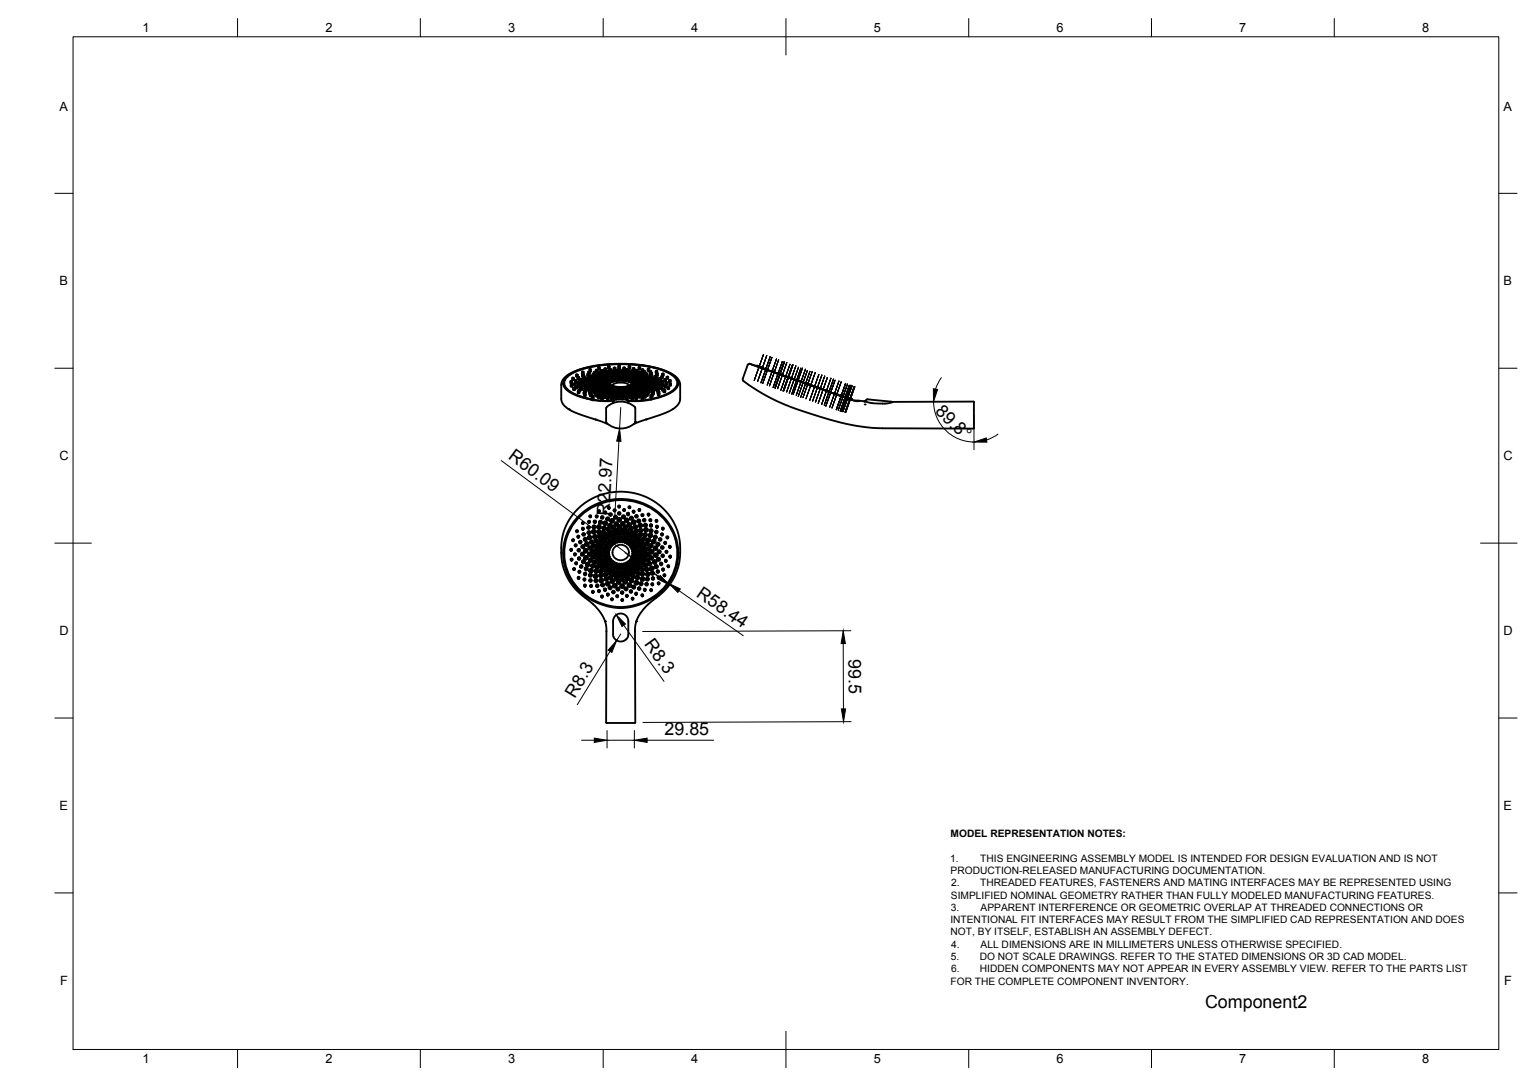
ISO-10303-21;
HEADER;
/* Generated by software containing ST-Developer
 * from STEP Tools, Inc. (www.steptools.com) 
 */

FILE_DESCRIPTION(
/* description */ ('STEP AP214'),
/* implementation_level */ '2;1');

FILE_NAME(
/* name */ 'Component2.step',
/* time_stamp */ '2026-10-06T11:02:40-07:00',
/* author */ (''),
/* organization */ (''),
/* preprocessor_version */ 'ST-DEVELOPER v20.2',
/* originating_system */ 'Autodesk Translation Framework v15.15.0.0',
/* authorisation */ '');

FILE_SCHEMA (('AUTOMOTIVE_DESIGN { 1 0 10303 214 3 1 1 }'));
ENDSEC;

DATA;
#10=MECHANICAL_DESIGN_GEOMETRIC_PRESENTATION_REPRESENTATION('',(#2937),#130910);
#45=B_SPLINE_SURFACE_WITH_KNOTS('',5,5,((#80582,#80583,#80584,#80585,#80586,
#80587),(#80588,#80589,#80590,#80591,#80592,#80593),(#80594,#80595,#80596,
#80597,#80598,#80599),(#80600,#80601,#80602,#80603,#80604,#80605),(#80606,
#80607,#80608,#80609,#80610,#80611),(#80612,#80613,#80614,#80615,#80616,
#80617),(#80618,#80619,#80620,#80621,#80622,#80623),(#80624,#80625,#80626,
#80627,#80628,#80629),(#80630,#80631,#80632,#80633,#80634,#80635),(#80636,
#80637,#80638,#80639,#80640,#80641),(#80642,#80643,#80644,#80645,#80646,
#80647),(#80648,#80649,#80650,#80651,#80652,#80653),(#80654,#80655,#80656,
#80657,#80658,#80659),(#80660,#80661,#80662,#80663,#80664,#80665),(#80666,
#80667,#80668,#80669,#80670,#80671),(#80672,#80673,#80674,#80675,#80676,
#80677),(#80678,#80679,#80680,#80681,#80682,#80683),(#80684,#80685,#80686,
#80687,#80688,#80689),(#80690,#80691,#80692,#80693,#80694,#80695),(#80696,
#80697,#80698,#80699,#80700,#80701),(#80702,#80703,#80704,#80705,#80706,
#80707),(#80708,#80709,#80710,#80711,#80712,#80713)),.UNSPECIFIED.,.F.,
 .F.,.F.,(6,4,4,4,4,6),(6,6),(0.,0.25,0.375,0.5,0.75,1.),(-5.17415755595432E-6,
1.),.UNSPECIFIED.);
#46=B_SPLINE_SURFACE_WITH_KNOTS('',5,5,((#80915,#80916,#80917,#80918,#80919,
#80920),(#80921,#80922,#80923,#80924,#80925,#80926),(#80927,#80928,#80929,
#80930,#80931,#80932),(#80933,#80934,#80935,#80936,#80937,#80938),(#80939,
#80940,#80941,#80942,#80943,#80944),(#80945,#80946,#80947,#80948,#80949,
#80950),(#80951,#80952,#80953,#80954,#80955,#80956),(#80957,#80958,#80959,
#80960,#80961,#80962),(#80963,#80964,#80965,#80966,#80967,#80968),(#80969,
#80970,#80971,#80972,#80973,#80974),(#80975,#80976,#80977,#80978,#80979,
#80980),(#80981,#80982,#80983,#80984,#80985,#80986),(#80987,#80988,#80989,
#80990,#80991,#80992),(#80993,#80994,#80995,#80996,#80997,#80998),(#80999,
#81000,#81001,#81002,#81003,#81004),(#81005,#81006,#81007,#81008,#81009,
#81010),(#81011,#81012,#81013,#81014,#81015,#81016),(#81017,#81018,#81019,
#81020,#81021,#81022),(#81023,#81024,#81025,#81026,#81027,#81028),(#81029,
#81030,#81031,#81032,#81033,#81034),(#81035,#81036,#81037,#81038,#81039,
#81040),(#81041,#81042,#81043,#81044,#81045,#81046)),.UNSPECIFIED.,.F.,
 .F.,.F.,(6,4,4,4,4,6),(6,6),(0.,0.25,0.5,0.625,0.75,1.),(-4.87729692394977E-6,
1.),.UNSPECIFIED.);
#47=B_SPLINE_SURFACE_WITH_KNOTS('',5,5,((#81337,#81338,#81339,#81340,#81341,
#81342),(#81343,#81344,#81345,#81346,#81347,#81348),(#81349,#81350,#81351,
#81352,#81353,#81354),(#81355,#81356,#81357,#81358,#81359,#81360),(#81361,
#81362,#81363,#81364,#81365,#81366),(#81367,#81368,#81369,#81370,#81371,
#81372),(#81373,#81374,#81375,#81376,#81377,#81378),(#81379,#81380,#81381,
#81382,#81383,#81384),(#81385,#81386,#81387,#81388,#81389,#81390),(#81391,
#81392,#81393,#81394,#81395,#81396),(#81397,#81398,#81399,#81400,#81401,
#81402),(#81403,#81404,#81405,#81406,#81407,#81408),(#81409,#81410,#81411,
#81412,#81413,#81414),(#81415,#81416,#81417,#81418,#81419,#81420),(#81421,
#81422,#81423,#81424,#81425,#81426),(#81427,#81428,#81429,#81430,#81431,
#81432),(#81433,#81434,#81435,#81436,#81437,#81438),(#81439,#81440,#81441,
#81442,#81443,#81444),(#81445,#81446,#81447,#81448,#81449,#81450),(#81451,
#81452,#81453,#81454,#81455,#81456),(#81457,#81458,#81459,#81460,#81461,
#81462),(#81463,#81464,#81465,#81466,#81467,#81468),(#81469,#81470,#81471,
#81472,#81473,#81474),(#81475,#81476,#81477,#81478,#81479,#81480),(#81481,
#81482,#81483,#81484,#81485,#81486),(#81487,#81488,#81489,#81490,#81491,
#81492),(#81493,#81494,#81495,#81496,#81497,#81498),(#81499,#81500,#81501,
#81502,#81503,#81504),(#81505,#81506,#81507,#81508,#81509,#81510),(#81511,
#81512,#81513,#81514,#81515,#81516),(#81517,#81518,#81519,#81520,#81521,
#81522),(#81523,#81524,#81525,#81526,#81527,#81528),(#81529,#81530,#81531,
#81532,#81533,#81534),(#81535,#81536,#81537,#81538,#81539,#81540),(#81541,
#81542,#81543,#81544,#81545,#81546),(#81547,#81548,#81549,#81550,#81551,
#81552),(#81553,#81554,#81555,#81556,#81557,#81558),(#81559,#81560,#81561,
#81562,#81563,#81564),(#81565,#81566,#81567,#81568,#81569,#81570),(#81571,
#81572,#81573,#81574,#81575,#81576),(#81577,#81578,#81579,#81580,#81581,
#81582),(#81583,#81584,#81585,#81586,#81587,#81588),(#81589,#81590,#81591,
#81592,#81593,#81594),(#81595,#81596,#81597,#81598,#81599,#81600),(#81601,
#81602,#81603,#81604,#81605,#81606),(#81607,#81608,#81609,#81610,#81611,
#81612)),.UNSPECIFIED.,.F.,.F.,.F.,(6,4,4,4,4,4,4,4,4,4,4,6),(6,6),(0.,
0.0625,0.125,0.25,0.3125,0.375,0.5,0.625,0.6875,0.75,0.875,1.),(0.,1.),
 .UNSPECIFIED.);
#48=B_SPLINE_SURFACE_WITH_KNOTS('',5,5,((#82412,#82413,#82414,#82415,#82416,
#82417),(#82418,#82419,#82420,#82421,#82422,#82423),(#82424,#82425,#82426,
#82427,#82428,#82429),(#82430,#82431,#82432,#82433,#82434,#82435),(#82436,
#82437,#82438,#82439,#82440,#82441),(#82442,#82443,#82444,#82445,#82446,
#82447),(#82448,#82449,#82450,#82451,#82452,#82453),(#82454,#82455,#82456,
#82457,#82458,#82459),(#82460,#82461,#82462,#82463,#82464,#82465),(#82466,
#82467,#82468,#82469,#82470,#82471)),.UNSPECIFIED.,.F.,.F.,.F.,(6,4,6),
(6,6),(0.,0.5,1.),(-3.3767936030343E-7,1.),.UNSPECIFIED.);
#49=B_SPLINE_SURFACE_WITH_KNOTS('',5,5,((#83493,#83494,#83495,#83496,#83497,
#83498),(#83499,#83500,#83501,#83502,#83503,#83504),(#83505,#83506,#83507,
#83508,#83509,#83510),(#83511,#83512,#83513,#83514,#83515,#83516),(#83517,
#83518,#83519,#83520,#83521,#83522),(#83523,#83524,#83525,#83526,#83527,
#83528),(#83529,#83530,#83531,#83532,#83533,#83534),(#83535,#83536,#83537,
#83538,#83539,#83540),(#83541,#83542,#83543,#83544,#83545,#83546),(#83547,
#83548,#83549,#83550,#83551,#83552)),.UNSPECIFIED.,.F.,.F.,.F.,(6,4,6),
(6,6),(0.,0.5,1.),(0.,1.),.UNSPECIFIED.);
#58=SPHERICAL_SURFACE('',#47449,40.9182954767619);
#59=SPHERICAL_SURFACE('',#47518,216.25);
#71=CONICAL_SURFACE('',#47414,8.99091713639496,1.30899693899566);
#72=CONICAL_SURFACE('',#47466,6.3031389659941,0.785398163397445);
#73=CONICAL_SURFACE('',#47469,6.3031389659941,0.785398163397445);
#74=CONICAL_SURFACE('',#47523,22.9751982564137,0.00349065850398867);
#75=CONICAL_SURFACE('',#47530,22.9751982564137,0.00349065850398867);
#83=FACE_BOUND('',#13544,.T.);
#84=FACE_BOUND('',#13545,.T.);
#85=FACE_BOUND('',#13546,.T.);
#86=FACE_BOUND('',#13547,.T.);
#87=FACE_BOUND('',#13548,.T.);
#88=FACE_BOUND('',#13549,.T.);
#89=FACE_BOUND('',#13550,.T.);
#90=FACE_BOUND('',#13551,.T.);
#91=FACE_BOUND('',#13552,.T.);
#92=FACE_BOUND('',#13553,.T.);
#93=FACE_BOUND('',#13554,.T.);
#94=FACE_BOUND('',#13555,.T.);
#95=FACE_BOUND('',#13556,.T.);
#96=FACE_BOUND('',#13557,.T.);
#97=FACE_BOUND('',#13558,.T.);
#98=FACE_BOUND('',#13559,.T.);
#99=FACE_BOUND('',#13560,.T.);
#100=FACE_BOUND('',#13561,.T.);
#101=FACE_BOUND('',#13562,.T.);
#102=FACE_BOUND('',#13563,.T.);
#103=FACE_BOUND('',#13564,.T.);
#104=FACE_BOUND('',#13565,.T.);
#105=FACE_BOUND('',#13566,.T.);
#106=FACE_BOUND('',#13567,.T.);
#107=FACE_BOUND('',#13568,.T.);
#108=FACE_BOUND('',#13569,.T.);
#109=FACE_BOUND('',#13570,.T.);
#110=FACE_BOUND('',#13571,.T.);
#111=FACE_BOUND('',#13572,.T.);
#112=FACE_BOUND('',#13573,.T.);
#113=FACE_BOUND('',#13574,.T.);
#114=FACE_BOUND('',#13575,.T.);
#115=FACE_BOUND('',#13576,.T.);
#116=FACE_BOUND('',#13577,.T.);
#117=FACE_BOUND('',#13578,.T.);
#118=FACE_BOUND('',#13579,.T.);
#119=FACE_BOUND('',#13580,.T.);
#120=FACE_BOUND('',#13581,.T.);
#121=FACE_BOUND('',#13582,.T.);
#122=FACE_BOUND('',#13583,.T.);
#123=FACE_BOUND('',#13584,.T.);
#124=FACE_BOUND('',#13585,.T.);
#125=FACE_BOUND('',#13586,.T.);
#126=FACE_BOUND('',#13587,.T.);
#127=FACE_BOUND('',#13588,.T.);
#128=FACE_BOUND('',#13589,.T.);
#129=FACE_BOUND('',#13590,.T.);
#130=FACE_BOUND('',#13591,.T.);
#131=FACE_BOUND('',#13605,.T.);
#132=FACE_BOUND('',#13670,.T.);
#133=FACE_BOUND('',#13671,.T.);
#134=FACE_BOUND('',#13672,.T.);
#135=FACE_BOUND('',#13673,.T.);
#136=FACE_BOUND('',#13674,.T.);
#137=FACE_BOUND('',#13675,.T.);
#138=FACE_BOUND('',#13676,.T.);
#139=FACE_BOUND('',#13677,.T.);
#140=FACE_BOUND('',#13678,.T.);
#141=FACE_BOUND('',#13679,.T.);
#142=FACE_BOUND('',#13680,.T.);
#143=FACE_BOUND('',#13681,.T.);
#144=FACE_BOUND('',#13682,.T.);
#145=FACE_BOUND('',#13683,.T.);
#146=FACE_BOUND('',#13684,.T.);
#147=FACE_BOUND('',#13685,.T.);
#148=FACE_BOUND('',#13686,.T.);
#149=FACE_BOUND('',#13687,.T.);
#150=FACE_BOUND('',#13689,.T.);
#151=FACE_BOUND('',#13690,.T.);
#152=FACE_BOUND('',#13691,.T.);
#153=FACE_BOUND('',#13692,.T.);
#154=FACE_BOUND('',#13693,.T.);
#155=FACE_BOUND('',#13694,.T.);
#156=FACE_BOUND('',#13695,.T.);
#157=FACE_BOUND('',#13696,.T.);
#158=FACE_BOUND('',#13697,.T.);
#159=FACE_BOUND('',#13698,.T.);
#160=FACE_BOUND('',#13699,.T.);
#161=FACE_BOUND('',#13700,.T.);
#162=FACE_BOUND('',#13701,.T.);
#163=FACE_BOUND('',#13702,.T.);
#164=FACE_BOUND('',#13703,.T.);
#165=FACE_BOUND('',#13704,.T.);
#166=FACE_BOUND('',#13705,.T.);
#167=FACE_BOUND('',#13706,.T.);
#168=FACE_BOUND('',#13707,.T.);
#169=FACE_BOUND('',#13708,.T.);
#170=FACE_BOUND('',#13709,.T.);
#171=FACE_BOUND('',#13710,.T.);
#172=FACE_BOUND('',#13711,.T.);
#173=FACE_BOUND('',#13712,.T.);
#174=FACE_BOUND('',#13713,.T.);
#175=FACE_BOUND('',#13714,.T.);
#176=FACE_BOUND('',#13715,.T.);
#177=FACE_BOUND('',#13716,.T.);
#178=FACE_BOUND('',#13717,.T.);
#179=FACE_BOUND('',#13718,.T.);
#180=FACE_BOUND('',#13719,.T.);
#181=FACE_BOUND('',#13720,.T.);
#182=FACE_BOUND('',#13721,.T.);
#183=FACE_BOUND('',#13722,.T.);
#184=FACE_BOUND('',#13723,.T.);
#185=FACE_BOUND('',#13724,.T.);
#186=FACE_BOUND('',#13725,.T.);
#187=FACE_BOUND('',#13726,.T.);
#188=FACE_BOUND('',#13727,.T.);
#189=FACE_BOUND('',#13728,.T.);
#190=FACE_BOUND('',#13729,.T.);
#191=FACE_BOUND('',#13730,.T.);
#192=FACE_BOUND('',#13731,.T.);
#193=FACE_BOUND('',#13732,.T.);
#194=FACE_BOUND('',#13733,.T.);
#195=FACE_BOUND('',#13734,.T.);
#196=FACE_BOUND('',#13735,.T.);
#197=FACE_BOUND('',#13736,.T.);
#198=FACE_BOUND('',#13737,.T.);
#199=FACE_BOUND('',#13738,.T.);
#200=FACE_BOUND('',#13739,.T.);
#201=FACE_BOUND('',#13740,.T.);
#202=FACE_BOUND('',#13741,.T.);
#203=FACE_BOUND('',#13742,.T.);
#204=FACE_BOUND('',#13743,.T.);
#205=FACE_BOUND('',#13744,.T.);
#206=FACE_BOUND('',#13745,.T.);
#207=FACE_BOUND('',#13746,.T.);
#208=FACE_BOUND('',#13747,.T.);
#209=FACE_BOUND('',#13748,.T.);
#210=FACE_BOUND('',#13749,.T.);
#211=FACE_BOUND('',#13750,.T.);
#212=FACE_BOUND('',#13751,.T.);
#213=FACE_BOUND('',#13752,.T.);
#214=FACE_BOUND('',#13753,.T.);
#215=FACE_BOUND('',#13754,.T.);
#216=FACE_BOUND('',#13755,.T.);
#217=FACE_BOUND('',#13756,.T.);
#218=FACE_BOUND('',#13757,.T.);
#219=FACE_BOUND('',#13758,.T.);
#220=FACE_BOUND('',#13759,.T.);
#221=FACE_BOUND('',#13760,.T.);
#222=FACE_BOUND('',#13761,.T.);
#223=FACE_BOUND('',#13762,.T.);
#224=FACE_BOUND('',#13763,.T.);
#225=FACE_BOUND('',#13764,.T.);
#226=FACE_BOUND('',#13765,.T.);
#227=FACE_BOUND('',#13766,.T.);
#228=FACE_BOUND('',#13767,.T.);
#229=FACE_BOUND('',#13768,.T.);
#230=FACE_BOUND('',#13769,.T.);
#231=FACE_BOUND('',#13770,.T.);
#232=FACE_BOUND('',#13771,.T.);
#233=FACE_BOUND('',#13772,.T.);
#234=FACE_BOUND('',#13773,.T.);
#235=FACE_BOUND('',#13774,.T.);
#236=FACE_BOUND('',#13775,.T.);
#237=FACE_BOUND('',#13776,.T.);
#238=FACE_BOUND('',#13777,.T.);
#239=FACE_BOUND('',#13778,.T.);
#240=FACE_BOUND('',#13779,.T.);
#241=FACE_BOUND('',#13780,.T.);
#242=FACE_BOUND('',#13781,.T.);
#243=FACE_BOUND('',#13782,.T.);
#244=FACE_BOUND('',#13783,.T.);
#245=FACE_BOUND('',#13784,.T.);
#246=FACE_BOUND('',#13785,.T.);
#247=FACE_BOUND('',#13786,.T.);
#248=FACE_BOUND('',#13787,.T.);
#249=FACE_BOUND('',#13788,.T.);
#250=FACE_BOUND('',#13789,.T.);
#251=FACE_BOUND('',#13790,.T.);
#252=FACE_BOUND('',#13791,.T.);
#253=FACE_BOUND('',#13792,.T.);
#254=FACE_BOUND('',#13793,.T.);
#255=FACE_BOUND('',#13794,.T.);
#256=FACE_BOUND('',#13795,.T.);
#257=FACE_BOUND('',#13796,.T.);
#258=FACE_BOUND('',#13797,.T.);
#259=FACE_BOUND('',#13798,.T.);
#260=FACE_BOUND('',#13799,.T.);
#261=FACE_BOUND('',#13800,.T.);
#262=FACE_BOUND('',#13801,.T.);
#263=FACE_BOUND('',#13802,.T.);
#264=FACE_BOUND('',#13803,.T.);
#265=FACE_BOUND('',#13804,.T.);
#266=FACE_BOUND('',#13805,.T.);
#267=FACE_BOUND('',#13806,.T.);
#268=FACE_BOUND('',#13807,.T.);
#269=FACE_BOUND('',#13808,.T.);
#270=FACE_BOUND('',#13809,.T.);
#271=FACE_BOUND('',#13810,.T.);
#272=FACE_BOUND('',#13811,.T.);
#273=FACE_BOUND('',#13812,.T.);
#274=FACE_BOUND('',#13813,.T.);
#275=FACE_BOUND('',#13814,.T.);
#276=FACE_BOUND('',#13815,.T.);
#277=FACE_BOUND('',#13816,.T.);
#278=FACE_BOUND('',#13817,.T.);
#279=FACE_BOUND('',#13818,.T.);
#280=FACE_BOUND('',#13819,.T.);
#281=FACE_BOUND('',#13820,.T.);
#282=FACE_BOUND('',#13821,.T.);
#283=FACE_BOUND('',#13822,.T.);
#284=FACE_BOUND('',#13823,.T.);
#285=FACE_BOUND('',#13824,.T.);
#286=FACE_BOUND('',#13825,.T.);
#287=FACE_BOUND('',#13826,.T.);
#288=FACE_BOUND('',#13827,.T.);
#289=FACE_BOUND('',#13828,.T.);
#290=FACE_BOUND('',#13829,.T.);
#291=FACE_BOUND('',#13830,.T.);
#292=FACE_BOUND('',#13831,.T.);
#293=FACE_BOUND('',#13832,.T.);
#294=FACE_BOUND('',#13833,.T.);
#295=FACE_BOUND('',#13834,.T.);
#296=FACE_BOUND('',#13835,.T.);
#297=FACE_BOUND('',#13836,.T.);
#298=FACE_BOUND('',#13837,.T.);
#299=FACE_BOUND('',#13838,.T.);
#300=FACE_BOUND('',#13839,.T.);
#301=FACE_BOUND('',#13840,.T.);
#302=FACE_BOUND('',#13841,.T.);
#303=FACE_BOUND('',#13842,.T.);
#304=FACE_BOUND('',#13843,.T.);
#305=FACE_BOUND('',#13844,.T.);
#306=FACE_BOUND('',#13845,.T.);
#307=FACE_BOUND('',#13846,.T.);
#308=FACE_BOUND('',#13847,.T.);
#309=FACE_BOUND('',#13848,.T.);
#310=FACE_BOUND('',#13849,.T.);
#311=FACE_BOUND('',#13850,.T.);
#312=FACE_BOUND('',#13851,.T.);
#313=FACE_BOUND('',#13852,.T.);
#314=FACE_BOUND('',#13853,.T.);
#315=FACE_BOUND('',#13854,.T.);
#316=FACE_BOUND('',#13855,.T.);
#317=FACE_BOUND('',#13856,.T.);
#318=FACE_BOUND('',#13857,.T.);
#319=FACE_BOUND('',#13858,.T.);
#320=FACE_BOUND('',#13859,.T.);
#321=FACE_BOUND('',#13860,.T.);
#322=FACE_BOUND('',#13861,.T.);
#323=FACE_BOUND('',#13862,.T.);
#324=FACE_BOUND('',#13863,.T.);
#325=FACE_BOUND('',#13864,.T.);
#326=FACE_BOUND('',#13865,.T.);
#327=FACE_BOUND('',#13866,.T.);
#328=FACE_BOUND('',#13867,.T.);
#329=FACE_BOUND('',#13868,.T.);
#330=FACE_BOUND('',#13869,.T.);
#331=FACE_BOUND('',#13870,.T.);
#332=FACE_BOUND('',#13871,.T.);
#333=FACE_BOUND('',#13872,.T.);
#334=FACE_BOUND('',#13873,.T.);
#335=FACE_BOUND('',#13874,.T.);
#336=FACE_BOUND('',#13875,.T.);
#337=FACE_BOUND('',#13876,.T.);
#338=FACE_BOUND('',#13877,.T.);
#339=FACE_BOUND('',#13878,.T.);
#340=FACE_BOUND('',#13879,.T.);
#341=FACE_BOUND('',#13880,.T.);
#342=FACE_BOUND('',#13881,.T.);
#343=FACE_BOUND('',#13882,.T.);
#344=FACE_BOUND('',#13883,.T.);
#345=FACE_BOUND('',#13884,.T.);
#346=FACE_BOUND('',#13885,.T.);
#347=FACE_BOUND('',#13886,.T.);
#348=FACE_BOUND('',#13887,.T.);
#349=FACE_BOUND('',#13888,.T.);
#350=FACE_BOUND('',#13889,.T.);
#351=FACE_BOUND('',#13890,.T.);
#352=FACE_BOUND('',#13891,.T.);
#353=FACE_BOUND('',#13892,.T.);
#354=FACE_BOUND('',#13893,.T.);
#355=FACE_BOUND('',#13894,.T.);
#356=FACE_BOUND('',#13895,.T.);
#357=FACE_BOUND('',#13896,.T.);
#358=FACE_BOUND('',#13897,.T.);
#359=FACE_BOUND('',#13898,.T.);
#360=FACE_BOUND('',#13899,.T.);
#361=FACE_BOUND('',#13900,.T.);
#362=FACE_BOUND('',#13901,.T.);
#363=FACE_BOUND('',#13902,.T.);
#364=FACE_BOUND('',#13903,.T.);
#365=FACE_BOUND('',#13904,.T.);
#366=FACE_BOUND('',#13905,.T.);
#367=FACE_BOUND('',#13906,.T.);
#368=FACE_BOUND('',#13907,.T.);
#369=FACE_BOUND('',#13908,.T.);
#370=FACE_BOUND('',#13909,.T.);
#371=FACE_BOUND('',#13910,.T.);
#372=FACE_BOUND('',#13911,.T.);
#373=FACE_BOUND('',#13912,.T.);
#374=FACE_BOUND('',#13913,.T.);
#375=FACE_BOUND('',#13914,.T.);
#376=FACE_BOUND('',#13915,.T.);
#377=FACE_BOUND('',#13916,.T.);
#378=FACE_BOUND('',#13917,.T.);
#379=FACE_BOUND('',#13918,.T.);
#380=FACE_BOUND('',#13919,.T.);
#381=FACE_BOUND('',#13920,.T.);
#382=FACE_BOUND('',#13921,.T.);
#383=FACE_BOUND('',#13922,.T.);
#384=FACE_BOUND('',#13923,.T.);
#385=FACE_BOUND('',#13924,.T.);
#386=FACE_BOUND('',#13933,.T.);
#387=FACE_BOUND('',#13936,.T.);
#388=FACE_BOUND('',#13939,.T.);
#389=FACE_BOUND('',#13942,.T.);
#390=FACE_BOUND('',#13945,.T.);
#391=FACE_BOUND('',#13948,.T.);
#392=FACE_BOUND('',#13951,.T.);
#393=FACE_BOUND('',#13954,.T.);
#394=FACE_BOUND('',#13957,.T.);
#395=FACE_BOUND('',#13960,.T.);
#396=FACE_BOUND('',#13963,.T.);
#397=FACE_BOUND('',#13966,.T.);
#398=FACE_BOUND('',#13969,.T.);
#399=FACE_BOUND('',#13972,.T.);
#400=FACE_BOUND('',#13975,.T.);
#401=FACE_BOUND('',#13978,.T.);
#402=FACE_BOUND('',#13981,.T.);
#403=FACE_BOUND('',#13984,.T.);
#404=FACE_BOUND('',#13987,.T.);
#405=FACE_BOUND('',#13990,.T.);
#406=FACE_BOUND('',#13993,.T.);
#407=FACE_BOUND('',#13996,.T.);
#408=FACE_BOUND('',#13999,.T.);
#409=FACE_BOUND('',#14002,.T.);
#410=FACE_BOUND('',#14005,.T.);
#411=FACE_BOUND('',#14008,.T.);
#412=FACE_BOUND('',#14011,.T.);
#413=FACE_BOUND('',#14014,.T.);
#414=FACE_BOUND('',#14017,.T.);
#415=FACE_BOUND('',#14020,.T.);
#416=FACE_BOUND('',#14023,.T.);
#417=FACE_BOUND('',#14026,.T.);
#418=FACE_BOUND('',#14029,.T.);
#419=FACE_BOUND('',#14032,.T.);
#420=FACE_BOUND('',#14035,.T.);
#421=FACE_BOUND('',#14038,.T.);
#422=FACE_BOUND('',#14041,.T.);
#423=FACE_BOUND('',#14044,.T.);
#424=FACE_BOUND('',#14047,.T.);
#425=FACE_BOUND('',#14050,.T.);
#426=FACE_BOUND('',#14053,.T.);
#427=FACE_BOUND('',#14056,.T.);
#428=FACE_BOUND('',#14059,.T.);
#429=FACE_BOUND('',#14062,.T.);
#430=FACE_BOUND('',#14065,.T.);
#431=FACE_BOUND('',#14068,.T.);
#432=FACE_BOUND('',#14071,.T.);
#433=FACE_BOUND('',#14074,.T.);
#434=FACE_BOUND('',#14077,.T.);
#435=FACE_BOUND('',#14080,.T.);
#436=FACE_BOUND('',#14083,.T.);
#437=FACE_BOUND('',#14086,.T.);
#438=FACE_BOUND('',#14089,.T.);
#439=FACE_BOUND('',#14092,.T.);
#440=FACE_BOUND('',#14095,.T.);
#441=FACE_BOUND('',#14098,.T.);
#442=FACE_BOUND('',#14101,.T.);
#443=FACE_BOUND('',#14104,.T.);
#444=FACE_BOUND('',#14107,.T.);
#445=FACE_BOUND('',#14110,.T.);
#446=FACE_BOUND('',#14113,.T.);
#447=FACE_BOUND('',#14116,.T.);
#448=FACE_BOUND('',#14119,.T.);
#449=FACE_BOUND('',#14122,.T.);
#450=FACE_BOUND('',#14125,.T.);
#451=FACE_BOUND('',#14128,.T.);
#452=FACE_BOUND('',#14131,.T.);
#453=FACE_BOUND('',#14134,.T.);
#454=FACE_BOUND('',#14137,.T.);
#455=FACE_BOUND('',#14140,.T.);
#456=FACE_BOUND('',#14143,.T.);
#457=FACE_BOUND('',#14146,.T.);
#458=FACE_BOUND('',#14149,.T.);
#459=FACE_BOUND('',#14152,.T.);
#460=FACE_BOUND('',#14155,.T.);
#461=FACE_BOUND('',#14158,.T.);
#462=FACE_BOUND('',#14161,.T.);
#463=FACE_BOUND('',#14164,.T.);
#464=FACE_BOUND('',#14167,.T.);
#465=FACE_BOUND('',#14170,.T.);
#466=FACE_BOUND('',#14173,.T.);
#467=FACE_BOUND('',#14176,.T.);
#468=FACE_BOUND('',#14179,.T.);
#469=FACE_BOUND('',#14182,.T.);
#470=FACE_BOUND('',#14185,.T.);
#471=FACE_BOUND('',#14188,.T.);
#472=FACE_BOUND('',#14191,.T.);
#473=FACE_BOUND('',#14194,.T.);
#474=FACE_BOUND('',#14197,.T.);
#475=FACE_BOUND('',#14200,.T.);
#476=FACE_BOUND('',#14203,.T.);
#477=FACE_BOUND('',#14206,.T.);
#478=FACE_BOUND('',#14209,.T.);
#479=FACE_BOUND('',#14212,.T.);
#480=FACE_BOUND('',#14215,.T.);
#481=FACE_BOUND('',#14218,.T.);
#482=FACE_BOUND('',#14221,.T.);
#483=FACE_BOUND('',#14224,.T.);
#484=FACE_BOUND('',#14227,.T.);
#485=FACE_BOUND('',#14230,.T.);
#486=FACE_BOUND('',#14233,.T.);
#487=FACE_BOUND('',#14236,.T.);
#488=FACE_BOUND('',#14239,.T.);
#489=FACE_BOUND('',#14242,.T.);
#490=FACE_BOUND('',#14245,.T.);
#491=FACE_BOUND('',#14248,.T.);
#492=FACE_BOUND('',#14251,.T.);
#493=FACE_BOUND('',#14254,.T.);
#494=FACE_BOUND('',#14257,.T.);
#495=FACE_BOUND('',#14260,.T.);
#496=FACE_BOUND('',#14263,.T.);
#497=FACE_BOUND('',#14266,.T.);
#498=FACE_BOUND('',#14269,.T.);
#499=FACE_BOUND('',#14272,.T.);
#500=FACE_BOUND('',#14275,.T.);
#501=FACE_BOUND('',#14278,.T.);
#502=FACE_BOUND('',#14281,.T.);
#503=FACE_BOUND('',#14284,.T.);
#504=FACE_BOUND('',#14287,.T.);
#505=FACE_BOUND('',#14290,.T.);
#506=FACE_BOUND('',#14293,.T.);
#507=FACE_BOUND('',#14296,.T.);
#508=FACE_BOUND('',#14299,.T.);
#509=FACE_BOUND('',#14302,.T.);
#510=FACE_BOUND('',#14305,.T.);
#511=FACE_BOUND('',#14308,.T.);
#512=FACE_BOUND('',#14311,.T.);
#513=FACE_BOUND('',#14314,.T.);
#514=FACE_BOUND('',#14317,.T.);
#515=FACE_BOUND('',#14320,.T.);
#516=FACE_BOUND('',#14323,.T.);
#517=FACE_BOUND('',#14326,.T.);
#518=FACE_BOUND('',#14329,.T.);
#519=FACE_BOUND('',#14332,.T.);
#520=FACE_BOUND('',#14335,.T.);
#521=FACE_BOUND('',#14338,.T.);
#522=FACE_BOUND('',#14341,.T.);
#523=FACE_BOUND('',#14344,.T.);
#524=FACE_BOUND('',#14347,.T.);
#525=FACE_BOUND('',#14350,.T.);
#526=FACE_BOUND('',#14353,.T.);
#527=FACE_BOUND('',#14356,.T.);
#528=FACE_BOUND('',#14359,.T.);
#529=FACE_BOUND('',#14362,.T.);
#530=FACE_BOUND('',#14365,.T.);
#531=FACE_BOUND('',#14368,.T.);
#532=FACE_BOUND('',#14371,.T.);
#533=FACE_BOUND('',#14374,.T.);
#534=FACE_BOUND('',#14377,.T.);
#535=FACE_BOUND('',#14380,.T.);
#536=FACE_BOUND('',#14383,.T.);
#537=FACE_BOUND('',#14386,.T.);
#538=FACE_BOUND('',#14389,.T.);
#539=FACE_BOUND('',#14392,.T.);
#540=FACE_BOUND('',#14395,.T.);
#541=FACE_BOUND('',#14398,.T.);
#542=FACE_BOUND('',#14401,.T.);
#543=FACE_BOUND('',#14404,.T.);
#544=FACE_BOUND('',#14407,.T.);
#545=FACE_BOUND('',#14410,.T.);
#546=FACE_BOUND('',#14413,.T.);
#547=FACE_BOUND('',#14416,.T.);
#548=FACE_BOUND('',#14419,.T.);
#549=FACE_BOUND('',#14422,.T.);
#550=FACE_BOUND('',#14425,.T.);
#551=FACE_BOUND('',#14428,.T.);
#552=FACE_BOUND('',#14431,.T.);
#553=FACE_BOUND('',#14434,.T.);
#554=FACE_BOUND('',#14437,.T.);
#555=FACE_BOUND('',#14440,.T.);
#556=FACE_BOUND('',#14443,.T.);
#557=FACE_BOUND('',#14446,.T.);
#558=FACE_BOUND('',#14449,.T.);
#559=FACE_BOUND('',#14452,.T.);
#560=FACE_BOUND('',#14455,.T.);
#561=FACE_BOUND('',#14458,.T.);
#562=FACE_BOUND('',#14461,.T.);
#563=FACE_BOUND('',#14464,.T.);
#564=FACE_BOUND('',#14467,.T.);
#565=FACE_BOUND('',#14470,.T.);
#566=FACE_BOUND('',#14473,.T.);
#567=FACE_BOUND('',#14476,.T.);
#568=FACE_BOUND('',#14479,.T.);
#569=FACE_BOUND('',#14482,.T.);
#570=FACE_BOUND('',#14485,.T.);
#571=FACE_BOUND('',#14488,.T.);
#572=FACE_BOUND('',#14491,.T.);
#573=FACE_BOUND('',#14494,.T.);
#574=FACE_BOUND('',#14497,.T.);
#575=FACE_BOUND('',#14500,.T.);
#576=FACE_BOUND('',#14503,.T.);
#577=FACE_BOUND('',#14506,.T.);
#578=FACE_BOUND('',#14509,.T.);
#579=FACE_BOUND('',#14512,.T.);
#580=FACE_BOUND('',#14515,.T.);
#581=FACE_BOUND('',#14518,.T.);
#582=FACE_BOUND('',#14521,.T.);
#583=FACE_BOUND('',#14524,.T.);
#584=FACE_BOUND('',#14527,.T.);
#585=FACE_BOUND('',#14530,.T.);
#586=FACE_BOUND('',#14533,.T.);
#587=FACE_BOUND('',#14536,.T.);
#588=FACE_BOUND('',#14539,.T.);
#589=FACE_BOUND('',#14542,.T.);
#590=FACE_BOUND('',#14545,.T.);
#591=FACE_BOUND('',#14548,.T.);
#592=FACE_BOUND('',#14551,.T.);
#593=FACE_BOUND('',#14554,.T.);
#594=FACE_BOUND('',#14557,.T.);
#595=FACE_BOUND('',#14560,.T.);
#596=FACE_BOUND('',#14563,.T.);
#597=FACE_BOUND('',#14566,.T.);
#598=FACE_BOUND('',#14569,.T.);
#599=FACE_BOUND('',#14572,.T.);
#600=FACE_BOUND('',#14575,.T.);
#601=FACE_BOUND('',#14578,.T.);
#602=FACE_BOUND('',#14581,.T.);
#603=FACE_BOUND('',#14584,.T.);
#604=FACE_BOUND('',#14587,.T.);
#605=FACE_BOUND('',#14590,.T.);
#606=FACE_BOUND('',#14593,.T.);
#607=FACE_BOUND('',#14596,.T.);
#608=FACE_BOUND('',#14599,.T.);
#609=FACE_BOUND('',#14602,.T.);
#610=FACE_BOUND('',#14605,.T.);
#611=FACE_BOUND('',#14608,.T.);
#612=FACE_BOUND('',#14611,.T.);
#613=FACE_BOUND('',#14614,.T.);
#614=FACE_BOUND('',#14617,.T.);
#615=FACE_BOUND('',#14620,.T.);
#616=FACE_BOUND('',#14623,.T.);
#617=FACE_BOUND('',#14626,.T.);
#618=FACE_BOUND('',#14629,.T.);
#619=FACE_BOUND('',#14632,.T.);
#620=FACE_BOUND('',#14635,.T.);
#621=FACE_BOUND('',#14638,.T.);
#622=FACE_BOUND('',#14641,.T.);
#623=FACE_BOUND('',#14644,.T.);
#624=FACE_BOUND('',#14647,.T.);
#625=FACE_BOUND('',#14650,.T.);
#626=FACE_BOUND('',#14653,.T.);
#627=FACE_BOUND('',#14656,.T.);
#628=FACE_BOUND('',#14659,.T.);
#629=FACE_BOUND('',#14662,.T.);
#630=FACE_BOUND('',#14665,.T.);
#631=FACE_BOUND('',#14668,.T.);
#632=FACE_BOUND('',#14671,.T.);
#633=FACE_BOUND('',#14674,.T.);
#634=FACE_BOUND('',#14677,.T.);
#635=FACE_BOUND('',#14680,.T.);
#636=FACE_BOUND('',#14683,.T.);
#637=FACE_BOUND('',#14686,.T.);
#638=FACE_BOUND('',#14689,.T.);
#639=FACE_BOUND('',#14692,.T.);
#640=FACE_BOUND('',#14695,.T.);
#641=FACE_BOUND('',#14698,.T.);
#642=FACE_BOUND('',#14701,.T.);
#643=FACE_BOUND('',#14704,.T.);
#644=FACE_BOUND('',#14707,.T.);
#645=FACE_BOUND('',#14710,.T.);
#646=FACE_BOUND('',#14713,.T.);
#647=FACE_BOUND('',#14716,.T.);
#648=FACE_BOUND('',#14719,.T.);
#649=FACE_BOUND('',#14722,.T.);
#650=FACE_BOUND('',#14725,.T.);
#651=FACE_BOUND('',#14728,.T.);
#652=FACE_BOUND('',#14731,.T.);
#653=FACE_BOUND('',#14734,.T.);
#654=FACE_BOUND('',#14737,.T.);
#655=FACE_BOUND('',#14740,.T.);
#656=FACE_BOUND('',#14743,.T.);
#657=FACE_BOUND('',#14746,.T.);
#658=FACE_BOUND('',#14749,.T.);
#659=FACE_BOUND('',#14752,.T.);
#660=FACE_BOUND('',#14755,.T.);
#661=FACE_BOUND('',#14758,.T.);
#662=FACE_BOUND('',#14761,.T.);
#663=FACE_BOUND('',#14764,.T.);
#664=FACE_BOUND('',#14767,.T.);
#665=FACE_BOUND('',#14770,.T.);
#666=FACE_BOUND('',#14773,.T.);
#667=FACE_BOUND('',#14776,.T.);
#668=FACE_BOUND('',#14779,.T.);
#669=FACE_BOUND('',#14782,.T.);
#670=FACE_BOUND('',#14785,.T.);
#671=FACE_BOUND('',#14788,.T.);
#672=FACE_BOUND('',#14791,.T.);
#673=FACE_BOUND('',#14794,.T.);
#674=FACE_BOUND('',#14797,.T.);
#675=FACE_BOUND('',#14800,.T.);
#676=FACE_BOUND('',#14803,.T.);
#677=FACE_BOUND('',#14806,.T.);
#678=FACE_BOUND('',#14809,.T.);
#679=FACE_BOUND('',#14812,.T.);
#680=FACE_BOUND('',#14815,.T.);
#681=FACE_BOUND('',#14818,.T.);
#682=FACE_BOUND('',#14821,.T.);
#683=FACE_BOUND('',#14824,.T.);
#684=FACE_BOUND('',#14827,.T.);
#685=FACE_BOUND('',#14830,.T.);
#686=FACE_BOUND('',#14833,.T.);
#687=FACE_BOUND('',#14836,.T.);
#688=FACE_BOUND('',#14839,.T.);
#689=FACE_BOUND('',#14842,.T.);
#690=FACE_BOUND('',#14845,.T.);
#691=FACE_BOUND('',#14848,.T.);
#692=FACE_BOUND('',#14851,.T.);
#693=FACE_BOUND('',#14854,.T.);
#694=FACE_BOUND('',#14857,.T.);
#695=FACE_BOUND('',#14860,.T.);
#696=FACE_BOUND('',#14863,.T.);
#697=FACE_BOUND('',#14866,.T.);
#698=FACE_BOUND('',#14869,.T.);
#699=FACE_BOUND('',#14872,.T.);
#700=FACE_BOUND('',#14875,.T.);
#701=FACE_BOUND('',#14878,.T.);
#702=FACE_BOUND('',#14881,.T.);
#703=FACE_BOUND('',#14884,.T.);
#704=FACE_BOUND('',#14887,.T.);
#705=FACE_BOUND('',#14890,.T.);
#706=FACE_BOUND('',#14893,.T.);
#707=FACE_BOUND('',#14896,.T.);
#708=FACE_BOUND('',#14899,.T.);
#709=FACE_BOUND('',#14901,.T.);
#710=FACE_BOUND('',#14904,.T.);
#711=FACE_BOUND('',#14907,.T.);
#712=FACE_BOUND('',#14910,.T.);
#713=FACE_BOUND('',#14913,.T.);
#714=FACE_BOUND('',#14916,.T.);
#1517=(
BOUNDED_SURFACE()
B_SPLINE_SURFACE(2,2,((#77343,#77344,#77345,#77346,#77347,#77348,#77349,
#77350,#77351),(#77352,#77353,#77354,#77355,#77356,#77357,#77358,#77359,
#77360),(#77361,#77362,#77363,#77364,#77365,#77366,#77367,#77368,#77369)),
 .UNSPECIFIED.,.F.,.F.,.F.)
B_SPLINE_SURFACE_WITH_KNOTS((3,3),(3,2,2,2,3),(1.3311777581657,1.5707963267949),
(-2.52686466384705,-1.26345162727942,-3.85907117990136E-5,1.26337444585582,
2.52678748242345),.UNSPECIFIED.)
GEOMETRIC_REPRESENTATION_ITEM()
RATIONAL_B_SPLINE_SURFACE(((1.,0.807020945928444,1.,0.807020945928444,1.,
0.807020945928444,1.,0.807020945928444,1.),(0.992831448793889,0.801235774953152,
0.992831448793889,0.801235774953152,0.992831448793889,0.801235774953152,
0.992831448793889,0.801235774953152,0.992831448793889),(1.,0.807020945928444,
1.,0.807020945928444,1.,0.807020945928444,1.,0.807020945928444,1.)))
REPRESENTATION_ITEM('')
SURFACE()
);
#1518=(
BOUNDED_SURFACE()
B_SPLINE_SURFACE(2,3,((#77987,#77988,#77989,#77990),(#77991,#77992,#77993,
#77994),(#77995,#77996,#77997,#77998)),.UNSPECIFIED.,.F.,.F.,.F.)
B_SPLINE_SURFACE_WITH_KNOTS((3,3),(4,4),(0.122256864728636,0.285813497577799),
(0.,1.),.UNSPECIFIED.)
GEOMETRIC_REPRESENTATION_ITEM()
RATIONAL_B_SPLINE_SURFACE(((1.,0.999857188395218,0.999857188395218,1.),
(1.,0.999857188395218,0.999857188395218,1.),(1.,0.999857188395218,0.999857188395218,
1.)))
REPRESENTATION_ITEM('')
SURFACE()
);
#1519=(
BOUNDED_SURFACE()
B_SPLINE_SURFACE(3,2,((#78330,#78331,#78332),(#78333,#78334,#78335),(#78336,
#78337,#78338),(#78339,#78340,#78341),(#78342,#78343,#78344),(#78345,#78346,
#78347),(#78348,#78349,#78350),(#78351,#78352,#78353)),.UNSPECIFIED.,.F.,
 .F.,.F.)
B_SPLINE_SURFACE_WITH_KNOTS((4,2,2,4),(3,3),(-0.000825561057166025,0.00287128254447656,
0.00574256508895301,0.012310691235072),(0.,1.00082556105717),
 .UNSPECIFIED.)
GEOMETRIC_REPRESENTATION_ITEM()
RATIONAL_B_SPLINE_SURFACE(((1.,0.548378337711978,1.00074568251392),(1.,
0.548355519536473,1.00074572018951),(1.,0.548039556019421,1.00074624188386),
(1.,0.550338775294527,1.00074244559207),(1.,0.552341143417591,1.00073913943778),
(1.,0.563047839052552,1.00072146137585),(1.,0.577111435906181,1.00069824066007),
(1.,0.593159390799436,1.00067174352686)))
REPRESENTATION_ITEM('')
SURFACE()
);
#1520=(
BOUNDED_SURFACE()
B_SPLINE_SURFACE(3,2,((#78409,#78410,#78411),(#78412,#78413,#78414),(#78415,
#78416,#78417),(#78418,#78419,#78420),(#78421,#78422,#78423),(#78424,#78425,
#78426),(#78427,#78428,#78429),(#78430,#78431,#78432),(#78433,#78434,#78435),
(#78436,#78437,#78438),(#78439,#78440,#78441),(#78442,#78443,#78444),(#78445,
#78446,#78447),(#78448,#78449,#78450),(#78451,#78452,#78453),(#78454,#78455,
#78456),(#78457,#78458,#78459),(#78460,#78461,#78462),(#78463,#78464,#78465),
(#78466,#78467,#78468),(#78469,#78470,#78471),(#78472,#78473,#78474),(#78475,
#78476,#78477),(#78478,#78479,#78480),(#78481,#78482,#78483),(#78484,#78485,
#78486),(#78487,#78488,#78489),(#78490,#78491,#78492),(#78493,#78494,#78495),
(#78496,#78497,#78498),(#78499,#78500,#78501),(#78502,#78503,#78504),(#78505,
#78506,#78507),(#78508,#78509,#78510),(#78511,#78512,#78513),(#78514,#78515,
#78516),(#78517,#78518,#78519),(#78520,#78521,#78522),(#78523,#78524,#78525),
(#78526,#78527,#78528),(#78529,#78530,#78531),(#78532,#78533,#78534),(#78535,
#78536,#78537),(#78538,#78539,#78540),(#78541,#78542,#78543),(#78544,#78545,
#78546),(#78547,#78548,#78549),(#78550,#78551,#78552),(#78553,#78554,#78555),
(#78556,#78557,#78558)),.UNSPECIFIED.,.F.,.F.,.F.)
B_SPLINE_SURFACE_WITH_KNOTS((4,2,2,2,2,2,2,2,2,2,2,2,2,2,2,2,2,2,2,2,2,
2,2,2,4),(3,3),(-8.67361737988404E-19,0.00173990906147062,0.00260986359220593,
0.00347981812294124,0.00521972718441186,0.00608968171514717,0.00695963624588248,
0.00869954530735309,0.0095694998380884,0.0104394543688237,0.011309408899559,
0.0121793634302943,0.013919272491765,0.0147892270225003,0.0156591815532356,
0.0173990906147062,0.0182690451454415,0.0191389996761768,0.0200089542069121,
0.0208789087376474,0.022618817799118,0.0234887723298534,0.0243587268605887,
0.0260986359220593,0.0278385449835299),(0.,1.),.UNSPECIFIED.)
GEOMETRIC_REPRESENTATION_ITEM()
RATIONAL_B_SPLINE_SURFACE(((1.,0.587551834406292,1.),(1.,0.594699344437623,
1.),(1.,0.60382457287242,1.),(1.,0.618585716818677,1.),(1.,0.623688783259158,
1.),(1.,0.63402443640501,1.),(1.,0.639270861094579,1.),(1.,0.654612725815785,
1.),(1.,0.664393776262156,1.),(1.,0.677891309661685,1.),(1.,0.682215510713266,
1.),(1.,0.690382450875376,1.),(1.,0.694194502561824,1.),(1.,0.70485633352738,
1.),(1.,0.710933841358089,1.),(1.,0.718683431814466,1.),(1.,0.721040520492153,
1.),(1.,0.72523171526594,1.),(1.,0.727081934015882,1.),(1.,0.730342541173125,
1.),(1.,0.731752928390573,1.),(1.,0.734165338317436,1.),(1.,0.735170559598651,
1.),(1.,0.73756891973958,1.),(1.,0.738337302433501,1.),(1.,0.738350513419653,
1.),(1.,0.738161957403833,1.),(1.,0.737381790844921,1.),(1.,0.736790346153837,
1.),(1.,0.734428150437933,1.),(1.,0.732073793565705,1.),(1.,0.727166869065942,
1.),(1.,0.72528892033234,1.),(1.,0.721100474370705,1.),(1.,0.718783894149779,
1.),(1.,0.713670637512177,1.),(1.,0.710873855381012,1.),(1.,0.704754666210018,
1.),(1.,0.701414681407374,1.),(1.,0.690657616069657,1.),(1.,0.682568234525227,
1.),(1.,0.66911478968892,1.),(1.,0.664412058412855,1.),(1.,0.654618386970392,
1.),(1.,0.64955633063672,1.),(1.,0.634259701134918,1.),(1.,0.623798684793027,
1.),(1.,0.603998854527123,1.),(1.,0.594654550866798,1.),(1.,0.587551863023681,
1.)))
REPRESENTATION_ITEM('')
SURFACE()
);
#1521=(
BOUNDED_SURFACE()
B_SPLINE_SURFACE(3,2,((#78907,#78908,#78909),(#78910,#78911,#78912),(#78913,
#78914,#78915),(#78916,#78917,#78918),(#78919,#78920,#78921),(#78922,#78923,
#78924),(#78925,#78926,#78927),(#78928,#78929,#78930)),.UNSPECIFIED.,.F.,
 .F.,.F.)
B_SPLINE_SURFACE_WITH_KNOTS((4,2,2,4),(3,3),(-0.000839894778808834,0.00577703258153561,
0.00866554887230341,0.0123250319154216),(0.,1.00083989477881),
 .UNSPECIFIED.)
GEOMETRIC_REPRESENTATION_ITEM()
RATIONAL_B_SPLINE_SURFACE(((1.,0.59326054090623,1.00068323669606),(1.,0.577077765226871,
1.00071042035366),(1.,0.562913931262478,1.00073421261405),(1.,0.552227354080058,
1.0007521638148),(1.,0.550251225165873,1.00075548329552),(1.,0.548035546079893,
1.00075920517011),(1.,0.548356794981543,1.00075866553956),(1.,0.548365499452713,
1.00075865091788)))
REPRESENTATION_ITEM('')
SURFACE()
);
#1522=(
BOUNDED_SURFACE()
B_SPLINE_SURFACE(3,2,((#79061,#79062,#79063),(#79064,#79065,#79066),(#79067,
#79068,#79069),(#79070,#79071,#79072)),.UNSPECIFIED.,.F.,.F.,.F.)
B_SPLINE_SURFACE_WITH_KNOTS((4,4),(3,3),(0.,0.00312507179263297),(0.,1.),
 .UNSPECIFIED.)
GEOMETRIC_REPRESENTATION_ITEM()
RATIONAL_B_SPLINE_SURFACE(((1.,0.705667563680649,1.),(1.,0.683141011037701,
1.),(1.,0.667195074226265,1.),(1.,0.657315835427036,1.)))
REPRESENTATION_ITEM('')
SURFACE()
);
#1523=(
BOUNDED_SURFACE()
B_SPLINE_SURFACE(3,2,((#79086,#79087,#79088),(#79089,#79090,#79091),(#79092,
#79093,#79094),(#79095,#79096,#79097),(#79098,#79099,#79100),(#79101,#79102,
#79103),(#79104,#79105,#79106),(#79107,#79108,#79109),(#79110,#79111,#79112),
(#79113,#79114,#79115),(#79116,#79117,#79118),(#79119,#79120,#79121),(#79122,
#79123,#79124),(#79125,#79126,#79127),(#79128,#79129,#79130),(#79131,#79132,
#79133),(#79134,#79135,#79136),(#79137,#79138,#79139),(#79140,#79141,#79142),
(#79143,#79144,#79145),(#79146,#79147,#79148),(#79149,#79150,#79151),(#79152,
#79153,#79154),(#79155,#79156,#79157),(#79158,#79159,#79160),(#79161,#79162,
#79163),(#79164,#79165,#79166),(#79167,#79168,#79169),(#79170,#79171,#79172),
(#79173,#79174,#79175),(#79176,#79177,#79178),(#79179,#79180,#79181),(#79182,
#79183,#79184),(#79185,#79186,#79187),(#79188,#79189,#79190),(#79191,#79192,
#79193),(#79194,#79195,#79196),(#79197,#79198,#79199)),.UNSPECIFIED.,.F.,
 .F.,.F.)
B_SPLINE_SURFACE_WITH_KNOTS((4,2,2,2,2,2,2,2,2,2,2,2,2,2,2,2,2,2,4),(3,
3),(0.177629622043919,0.182227008052906,0.186824394061894,0.191421780070882,
0.19601916607987,0.200616552088858,0.205213938097846,0.209811324106834,
0.212110017111328,0.214408710115822,0.21900609612481,0.223603482133797,
0.228200868142785,0.230499561147279,0.232798254151773,0.237395640160761,
0.241993026169749,0.246590412178737,0.251187798187725),(-0.0011272803117177,
1.),.UNSPECIFIED.)
GEOMETRIC_REPRESENTATION_ITEM()
RATIONAL_B_SPLINE_SURFACE(((1.00066433836603,0.705335771802172,1.),(1.0006672369253,
0.704050129161315,1.),(1.00067174234902,0.702051769185273,1.),(1.00067937529164,
0.698666212576715,1.),(1.00068246888629,0.697294062890189,1.),(1.00068363404296,
0.696777263006209,1.),(1.00068168398229,0.697642203450054,1.),(1.00067057469206,
0.702569678060129,1.),(1.0006614418033,0.706620528884515,1.),(1.00063696614129,
0.717476596249883,1.),(1.0006216381699,0.724275247496527,1.),(1.00058883922152,
0.738823070267793,1.),(1.00057145082916,0.746535611763709,1.),(1.00054028106102,
0.760360819129251,1.),(1.00052657168104,0.766441551595995,1.),(1.00051230540889,
0.772769291024644,1.),(1.00050858517592,0.774419383257745,1.),(1.00050358230416,
0.776638384027486,1.),(1.00050231593974,0.777200074144778,1.),(1.00050237161857,
0.777175378053496,1.),(1.00050761438758,0.774849971960635,1.),(1.00052653204965,
0.766459129919287,1.),(1.00054018535901,0.760403267317986,1.),(1.00057139341204,
0.746561078861873,1.),(1.00058887691054,0.738806353479752,1.),(1.00061367660858,
0.727806561420185,1.),(1.00062171490961,0.724241209950337,1.),(1.00063661263986,
0.717633390187928,1.),(1.0006434784523,0.714588090641112,1.),(1.00066174186374,
0.706487438457221,1.),(1.00067070720977,0.702510900441748,1.),(1.00068161675471,
0.69767202193592,1.),(1.00068360383072,0.696790663504269,1.),(1.00068252855983,
0.697267594964546,1.),(1.00067947813414,0.698620597255677,1.),(1.00067181783581,
0.702018287367237,1.),(1.00066724002584,0.704048753932027,1.),(1.00066433837343,
0.705335768520302,1.)))
REPRESENTATION_ITEM('')
SURFACE()
);
#1524=(
BOUNDED_SURFACE()
B_SPLINE_SURFACE(3,2,((#79482,#79483,#79484),(#79485,#79486,#79487),(#79488,
#79489,#79490),(#79491,#79492,#79493)),.UNSPECIFIED.,.F.,.F.,.F.)
B_SPLINE_SURFACE_WITH_KNOTS((4,4),(3,3),(-2.75071984392645E-5,0.00458060955690249),
(0.,1.),.UNSPECIFIED.)
GEOMETRIC_REPRESENTATION_ITEM()
RATIONAL_B_SPLINE_SURFACE(((1.,0.641978469944238,1.),(1.,0.641650471821333,
1.),(1.,0.64244455436399,1.),(1.,0.657315835410222,1.)))
REPRESENTATION_ITEM('')
SURFACE()
);
#1525=(
BOUNDED_SURFACE()
B_SPLINE_SURFACE(3,2,((#79501,#79502,#79503),(#79504,#79505,#79506),(#79507,
#79508,#79509),(#79510,#79511,#79512)),.UNSPECIFIED.,.F.,.F.,.F.)
B_SPLINE_SURFACE_WITH_KNOTS((4,4),(3,3),(-2.46898855527089E-13,0.00312495174925659),
(0.,1.),.UNSPECIFIED.)
GEOMETRIC_REPRESENTATION_ITEM()
RATIONAL_B_SPLINE_SURFACE(((1.,0.657316968304524,1.),(1.,0.667197332814039,
1.),(1.,0.683144406660839,1.),(1.,0.7056675669599,1.)))
REPRESENTATION_ITEM('')
SURFACE()
);
#1526=(
BOUNDED_SURFACE()
B_SPLINE_SURFACE(3,2,((#79523,#79524,#79525),(#79526,#79527,#79528),(#79529,
#79530,#79531),(#79532,#79533,#79534)),.UNSPECIFIED.,.F.,.F.,.F.)
B_SPLINE_SURFACE_WITH_KNOTS((4,4),(3,3),(-2.7488975911652E-5,0.00458149598527533),
(0.,1.),.UNSPECIFIED.)
GEOMETRIC_REPRESENTATION_ITEM()
RATIONAL_B_SPLINE_SURFACE(((1.,0.641978587954326,1.),(1.,0.641650294890703,
1.),(1.,0.642442143358719,1.),(1.,0.657316968289027,1.)))
REPRESENTATION_ITEM('')
SURFACE()
);
#1527=(
BOUNDED_SURFACE()
B_SPLINE_SURFACE(3,2,((#79542,#79543,#79544),(#79545,#79546,#79547),(#79548,
#79549,#79550),(#79551,#79552,#79553),(#79554,#79555,#79556),(#79557,#79558,
#79559),(#79560,#79561,#79562),(#79563,#79564,#79565)),.UNSPECIFIED.,.F.,
 .F.,.F.)
B_SPLINE_SURFACE_WITH_KNOTS((4,2,2,4),(3,3),(0.,0.000314760444717589,0.000629520889435179,
0.00125904177887036),(0.,1.),.UNSPECIFIED.)
GEOMETRIC_REPRESENTATION_ITEM()
RATIONAL_B_SPLINE_SURFACE(((1.,0.705871570678672,1.),(1.,0.705832198773769,
1.),(1.,0.705802677875688,1.),(1.,0.705762810535011,1.),(1.,0.705752530546662,
1.),(1.,0.705752443860712,1.),(1.,0.705792484302677,1.),(1.,0.705871570678672,
1.)))
REPRESENTATION_ITEM('')
SURFACE()
);
#1528=(
BOUNDED_SURFACE()
B_SPLINE_SURFACE(3,2,((#79592,#79593,#79594),(#79595,#79596,#79597),(#79598,
#79599,#79600),(#79601,#79602,#79603),(#79604,#79605,#79606),(#79607,#79608,
#79609),(#79610,#79611,#79612),(#79613,#79614,#79615)),.UNSPECIFIED.,.F.,
 .F.,.F.)
B_SPLINE_SURFACE_WITH_KNOTS((4,2,2,4),(3,3),(0.,0.000314760444717589,0.000629520889435178,
0.00125904177887036),(0.,1.),.UNSPECIFIED.)
GEOMETRIC_REPRESENTATION_ITEM()
RATIONAL_B_SPLINE_SURFACE(((1.,0.705871570678664,1.),(1.,0.705832198778323,
1.),(1.,0.705802677887727,1.),(1.,0.705762810539017,1.),(1.,0.705752530546526,
1.),(1.,0.705752443861208,1.),(1.,0.705792484282721,1.),(1.,0.705871570678672,
1.)))
REPRESENTATION_ITEM('')
SURFACE()
);
#1529=(
BOUNDED_SURFACE()
B_SPLINE_SURFACE(3,2,((#79636,#79637,#79638),(#79639,#79640,#79641),(#79642,
#79643,#79644),(#79645,#79646,#79647),(#79648,#79649,#79650),(#79651,#79652,
#79653),(#79654,#79655,#79656),(#79657,#79658,#79659)),.UNSPECIFIED.,.F.,
 .F.,.F.)
B_SPLINE_SURFACE_WITH_KNOTS((4,2,2,4),(3,3),(0.,0.000314760444717595,0.000629520889435189,
0.00125904177887038),(0.,1.),.UNSPECIFIED.)
GEOMETRIC_REPRESENTATION_ITEM()
RATIONAL_B_SPLINE_SURFACE(((1.,0.705871570678672,1.),(1.,0.705832198778314,
1.),(1.,0.705802677887727,1.),(1.,0.705762810539017,1.),(1.,0.705752530546536,
1.),(1.,0.7057524438612,1.),(1.,0.705792484282725,1.),(1.,0.705871570678672,
1.)))
REPRESENTATION_ITEM('')
SURFACE()
);
#1530=(
BOUNDED_SURFACE()
B_SPLINE_SURFACE(3,2,((#79683,#79684,#79685),(#79686,#79687,#79688),(#79689,
#79690,#79691),(#79692,#79693,#79694),(#79695,#79696,#79697),(#79698,#79699,
#79700),(#79701,#79702,#79703),(#79704,#79705,#79706)),.UNSPECIFIED.,.F.,
 .F.,.F.)
B_SPLINE_SURFACE_WITH_KNOTS((4,2,2,4),(3,3),(-1.36609473733174E-17,0.000314760444717569,
0.000629520889435153,0.00125904177887032),(0.,1.),.UNSPECIFIED.)
GEOMETRIC_REPRESENTATION_ITEM()
RATIONAL_B_SPLINE_SURFACE(((1.,0.705871570678672,1.),(1.,0.705832198773852,
1.),(1.,0.705802677875577,1.),(1.,0.705762810535121,1.),(1.,0.705752530546451,
1.),(1.,0.705752443861133,1.),(1.,0.705792484302369,1.),(1.,0.705871570678672,
1.)))
REPRESENTATION_ITEM('')
SURFACE()
);
#1531=(
BOUNDED_SURFACE()
B_SPLINE_SURFACE(3,2,((#79724,#79725,#79726),(#79727,#79728,#79729),(#79730,
#79731,#79732),(#79733,#79734,#79735),(#79736,#79737,#79738),(#79739,#79740,
#79741),(#79742,#79743,#79744),(#79745,#79746,#79747),(#79748,#79749,#79750),
(#79751,#79752,#79753),(#79754,#79755,#79756),(#79757,#79758,#79759),(#79760,
#79761,#79762),(#79763,#79764,#79765)),.UNSPECIFIED.,.F.,.F.,.F.)
B_SPLINE_SURFACE_WITH_KNOTS((4,2,2,2,2,2,4),(3,3),(0.0964178567359105,0.0969969483064025,
0.097141430047764,0.0974303935304871,0.0980083204959333,0.0991641744268257,
0.101910812839202),(-0.0156147939957968,0.908717315728862),
 .UNSPECIFIED.)
GEOMETRIC_REPRESENTATION_ITEM()
RATIONAL_B_SPLINE_SURFACE(((1.01039996590636,0.697849574056477,0.945601885810221),
(1.00920776855038,0.732486508654537,0.951837799321068),(1.00928443570073,
0.730259096339428,0.951436783737236),(1.00928198827333,0.730330201498752,
0.951449585263377),(1.00928121023475,0.730352805869793,0.9514536548759),
(1.00927803608829,0.730445024412888,0.951470257582389),(1.00927479988541,
0.730539045882487,0.951487184881511),(1.00926195866405,0.73091212215395,
0.951554352238807),(1.00924922181827,0.731282165999437,0.951620973648653),
(1.00920031293424,0.73270311682538,0.951876796704491),(1.00915348816192,
0.734063517910211,0.952121718595055),(1.00896275601819,0.739604862851685,
0.953119363109207),(1.00877459790181,0.745071424523457,0.954103543902988),
(1.00857970487406,0.750733655715106,0.955122952358132)))
REPRESENTATION_ITEM('')
SURFACE()
);
#1532=(
BOUNDED_SURFACE()
B_SPLINE_SURFACE(3,2,((#79838,#79839,#79840),(#79841,#79842,#79843),(#79844,
#79845,#79846),(#79847,#79848,#79849),(#79850,#79851,#79852),(#79853,#79854,
#79855),(#79856,#79857,#79858),(#79859,#79860,#79861),(#79862,#79863,#79864),
(#79865,#79866,#79867),(#79868,#79869,#79870),(#79871,#79872,#79873),(#79874,
#79875,#79876),(#79877,#79878,#79879)),.UNSPECIFIED.,.F.,.F.,.F.)
B_SPLINE_SURFACE_WITH_KNOTS((4,2,2,2,2,2,4),(3,3),(0.0924478328249838,0.0927448966007841,
0.0928885691804298,0.0931759143397212,0.0937506046583039,0.0948999852954695,
0.0973806489601807),(0.0912830955164557,1.),.UNSPECIFIED.)
GEOMETRIC_REPRESENTATION_ITEM()
RATIONAL_B_SPLINE_SURFACE(((0.950792246120108,0.730466229253696,1.),(0.951545496940602,
0.734592134582775,1.),(0.951441568640601,0.734022870912366,1.),(0.951449313493617,
0.734065293077013,1.),(0.951453334853521,0.734087319936867,1.),(0.951469744567059,
0.734177203575482,1.),(0.951486478882703,0.734268865210911,1.),(0.951552891707438,
0.734632639162483,1.),(0.951618775955208,0.734993517851996,1.),(0.951871831973123,
0.736379623441885,1.),(0.9521141728944,0.737707037460359,1.),(0.95303809490497,
0.742767788332922,1.),(0.953900490476868,0.747491530264648,1.),(0.954811659448391,
0.752482426806707,1.)))
REPRESENTATION_ITEM('')
SURFACE()
);
#1533=(
BOUNDED_SURFACE()
B_SPLINE_SURFACE(3,2,((#79936,#79937,#79938),(#79939,#79940,#79941),(#79942,
#79943,#79944),(#79945,#79946,#79947),(#79948,#79949,#79950),(#79951,#79952,
#79953),(#79954,#79955,#79956),(#79957,#79958,#79959),(#79960,#79961,#79962),
(#79963,#79964,#79965),(#79966,#79967,#79968),(#79969,#79970,#79971),(#79972,
#79973,#79974),(#79975,#79976,#79977),(#79978,#79979,#79980),(#79981,#79982,
#79983),(#79984,#79985,#79986),(#79987,#79988,#79989),(#79990,#79991,#79992),
(#79993,#79994,#79995),(#79996,#79997,#79998),(#79999,#80000,#80001),(#80002,
#80003,#80004),(#80005,#80006,#80007),(#80008,#80009,#80010),(#80011,#80012,
#80013)),.UNSPECIFIED.,.F.,.F.,.F.)
B_SPLINE_SURFACE_WITH_KNOTS((4,2,2,2,2,2,2,2,2,2,2,2,4),(3,3),(0.0594208250393089,
0.0624427293703808,0.0654646337014528,0.0684865380325247,0.0715084423635966,
0.0745303466946686,0.0775522510257405,0.0835960596878844,0.0896398683500283,
0.0956836770121721,0.101727485674316,0.104749390005388,0.10777129433646),
(0.,1.),.UNSPECIFIED.)
GEOMETRIC_REPRESENTATION_ITEM()
RATIONAL_B_SPLINE_SURFACE(((1.,0.910520832001509,1.),(1.,0.9105597736334,
1.),(1.,0.910319336406336,1.),(1.,0.908142721689739,1.),(1.,0.906245529262798,
1.),(1.,0.901234434942702,1.),(1.,0.898144388409968,1.),(1.,0.891406127314929,
1.),(1.,0.887761424599258,1.),(1.,0.880392731230951,1.),(1.,0.876718575830069,
1.),(1.,0.869691185417515,1.),(1.,0.866327693994065,1.),(1.,0.856764909704854,
1.),(1.,0.851141864877978,1.),(1.,0.840201694261591,1.),(1.,0.834927827340277,
1.),(1.,0.822462805562699,1.),(1.,0.815237195282872,1.),(1.,0.796337704941202,
1.),(1.,0.784465640270227,1.),(1.,0.763309807388115,1.),(1.,0.755741399790356,
1.),(1.,0.740595302762885,1.),(1.,0.733036463112068,1.),(1.,0.726414797481264,
1.)))
REPRESENTATION_ITEM('')
SURFACE()
);
#1534=(
BOUNDED_SURFACE()
B_SPLINE_SURFACE(3,2,((#80259,#80260,#80261),(#80262,#80263,#80264),(#80265,
#80266,#80267),(#80268,#80269,#80270),(#80271,#80272,#80273),(#80274,#80275,
#80276),(#80277,#80278,#80279),(#80280,#80281,#80282),(#80283,#80284,#80285),
(#80286,#80287,#80288),(#80289,#80290,#80291),(#80292,#80293,#80294),(#80295,
#80296,#80297),(#80298,#80299,#80300),(#80301,#80302,#80303),(#80304,#80305,
#80306),(#80307,#80308,#80309),(#80310,#80311,#80312),(#80313,#80314,#80315),
(#80316,#80317,#80318),(#80319,#80320,#80321),(#80322,#80323,#80324),(#80325,
#80326,#80327),(#80328,#80329,#80330)),.UNSPECIFIED.,.F.,.F.,.F.)
B_SPLINE_SURFACE_WITH_KNOTS((4,2,2,2,2,2,2,2,2,2,2,4),(3,3),(0.0606605585620472,
0.0636555247412189,0.0666504909203906,0.0696454570995622,0.0726404232787339,
0.0786303556370772,0.0846202879954206,0.0906102203537639,0.0966001527121072,
0.102590085070451,0.105585051249622,0.108580017428794),(0.,1.),
 .UNSPECIFIED.)
GEOMETRIC_REPRESENTATION_ITEM()
RATIONAL_B_SPLINE_SURFACE(((1.,0.910520832008251,1.),(1.,0.910557149201625,
1.),(1.,0.910326426062521,1.),(1.,0.908197427220197,1.),(1.,0.906334049728144,
1.),(1.,0.901360304418425,1.),(1.,0.898273108952946,1.),(1.,0.891491725305196,
1.),(1.,0.887782421911941,1.),(1.,0.876777623836887,1.),(1.,0.869626693180036,
1.),(1.,0.856891658692805,1.),(1.,0.851262654293129,1.),(1.,0.8403112833867,
1.),(1.,0.835034820594825,1.),(1.,0.822574702116822,1.),(1.,0.815355066496494,
1.),(1.,0.796454715054513,1.),(1.,0.784574360623197,1.),(1.,0.763378174579001,
1.),(1.,0.755789676929053,1.),(1.,0.740619606484873,1.),(1.,0.733047686471531,
1.),(1.,0.726415577619866,1.)))
REPRESENTATION_ITEM('')
SURFACE()
);
#1535=(
BOUNDED_SURFACE()
B_SPLINE_SURFACE(3,2,((#82000,#82001,#82002),(#82003,#82004,#82005),(#82006,
#82007,#82008),(#82009,#82010,#82011)),.UNSPECIFIED.,.F.,.F.,.F.)
B_SPLINE_SURFACE_WITH_KNOTS((4,4),(3,3),(0.216396890133946,0.218669589029756),
(-1.61816610990125E-8,1.00000001618164),.UNSPECIFIED.)
GEOMETRIC_REPRESENTATION_ITEM()
RATIONAL_B_SPLINE_SURFACE(((1.00000000633075,0.804385064253204,1.00000000633074),
(1.0000000063304,0.804395878645463,1.00000000633039),(1.00000000633075,
0.804385034103866,1.00000000633074),(1.00000000632997,0.804409130794161,
1.00000000632996)))
REPRESENTATION_ITEM('')
SURFACE()
);
#1536=(
BOUNDED_SURFACE()
B_SPLINE_SURFACE(3,2,((#82049,#82050,#82051),(#82052,#82053,#82054),(#82055,
#82056,#82057),(#82058,#82059,#82060),(#82061,#82062,#82063),(#82064,#82065,
#82066),(#82067,#82068,#82069),(#82070,#82071,#82072),(#82073,#82074,#82075),
(#82076,#82077,#82078),(#82079,#82080,#82081),(#82082,#82083,#82084),(#82085,
#82086,#82087),(#82088,#82089,#82090),(#82091,#82092,#82093),(#82094,#82095,
#82096),(#82097,#82098,#82099),(#82100,#82101,#82102),(#82103,#82104,#82105),
(#82106,#82107,#82108),(#82109,#82110,#82111),(#82112,#82113,#82114),(#82115,
#82116,#82117),(#82118,#82119,#82120),(#82121,#82122,#82123),(#82124,#82125,
#82126),(#82127,#82128,#82129),(#82130,#82131,#82132),(#82133,#82134,#82135),
(#82136,#82137,#82138),(#82139,#82140,#82141),(#82142,#82143,#82144)),
 .UNSPECIFIED.,.F.,.F.,.F.)
B_SPLINE_SURFACE_WITH_KNOTS((4,2,2,2,2,2,2,2,2,2,2,2,2,2,2,4),(3,3),(0.0174491083826989,
0.0224393045100345,0.0274148701487939,0.0373660014263126,0.0473171327038314,
0.0572682639813502,0.0622438296201096,0.067219395258869,0.0721949608976284,
0.0771705265363878,0.0796583093557675,0.0821460921751472,0.0871216578139065,
0.0896094406332862,0.0920972234526659,0.0970881741758769),(-1.53850844515961E-5,
1.),.UNSPECIFIED.)
GEOMETRIC_REPRESENTATION_ITEM()
RATIONAL_B_SPLINE_SURFACE(((1.00000601573862,0.804494455691282,1.),(1.00000601347822,
0.804567916370663,1.),(1.00000598439474,0.80551310069534,1.),(1.00000592861333,
0.807325941125275,1.),(1.00000590213421,0.808186486425802,1.),(1.00000584309961,
0.8101050523979,1.),(1.00000582785138,0.810600604914554,1.),(1.00000576773212,
0.812554421336114,1.),(1.00000572109564,0.814070060616225,1.),(1.00000555112649,
0.819593889563631,1.),(1.00000542866216,0.823573859054488,1.),(1.00000517883153,
0.831693106854347,1.),(1.00000508467203,0.834753197277551,1.),(1.00000487522662,
0.841559965551597,1.),(1.00000475986163,0.845309213420213,1.),(1.00000450905516,
0.853460175211236,1.),(1.00000437351983,0.857864939115207,1.),(1.00000408592671,
0.867211430603691,1.),(1.00000393358681,0.872162326389599,1.),(1.00000370102243,
0.879720438187042,1.),(1.00000362262617,0.882268239125395,1.),(1.00000347023075,
0.887220939280501,1.),(1.00000339603593,0.889632197256966,1.),(1.00000318536523,
0.896478786368241,1.),(1.00000306133323,0.900509703409517,1.),(1.00000292228749,
0.90502855208934,1.),(1.00000288369192,0.906282870115633,1.),(1.00000282289798,
0.908258612681891,1.),(1.00000280075343,0.908978288843577,1.),(1.00000275537084,
0.910453178046207,1.),(1.00000275328214,0.910521058617971,1.),(1.000002752855,
0.910534940276836,0.999999999999999)))
REPRESENTATION_ITEM('')
SURFACE()
);
#1537=(
BOUNDED_SURFACE()
B_SPLINE_SURFACE(3,2,((#82158,#82159,#82160),(#82161,#82162,#82163),(#82164,
#82165,#82166),(#82167,#82168,#82169),(#82170,#82171,#82172),(#82173,#82174,
#82175),(#82176,#82177,#82178),(#82179,#82180,#82181),(#82182,#82183,#82184),
(#82185,#82186,#82187),(#82188,#82189,#82190),(#82191,#82192,#82193),(#82194,
#82195,#82196),(#82197,#82198,#82199),(#82200,#82201,#82202),(#82203,#82204,
#82205),(#82206,#82207,#82208),(#82209,#82210,#82211),(#82212,#82213,#82214),
(#82215,#82216,#82217),(#82218,#82219,#82220),(#82221,#82222,#82223),(#82224,
#82225,#82226),(#82227,#82228,#82229),(#82230,#82231,#82232),(#82233,#82234,
#82235),(#82236,#82237,#82238),(#82239,#82240,#82241),(#82242,#82243,#82244),
(#82245,#82246,#82247),(#82248,#82249,#82250),(#82251,#82252,#82253),(#82254,
#82255,#82256),(#82257,#82258,#82259),(#82260,#82261,#82262),(#82263,#82264,
#82265),(#82266,#82267,#82268),(#82269,#82270,#82271),(#82272,#82273,#82274),
(#82275,#82276,#82277),(#82278,#82279,#82280),(#82281,#82282,#82283)),
 .UNSPECIFIED.,.F.,.F.,.F.)
B_SPLINE_SURFACE_WITH_KNOTS((4,2,2,2,2,2,2,2,2,2,2,2,2,2,2,2,2,2,2,2,4),
(3,3),(0.0202219973471745,0.0205361900892103,0.0206932864602282,0.0208503828312461,
0.0214787683153177,0.0227355392834609,0.0252490812197474,0.0302761650923202,
0.0403303328374658,0.0503845005826114,0.060438668327757,0.0654657522003299,
0.0704928360729027,0.0755199199454755,0.0805470038180483,0.0830605457543347,
0.0855740876906211,0.0906011715631939,0.0956282554357667,0.0981417973720531,
0.10065533930834),(0.,1.),.UNSPECIFIED.)
GEOMETRIC_REPRESENTATION_ITEM()
RATIONAL_B_SPLINE_SURFACE(((1.,0.807165688592199,1.),(1.,0.806582212610433,
1.),(1.,0.805998311839245,1.),(1.,0.805121971305601,1.),(1.,0.804829775055439,
1.),(1.,0.804245234526162,1.),(1.,0.804494537678017,1.),(1.,0.804512504992895,
1.),(1.,0.804541617021244,1.),(1.,0.804665694249588,1.),(1.,0.804797226303217,
1.),(1.,0.805283123878148,1.),(1.,0.805724879158345,1.),(1.,0.807081366668598,
1.),(1.,0.807987348168922,1.),(1.,0.810007014899584,1.),(1.,0.810518600716015,
1.),(1.,0.812400911040395,1.),(1.,0.813844794272986,1.),(1.,0.819230623807962,
1.),(1.,0.823143123389045,1.),(1.,0.831181433207098,1.),(1.,0.834218469870357,
1.),(1.,0.840986673920921,1.),(1.,0.844720392224904,1.),(1.,0.852849711004914,
1.),(1.,0.85724827861479,1.),(1.,0.866596658340533,1.),(1.,0.871555644103613,
1.),(1.,0.879143902650669,1.),(1.,0.881695428003563,1.),(1.,0.886744320440305,
1.),(1.,0.88920804734286,1.),(1.,0.896192729532698,1.),(1.,0.900300234614913,
1.),(1.,0.906436112516518,1.),(1.,0.908421979022621,1.),(1.,0.909940953080824,
1.),(1.,0.910217476180097,1.),(1.,0.910507345346127,1.),(1.,0.910523722940057,
1.),(1.,0.910536186741694,1.)))
REPRESENTATION_ITEM('')
SURFACE()
);
#1538=(
BOUNDED_SURFACE()
B_SPLINE_SURFACE(3,2,((#82322,#82323,#82324),(#82325,#82326,#82327),(#82328,
#82329,#82330),(#82331,#82332,#82333)),.UNSPECIFIED.,.F.,.F.,.F.)
B_SPLINE_SURFACE_WITH_KNOTS((4,4),(3,3),(0.216508113827287,0.218767312738254),
(0.,1.),.UNSPECIFIED.)
GEOMETRIC_REPRESENTATION_ITEM()
RATIONAL_B_SPLINE_SURFACE(((1.,0.804378955100775,1.),(1.,0.804378707109012,
1.),(1.,0.804379610342439,1.),(1.,0.804401469359353,1.)))
REPRESENTATION_ITEM('')
SURFACE()
);
#1539=(
BOUNDED_SURFACE()
B_SPLINE_SURFACE(3,2,((#82334,#82335,#82336),(#82337,#82338,#82339),(#82340,
#82341,#82342),(#82343,#82344,#82345)),.UNSPECIFIED.,.F.,.F.,.F.)
B_SPLINE_SURFACE_WITH_KNOTS((4,4),(3,3),(0.10574004256303,0.205836563902916),
(-5.04238789072631E-7,1.00000050424698),.UNSPECIFIED.)
GEOMETRIC_REPRESENTATION_ITEM()
RATIONAL_B_SPLINE_SURFACE(((1.00000008857927,0.912165313998971,1.00000008858071),
(1.00000008909479,0.91165412809819,1.00000008909623),(1.00000008961932,
0.911134000853112,1.00000008962078),(1.00000009015337,0.910604444656701,
1.00000009015483)))
REPRESENTATION_ITEM('')
SURFACE()
);
#1540=(
BOUNDED_SURFACE()
B_SPLINE_SURFACE(3,2,((#82358,#82359,#82360),(#82361,#82362,#82363),(#82364,
#82365,#82366),(#82367,#82368,#82369)),.UNSPECIFIED.,.F.,.F.,.F.)
B_SPLINE_SURFACE_WITH_KNOTS((4,4),(3,3),(0.115644169265868,0.215740688922389),
(-5.04243592763465E-7,1.00000050424162),.UNSPECIFIED.)
GEOMETRIC_REPRESENTATION_ITEM()
RATIONAL_B_SPLINE_SURFACE(((1.00000009015423,0.910604444683308,1.00000009015387),
(1.00000008962018,0.911134000870471,1.00000008961982),(1.00000008909563,
0.911654128106663,1.00000008909529),(1.00000008858011,0.912165313998868,
1.00000008857976)))
REPRESENTATION_ITEM('')
SURFACE()
);
#1541=(
BOUNDED_SURFACE()
B_SPLINE_SURFACE(3,2,((#82378,#82379,#82380),(#82381,#82382,#82383),(#82384,
#82385,#82386),(#82387,#82388,#82389)),.UNSPECIFIED.,.F.,.F.,.F.)
B_SPLINE_SURFACE_WITH_KNOTS((4,4),(3,3),(0.10574004257307,0.205836562229605),
(-5.04246958612367E-7,1.00000050424698),.UNSPECIFIED.)
GEOMETRIC_REPRESENTATION_ITEM()
RATIONAL_B_SPLINE_SURFACE(((1.0000000885807,0.9121653139981,1.00000008858071),
(1.00000008909623,0.911654128105911,1.00000008909623),(1.00000008962077,
0.911134000869722,1.00000008962078),(1.00000009015483,0.910604444682528,
1.00000009015483)))
REPRESENTATION_ITEM('')
SURFACE()
);
#1542=(
BOUNDED_SURFACE()
B_SPLINE_SURFACE(3,2,((#82394,#82395,#82396),(#82397,#82398,#82399),(#82400,
#82401,#82402),(#82403,#82404,#82405)),.UNSPECIFIED.,.F.,.F.,.F.)
B_SPLINE_SURFACE_WITH_KNOTS((4,4),(3,3),(0.11564416787367,0.21574068893074),
(-5.04246457809262E-7,1.00000050424698),.UNSPECIFIED.)
GEOMETRIC_REPRESENTATION_ITEM()
RATIONAL_B_SPLINE_SURFACE(((1.00000009015474,0.910604444660476,1.00000009015483),
(1.00000008962069,0.911134000855317,1.00000008962078),(1.00000008909614,
0.911654128098913,1.00000008909623),(1.00000008858061,0.912165313998272,
1.00000008858071)))
REPRESENTATION_ITEM('')
SURFACE()
);
#1543=(
BOUNDED_SURFACE()
B_SPLINE_SURFACE(3,2,((#82662,#82663,#82664),(#82665,#82666,#82667),(#82668,
#82669,#82670),(#82671,#82672,#82673),(#82674,#82675,#82676),(#82677,#82678,
#82679),(#82680,#82681,#82682),(#82683,#82684,#82685),(#82686,#82687,#82688),
(#82689,#82690,#82691),(#82692,#82693,#82694),(#82695,#82696,#82697),(#82698,
#82699,#82700),(#82701,#82702,#82703),(#82704,#82705,#82706),(#82707,#82708,
#82709),(#82710,#82711,#82712),(#82713,#82714,#82715),(#82716,#82717,#82718),
(#82719,#82720,#82721),(#82722,#82723,#82724),(#82725,#82726,#82727),(#82728,
#82729,#82730),(#82731,#82732,#82733),(#82734,#82735,#82736),(#82737,#82738,
#82739),(#82740,#82741,#82742),(#82743,#82744,#82745),(#82746,#82747,#82748),
(#82749,#82750,#82751),(#82752,#82753,#82754),(#82755,#82756,#82757),(#82758,
#82759,#82760),(#82761,#82762,#82763),(#82764,#82765,#82766),(#82767,#82768,
#82769),(#82770,#82771,#82772),(#82773,#82774,#82775)),.UNSPECIFIED.,.F.,
 .F.,.F.)
B_SPLINE_SURFACE_WITH_KNOTS((4,2,2,2,2,2,2,2,2,2,2,2,2,2,2,2,2,2,4),(3,
3),(-0.000153005044684754,0.00487935154325309,0.00975870308650617,0.0146380546297593,
0.0195174061730123,0.0219570819446389,0.0243967577162654,0.0292761092595185,
0.0341554608027716,0.0390348123460247,0.0414744881176512,0.0439141638892778,
0.0487935154325309,0.0536728669757839,0.058552218519037,0.0634315700622901,
0.0683109216055432,0.0731902731487963,0.0782226297367341),(-0.0169255195142288,
1.00015300504468),.UNSPECIFIED.)
GEOMETRIC_REPRESENTATION_ITEM()
RATIONAL_B_SPLINE_SURFACE(((1.0100822613812,0.702111663841635,1.00008963941067),
(1.0100867902307,0.701977855424187,1.00008967967579),(1.01004679985172,
0.703159402599464,1.00008932412916),(1.00994454152905,0.706180705107466,
1.00008841497045),(1.00988572291064,0.707918547414101,1.00008789202564),
(1.00982367182762,0.709751895427783,1.00008734034161),(1.00982036137587,
0.70984970532654,1.00008731090904),(1.00991672914796,0.707002443764782,
1.00008816769602),(1.01001697409506,0.704040628020217,1.0000890589542),
(1.01025875007564,0.696897166662037,1.00009120853708),(1.0103545597349,
0.694066394982443,1.00009206036199),(1.01057160703966,0.68765356178565,
1.00009399008705),(1.01069283755543,0.684071710922103,1.00009506792382),
(1.01108293972011,0.672545835885354,1.00009853624574),(1.01137949432823,
0.663783896926268,1.00010117285466),(1.01194225591252,0.647156663644023,
1.00010617625765),(1.01220631384047,0.639354864639494,1.00010852394495),
(1.01258477234773,0.628173010611811,1.0001118887454),(1.01269712171499,
0.624853560260868,1.00011288762161),(1.01270485754633,0.624624999044277,
1.00011295639937),(1.0126812274977,0.625323167401867,1.00011274630924),
(1.01258396260394,0.628196935128459,1.00011188154612),(1.01251079042069,
0.630358864788737,1.00011123098658),(1.01223331549631,0.638557079497002,
1.00010876401139),(1.01197060246929,0.646319142346594,1.00010642828133),
(1.01140779312517,0.662947786730735,1.00010142445372),(1.01110987446146,
0.671750027784363,1.00009877571724),(1.01058580635657,0.687234031808314,
1.0000941163304),(1.01036033377541,0.693895796417769,1.00009211169785),
(1.0100292848136,0.703676898165709,1.00008916840639),(1.00992329109318,
0.706808565936043,1.00008822603699),(1.0098208881916,0.709834140141601,
1.00008731559285),(1.00982288319264,0.709775196268177,1.00008733333001),
(1.00988403419022,0.707968441985946,1.00008787701155),(1.00994325766289,
0.706218637942392,1.00008840355585),(1.01004641341464,0.703170820186587,
1.00008932069343),(1.010086856497,0.701975897534046,1.00008968026495),(1.01008225630153,
0.7021118139247,1.00008963936551)))
REPRESENTATION_ITEM('')
SURFACE()
);
#1544=(
BOUNDED_SURFACE()
B_SPLINE_SURFACE(3,2,((#82814,#82815,#82816),(#82817,#82818,#82819),(#82820,
#82821,#82822),(#82823,#82824,#82825),(#82826,#82827,#82828),(#82829,#82830,
#82831),(#82832,#82833,#82834),(#82835,#82836,#82837),(#82838,#82839,#82840),
(#82841,#82842,#82843),(#82844,#82845,#82846),(#82847,#82848,#82849),(#82850,
#82851,#82852),(#82853,#82854,#82855),(#82856,#82857,#82858),(#82859,#82860,
#82861),(#82862,#82863,#82864),(#82865,#82866,#82867),(#82868,#82869,#82870),
(#82871,#82872,#82873),(#82874,#82875,#82876),(#82877,#82878,#82879),(#82880,
#82881,#82882),(#82883,#82884,#82885),(#82886,#82887,#82888),(#82889,#82890,
#82891),(#82892,#82893,#82894),(#82895,#82896,#82897),(#82898,#82899,#82900),
(#82901,#82902,#82903),(#82904,#82905,#82906),(#82907,#82908,#82909),(#82910,
#82911,#82912),(#82913,#82914,#82915),(#82916,#82917,#82918),(#82919,#82920,
#82921),(#82922,#82923,#82924),(#82925,#82926,#82927),(#82928,#82929,#82930),
(#82931,#82932,#82933),(#82934,#82935,#82936),(#82937,#82938,#82939),(#82940,
#82941,#82942),(#82943,#82944,#82945),(#82946,#82947,#82948),(#82949,#82950,
#82951),(#82952,#82953,#82954),(#82955,#82956,#82957),(#82958,#82959,#82960),
(#82961,#82962,#82963),(#82964,#82965,#82966),(#82967,#82968,#82969),(#82970,
#82971,#82972),(#82973,#82974,#82975),(#82976,#82977,#82978),(#82979,#82980,
#82981),(#82982,#82983,#82984),(#82985,#82986,#82987),(#82988,#82989,#82990),
(#82991,#82992,#82993),(#82994,#82995,#82996),(#82997,#82998,#82999),(#83000,
#83001,#83002),(#83003,#83004,#83005),(#83006,#83007,#83008),(#83009,#83010,
#83011),(#83012,#83013,#83014),(#83015,#83016,#83017),(#83018,#83019,#83020),
(#83021,#83022,#83023),(#83024,#83025,#83026),(#83027,#83028,#83029),(#83030,
#83031,#83032),(#83033,#83034,#83035),(#83036,#83037,#83038),(#83039,#83040,
#83041),(#83042,#83043,#83044),(#83045,#83046,#83047),(#83048,#83049,#83050),
(#83051,#83052,#83053),(#83054,#83055,#83056),(#83057,#83058,#83059),(#83060,
#83061,#83062),(#83063,#83064,#83065)),.UNSPECIFIED.,.F.,.F.,.F.)
B_SPLINE_SURFACE_WITH_KNOTS((4,2,2,2,2,2,2,2,2,2,2,2,2,2,2,2,2,2,2,2,2,
2,2,2,2,2,2,2,2,2,2,2,2,2,2,2,2,2,2,2,2,4),(3,3),(0.143336734946112,0.145077233025809,
0.14676220431832,0.14844717561083,0.149289661257085,0.150132146903341,0.150974632549596,
0.151395875372724,0.151817118195851,0.152238361018979,0.152659603842107,
0.153080846665234,0.153502089488362,0.154344575134617,0.155187060780872,
0.156029546427128,0.156872032073383,0.158557003365894,0.160241974658404,
0.163611917243425,0.166981859828446,0.170351802413467,0.173721744998489,
0.17709168758351,0.180461630168531,0.182146601461041,0.183831572753552,
0.184674058399807,0.185516544046062,0.186359029692318,0.187201515338573,
0.187622758161701,0.188044000984828,0.188465243807956,0.188886486631084,
0.189728972277339,0.190571457923594,0.191413943569849,0.192256429216105,
0.193941400508615,0.195626371801126,0.197366417069027),(-5.55267871867606E-5,
1.),.UNSPECIFIED.)
GEOMETRIC_REPRESENTATION_ITEM()
RATIONAL_B_SPLINE_SURFACE(((1.0000007961373,0.992831051955489,1.),(1.00000079614004,
0.99283102735741,1.),(1.00000079610334,0.992831357779363,1.),(1.00000079553568,
0.992836469390048,1.),(1.00000079502573,0.992841061353999,1.),(1.00000079388901,
0.992851297090919,1.),(1.00000079321307,0.992857383722212,1.),(1.00000079328263,
0.992856757367858,1.),(1.00000079349646,0.992854831864327,1.),(1.00000079489792,
0.99284221223048,1.),(1.0000007960679,0.992831676885065,1.),(1.00000080065879,
0.992790337525115,1.),(1.00000080402759,0.99276000259259,1.),(1.00000081291108,
0.99268000979147,1.),(1.0000008165308,0.992647415417328,1.),(1.00000082570108,
0.992564840127059,1.),(1.00000083126436,0.992514744632364,1.),(1.00000084494363,
0.992391567460146,1.),(1.00000085308652,0.992318243506232,1.),(1.00000087193122,
0.992148553332822,1.),(1.00000088262546,0.992052255238254,1.),(1.00000090544812,
0.99184674487725,1.),(1.00000091755832,0.99173769661988,1.),(1.00000094174194,
0.9915199312853,1.),(1.00000095374568,0.991411841667855,1.),(1.0000009885794,
0.991098175741489,1.),(1.00000101018179,0.990903653484852,1.),(1.0000010498042,
0.990546867101254,1.),(1.00000106791611,0.990383775459736,1.),(1.00000110147245,
0.990081611875504,1.),(1.000001116925,0.989942466912265,1.),(1.00000114577958,
0.989682641089782,1.),(1.00000115917998,0.989561975013968,1.),(1.00000119692308,
0.989222111151196,1.),(1.00000121884368,0.98902472358164,1.),(1.0000012581359,
0.988670910349041,1.),(1.00000127548289,0.988514706508194,1.),(1.00000132214589,
0.98809452195995,1.),(1.00000134616352,0.987878251318118,1.),(1.0000013836916,
0.987540323616174,1.),(1.00000139708822,0.987419691529657,1.),(1.00000141461613,
0.987261858649905,1.),(1.00000141873575,0.987224762828979,1.),(1.00000141813951,
0.987230131741563,1.),(1.00000141342297,0.987272602591746,1.),(1.00000139474718,
0.987440771836899,1.),(1.00000138080777,0.987566291546218,1.),(1.00000134224022,
0.987913579257289,1.),(1.00000131768873,0.988134657203702,1.),(1.00000127005862,
0.98856355026087,1.),(1.00000125236095,0.988722911871249,1.),(1.00000121226484,
0.98908396376986,1.),(1.0000011898936,0.989285409256699,1.),(1.00000115132915,
0.989632669120568,1.),(1.00000113763001,0.989756025257267,1.),(1.00000110810876,
0.990021854183857,1.),(1.00000109228755,0.990164318811314,1.),(1.00000105790784,
0.990473896506666,1.),(1.00000103933542,0.990641134935092,1.),(1.00000099876335,
0.991006472756129,1.),(1.00000097663901,0.991205694949805,1.),(1.00000094145119,
0.991522549380576,1.),(1.00000092941198,0.991630958408669,1.),(1.00000090553833,
0.991845932574461,1.),(1.00000089369581,0.991952570533307,1.),(1.00000087196574,
0.992148242439595,1.),(1.00000086207814,0.992237276976211,1.),(1.00000084501282,
0.992390944434512,1.),(1.0000008378228,0.992455688157901,1.),(1.00000081985816,
0.992617453680996,1.),(1.00000081255367,0.992683228105805,1.),(1.0000008023705,
0.992774924164358,1.),(1.00000079947944,0.992800957134375,1.),(1.00000079555182,
0.992836324009601,1.),(1.00000079455633,0.992845288063244,1.),(1.00000079339196,
0.992855772879035,1.),(1.00000079324102,0.992857132057369,1.),(1.00000079329672,
0.992856630423569,1.),(1.00000079396815,0.992850584467251,1.),(1.00000079508137,
0.992840560290287,1.),(1.00000079556752,0.992836182715642,1.),(1.00000079610664,
0.99283132804581,1.),(1.00000079613978,0.992831029688952,1.),(1.00000079613732,
0.992831051827691,1.)))
REPRESENTATION_ITEM('')
SURFACE()
);
#1545=(
BOUNDED_SURFACE()
B_SPLINE_SURFACE(3,2,((#83553,#83554,#83555),(#83556,#83557,#83558),(#83559,
#83560,#83561),(#83562,#83563,#83564),(#83565,#83566,#83567),(#83568,#83569,
#83570),(#83571,#83572,#83573),(#83574,#83575,#83576),(#83577,#83578,#83579),
(#83580,#83581,#83582),(#83583,#83584,#83585),(#83586,#83587,#83588),(#83589,
#83590,#83591),(#83592,#83593,#83594),(#83595,#83596,#83597),(#83598,#83599,
#83600),(#83601,#83602,#83603),(#83604,#83605,#83606),(#83607,#83608,#83609),
(#83610,#83611,#83612),(#83613,#83614,#83615),(#83616,#83617,#83618),(#83619,
#83620,#83621),(#83622,#83623,#83624),(#83625,#83626,#83627),(#83628,#83629,
#83630),(#83631,#83632,#83633),(#83634,#83635,#83636),(#83637,#83638,#83639),
(#83640,#83641,#83642),(#83643,#83644,#83645),(#83646,#83647,#83648),(#83649,
#83650,#83651),(#83652,#83653,#83654),(#83655,#83656,#83657),(#83658,#83659,
#83660),(#83661,#83662,#83663),(#83664,#83665,#83666),(#83667,#83668,#83669),
(#83670,#83671,#83672),(#83673,#83674,#83675),(#83676,#83677,#83678),(#83679,
#83680,#83681),(#83682,#83683,#83684),(#83685,#83686,#83687),(#83688,#83689,
#83690)),.UNSPECIFIED.,.F.,.F.,.F.)
B_SPLINE_SURFACE_WITH_KNOTS((4,2,2,2,2,2,2,2,2,2,2,2,2,2,2,2,2,2,2,2,2,
2,4),(3,3),(0.,0.00173795884810334,0.00260693827215501,0.00347591769620668,
0.00521387654431002,0.00608285596836169,0.00695183539241337,0.00868979424051671,
0.01042775308862,0.0112967325126717,0.0121657119367234,0.0139036707848267,
0.0147726502088784,0.0156416296329301,0.0173795884810334,0.0191175473291368,
0.0199865267531884,0.0208555061772401,0.0225934650253434,0.0234624444493951,
0.0243314238734468,0.0260693827215501,0.0278073415696535),(0.,1.),
 .UNSPECIFIED.)
GEOMETRIC_REPRESENTATION_ITEM()
RATIONAL_B_SPLINE_SURFACE(((1.,0.548774182857018,1.),(1.,0.548893499031212,
1.),(1.,0.551454790284224,1.),(1.,0.558414139525284,1.),(1.,0.561252468336352,
1.),(1.,0.567859325258193,1.),(1.,0.571621573059519,1.),(1.,0.583808409735634,
1.),(1.,0.593194455071645,1.),(1.,0.608188368401722,1.),(1.,0.613360873897966,
1.),(1.,0.62366572039419,1.),(1.,0.628817963503084,1.),(1.,0.644073171070199,
1.),(1.,0.654001656968634,1.),(1.,0.67225025019413,1.),(1.,0.68032620635555,
1.),(1.,0.690419184626026,1.),(1.,0.693446892845268,1.),(1.,0.698746884637556,
1.),(1.,0.7010212029547,1.),(1.,0.70645959379097,1.),(1.,0.708316472383437,
1.),(1.,0.70835119300799,1.),(1.,0.70789791374197,1.),(1.,0.706062313929642,
1.),(1.,0.70469165429023,1.),(1.,0.699305887702423,1.),(1.,0.69401802314486,
1.),(1.,0.680392676022202,1.),(1.,0.672280667494579,1.),(1.,0.658740368498969,
1.),(1.,0.653997319012882,1.),(1.,0.644149376735424,1.),(1.,0.639064976044898,
1.),(1.,0.623754379898659,1.),(1.,0.613373212611566,1.),(1.,0.598394950949806,
1.),(1.,0.593477175295379,1.),(1.,0.584180333306127,1.),(1.,0.579796878582778,
1.),(1.,0.567666674638681,1.),(1.,0.560935688280663,1.),(1.,0.551485305881092,
1.),(1.,0.548874864843112,1.),(1.,0.548774182857018,1.)))
REPRESENTATION_ITEM('')
SURFACE()
);
#1546=(
BOUNDED_SURFACE()
B_SPLINE_SURFACE(2,3,((#84213,#84214,#84215,#84216),(#84217,#84218,#84219,
#84220),(#84221,#84222,#84223,#84224)),.UNSPECIFIED.,.F.,.F.,.F.)
B_SPLINE_SURFACE_WITH_KNOTS((3,3),(4,4),(0.119519500000458,0.283084102927177),
(0.,1.),.UNSPECIFIED.)
GEOMETRIC_REPRESENTATION_ITEM()
RATIONAL_B_SPLINE_SURFACE(((1.,0.999857616157758,0.999857616157758,1.),
(1.,0.999857616157758,0.999857616157758,1.),(1.,0.999857616157758,0.999857616157758,
1.)))
REPRESENTATION_ITEM('')
SURFACE()
);
#1547=(
BOUNDED_SURFACE()
B_SPLINE_SURFACE(2,3,((#84226,#84227,#84228,#84229),(#84230,#84231,#84232,
#84233),(#84234,#84235,#84236,#84237)),.UNSPECIFIED.,.F.,.F.,.F.)
B_SPLINE_SURFACE_WITH_KNOTS((3,3),(4,4),(0.446518847929411,0.592183392830318),
(0.,1.),.UNSPECIFIED.)
GEOMETRIC_REPRESENTATION_ITEM()
RATIONAL_B_SPLINE_SURFACE(((1.,0.999895190835713,0.999895190835713,1.),
(1.,0.999895190835713,0.999895190835713,1.),(1.,0.999895190835713,0.999895190835713,
1.)))
REPRESENTATION_ITEM('')
SURFACE()
);
#1548=(
BOUNDED_SURFACE()
B_SPLINE_SURFACE(2,3,((#84239,#84240,#84241,#84242),(#84243,#84244,#84245,
#84246),(#84247,#84248,#84249,#84250)),.UNSPECIFIED.,.F.,.F.,.F.)
B_SPLINE_SURFACE_WITH_KNOTS((3,3),(4,4),(0.444107179195925,0.589622570294522),
(0.,1.),.UNSPECIFIED.)
GEOMETRIC_REPRESENTATION_ITEM()
RATIONAL_B_SPLINE_SURFACE(((1.,0.999894134350414,0.999894134350414,1.),
(1.,0.999894134350414,0.999894134350414,1.),(1.,0.999894134350414,0.999894134350414,
1.)))
REPRESENTATION_ITEM('')
SURFACE()
);
#1549=(
BOUNDED_SURFACE()
B_SPLINE_SURFACE(2,3,((#84252,#84253,#84254,#84255),(#84256,#84257,#84258,
#84259),(#84260,#84261,#84262,#84263)),.UNSPECIFIED.,.F.,.F.,.F.)
B_SPLINE_SURFACE_WITH_KNOTS((3,3),(4,4),(0.116491116663128,0.280009921526958),
(0.,1.),.UNSPECIFIED.)
GEOMETRIC_REPRESENTATION_ITEM()
RATIONAL_B_SPLINE_SURFACE(((1.,0.999856284631683,0.999856284631683,1.),
(1.,0.999856284631683,0.999856284631683,1.),(1.,0.999856284631683,0.999856284631683,
1.)))
REPRESENTATION_ITEM('')
SURFACE()
);
#1550=(
BOUNDED_SURFACE()
B_SPLINE_SURFACE(2,3,((#84265,#84266,#84267,#84268),(#84269,#84270,#84271,
#84272),(#84273,#84274,#84275,#84276)),.UNSPECIFIED.,.F.,.F.,.F.)
B_SPLINE_SURFACE_WITH_KNOTS((3,3),(4,4),(0.4413524597824,0.586836701733118),
(0.,1.),.UNSPECIFIED.)
GEOMETRIC_REPRESENTATION_ITEM()
RATIONAL_B_SPLINE_SURFACE(((1.,0.99989457919486,0.99989457919486,1.),(1.,
0.99989457919486,0.99989457919486,1.),(1.,0.99989457919486,0.99989457919486,
1.)))
REPRESENTATION_ITEM('')
SURFACE()
);
#1551=(
BOUNDED_SURFACE()
B_SPLINE_SURFACE(2,3,((#84278,#84279,#84280,#84281),(#84282,#84283,#84284,
#84285),(#84286,#84287,#84288,#84289)),.UNSPECIFIED.,.F.,.F.,.F.)
B_SPLINE_SURFACE_WITH_KNOTS((3,3),(4,4),(0.11378820966997,0.27774209483516),
(0.,1.),.UNSPECIFIED.)
GEOMETRIC_REPRESENTATION_ITEM()
RATIONAL_B_SPLINE_SURFACE(((1.,0.99985641298154,0.99985641298154,1.),(1.,
0.99985641298154,0.99985641298154,1.),(1.,0.99985641298154,0.99985641298154,
1.)))
REPRESENTATION_ITEM('')
SURFACE()
);
#1552=(
BOUNDED_SURFACE()
B_SPLINE_SURFACE(2,3,((#84291,#84292,#84293,#84294),(#84295,#84296,#84297,
#84298),(#84299,#84300,#84301,#84302)),.UNSPECIFIED.,.F.,.F.,.F.)
B_SPLINE_SURFACE_WITH_KNOTS((3,3),(4,4),(0.439204842985634,0.585079578178692),
(0.,1.),.UNSPECIFIED.)
GEOMETRIC_REPRESENTATION_ITEM()
RATIONAL_B_SPLINE_SURFACE(((1.,0.999894006880548,0.999894006880548,1.),
(1.,0.999894006880548,0.999894006880548,1.),(1.,0.999894006880548,0.999894006880548,
1.)))
REPRESENTATION_ITEM('')
SURFACE()
);
#1553=(
BOUNDED_SURFACE()
B_SPLINE_SURFACE(2,3,((#84304,#84305,#84306,#84307),(#84308,#84309,#84310,
#84311),(#84312,#84313,#84314,#84315)),.UNSPECIFIED.,.F.,.F.,.F.)
B_SPLINE_SURFACE_WITH_KNOTS((3,3),(4,4),(0.111781170302558,0.275355623142002),
(0.,1.),.UNSPECIFIED.)
GEOMETRIC_REPRESENTATION_ITEM()
RATIONAL_B_SPLINE_SURFACE(((1.,0.999855716855875,0.999855716855875,1.),
(1.,0.999855716855875,0.999855716855875,1.),(1.,0.999855716855875,0.999855716855875,
1.)))
REPRESENTATION_ITEM('')
SURFACE()
);
#1554=(
BOUNDED_SURFACE()
B_SPLINE_SURFACE(2,3,((#84317,#84318,#84319,#84320),(#84321,#84322,#84323,
#84324),(#84325,#84326,#84327,#84328)),.UNSPECIFIED.,.F.,.F.,.F.)
B_SPLINE_SURFACE_WITH_KNOTS((3,3),(4,4),(0.437631507199148,0.58331506862024),
(0.,1.),.UNSPECIFIED.)
GEOMETRIC_REPRESENTATION_ITEM()
RATIONAL_B_SPLINE_SURFACE(((1.,0.999893875799735,0.999893875799735,1.),
(1.,0.999893875799735,0.999893875799735,1.),(1.,0.999893875799735,0.999893875799735,
1.)))
REPRESENTATION_ITEM('')
SURFACE()
);
#1555=(
BOUNDED_SURFACE()
B_SPLINE_SURFACE(2,3,((#84330,#84331,#84332,#84333),(#84334,#84335,#84336,
#84337),(#84338,#84339,#84340,#84341)),.UNSPECIFIED.,.F.,.F.,.F.)
B_SPLINE_SURFACE_WITH_KNOTS((3,3),(4,4),(0.109326350548543,0.273102821567692),
(0.,1.),.UNSPECIFIED.)
GEOMETRIC_REPRESENTATION_ITEM()
RATIONAL_B_SPLINE_SURFACE(((1.,0.999856457285684,0.999856457285684,1.),
(1.,0.999856457285684,0.999856457285684,1.),(1.,0.999856457285684,0.999856457285684,
1.)))
REPRESENTATION_ITEM('')
SURFACE()
);
#1556=(
BOUNDED_SURFACE()
B_SPLINE_SURFACE(2,3,((#84343,#84344,#84345,#84346),(#84347,#84348,#84349,
#84350),(#84351,#84352,#84353,#84354)),.UNSPECIFIED.,.F.,.F.,.F.)
B_SPLINE_SURFACE_WITH_KNOTS((3,3),(4,4),(0.4362431045186,0.582003553328225),
(0.,1.),.UNSPECIFIED.)
GEOMETRIC_REPRESENTATION_ITEM()
RATIONAL_B_SPLINE_SURFACE(((1.,0.999894314506178,0.999894314506178,1.),
(1.,0.999894314506178,0.999894314506178,1.),(1.,0.999894314506178,0.999894314506178,
1.)))
REPRESENTATION_ITEM('')
SURFACE()
);
#1557=(
BOUNDED_SURFACE()
B_SPLINE_SURFACE(2,3,((#84356,#84357,#84358,#84359),(#84360,#84361,#84362,
#84363),(#84364,#84365,#84366,#84367)),.UNSPECIFIED.,.F.,.F.,.F.)
B_SPLINE_SURFACE_WITH_KNOTS((3,3),(4,4),(0.107751460645953,0.271675591859108),
(0.,1.),.UNSPECIFIED.)
GEOMETRIC_REPRESENTATION_ITEM()
RATIONAL_B_SPLINE_SURFACE(((1.,0.999855488146839,0.999855488146839,1.),
(1.,0.999855488146839,0.999855488146839,1.),(1.,0.999855488146839,0.999855488146839,
1.)))
REPRESENTATION_ITEM('')
SURFACE()
);
#1558=(
BOUNDED_SURFACE()
B_SPLINE_SURFACE(2,3,((#84369,#84370,#84371,#84372),(#84373,#84374,#84375,
#84376),(#84377,#84378,#84379,#84380)),.UNSPECIFIED.,.F.,.F.,.F.)
B_SPLINE_SURFACE_WITH_KNOTS((3,3),(4,4),(0.435648728780737,0.581287225202112),
(0.,1.),.UNSPECIFIED.)
GEOMETRIC_REPRESENTATION_ITEM()
RATIONAL_B_SPLINE_SURFACE(((1.,0.999893801137434,0.999893801137434,1.),
(1.,0.999893801137434,0.999893801137434,1.),(1.,0.999893801137434,0.999893801137434,
1.)))
REPRESENTATION_ITEM('')
SURFACE()
);
#1559=(
BOUNDED_SURFACE()
B_SPLINE_SURFACE(2,3,((#84382,#84383,#84384,#84385),(#84386,#84387,#84388,
#84389),(#84390,#84391,#84392,#84393)),.UNSPECIFIED.,.F.,.F.,.F.)
B_SPLINE_SURFACE_WITH_KNOTS((3,3),(4,4),(0.106721261020608,0.270558651464622),
(0.,1.),.UNSPECIFIED.)
GEOMETRIC_REPRESENTATION_ITEM()
RATIONAL_B_SPLINE_SURFACE(((1.,0.999855390875252,0.999855390875252,1.),
(1.,0.999855390875252,0.999855390875252,1.),(1.,0.999855390875252,0.999855390875252,
1.)))
REPRESENTATION_ITEM('')
SURFACE()
);
#1560=(
BOUNDED_SURFACE()
B_SPLINE_SURFACE(2,3,((#84397,#84398,#84399,#84400),(#84401,#84402,#84403,
#84404),(#84405,#84406,#84407,#84408)),.UNSPECIFIED.,.F.,.F.,.F.)
B_SPLINE_SURFACE_WITH_KNOTS((3,3),(4,4),(0.435592989219888,0.580856308187753),
(0.,1.),.UNSPECIFIED.)
GEOMETRIC_REPRESENTATION_ITEM()
RATIONAL_B_SPLINE_SURFACE(((1.,0.999893836126727,0.999893836126727,1.),
(1.,0.999893836126727,0.999893836126727,1.),(1.,0.999893836126727,0.999893836126727,
1.)))
REPRESENTATION_ITEM('')
SURFACE()
);
#1561=(
BOUNDED_SURFACE()
B_SPLINE_SURFACE(2,3,((#84410,#84411,#84412,#84413),(#84414,#84415,#84416,
#84417),(#84418,#84419,#84420,#84421)),.UNSPECIFIED.,.F.,.F.,.F.)
B_SPLINE_SURFACE_WITH_KNOTS((3,3),(4,4),(0.106356611558605,0.270154561740801),
(0.,1.),.UNSPECIFIED.)
GEOMETRIC_REPRESENTATION_ITEM()
RATIONAL_B_SPLINE_SURFACE(((1.,0.999856152844613,0.999856152844613,1.),
(1.,0.999856152844613,0.999856152844613,1.),(1.,0.999856152844613,0.999856152844613,
1.)))
REPRESENTATION_ITEM('')
SURFACE()
);
#1562=(
BOUNDED_SURFACE()
B_SPLINE_SURFACE(2,3,((#84425,#84426,#84427,#84428),(#84429,#84430,#84431,
#84432),(#84433,#84434,#84435,#84436)),.UNSPECIFIED.,.F.,.F.,.F.)
B_SPLINE_SURFACE_WITH_KNOTS((3,3),(4,4),(0.435593699966305,0.581365752295347),
(0.,1.),.UNSPECIFIED.)
GEOMETRIC_REPRESENTATION_ITEM()
RATIONAL_B_SPLINE_SURFACE(((1.,0.999894372975926,0.999894372975926,1.),
(1.,0.999894372975926,0.999894372975926,1.),(1.,0.999894372975926,0.999894372975926,
1.)))
REPRESENTATION_ITEM('')
SURFACE()
);
#1563=(
BOUNDED_SURFACE()
B_SPLINE_SURFACE(2,3,((#84438,#84439,#84440,#84441),(#84442,#84443,#84444,
#84445),(#84446,#84447,#84448,#84449)),.UNSPECIFIED.,.F.,.F.,.F.)
B_SPLINE_SURFACE_WITH_KNOTS((3,3),(4,4),(0.10645020218376,0.269987102818262),
(0.,1.),.UNSPECIFIED.)
GEOMETRIC_REPRESENTATION_ITEM()
RATIONAL_B_SPLINE_SURFACE(((1.,0.999855425942098,0.999855425942098,1.),
(1.,0.999855425942098,0.999855425942098,1.),(1.,0.999855425942098,0.999855425942098,
1.)))
REPRESENTATION_ITEM('')
SURFACE()
);
#1564=(
BOUNDED_SURFACE()
B_SPLINE_SURFACE(2,3,((#84455,#84456,#84457,#84458),(#84459,#84460,#84461,
#84462),(#84463,#84464,#84465,#84466)),.UNSPECIFIED.,.F.,.F.,.F.)
B_SPLINE_SURFACE_WITH_KNOTS((3,3),(4,4),(0.43676522787172,0.582408838010634),
(0.,1.),.UNSPECIFIED.)
GEOMETRIC_REPRESENTATION_ITEM()
RATIONAL_B_SPLINE_SURFACE(((1.,0.999893765134106,0.999893765134106,1.),
(1.,0.999893765134106,0.999893765134106,1.),(1.,0.999893765134106,0.999893765134106,
1.)))
REPRESENTATION_ITEM('')
SURFACE()
);
#1565=(
BOUNDED_SURFACE()
B_SPLINE_SURFACE(2,3,((#84468,#84469,#84470,#84471),(#84472,#84473,#84474,
#84475),(#84476,#84477,#84478,#84479)),.UNSPECIFIED.,.F.,.F.,.F.)
B_SPLINE_SURFACE_WITH_KNOTS((3,3),(4,4),(0.106848672671777,0.270925177669003),
(0.,1.),.UNSPECIFIED.)
GEOMETRIC_REPRESENTATION_ITEM()
RATIONAL_B_SPLINE_SURFACE(((1.,0.999855651237632,0.999855651237632,1.),
(1.,0.999855651237632,0.999855651237632,1.),(1.,0.999855651237632,0.999855651237632,
1.)))
REPRESENTATION_ITEM('')
SURFACE()
);
#1566=(
BOUNDED_SURFACE()
B_SPLINE_SURFACE(2,3,((#84485,#84486,#84487,#84488),(#84489,#84490,#84491,
#84492),(#84493,#84494,#84495,#84496)),.UNSPECIFIED.,.F.,.F.,.F.)
B_SPLINE_SURFACE_WITH_KNOTS((3,3),(4,4),(0.437930879651441,0.583845036959533),
(0.,1.),.UNSPECIFIED.)
GEOMETRIC_REPRESENTATION_ITEM()
RATIONAL_B_SPLINE_SURFACE(((1.,0.999894219919845,0.999894219919845,1.),
(1.,0.999894219919845,0.999894219919845,1.),(1.,0.999894219919845,0.999894219919845,
1.)))
REPRESENTATION_ITEM('')
SURFACE()
);
#1567=(
BOUNDED_SURFACE()
B_SPLINE_SURFACE(2,3,((#84498,#84499,#84500,#84501),(#84502,#84503,#84504,
#84505),(#84506,#84507,#84508,#84509)),.UNSPECIFIED.,.F.,.F.,.F.)
B_SPLINE_SURFACE_WITH_KNOTS((3,3),(4,4),(0.108080512552553,0.271754524433647),
(0.,1.),.UNSPECIFIED.)
GEOMETRIC_REPRESENTATION_ITEM()
RATIONAL_B_SPLINE_SURFACE(((1.,0.999855950268206,0.999855950268206,1.),
(1.,0.999855950268206,0.999855950268206,1.),(1.,0.999855950268206,0.999855950268206,
1.)))
REPRESENTATION_ITEM('')
SURFACE()
);
#1568=(
BOUNDED_SURFACE()
B_SPLINE_SURFACE(2,3,((#84511,#84512,#84513,#84514),(#84515,#84516,#84517,
#84518),(#84519,#84520,#84521,#84522)),.UNSPECIFIED.,.F.,.F.,.F.)
B_SPLINE_SURFACE_WITH_KNOTS((3,3),(4,4),(0.439818550318335,0.585360171796468),
(0.,1.),.UNSPECIFIED.)
GEOMETRIC_REPRESENTATION_ITEM()
RATIONAL_B_SPLINE_SURFACE(((1.,0.999894184107649,0.999894184107649,1.),
(1.,0.999894184107649,0.999894184107649,1.),(1.,0.999894184107649,0.999894184107649,
1.)))
REPRESENTATION_ITEM('')
SURFACE()
);
#1569=(
BOUNDED_SURFACE()
B_SPLINE_SURFACE(2,3,((#84524,#84525,#84526,#84527),(#84528,#84529,#84530,
#84531),(#84532,#84533,#84534,#84535)),.UNSPECIFIED.,.F.,.F.,.F.)
B_SPLINE_SURFACE_WITH_KNOTS((3,3),(4,4),(0.110237303004777,0.27386314548445),
(0.,1.),.UNSPECIFIED.)
GEOMETRIC_REPRESENTATION_ITEM()
RATIONAL_B_SPLINE_SURFACE(((1.,0.999855610234961,0.999855610234961,1.),
(1.,0.999855610234961,0.999855610234961,1.),(1.,0.999855610234961,0.999855610234961,
1.)))
REPRESENTATION_ITEM('')
SURFACE()
);
#1570=(
BOUNDED_SURFACE()
B_SPLINE_SURFACE(2,3,((#84537,#84538,#84539,#84540),(#84541,#84542,#84543,
#84544),(#84545,#84546,#84547,#84548)),.UNSPECIFIED.,.F.,.F.,.F.)
B_SPLINE_SURFACE_WITH_KNOTS((3,3),(4,4),(0.442417506739257,0.587930688159455),
(0.,1.),.UNSPECIFIED.)
GEOMETRIC_REPRESENTATION_ITEM()
RATIONAL_B_SPLINE_SURFACE(((1.,0.999894126686531,0.999894126686531,1.),
(1.,0.999894126686531,0.999894126686531,1.),(1.,0.999894126686531,0.999894126686531,
1.)))
REPRESENTATION_ITEM('')
SURFACE()
);
#1571=(
BOUNDED_SURFACE()
B_SPLINE_SURFACE(2,3,((#84550,#84551,#84552,#84553),(#84554,#84555,#84556,
#84557),(#84558,#84559,#84560,#84561)),.UNSPECIFIED.,.F.,.F.,.F.)
B_SPLINE_SURFACE_WITH_KNOTS((3,3),(4,4),(0.112034372975308,0.275982742979846),
(0.,1.),.UNSPECIFIED.)
GEOMETRIC_REPRESENTATION_ITEM()
RATIONAL_B_SPLINE_SURFACE(((1.,0.99985664856181,0.99985664856181,1.),(1.,
0.99985664856181,0.99985664856181,1.),(1.,0.99985664856181,0.99985664856181,
1.)))
REPRESENTATION_ITEM('')
SURFACE()
);
#1572=(
BOUNDED_SURFACE()
B_SPLINE_SURFACE(2,3,((#84563,#84564,#84565,#84566),(#84567,#84568,#84569,
#84570),(#84571,#84572,#84573,#84574)),.UNSPECIFIED.,.F.,.F.,.F.)
B_SPLINE_SURFACE_WITH_KNOTS((3,3),(4,4),(0.444647530372542,0.590398629876671),
(0.,1.),.UNSPECIFIED.)
GEOMETRIC_REPRESENTATION_ITEM()
RATIONAL_B_SPLINE_SURFACE(((1.,0.999894743750065,0.999894743750065,1.),
(1.,0.999894743750065,0.999894743750065,1.),(1.,0.999894743750065,0.999894743750065,
1.)))
REPRESENTATION_ITEM('')
SURFACE()
);
#1573=(
BOUNDED_SURFACE()
B_SPLINE_SURFACE(2,3,((#84576,#84577,#84578,#84579),(#84580,#84581,#84582,
#84583),(#84584,#84585,#84586,#84587)),.UNSPECIFIED.,.F.,.F.,.F.)
B_SPLINE_SURFACE_WITH_KNOTS((3,3),(4,4),(0.114586911656446,0.278222488663965),
(0.,1.),.UNSPECIFIED.)
GEOMETRIC_REPRESENTATION_ITEM()
RATIONAL_B_SPLINE_SURFACE(((1.,0.99985598038009,0.99985598038009,1.),(1.,
0.99985598038009,0.99985598038009,1.),(1.,0.99985598038009,0.99985598038009,
1.)))
REPRESENTATION_ITEM('')
SURFACE()
);
#1574=(
BOUNDED_SURFACE()
B_SPLINE_SURFACE(2,3,((#84589,#84590,#84591,#84592),(#84593,#84594,#84595,
#84596),(#84597,#84598,#84599,#84600)),.UNSPECIFIED.,.F.,.F.,.F.)
B_SPLINE_SURFACE_WITH_KNOTS((3,3),(4,4),(0.447384652812814,0.592887765650982),
(0.,1.),.UNSPECIFIED.)
GEOMETRIC_REPRESENTATION_ITEM()
RATIONAL_B_SPLINE_SURFACE(((1.,0.999894664792425,0.999894664792425,1.),
(1.,0.999894664792425,0.999894664792425,1.),(1.,0.999894664792425,0.999894664792425,
1.)))
REPRESENTATION_ITEM('')
SURFACE()
);
#1575=(
BOUNDED_SURFACE()
B_SPLINE_SURFACE(2,3,((#84602,#84603,#84604,#84605),(#84606,#84607,#84608,
#84609),(#84610,#84611,#84612,#84613)),.UNSPECIFIED.,.F.,.F.,.F.)
B_SPLINE_SURFACE_WITH_KNOTS((3,3),(4,4),(0.117361364034985,0.281017412150302),
(0.,1.),.UNSPECIFIED.)
GEOMETRIC_REPRESENTATION_ITEM()
RATIONAL_B_SPLINE_SURFACE(((1.,0.99985654046593,0.99985654046593,1.),(1.,
0.99985654046593,0.99985654046593,1.),(1.,0.99985654046593,0.99985654046593,
1.)))
REPRESENTATION_ITEM('')
SURFACE()
);
#1576=(
BOUNDED_SURFACE()
B_SPLINE_SURFACE(2,3,((#84615,#84616,#84617,#84618),(#84619,#84620,#84621,
#84622),(#84623,#84624,#84625,#84626)),.UNSPECIFIED.,.F.,.F.,.F.)
B_SPLINE_SURFACE_WITH_KNOTS((3,3),(4,4),(0.450061410330926,0.59563674968253),
(0.,1.),.UNSPECIFIED.)
GEOMETRIC_REPRESENTATION_ITEM()
RATIONAL_B_SPLINE_SURFACE(((1.,0.999895034648578,0.999895034648578,1.),
(1.,0.999895034648578,0.999895034648578,1.),(1.,0.999895034648578,0.999895034648578,
1.)))
REPRESENTATION_ITEM('')
SURFACE()
);
#1577=(
BOUNDED_SURFACE()
B_SPLINE_SURFACE(2,3,((#84628,#84629,#84630,#84631),(#84632,#84633,#84634,
#84635),(#84636,#84637,#84638,#84639)),.UNSPECIFIED.,.F.,.F.,.F.)
B_SPLINE_SURFACE_WITH_KNOTS((3,3),(4,4),(0.120146383290712,0.283727976150696),
(0.,1.),.UNSPECIFIED.)
GEOMETRIC_REPRESENTATION_ITEM()
RATIONAL_B_SPLINE_SURFACE(((1.,0.999857826216213,0.999857826216213,1.),
(1.,0.999857826216213,0.999857826216213,1.),(1.,0.999857826216213,0.999857826216213,
1.)))
REPRESENTATION_ITEM('')
SURFACE()
);
#1578=(
BOUNDED_SURFACE()
B_SPLINE_SURFACE(2,3,((#84641,#84642,#84643,#84644),(#84645,#84646,#84647,
#84648),(#84649,#84650,#84651,#84652)),.UNSPECIFIED.,.F.,.F.,.F.)
B_SPLINE_SURFACE_WITH_KNOTS((3,3),(4,4),(0.452662415799281,0.598065007501956),
(0.,1.),.UNSPECIFIED.)
GEOMETRIC_REPRESENTATION_ITEM()
RATIONAL_B_SPLINE_SURFACE(((1.,0.999894544464411,0.999894544464411,1.),
(1.,0.999894544464411,0.999894544464411,1.),(1.,0.999894544464411,0.999894544464411,
1.)))
REPRESENTATION_ITEM('')
SURFACE()
);
#1579=(
BOUNDED_SURFACE()
B_SPLINE_SURFACE(2,3,((#84654,#84655,#84656,#84657),(#84658,#84659,#84660,
#84661),(#84662,#84663,#84664,#84665)),.UNSPECIFIED.,.F.,.F.,.F.)
B_SPLINE_SURFACE_WITH_KNOTS((3,3),(4,4),(0.123248945302883,0.286626574700324),
(0.,1.),.UNSPECIFIED.)
GEOMETRIC_REPRESENTATION_ITEM()
RATIONAL_B_SPLINE_SURFACE(((1.,0.999857334762909,0.999857334762909,1.),
(1.,0.999857334762909,0.999857334762909,1.),(1.,0.999857334762909,0.999857334762909,
1.)))
REPRESENTATION_ITEM('')
SURFACE()
);
#1580=(
BOUNDED_SURFACE()
B_SPLINE_SURFACE(2,3,((#84667,#84668,#84669,#84670),(#84671,#84672,#84673,
#84674),(#84675,#84676,#84677,#84678)),.UNSPECIFIED.,.F.,.F.,.F.)
B_SPLINE_SURFACE_WITH_KNOTS((3,3),(4,4),(0.455532155630731,0.600703145607525),
(0.,1.),.UNSPECIFIED.)
GEOMETRIC_REPRESENTATION_ITEM()
RATIONAL_B_SPLINE_SURFACE(((1.,0.999895073920667,0.999895073920667,1.),
(1.,0.999895073920667,0.999895073920667,1.),(1.,0.999895073920667,0.999895073920667,
1.)))
REPRESENTATION_ITEM('')
SURFACE()
);
#1581=(
BOUNDED_SURFACE()
B_SPLINE_SURFACE(2,3,((#84680,#84681,#84682,#84683),(#84684,#84685,#84686,
#84687),(#84688,#84689,#84690,#84691)),.UNSPECIFIED.,.F.,.F.,.F.)
B_SPLINE_SURFACE_WITH_KNOTS((3,3),(4,4),(0.125578640126081,0.289268722273738),
(0.,1.),.UNSPECIFIED.)
GEOMETRIC_REPRESENTATION_ITEM()
RATIONAL_B_SPLINE_SURFACE(((1.,0.999857143537026,0.999857143537026,1.),
(1.,0.999857143537026,0.999857143537026,1.),(1.,0.999857143537026,0.999857143537026,
1.)))
REPRESENTATION_ITEM('')
SURFACE()
);
#1582=(
BOUNDED_SURFACE()
B_SPLINE_SURFACE(2,3,((#84693,#84694,#84695,#84696),(#84697,#84698,#84699,
#84700),(#84701,#84702,#84703,#84704)),.UNSPECIFIED.,.F.,.F.,.F.)
B_SPLINE_SURFACE_WITH_KNOTS((3,3),(4,4),(0.45725674537802,0.602810602402847),
(0.,1.),.UNSPECIFIED.)
GEOMETRIC_REPRESENTATION_ITEM()
RATIONAL_B_SPLINE_SURFACE(((1.,0.999895364461255,0.999895364461255,1.),
(1.,0.999895364461255,0.999895364461255,1.),(1.,0.999895364461255,0.999895364461255,
1.)))
REPRESENTATION_ITEM('')
SURFACE()
);
#1583=(
BOUNDED_SURFACE()
B_SPLINE_SURFACE(2,3,((#84706,#84707,#84708,#84709),(#84710,#84711,#84712,
#84713),(#84714,#84715,#84716,#84717)),.UNSPECIFIED.,.F.,.F.,.F.)
B_SPLINE_SURFACE_WITH_KNOTS((3,3),(4,4),(0.128000754786,0.291182820426702),
(0.,1.),.UNSPECIFIED.)
GEOMETRIC_REPRESENTATION_ITEM()
RATIONAL_B_SPLINE_SURFACE(((1.,0.999856825985705,0.999856825985705,1.),
(1.,0.999856825985705,0.999856825985705,1.),(1.,0.999856825985705,0.999856825985705,
1.)))
REPRESENTATION_ITEM('')
SURFACE()
);
#1584=(
BOUNDED_SURFACE()
B_SPLINE_SURFACE(2,3,((#84719,#84720,#84721,#84722),(#84723,#84724,#84725,
#84726),(#84727,#84728,#84729,#84730)),.UNSPECIFIED.,.F.,.F.,.F.)
B_SPLINE_SURFACE_WITH_KNOTS((3,3),(4,4),(0.459038110287163,0.604290998985184),
(0.,1.),.UNSPECIFIED.)
GEOMETRIC_REPRESENTATION_ITEM()
RATIONAL_B_SPLINE_SURFACE(((1.,0.999895063286365,0.999895063286365,1.),
(1.,0.999895063286365,0.999895063286365,1.),(1.,0.999895063286365,0.999895063286365,
1.)))
REPRESENTATION_ITEM('')
SURFACE()
);
#1585=(
BOUNDED_SURFACE()
B_SPLINE_SURFACE(2,3,((#84732,#84733,#84734,#84735),(#84736,#84737,#84738,
#84739),(#84740,#84741,#84742,#84743)),.UNSPECIFIED.,.F.,.F.,.F.)
B_SPLINE_SURFACE_WITH_KNOTS((3,3),(4,4),(0.130338341892577,0.293624277563459),
(0.,1.),.UNSPECIFIED.)
GEOMETRIC_REPRESENTATION_ITEM()
RATIONAL_B_SPLINE_SURFACE(((1.,0.99985730936314,0.99985730936314,1.),(1.,
0.99985730936314,0.99985730936314,1.),(1.,0.99985730936314,0.99985730936314,
1.)))
REPRESENTATION_ITEM('')
SURFACE()
);
#1586=(
BOUNDED_SURFACE()
B_SPLINE_SURFACE(2,3,((#84745,#84746,#84747,#84748),(#84749,#84750,#84751,
#84752),(#84753,#84754,#84755,#84756)),.UNSPECIFIED.,.F.,.F.,.F.)
B_SPLINE_SURFACE_WITH_KNOTS((3,3),(4,4),(0.46039588922153,0.605713534640108),
(0.,1.),.UNSPECIFIED.)
GEOMETRIC_REPRESENTATION_ITEM()
RATIONAL_B_SPLINE_SURFACE(((1.,0.999895090466177,0.999895090466177,1.),
(1.,0.999895090466177,0.999895090466177,1.),(1.,0.999895090466177,0.999895090466177,
1.)))
REPRESENTATION_ITEM('')
SURFACE()
);
#1587=(
BOUNDED_SURFACE()
B_SPLINE_SURFACE(2,3,((#84758,#84759,#84760,#84761),(#84762,#84763,#84764,
#84765),(#84766,#84767,#84768,#84769)),.UNSPECIFIED.,.F.,.F.,.F.)
B_SPLINE_SURFACE_WITH_KNOTS((3,3),(4,4),(0.131726348549557,0.295159314599406),
(0.,1.),.UNSPECIFIED.)
GEOMETRIC_REPRESENTATION_ITEM()
RATIONAL_B_SPLINE_SURFACE(((1.,0.999857853682077,0.999857853682077,1.),
(1.,0.999857853682077,0.999857853682077,1.),(1.,0.999857853682077,0.999857853682077,
1.)))
REPRESENTATION_ITEM('')
SURFACE()
);
#1588=(
BOUNDED_SURFACE()
B_SPLINE_SURFACE(2,3,((#84771,#84772,#84773,#84774),(#84775,#84776,#84777,
#84778),(#84779,#84780,#84781,#84782)),.UNSPECIFIED.,.F.,.F.,.F.)
B_SPLINE_SURFACE_WITH_KNOTS((3,3),(4,4),(0.461107076972092,0.606286854344933),
(0.,1.),.UNSPECIFIED.)
GEOMETRIC_REPRESENTATION_ITEM()
RATIONAL_B_SPLINE_SURFACE(((1.,0.999895120190421,0.999895120190421,1.),
(1.,0.999895120190421,0.999895120190421,1.),(1.,0.999895120190421,0.999895120190421,
1.)))
REPRESENTATION_ITEM('')
SURFACE()
);
#1589=(
BOUNDED_SURFACE()
B_SPLINE_SURFACE(2,3,((#84784,#84785,#84786,#84787),(#84788,#84789,#84790,
#84791),(#84792,#84793,#84794,#84795)),.UNSPECIFIED.,.F.,.F.,.F.)
B_SPLINE_SURFACE_WITH_KNOTS((3,3),(4,4),(0.132862776548585,0.29611733043446),
(0.,1.),.UNSPECIFIED.)
GEOMETRIC_REPRESENTATION_ITEM()
RATIONAL_B_SPLINE_SURFACE(((1.,0.999857587798397,0.999857587798397,1.),
(1.,0.999857587798397,0.999857587798397,1.),(1.,0.999857587798397,0.999857587798397,
1.)))
REPRESENTATION_ITEM('')
SURFACE()
);
#1590=(
BOUNDED_SURFACE()
B_SPLINE_SURFACE(2,3,((#84797,#84798,#84799,#84800),(#84801,#84802,#84803,
#84804),(#84805,#84806,#84807,#84808)),.UNSPECIFIED.,.F.,.F.,.F.)
B_SPLINE_SURFACE_WITH_KNOTS((3,3),(4,4),(0.46154805509299,0.606328036429091),
(0.,1.),.UNSPECIFIED.)
GEOMETRIC_REPRESENTATION_ITEM()
RATIONAL_B_SPLINE_SURFACE(((1.,0.999895578580056,0.999895578580056,1.),
(1.,0.999895578580056,0.999895578580056,1.),(1.,0.999895578580056,0.999895578580056,
1.)))
REPRESENTATION_ITEM('')
SURFACE()
);
#1591=(
BOUNDED_SURFACE()
B_SPLINE_SURFACE(2,3,((#84810,#84811,#84812,#84813),(#84814,#84815,#84816,
#84817),(#84818,#84819,#84820,#84821)),.UNSPECIFIED.,.F.,.F.,.F.)
B_SPLINE_SURFACE_WITH_KNOTS((3,3),(4,4),(0.133282157276565,0.296502083979664),
(0.,1.),.UNSPECIFIED.)
GEOMETRIC_REPRESENTATION_ITEM()
RATIONAL_B_SPLINE_SURFACE(((1.,0.999857405537845,0.999857405537845,1.),
(1.,0.999857405537845,0.999857405537845,1.),(1.,0.999857405537845,0.999857405537845,
1.)))
REPRESENTATION_ITEM('')
SURFACE()
);
#1592=(
BOUNDED_SURFACE()
B_SPLINE_SURFACE(2,3,((#84823,#84824,#84825,#84826),(#84827,#84828,#84829,
#84830),(#84831,#84832,#84833,#84834)),.UNSPECIFIED.,.F.,.F.,.F.)
B_SPLINE_SURFACE_WITH_KNOTS((3,3),(4,4),(0.461051817256631,0.606319374173236),
(0.,1.),.UNSPECIFIED.)
GEOMETRIC_REPRESENTATION_ITEM()
RATIONAL_B_SPLINE_SURFACE(((1.,0.999895294476726,0.999895294476726,1.),
(1.,0.999895294476726,0.999895294476726,1.),(1.,0.999895294476726,0.999895294476726,
1.)))
REPRESENTATION_ITEM('')
SURFACE()
);
#1593=(
BOUNDED_SURFACE()
B_SPLINE_SURFACE(2,3,((#84836,#84837,#84838,#84839),(#84840,#84841,#84842,
#84843),(#84844,#84845,#84846,#84847)),.UNSPECIFIED.,.F.,.F.,.F.)
B_SPLINE_SURFACE_WITH_KNOTS((3,3),(4,4),(0.133462377346205,0.296408008484315),
(0.,1.),.UNSPECIFIED.)
GEOMETRIC_REPRESENTATION_ITEM()
RATIONAL_B_SPLINE_SURFACE(((1.,0.99985728327432,0.99985728327432,1.),(1.,
0.99985728327432,0.99985728327432,1.),(1.,0.99985728327432,0.99985728327432,
1.)))
REPRESENTATION_ITEM('')
SURFACE()
);
#1594=(
BOUNDED_SURFACE()
B_SPLINE_SURFACE(2,3,((#84849,#84850,#84851,#84852),(#84853,#84854,#84855,
#84856),(#84857,#84858,#84859,#84860)),.UNSPECIFIED.,.F.,.F.,.F.)
B_SPLINE_SURFACE_WITH_KNOTS((3,3),(4,4),(0.459951997369159,0.605164063679616),
(0.,1.),.UNSPECIFIED.)
GEOMETRIC_REPRESENTATION_ITEM()
RATIONAL_B_SPLINE_SURFACE(((1.,0.999894901788882,0.999894901788882,1.),
(1.,0.999894901788882,0.999894901788882,1.),(1.,0.999894901788882,0.999894901788882,
1.)))
REPRESENTATION_ITEM('')
SURFACE()
);
#1595=(
BOUNDED_SURFACE()
B_SPLINE_SURFACE(2,3,((#84862,#84863,#84864,#84865),(#84866,#84867,#84868,
#84869),(#84870,#84871,#84872,#84873)),.UNSPECIFIED.,.F.,.F.,.F.)
B_SPLINE_SURFACE_WITH_KNOTS((3,3),(4,4),(0.132492075185841,0.296014197565379),
(0.,1.),.UNSPECIFIED.)
GEOMETRIC_REPRESENTATION_ITEM()
RATIONAL_B_SPLINE_SURFACE(((1.,0.999857956642642,0.999857956642642,1.),
(1.,0.999857956642642,0.999857956642642,1.),(1.,0.999857956642642,0.999857956642642,
1.)))
REPRESENTATION_ITEM('')
SURFACE()
);
#1596=(
BOUNDED_SURFACE()
B_SPLINE_SURFACE(2,3,((#84875,#84876,#84877,#84878),(#84879,#84880,#84881,
#84882),(#84883,#84884,#84885,#84886)),.UNSPECIFIED.,.F.,.F.,.F.)
B_SPLINE_SURFACE_WITH_KNOTS((3,3),(4,4),(0.458503447428235,0.604044265656637),
(0.,1.),.UNSPECIFIED.)
GEOMETRIC_REPRESENTATION_ITEM()
RATIONAL_B_SPLINE_SURFACE(((1.,0.99989525299666,0.99989525299666,1.),(1.,
0.99989525299666,0.99989525299666,1.),(1.,0.99989525299666,0.99989525299666,
1.)))
REPRESENTATION_ITEM('')
SURFACE()
);
#1597=(
BOUNDED_SURFACE()
B_SPLINE_SURFACE(2,3,((#84888,#84889,#84890,#84891),(#84892,#84893,#84894,
#84895),(#84896,#84897,#84898,#84899)),.UNSPECIFIED.,.F.,.F.,.F.)
B_SPLINE_SURFACE_WITH_KNOTS((3,3),(4,4),(0.13173580484991,0.294818644607769),
(0.,1.),.UNSPECIFIED.)
GEOMETRIC_REPRESENTATION_ITEM()
RATIONAL_B_SPLINE_SURFACE(((1.,0.999857776424627,0.999857776424627,1.),
(1.,0.999857776424627,0.999857776424627,1.),(1.,0.999857776424627,0.999857776424627,
1.)))
REPRESENTATION_ITEM('')
SURFACE()
);
#1598=(
BOUNDED_SURFACE()
B_SPLINE_SURFACE(2,3,((#84901,#84902,#84903,#84904),(#84905,#84906,#84907,
#84908),(#84909,#84910,#84911,#84912)),.UNSPECIFIED.,.F.,.F.,.F.)
B_SPLINE_SURFACE_WITH_KNOTS((3,3),(4,4),(0.457070219990733,0.602201786761517),
(0.,1.),.UNSPECIFIED.)
GEOMETRIC_REPRESENTATION_ITEM()
RATIONAL_B_SPLINE_SURFACE(((1.,0.999895375004805,0.999895375004805,1.),
(1.,0.999895375004805,0.999895375004805,1.),(1.,0.999895375004805,0.999895375004805,
1.)))
REPRESENTATION_ITEM('')
SURFACE()
);
#1599=(
BOUNDED_SURFACE()
B_SPLINE_SURFACE(2,3,((#84914,#84915,#84916,#84917),(#84918,#84919,#84920,
#84921),(#84922,#84923,#84924,#84925)),.UNSPECIFIED.,.F.,.F.,.F.)
B_SPLINE_SURFACE_WITH_KNOTS((3,3),(4,4),(0.129525912426222,0.29278263731982),
(0.,1.),.UNSPECIFIED.)
GEOMETRIC_REPRESENTATION_ITEM()
RATIONAL_B_SPLINE_SURFACE(((1.,0.999856990812476,0.999856990812476,1.),
(1.,0.999856990812476,0.999856990812476,1.),(1.,0.999856990812476,0.999856990812476,
1.)))
REPRESENTATION_ITEM('')
SURFACE()
);
#1600=(
BOUNDED_SURFACE()
B_SPLINE_SURFACE(2,3,((#84927,#84928,#84929,#84930),(#84931,#84932,#84933,
#84934),(#84935,#84936,#84937,#84938)),.UNSPECIFIED.,.F.,.F.,.F.)
B_SPLINE_SURFACE_WITH_KNOTS((3,3),(4,4),(0.454381854054376,0.599708978407689),
(0.,1.),.UNSPECIFIED.)
GEOMETRIC_REPRESENTATION_ITEM()
RATIONAL_B_SPLINE_SURFACE(((1.,0.999894752812304,0.999894752812304,1.),
(1.,0.999894752812304,0.999894752812304,1.),(1.,0.999894752812304,0.999894752812304,
1.)))
REPRESENTATION_ITEM('')
SURFACE()
);
#1601=(
BOUNDED_SURFACE()
B_SPLINE_SURFACE(2,3,((#84940,#84941,#84942,#84943),(#84944,#84945,#84946,
#84947),(#84948,#84949,#84950,#84951)),.UNSPECIFIED.,.F.,.F.,.F.)
B_SPLINE_SURFACE_WITH_KNOTS((3,3),(4,4),(0.127384118218686,0.29096643518866),
(0.,1.),.UNSPECIFIED.)
GEOMETRIC_REPRESENTATION_ITEM()
RATIONAL_B_SPLINE_SURFACE(((1.,0.999857013359022,0.999857013359022,1.),
(1.,0.999857013359022,0.999857013359022,1.),(1.,0.999857013359022,0.999857013359022,
1.)))
REPRESENTATION_ITEM('')
SURFACE()
);
#1602=(
BOUNDED_SURFACE()
B_SPLINE_SURFACE(2,3,((#84953,#84954,#84955,#84956),(#84957,#84958,#84959,
#84960),(#84961,#84962,#84963,#84964)),.UNSPECIFIED.,.F.,.F.,.F.)
B_SPLINE_SURFACE_WITH_KNOTS((3,3),(4,4),(0.451885461485502,0.597476529771293),
(0.,1.),.UNSPECIFIED.)
GEOMETRIC_REPRESENTATION_ITEM()
RATIONAL_B_SPLINE_SURFACE(((1.,0.999894655481396,0.999894655481396,1.),
(1.,0.999894655481396,0.999894655481396,1.),(1.,0.999894655481396,0.999894655481396,
1.)))
REPRESENTATION_ITEM('')
SURFACE()
);
#1603=(
BOUNDED_SURFACE()
B_SPLINE_SURFACE(2,3,((#84966,#84967,#84968,#84969),(#84970,#84971,#84972,
#84973),(#84974,#84975,#84976,#84977)),.UNSPECIFIED.,.F.,.F.,.F.)
B_SPLINE_SURFACE_WITH_KNOTS((3,3),(4,4),(0.125053932102849,0.288479498956097),
(0.,1.),.UNSPECIFIED.)
GEOMETRIC_REPRESENTATION_ITEM()
RATIONAL_B_SPLINE_SURFACE(((1.,0.999857122345165,0.999857122345165,1.),
(1.,0.999857122345165,0.999857122345165,1.),(1.,0.999857122345165,0.999857122345165,
1.)))
REPRESENTATION_ITEM('')
SURFACE()
);
#1604=(
BOUNDED_SURFACE()
B_SPLINE_SURFACE(2,3,((#84979,#84980,#84981,#84982),(#84983,#84984,#84985,
#84986),(#84987,#84988,#84989,#84990)),.UNSPECIFIED.,.F.,.F.,.F.)
B_SPLINE_SURFACE_WITH_KNOTS((3,3),(4,4),(0.449312907381874,0.594798425786394),
(0.,1.),.UNSPECIFIED.)
GEOMETRIC_REPRESENTATION_ITEM()
RATIONAL_B_SPLINE_SURFACE(((1.,0.999894852716433,0.999894852716433,1.),
(1.,0.999894852716433,0.999894852716433,1.),(1.,0.999894852716433,0.999894852716433,
1.)))
REPRESENTATION_ITEM('')
SURFACE()
);
#1808=B_SPLINE_CURVE_WITH_KNOTS('',3,(#65625,#65626,#65627,#65628,#65629,
#65630,#65631,#65632,#65633,#65634,#65635,#65636,#65637,#65638,#65639,#65640,
#65641,#65642,#65643,#65644,#65645),.UNSPECIFIED.,.F.,.F.,(4,2,2,2,2,2,
2,2,3,4),(-0.301207075635748,-0.262710648076985,-0.224963089028706,-0.187920887348923,
-0.151298118741226,-0.114507144214601,-0.0770611386627541,-0.0389186460799617,
0.,0.000154759158804522),.UNSPECIFIED.);
#1809=B_SPLINE_CURVE_WITH_KNOTS('',3,(#65648,#65649,#65650,#65651,#65652,
#65653,#65654,#65655,#65656,#65657,#65658,#65659,#65660,#65661,#65662,#65663,
#65664,#65665,#65666,#65667,#65668,#65669,#65670,#65671,#65672,#65673,#65674,
#65675,#65676,#65677,#65678,#65679,#65680,#65681,#65682,#65683),
 .UNSPECIFIED.,.T.,.F.,(4,2,2,2,2,2,2,2,2,2,2,2,2,2,2,2,2,4),(0.,0.0355202696276814,
0.0730229242192624,0.109881947978595,0.147332215352117,0.185244244852364,
0.223245130807779,0.259644256147526,0.294838797511801,0.330228485407574,
0.366554345821638,0.404791218300025,0.442165216596553,0.480056587425708,
0.518291371447407,0.552548743077857,0.58852966840272,0.599949959198704),
 .UNSPECIFIED.);
#1810=B_SPLINE_CURVE_WITH_KNOTS('',3,(#65684,#65685,#65686,#65687,#65688,
#65689,#65690,#65691,#65692,#65693,#65694,#65695,#65696,#65697,#65698,#65699,
#65700,#65701,#65702,#65703),.UNSPECIFIED.,.F.,.F.,(4,2,2,2,2,2,2,2,2,4),
(0.000154759158804522,0.0372889614373737,0.0752199300055963,0.112924529730869,
0.149859365579758,0.187155736640999,0.224850670418274,0.262646502930588,
0.300853550272872,0.301114086264827),.UNSPECIFIED.);
#1811=B_SPLINE_CURVE_WITH_KNOTS('',3,(#65709,#65710,#65711,#65712,#65713,
#65714,#65715,#65716,#65717,#65718,#65719,#65720,#65721,#65722,#65723,#65724,
#65725,#65726,#65727,#65728,#65729,#65730,#65731,#65732,#65733,#65734,#65735,
#65736,#65737,#65738,#65739,#65740,#65741,#65742),.UNSPECIFIED.,.T.,.F.,
(4,2,2,2,2,2,2,2,2,2,2,2,2,2,2,2,4),(-0.31764321474939,-0.297585218798245,
-0.277672851988763,-0.258107799080609,-0.238754678175866,-0.21934156864919,
-0.199630721249192,-0.179486526168813,-0.159056300074024,-0.13875563311955,
-0.118621969325576,-0.0989972178555827,-0.0795589853250667,-0.0601192898607882,
-0.040316055511345,-0.0202331842178355,0.),.UNSPECIFIED.);
#1812=B_SPLINE_CURVE_WITH_KNOTS('',3,(#65746,#65747,#65748,#65749,#65750,
#65751,#65752,#65753,#65754,#65755,#65756,#65757,#65758,#65759,#65760,#65761,
#65762,#65763,#65764,#65765),.UNSPECIFIED.,.F.,.F.,(4,2,2,2,2,2,2,2,2,4),
(-0.322456793629602,-0.321930945694818,-0.281120714431957,-0.240874004386435,
-0.200756138465722,-0.160810087223787,-0.12089229981328,-0.0807982385809383,
-0.0404605678798725,-5.67197663269965E-6),.UNSPECIFIED.);
#1813=B_SPLINE_CURVE_WITH_KNOTS('',3,(#65768,#65769,#65770,#65771,#65772,
#65773,#65774,#65775,#65776,#65777,#65778,#65779,#65780,#65781,#65782,#65783,
#65784,#65785,#65786,#65787,#65788,#65789,#65790,#65791,#65792,#65793,#65794,
#65795,#65796,#65797,#65798,#65799,#65800,#65801,#65802,#65803),
 .UNSPECIFIED.,.T.,.F.,(4,2,2,2,2,2,2,2,2,2,2,2,2,2,2,2,2,4),(0.,0.0399541104209996,
0.0799101633968203,0.120042188030658,0.160349494009884,0.200700062460061,
0.240669149748206,0.281146928547698,0.321688268052451,0.361827692829584,
0.401937446248238,0.441912733331546,0.482224630786286,0.523014478227826,
0.563360237934725,0.603655558776063,0.623959945525968,0.644496878439197),
 .UNSPECIFIED.);
#1814=B_SPLINE_CURVE_WITH_KNOTS('',3,(#65804,#65805,#65806,#65807,#65808,
#65809,#65810,#65811,#65812,#65813,#65814,#65815,#65816,#65817,#65818,#65819,
#65820,#65821,#65822,#65823,#65824),.UNSPECIFIED.,.F.,.F.,(4,3,2,2,2,2,
2,2,2,4),(-5.67197663269965E-6,0.,0.0395310619276315,0.0803390393793353,
0.120710239662218,0.161056371560083,0.201562793815772,0.242068779839465,
0.282414440590624,0.322260650653274),.UNSPECIFIED.);
#1815=B_SPLINE_CURVE_WITH_KNOTS('',3,(#65830,#65831,#65832,#65833,#65834,
#65835,#65836,#65837,#65838,#65839,#65840,#65841,#65842,#65843,#65844,#65845,
#65846,#65847,#65848,#65849,#65850,#65851,#65852,#65853,#65854,#65855,#65856,
#65857,#65858,#65859,#65860,#65861,#65862,#65863),.UNSPECIFIED.,.T.,.F.,
(4,2,2,2,2,2,2,2,2,2,2,2,2,2,2,2,4),(-0.315589981954352,-0.297256657266753,
-0.277538667548594,-0.257873603172813,-0.238278181150012,-0.218708538295045,
-0.199094835855894,-0.179399406131129,-0.159642486979386,-0.139670907982114,
-0.119619104317766,-0.0996819381389054,-0.0797621233342936,-0.0598091169008165,
-0.039854339317345,-0.0199328473099917,0.),.UNSPECIFIED.);
#1816=B_SPLINE_CURVE_WITH_KNOTS('',3,(#65867,#65868,#65869,#65870,#65871,
#65872,#65873,#65874,#65875,#65876,#65877,#65878,#65879,#65880,#65881,#65882,
#65883,#65884,#65885,#65886,#65887,#65888,#65889),.UNSPECIFIED.,.F.,.F.,
(4,2,2,2,2,2,2,2,2,3,4),(-0.301165935385473,-0.300788234391116,-0.262281544053756,
-0.22421926833655,-0.186818821875507,-0.15004770924054,-0.113427897963337,
-0.0763613905919923,-0.0385473925034182,0.,0.000181127945344951),
 .UNSPECIFIED.);
#1817=B_SPLINE_CURVE_WITH_KNOTS('',3,(#65892,#65893,#65894,#65895,#65896,
#65897,#65898,#65899,#65900,#65901,#65902,#65903,#65904,#65905,#65906,#65907,
#65908,#65909,#65910,#65911,#65912,#65913,#65914,#65915,#65916,#65917,#65918,
#65919,#65920,#65921,#65922,#65923,#65924,#65925,#65926,#65927),
 .UNSPECIFIED.,.T.,.F.,(4,2,2,2,2,2,2,2,2,2,2,2,2,2,2,2,2,4),(0.,0.0355202696276384,
0.0730229242190651,0.109881947978276,0.14733221535191,0.18524424485214,
0.223245130807427,0.259644256147236,0.294838797511598,0.330228485407464,
0.366554345821612,0.4047912183001,0.442165216596848,0.480056587426246,0.518291371448191,
0.552548743078774,0.588529668403866,0.599949959199946),.UNSPECIFIED.);
#1818=B_SPLINE_CURVE_WITH_KNOTS('',3,(#65928,#65929,#65930,#65931,#65932,
#65933,#65934,#65935,#65936,#65937,#65938,#65939,#65940,#65941,#65942,#65943,
#65944,#65945),.UNSPECIFIED.,.F.,.F.,(4,2,2,2,2,2,2,2,4),(0.000181127945344951,
0.0376469167067535,0.0758399504044883,0.113626377029077,0.151312096065185,
0.18817171823677,0.225871250407431,0.263579914127532,0.301176733243773),
 .UNSPECIFIED.);
#1819=B_SPLINE_CURVE_WITH_KNOTS('',3,(#65951,#65952,#65953,#65954,#65955,
#65956,#65957,#65958,#65959,#65960,#65961,#65962,#65963,#65964,#65965,#65966,
#65967,#65968,#65969,#65970,#65971,#65972,#65973,#65974,#65975,#65976,#65977,
#65978,#65979,#65980,#65981,#65982,#65983,#65984),.UNSPECIFIED.,.T.,.F.,
(4,2,2,2,2,2,2,2,2,2,2,2,2,2,2,2,4),(-0.317651970798428,-0.29815178689123,
-0.277708377482877,-0.257961131709923,-0.238526287372716,-0.219184977021519,
-0.19965572209791,-0.179773340350517,-0.159321772514999,-0.13892751869627,
-0.118697905777899,-0.0986211371345974,-0.0791085006013058,-0.0596989356638533,
-0.0401874040480438,-0.0201536713619323,0.),.UNSPECIFIED.);
#1820=B_SPLINE_CURVE_WITH_KNOTS('',3,(#65988,#65989,#65990,#65991,#65992,
#65993,#65994,#65995,#65996,#65997,#65998,#65999,#66000,#66001,#66002,#66003,
#66004,#66005,#66006,#66007),.UNSPECIFIED.,.F.,.F.,(4,2,2,2,2,2,2,2,2,4),
(-0.322457248719835,-0.321529294029697,-0.281003068363887,-0.240747294879843,
-0.20053995746929,-0.160507771051919,-0.120603186514104,-0.0806274654213206,
-0.0404172639125648,-3.12966711858995E-5),.UNSPECIFIED.);
#1821=B_SPLINE_CURVE_WITH_KNOTS('',3,(#66010,#66011,#66012,#66013,#66014,
#66015,#66016,#66017,#66018,#66019,#66020,#66021,#66022,#66023,#66024,#66025,
#66026,#66027,#66028,#66029,#66030,#66031,#66032,#66033,#66034,#66035,#66036,
#66037,#66038,#66039,#66040,#66041,#66042,#66043,#66044,#66045),
 .UNSPECIFIED.,.T.,.F.,(4,2,2,2,2,2,2,2,2,2,2,2,2,2,2,2,2,4),(0.,0.0399541104211576,
0.0799101633974278,0.120042188031722,0.160349494011448,0.20070006246199,
0.240669149750381,0.281146928550143,0.321688268055072,0.361827692832458,
0.401937446251656,0.44191273333538,0.482224630790607,0.523014478232421,
0.563360237939489,0.603655558781071,0.623959945531265,0.644496878444614),
 .UNSPECIFIED.);
#1822=B_SPLINE_CURVE_WITH_KNOTS('',3,(#66046,#66047,#66048,#66049,#66050,
#66051,#66052,#66053,#66054,#66055,#66056,#66057,#66058,#66059,#66060,#66061,
#66062,#66063,#66064,#66065,#66066),.UNSPECIFIED.,.F.,.F.,(4,3,2,2,2,2,
2,2,2,4),(-3.12966711858995E-5,0.,0.0394735202592785,0.0806056751944302,
0.121148951974962,0.161462087232505,0.201894298596311,0.242442947719733,
0.282882236373443,0.322267164573172),.UNSPECIFIED.);
#1823=B_SPLINE_CURVE_WITH_KNOTS('',3,(#66072,#66073,#66074,#66075,#66076,
#66077,#66078,#66079,#66080,#66081,#66082,#66083,#66084,#66085,#66086,#66087,
#66088,#66089,#66090,#66091,#66092,#66093,#66094,#66095,#66096,#66097,#66098,
#66099,#66100,#66101,#66102,#66103,#66104,#66105),.UNSPECIFIED.,.T.,.F.,
(4,2,2,2,2,2,2,2,2,2,2,2,2,2,2,2,4),(-0.315593239578836,-0.297155229491326,
-0.277429616910152,-0.257728814722726,-0.238097547859077,-0.218523354285244,
-0.198942519291424,-0.179292718177143,-0.159563077843648,-0.139793456325068,
-0.119664685919836,-0.0996815350600369,-0.0797642526410489,-0.0598256812499414,
-0.0398597186100538,-0.0199163208441135,0.),.UNSPECIFIED.);
#1824=B_SPLINE_CURVE_WITH_KNOTS('',3,(#66109,#66110,#66111,#66112,#66113,
#66114,#66115,#66116,#66117,#66118,#66119,#66120,#66121,#66122,#66123,#66124,
#66125,#66126,#66127,#66128,#66129,#66130,#66131),.UNSPECIFIED.,.F.,.F.,
(4,2,2,2,2,2,2,2,2,3,4),(-0.301161917452386,-0.300838295583177,-0.262579133327298,
-0.223756342411398,-0.185991834148995,-0.14894433741301,-0.112334627077444,
-0.0755690315276266,-0.0381431397130738,0.,0.000141379885012664),
 .UNSPECIFIED.);
#1825=B_SPLINE_CURVE_WITH_KNOTS('',3,(#66134,#66135,#66136,#66137,#66138,
#66139,#66140,#66141,#66142,#66143,#66144,#66145,#66146,#66147,#66148,#66149,
#66150,#66151,#66152,#66153,#66154,#66155,#66156,#66157,#66158,#66159,#66160,
#66161,#66162,#66163,#66164,#66165,#66166,#66167,#66168,#66169),
 .UNSPECIFIED.,.T.,.F.,(4,2,2,2,2,2,2,2,2,2,2,2,2,2,2,2,2,4),(0.,0.035520269627735,
0.0730229242195194,0.109881947979011,0.147332215352631,0.185244244852754,
0.223245130808132,0.259644256148007,0.294838797512386,0.330228485408292,
0.366554345822388,0.404791218300835,0.442165216597801,0.480056587427053,
0.518291371449001,0.552548743079509,0.588529668404388,0.599949959200391),
 .UNSPECIFIED.);
#1826=B_SPLINE_CURVE_WITH_KNOTS('',3,(#66170,#66171,#66172,#66173,#66174,
#66175,#66176,#66177,#66178,#66179,#66180,#66181,#66182,#66183,#66184,#66185,
#66186,#66187),.UNSPECIFIED.,.F.,.F.,(4,2,2,2,2,2,2,2,4),(0.000141379885012664,
0.0375906403896581,0.0761417945336856,0.114138356543264,0.151831601486628,
0.188756872156502,0.226035096963817,0.263685590536988,0.301167081091413),
 .UNSPECIFIED.);
#1827=B_SPLINE_CURVE_WITH_KNOTS('',3,(#66193,#66194,#66195,#66196,#66197,
#66198,#66199,#66200,#66201,#66202,#66203,#66204,#66205,#66206,#66207,#66208,
#66209,#66210,#66211,#66212,#66213,#66214,#66215,#66216,#66217,#66218,#66219,
#66220,#66221,#66222,#66223,#66224,#66225,#66226),.UNSPECIFIED.,.T.,.F.,
(4,2,2,2,2,2,2,2,2,2,2,2,2,2,2,2,4),(-0.317642803625192,-0.297848684457,
-0.277420857385532,-0.257494471404098,-0.237922107431991,-0.218574026097491,
-0.199176141984307,-0.179480980704758,-0.159354591123693,-0.138883902901578,
-0.118529867925916,-0.0983635747576582,-0.0787362066700163,-0.0593026472197343,
-0.0398721579205076,-0.0200860310405472,0.),.UNSPECIFIED.);
#1828=B_SPLINE_CURVE_WITH_KNOTS('',3,(#66230,#66231,#66232,#66233,#66234,
#66235,#66236,#66237,#66238,#66239,#66240,#66241,#66242,#66243,#66244,#66245,
#66246,#66247,#66248,#66249,#66250,#66251,#66252),.UNSPECIFIED.,.F.,.F.,
(4,2,2,2,2,2,2,2,2,3,4),(-0.322302397770585,-0.321865205480829,-0.281475562271467,
-0.240625403307893,-0.200376862230115,-0.160259298530777,-0.120320752093,
-0.0804184780332567,-0.0403383378354368,0.,0.000100255797653548),
 .UNSPECIFIED.);
#1829=B_SPLINE_CURVE_WITH_KNOTS('',3,(#66255,#66256,#66257,#66258,#66259,
#66260,#66261,#66262,#66263,#66264,#66265,#66266,#66267,#66268,#66269,#66270,
#66271,#66272,#66273,#66274,#66275,#66276,#66277,#66278,#66279,#66280,#66281,
#66282,#66283,#66284,#66285,#66286,#66287,#66288,#66289,#66290),
 .UNSPECIFIED.,.T.,.F.,(4,2,2,2,2,2,2,2,2,2,2,2,2,2,2,2,2,4),(0.,0.0399541104210705,
0.0799101633969787,0.120042188030797,0.160349494010289,0.200700062460403,
0.240669149748371,0.281146928547758,0.321688268052559,0.361827692829776,
0.401937446248424,0.441912733331591,0.482224630786227,0.523014478227558,
0.56336023793413,0.603655558775227,0.623959945525105,0.64449687843833),
 .UNSPECIFIED.);
#1830=B_SPLINE_CURVE_WITH_KNOTS('',3,(#66291,#66292,#66293,#66294,#66295,
#66296,#66297,#66298,#66299,#66300,#66301,#66302,#66303,#66304,#66305,#66306,
#66307,#66308),.UNSPECIFIED.,.F.,.F.,(4,2,2,2,2,2,2,2,4),(0.000100255797653548,
0.0395671716758544,0.0800121271978018,0.120938471359253,0.16136281430439,
0.201675954298304,0.242101002732803,0.282537408146094,0.322421957479456),
 .UNSPECIFIED.);
#1831=B_SPLINE_CURVE_WITH_KNOTS('',3,(#66314,#66315,#66316,#66317,#66318,
#66319,#66320,#66321,#66322,#66323,#66324,#66325,#66326,#66327,#66328,#66329,
#66330,#66331,#66332,#66333,#66334,#66335,#66336,#66337,#66338,#66339,#66340,
#66341,#66342,#66343,#66344,#66345,#66346,#66347),.UNSPECIFIED.,.T.,.F.,
(4,2,2,2,2,2,2,2,2,2,2,2,2,2,2,2,4),(-0.315594444981776,-0.297150257709209,
-0.277089673960405,-0.257371001063089,-0.237708755743781,-0.218118780490078,
-0.198554739122427,-0.178943293168605,-0.159244534976724,-0.139480293177502,
-0.119705544795745,-0.0996065223937357,-0.0796463317455234,-0.0597393894595519,
-0.0398237825108839,-0.019905987916103,0.),.UNSPECIFIED.);
#1832=B_SPLINE_CURVE_WITH_KNOTS('',3,(#66351,#66352,#66353,#66354,#66355,
#66356,#66357,#66358,#66359,#66360,#66361,#66362,#66363,#66364,#66365,#66366,
#66367,#66368,#66369,#66370,#66371,#66372,#66373),.UNSPECIFIED.,.F.,.F.,
(4,2,2,2,2,2,2,2,2,3,4),(-0.301138647978451,-0.300148980683225,-0.262187460405049,
-0.223694248594581,-0.185606204515038,-0.148180061349361,-0.111404035321645,
-0.0748077387741857,-0.0377816370688137,0.,9.36180134758838E-5),
 .UNSPECIFIED.);
#1833=B_SPLINE_CURVE_WITH_KNOTS('',3,(#66376,#66377,#66378,#66379,#66380,
#66381,#66382,#66383,#66384,#66385,#66386,#66387,#66388,#66389,#66390,#66391,
#66392,#66393,#66394,#66395,#66396,#66397,#66398,#66399,#66400,#66401,#66402,
#66403,#66404,#66405,#66406,#66407,#66408,#66409,#66410,#66411),
 .UNSPECIFIED.,.T.,.F.,(4,2,2,2,2,2,2,2,2,2,2,2,2,2,2,2,2,4),(0.,0.0355202696276501,
0.0730229242191375,0.109881947978365,0.147332215351896,0.185244244852142,
0.223245130807564,0.259644256147409,0.294838797511695,0.330228485407438,
0.366554345821406,0.404791218299827,0.442165216596728,0.48005658742597,
0.518291371447828,0.552548743078327,0.588529668403252,0.599949959199292),
 .UNSPECIFIED.);
#1834=B_SPLINE_CURVE_WITH_KNOTS('',3,(#66412,#66413,#66414,#66415,#66416,
#66417,#66418,#66419,#66420,#66421,#66422,#66423,#66424,#66425,#66426,#66427,
#66428,#66429),.UNSPECIFIED.,.F.,.F.,(4,2,2,2,2,2,2,2,4),(9.36180134758838E-5,
0.0374299437225984,0.0762103935681948,0.114435762991268,0.152233330864938,
0.189908215887392,0.226754855658746,0.264441309346417,0.301150344435867),
 .UNSPECIFIED.);
#1835=B_SPLINE_CURVE_WITH_KNOTS('',3,(#66435,#66436,#66437,#66438,#66439,
#66440,#66441,#66442,#66443,#66444,#66445,#66446,#66447,#66448,#66449,#66450,
#66451,#66452,#66453,#66454,#66455,#66456,#66457,#66458,#66459,#66460,#66461,
#66462,#66463,#66464,#66465,#66466,#66467,#66468),.UNSPECIFIED.,.T.,.F.,
(4,2,2,2,2,2,2,2,2,2,2,2,2,2,2,2,4),(-0.317624209562258,-0.298289597345508,
-0.277972697831312,-0.257527888571395,-0.237763251490301,-0.218322761768441,
-0.198992662014899,-0.179486146547689,-0.159624742417884,-0.139172721329641,
-0.118765873430163,-0.0985217268535809,-0.0784385072884339,-0.0589223902968011,
-0.0395209714294252,-0.0200261862458832,0.),.UNSPECIFIED.);
#1836=B_SPLINE_CURVE_WITH_KNOTS('',3,(#66472,#66473,#66474,#66475,#66476,
#66477,#66478,#66479,#66480,#66481,#66482,#66483,#66484,#66485,#66486,#66487,
#66488,#66489,#66490,#66491,#66492,#66493,#66494),.UNSPECIFIED.,.F.,.F.,
(4,2,2,2,2,2,2,2,2,3,4),(-0.322297560764302,-0.321398021306828,-0.281085553827047,
-0.240561930877692,-0.200304325379963,-0.16008994753857,-0.120052587150318,
-0.0801539535150511,-0.0401950225836323,0.,7.70459312222638E-5),
 .UNSPECIFIED.);
#1837=B_SPLINE_CURVE_WITH_KNOTS('',3,(#66497,#66498,#66499,#66500,#66501,
#66502,#66503,#66504,#66505,#66506,#66507,#66508,#66509,#66510,#66511,#66512,
#66513,#66514,#66515,#66516,#66517,#66518,#66519,#66520,#66521,#66522,#66523,
#66524,#66525,#66526,#66527,#66528,#66529,#66530,#66531,#66532),
 .UNSPECIFIED.,.T.,.F.,(4,2,2,2,2,2,2,2,2,2,2,2,2,2,2,2,2,4),(0.,0.0399541104210288,
0.0799101633969753,0.120042188031154,0.160349494011009,0.200700062461553,
0.240669149749968,0.281146928549773,0.321688268054745,0.361827692832095,
0.401937446251242,0.441912733335269,0.482224630790471,0.523014478232509,
0.563360237939814,0.603655558781587,0.623959945531849,0.644496878445225),
 .UNSPECIFIED.);
#1838=B_SPLINE_CURVE_WITH_KNOTS('',3,(#66533,#66534,#66535,#66536,#66537,
#66538,#66539,#66540,#66541,#66542,#66543,#66544,#66545,#66546,#66547,#66548,
#66549,#66550),.UNSPECIFIED.,.F.,.F.,(4,2,2,2,2,2,2,2,4),(7.70459312222638E-5,
0.0397955677791879,0.0802687034398072,0.121068716980965,0.161667866029956,
0.201985897549818,0.242384262176046,0.282897418235116,0.322422982766503),
 .UNSPECIFIED.);
#1839=B_SPLINE_CURVE_WITH_KNOTS('',3,(#66556,#66557,#66558,#66559,#66560,
#66561,#66562,#66563,#66564,#66565,#66566,#66567,#66568,#66569,#66570,#66571,
#66572,#66573,#66574,#66575,#66576,#66577,#66578,#66579,#66580,#66581,#66582,
#66583,#66584,#66585,#66586,#66587,#66588,#66589),.UNSPECIFIED.,.T.,.F.,
(4,2,2,2,2,2,2,2,2,2,2,2,2,2,2,2,4),(-0.315594596112197,-0.297212238945519,
-0.277244382715483,-0.257516629840736,-0.237813342886634,-0.218181203303342,
-0.198609433310666,-0.179033482143113,-0.159387625583977,-0.139657909631806,
-0.119884576737678,-0.0997305737884784,-0.0797274953574875,-0.0598072340293335,
-0.0398813658942522,-0.0199326208918523,0.),.UNSPECIFIED.);
#1840=B_SPLINE_CURVE_WITH_KNOTS('',3,(#66593,#66594,#66595,#66596,#66597,
#66598,#66599,#66600,#66601,#66602,#66603,#66604,#66605,#66606,#66607,#66608,
#66609,#66610,#66611,#66612,#66613,#66614,#66615),.UNSPECIFIED.,.F.,.F.,
(4,2,2,2,2,2,2,2,2,3,4),(-0.301061346698403,-0.300154233107256,-0.262390271276384,
-0.224265876054378,-0.185595957927573,-0.147776554844827,-0.110684741630273,
-0.0740733635944757,-0.0373547309855255,0.,9.9963037913639E-5),
 .UNSPECIFIED.);
#1841=B_SPLINE_CURVE_WITH_KNOTS('',3,(#66618,#66619,#66620,#66621,#66622,
#66623,#66624,#66625,#66626,#66627,#66628,#66629,#66630,#66631,#66632,#66633,
#66634,#66635,#66636,#66637,#66638,#66639,#66640,#66641,#66642,#66643,#66644,
#66645,#66646,#66647,#66648,#66649,#66650,#66651,#66652,#66653),
 .UNSPECIFIED.,.T.,.F.,(4,2,2,2,2,2,2,2,2,2,2,2,2,2,2,2,2,4),(0.,0.0355202696277959,
0.0730229242197281,0.109881947979451,0.14733221535353,0.185244244854458,
0.223245130810672,0.259644256151418,0.294838797516899,0.330228485413916,
0.366554345829066,0.404791218309081,0.442165216607522,0.480056587438502,
0.518291371462249,0.552548743094609,0.588529668421804,0.59994995921808),
 .UNSPECIFIED.);
#1842=B_SPLINE_CURVE_WITH_KNOTS('',3,(#66654,#66655,#66656,#66657,#66658,
#66659,#66660,#66661,#66662,#66663,#66664,#66665,#66666,#66667,#66668,#66669,
#66670,#66671),.UNSPECIFIED.,.F.,.F.,(4,2,2,2,2,2,2,2,4),(9.9963037913639E-5,
0.0375956597039427,0.0765101512186815,0.114950962752918,0.152884443087743,
0.190596119807599,0.227522757249408,0.264361209646464,0.301167798081618),
 .UNSPECIFIED.);
#1843=B_SPLINE_CURVE_WITH_KNOTS('',3,(#66677,#66678,#66679,#66680,#66681,
#66682,#66683,#66684,#66685,#66686,#66687,#66688,#66689,#66690,#66691,#66692,
#66693,#66694,#66695,#66696,#66697,#66698,#66699,#66700,#66701,#66702,#66703,
#66704,#66705,#66706,#66707,#66708,#66709,#66710),.UNSPECIFIED.,.T.,.F.,
(4,2,2,2,2,2,2,2,2,2,2,2,2,2,2,2,4),(-0.317595599740568,-0.297703490970376,
-0.277509143763147,-0.257154452491718,-0.237202102860055,-0.217609159241214,
-0.198259786702619,-0.178882547663072,-0.159219940579443,-0.139111795431245,
-0.118694444304224,-0.0983996654619764,-0.0782652805385247,-0.0586175735931439,
-0.0391812471909454,-0.0197681563368876,0.),.UNSPECIFIED.);
#1844=B_SPLINE_CURVE_WITH_KNOTS('',3,(#66714,#66715,#66716,#66717,#66718,
#66719,#66720,#66721,#66722,#66723,#66724,#66725,#66726,#66727,#66728,#66729,
#66730,#66731,#66732,#66733,#66734,#66735,#66736),.UNSPECIFIED.,.F.,.F.,
(4,2,2,2,2,2,2,2,2,3,4),(-0.322354039166853,-0.321726786837625,-0.28131793661759,
-0.241002699918155,-0.200356598490939,-0.160084029752791,-0.119921696599811,
-0.0799481541673699,-0.0400452631944034,0.,7.17856074681361E-6),
 .UNSPECIFIED.);
#1845=B_SPLINE_CURVE_WITH_KNOTS('',3,(#66739,#66740,#66741,#66742,#66743,
#66744,#66745,#66746,#66747,#66748,#66749,#66750,#66751,#66752,#66753,#66754,
#66755,#66756,#66757,#66758,#66759,#66760,#66761,#66762,#66763,#66764,#66765,
#66766,#66767,#66768,#66769,#66770,#66771,#66772,#66773,#66774),
 .UNSPECIFIED.,.T.,.F.,(4,2,2,2,2,2,2,2,2,2,2,2,2,2,2,2,2,4),(0.,0.0399541104211525,
0.0799101633973132,0.120042188031252,0.160349494010639,0.200700062460746,
0.24066914974878,0.281146928548183,0.321688268052773,0.361827692829693,
0.401937446248195,0.441912733331337,0.482224630785847,0.523014478227025,
0.563360237933407,0.603655558774048,0.623959945523888,0.644496878437146),
 .UNSPECIFIED.);
#1846=B_SPLINE_CURVE_WITH_KNOTS('',3,(#66775,#66776,#66777,#66778,#66779,
#66780,#66781,#66782,#66783,#66784,#66785,#66786,#66787,#66788,#66789,#66790,
#66791,#66792),.UNSPECIFIED.,.F.,.F.,(4,2,2,2,2,2,2,2,4),(7.17856074681361E-6,
0.0390237938020301,0.0794667944515802,0.120295929995562,0.16108166723615,
0.201434585894493,0.241793385121914,0.282373009958602,0.322362267042215),
 .UNSPECIFIED.);
#1847=B_SPLINE_CURVE_WITH_KNOTS('',3,(#66798,#66799,#66800,#66801,#66802,
#66803,#66804,#66805,#66806,#66807,#66808,#66809,#66810,#66811,#66812,#66813,
#66814,#66815,#66816,#66817,#66818,#66819,#66820,#66821,#66822,#66823,#66824,
#66825,#66826,#66827,#66828,#66829,#66830,#66831),.UNSPECIFIED.,.T.,.F.,
(4,2,2,2,2,2,2,2,2,2,2,2,2,2,2,2,4),(-0.315594622373487,-0.297533870662118,
-0.277622157510714,-0.257651723875446,-0.237921713542688,-0.218237311660376,
-0.198628601130043,-0.179061340536985,-0.159464238093167,-0.139788278396831,
-0.120041716967774,-0.0998694200192435,-0.0798494940937937,-0.0599296759610903,
-0.0399990336273364,-0.0200054074132563,0.),.UNSPECIFIED.);
#1848=B_SPLINE_CURVE_WITH_KNOTS('',3,(#66835,#66836,#66837,#66838,#66839,
#66840,#66841,#66842,#66843,#66844,#66845,#66846,#66847,#66848,#66849,#66850,
#66851,#66852,#66853,#66854),.UNSPECIFIED.,.F.,.F.,(4,2,2,2,2,2,2,2,2,4),
(-0.301147961624379,-0.300062316631199,-0.262394637047186,-0.224420968944876,
-0.185887448097902,-0.1477829056142,-0.110335991047362,-0.0735563535339244,
-0.036984133703636,-4.35690811094724E-5),.UNSPECIFIED.);
#1849=B_SPLINE_CURVE_WITH_KNOTS('',3,(#66857,#66858,#66859,#66860,#66861,
#66862,#66863,#66864,#66865,#66866,#66867,#66868,#66869,#66870,#66871,#66872,
#66873,#66874,#66875,#66876,#66877,#66878,#66879,#66880,#66881,#66882,#66883,
#66884,#66885,#66886,#66887,#66888,#66889,#66890,#66891,#66892),
 .UNSPECIFIED.,.T.,.F.,(4,2,2,2,2,2,2,2,2,2,2,2,2,2,2,2,2,4),(0.,0.0355202696275203,
0.0730229242186996,0.109881947977571,0.147332215350384,0.185244244849724,
0.223245130804017,0.259644256142594,0.294838797505521,0.330228485399748,
0.366554345812062,0.40479121828863,0.442165216583351,0.48005658741036,0.518291371429938,
0.552548743058257,0.588529668380768,0.599949959176512),.UNSPECIFIED.);
#1850=B_SPLINE_CURVE_WITH_KNOTS('',3,(#66893,#66894,#66895,#66896,#66897,
#66898,#66899,#66900,#66901,#66902,#66903,#66904,#66905,#66906,#66907,#66908,
#66909,#66910,#66911,#66912,#66913),.UNSPECIFIED.,.F.,.F.,(4,3,2,2,2,2,
2,2,2,4),(-4.35690811094724E-5,0.,0.0365327773178391,0.0750112777319575,
0.113889864865708,0.152210652521084,0.190038882754267,0.227668024742707,
0.264502667827508,0.301030361353156),.UNSPECIFIED.);
#1851=B_SPLINE_CURVE_WITH_KNOTS('',3,(#66919,#66920,#66921,#66922,#66923,
#66924,#66925,#66926,#66927,#66928,#66929,#66930,#66931,#66932,#66933,#66934,
#66935,#66936,#66937,#66938,#66939,#66940,#66941,#66942,#66943,#66944,#66945,
#66946,#66947,#66948,#66949,#66950,#66951,#66952),.UNSPECIFIED.,.T.,.F.,
(4,2,2,2,2,2,2,2,2,2,2,2,2,2,2,2,4),(-0.31757151244209,-0.298332728669395,
-0.27818234576115,-0.2578362591579,-0.23736096878236,-0.217588804779534,
-0.198148148450172,-0.178828387511107,-0.159338797938639,-0.139491768304976,
-0.119229310805976,-0.098777940027667,-0.078489708879422,-0.0583916924149346,
-0.0388763803889898,-0.0194825025044759,0.),.UNSPECIFIED.);
#1852=B_SPLINE_CURVE_WITH_KNOTS('',3,(#66956,#66957,#66958,#66959,#66960,
#66961,#66962,#66963,#66964,#66965,#66966,#66967,#66968,#66969,#66970,#66971,
#66972,#66973,#66974,#66975),.UNSPECIFIED.,.F.,.F.,(4,2,2,2,2,2,2,2,2,4),
(-0.322405728416197,-0.321546706061062,-0.281198364753022,-0.2408951979842,
-0.200323869063384,-0.160069256043837,-0.119861454351153,-0.0798327506359469,
-0.0399463257727349,-5.45498490094123E-5),.UNSPECIFIED.);
#1853=B_SPLINE_CURVE_WITH_KNOTS('',3,(#66978,#66979,#66980,#66981,#66982,
#66983,#66984,#66985,#66986,#66987,#66988,#66989,#66990,#66991,#66992,#66993,
#66994,#66995,#66996,#66997,#66998,#66999,#67000,#67001,#67002,#67003,#67004,
#67005,#67006,#67007,#67008,#67009,#67010,#67011,#67012,#67013),
 .UNSPECIFIED.,.T.,.F.,(4,2,2,2,2,2,2,2,2,2,2,2,2,2,2,2,2,4),(0.,0.0399541104209913,
0.0799101633967558,0.120042188030517,0.1603494940098,0.200700062459717,
0.240669149747544,0.281146928546853,0.321688268051145,0.361827692827755,
0.401937446246095,0.4419127333289,0.482224630783017,0.523014478224009,0.563360237930216,
0.603655558770796,0.623959945520647,0.644496878433936),.UNSPECIFIED.);
#1854=B_SPLINE_CURVE_WITH_KNOTS('',3,(#67014,#67015,#67016,#67017,#67018,
#67019,#67020,#67021,#67022,#67023,#67024,#67025,#67026,#67027,#67028,#67029,
#67030,#67031,#67032,#67033,#67034),.UNSPECIFIED.,.F.,.F.,(4,3,2,2,2,2,
2,2,2,4),(-5.45498490094123E-5,0.,0.0396635395521475,0.080088963912866,
0.12057975818371,0.161389406329886,0.202107242285931,0.242444716121441,
0.282765523937027,0.322306952019563),.UNSPECIFIED.);
#1855=B_SPLINE_CURVE_WITH_KNOTS('',3,(#67040,#67041,#67042,#67043,#67044,
#67045,#67046,#67047,#67048,#67049,#67050,#67051,#67052,#67053,#67054,#67055,
#67056,#67057,#67058,#67059,#67060,#67061,#67062,#67063,#67064,#67065,#67066,
#67067,#67068,#67069,#67070,#67071,#67072,#67073),.UNSPECIFIED.,.T.,.F.,
(4,2,2,2,2,2,2,2,2,2,2,2,2,2,2,2,4),(-0.315593063776311,-0.29700803323264,
-0.277101906790985,-0.25710555612465,-0.237377416904486,-0.217678261420823,
-0.198052738861469,-0.178487401632928,-0.158914692523433,-0.139266634878621,
-0.119529894293757,-0.0997490751108272,-0.0797713096896962,-0.05971623206454,
-0.0397855249884807,-0.0198939142348958,0.),.UNSPECIFIED.);
#1856=B_SPLINE_CURVE_WITH_KNOTS('',3,(#67077,#67078,#67079,#67080,#67081,
#67082,#67083,#67084,#67085,#67086,#67087,#67088,#67089,#67090,#67091,#67092,
#67093,#67094,#67095,#67096),.UNSPECIFIED.,.F.,.F.,(4,2,2,2,2,2,2,2,2,4),
(-0.301118946487766,-0.300527485838102,-0.262862138850157,-0.22510653196151,
-0.186960746251741,-0.148254876835345,-0.110408214249886,-0.0732924492929095,
-0.0366839954349046,-4.93896356226975E-5),.UNSPECIFIED.);
#1857=B_SPLINE_CURVE_WITH_KNOTS('',3,(#67099,#67100,#67101,#67102,#67103,
#67104,#67105,#67106,#67107,#67108,#67109,#67110,#67111,#67112,#67113,#67114,
#67115,#67116,#67117,#67118,#67119,#67120,#67121,#67122,#67123,#67124,#67125,
#67126,#67127,#67128,#67129,#67130,#67131,#67132,#67133,#67134),
 .UNSPECIFIED.,.T.,.F.,(4,2,2,2,2,2,2,2,2,2,2,2,2,2,2,2,2,4),(0.,0.0355202696277843,
0.0730229242196146,0.10988194797903,0.147332215352703,0.185244244852949,
0.223245130808307,0.25964425614813,0.294838797512346,0.330228485408035,
0.366554345822135,0.404791218300662,0.442165216597325,0.480056587426433,
0.51829137144813,0.552548743078511,0.588529668403261,0.599949959199294),
 .UNSPECIFIED.);
#1858=B_SPLINE_CURVE_WITH_KNOTS('',3,(#67135,#67136,#67137,#67138,#67139,
#67140,#67141,#67142,#67143,#67144,#67145,#67146,#67147,#67148,#67149,#67150,
#67151,#67152,#67153,#67154,#67155),.UNSPECIFIED.,.F.,.F.,(4,3,2,2,2,2,
2,2,2,4),(-4.93896356226975E-5,0.,0.0365695267012744,0.074616322225757,
0.113601961148227,0.152149562549399,0.190151155062694,0.227853759249584,
0.264779511262172,0.301013530103241),.UNSPECIFIED.);
#1859=B_SPLINE_CURVE_WITH_KNOTS('',3,(#67161,#67162,#67163,#67164,#67165,
#67166,#67167,#67168,#67169,#67170,#67171,#67172,#67173,#67174,#67175,#67176,
#67177,#67178,#67179,#67180,#67181,#67182,#67183,#67184,#67185,#67186,#67187,
#67188,#67189,#67190,#67191,#67192,#67193,#67194),.UNSPECIFIED.,.T.,.F.,
(4,2,2,2,2,2,2,2,2,2,2,2,2,2,2,2,4),(-0.317551766644571,-0.298486525081855,
-0.278428882026584,-0.258221088221274,-0.237842005071232,-0.217867604593861,
-0.198254586659461,-0.178902478996899,-0.159544153524827,-0.139911897737489,
-0.119838709236774,-0.0993894180525655,-0.0790440450201523,-0.0588750365855975,
-0.0388400330894688,-0.0194039455565196,0.),.UNSPECIFIED.);
#1860=B_SPLINE_CURVE_WITH_KNOTS('',3,(#67198,#67199,#67200,#67201,#67202,
#67203,#67204,#67205,#67206,#67207,#67208,#67209,#67210,#67211,#67212,#67213,
#67214,#67215,#67216,#67217),.UNSPECIFIED.,.F.,.F.,(4,2,2,2,2,2,2,2,2,4),
(-0.322355554522363,-0.322178904200381,-0.281704619582365,-0.241356636912598,
-0.201005058459337,-0.16025826339261,-0.119996742027504,-0.0798488072456165,
-0.0398898126128195,-2.20474994749807E-6),.UNSPECIFIED.);
#1861=B_SPLINE_CURVE_WITH_KNOTS('',3,(#67220,#67221,#67222,#67223,#67224,
#67225,#67226,#67227,#67228,#67229,#67230,#67231,#67232,#67233,#67234,#67235,
#67236,#67237,#67238,#67239,#67240,#67241,#67242,#67243,#67244,#67245,#67246,
#67247,#67248,#67249,#67250,#67251,#67252,#67253,#67254,#67255),
 .UNSPECIFIED.,.T.,.F.,(4,2,2,2,2,2,2,2,2,2,2,2,2,2,2,2,2,4),(0.,0.0399541104211012,
0.0799101633971579,0.120042188031192,0.160349494010781,0.200700062461153,
0.240669149749436,0.281146928549182,0.321688268054342,0.361827692831924,
0.401937446250896,0.441912733334278,0.482224630789236,0.523014478230996,
0.563360237938004,0.603655558779501,0.623959945529625,0.644496878442948),
 .UNSPECIFIED.);
#1862=B_SPLINE_CURVE_WITH_KNOTS('',3,(#67256,#67257,#67258,#67259,#67260,
#67261,#67262,#67263,#67264,#67265,#67266,#67267,#67268,#67269,#67270,#67271,
#67272,#67273,#67274,#67275,#67276),.UNSPECIFIED.,.F.,.F.,(4,3,2,2,2,2,
2,2,2,4),(-2.20474994749807E-6,0.,0.0391360015106571,0.0794317419925186,
0.119897010292482,0.160355079753466,0.201332782499759,0.241783415181495,
0.282097330185288,0.32235683326756),.UNSPECIFIED.);
#1863=B_SPLINE_CURVE_WITH_KNOTS('',3,(#67282,#67283,#67284,#67285,#67286,
#67287,#67288,#67289,#67290,#67291,#67292,#67293,#67294,#67295,#67296,#67297,
#67298,#67299,#67300,#67301,#67302,#67303,#67304,#67305,#67306,#67307,#67308,
#67309,#67310,#67311,#67312,#67313,#67314,#67315),.UNSPECIFIED.,.T.,.F.,
(4,2,2,2,2,2,2,2,2,2,2,2,2,2,2,2,4),(-0.315592915588056,-0.297157230115009,
-0.277242481766554,-0.257314550571046,-0.237282993015635,-0.217557856490286,
-0.197884126696601,-0.178286261599438,-0.158724647806166,-0.139124925349899,
-0.119439049162832,-0.0996807653366323,-0.0799033227642352,-0.0598016412664598,
-0.0398382198951536,-0.0199265333829655,0.),.UNSPECIFIED.);
#1864=B_SPLINE_CURVE_WITH_KNOTS('',3,(#67319,#67320,#67321,#67322,#67323,
#67324,#67325,#67326,#67327,#67328,#67329,#67330,#67331,#67332,#67333,#67334,
#67335,#67336,#67337,#67338),.UNSPECIFIED.,.F.,.F.,(4,2,2,2,2,2,2,2,2,4),
(-0.301058381607661,-0.300695934659419,-0.263083586410712,-0.225429745929767,
-0.187495787142987,-0.149014527999422,-0.110874845528449,-0.0733724375687369,
-0.0365583584387441,-2.17004182293026E-6),.UNSPECIFIED.);
#1865=B_SPLINE_CURVE_WITH_KNOTS('',3,(#67341,#67342,#67343,#67344,#67345,
#67346,#67347,#67348,#67349,#67350,#67351,#67352,#67353,#67354,#67355,#67356,
#67357,#67358,#67359,#67360,#67361,#67362,#67363,#67364,#67365,#67366,#67367,
#67368,#67369,#67370,#67371,#67372,#67373,#67374,#67375,#67376),
 .UNSPECIFIED.,.T.,.F.,(4,2,2,2,2,2,2,2,2,2,2,2,2,2,2,2,2,4),(0.,0.0355202696277563,
0.0730229242195573,0.109881947979313,0.147332215353586,0.185244244854587,
0.223245130811004,0.259644256151833,0.294838797517268,0.330228485414355,
0.366554345829942,0.404791218310431,0.442165216609281,0.480056587440684,
0.518291371464912,0.552548743097934,0.588529668425773,0.599949959222132),
 .UNSPECIFIED.);
#1866=B_SPLINE_CURVE_WITH_KNOTS('',3,(#67377,#67378,#67379,#67380,#67381,
#67382,#67383,#67384,#67385,#67386,#67387,#67388,#67389,#67390,#67391,#67392,
#67393,#67394,#67395,#67396,#67397),.UNSPECIFIED.,.F.,.F.,(4,3,2,2,2,2,
2,2,2,4),(-2.17004182293026E-6,0.,0.0357498274067009,0.0734077363203498,
0.111837190993789,0.150741885695325,0.189101783842794,0.226953230384565,
0.264585676093243,0.301058061735977),.UNSPECIFIED.);
#1867=B_SPLINE_CURVE_WITH_KNOTS('',3,(#67403,#67404,#67405,#67406,#67407,
#67408,#67409,#67410,#67411,#67412,#67413,#67414,#67415,#67416,#67417,#67418,
#67419,#67420,#67421,#67422,#67423,#67424,#67425,#67426,#67427,#67428,#67429,
#67430,#67431,#67432,#67433,#67434,#67435,#67436),.UNSPECIFIED.,.T.,.F.,
(4,2,2,2,2,2,2,2,2,2,2,2,2,2,2,2,4),(-0.31754433338207,-0.298803281332166,
-0.278807800538721,-0.258673081016315,-0.238343826302372,-0.217876028762562,
-0.19807748660554,-0.178620027297595,-0.159304922169407,-0.139840169793005,
-0.120023736794459,-0.0997855989498413,-0.0793300681815676,-0.0590301788462695,
-0.0389218783466252,-0.0193925721148871,0.),.UNSPECIFIED.);
#1868=B_SPLINE_CURVE_WITH_KNOTS('',3,(#67440,#67441,#67442,#67443,#67444,
#67445,#67446,#67447,#67448,#67449,#67450,#67451,#67452,#67453,#67454,#67455,
#67456,#67457,#67458,#67459),.UNSPECIFIED.,.F.,.F.,(4,2,2,2,2,2,2,2,2,4),
(-0.322354756361963,-0.322205918870643,-0.281689949818391,-0.241237699113221,
-0.20092186741425,-0.160456629709274,-0.120204465960691,-0.0799716249211841,
-0.039906809364872,-5.39397368838195E-6),.UNSPECIFIED.);
#1869=B_SPLINE_CURVE_WITH_KNOTS('',3,(#67462,#67463,#67464,#67465,#67466,
#67467,#67468,#67469,#67470,#67471,#67472,#67473,#67474,#67475,#67476,#67477,
#67478,#67479,#67480,#67481,#67482,#67483,#67484,#67485,#67486,#67487,#67488,
#67489,#67490,#67491,#67492,#67493,#67494,#67495,#67496,#67497),
 .UNSPECIFIED.,.T.,.F.,(4,2,2,2,2,2,2,2,2,2,2,2,2,2,2,2,2,4),(0.,0.0399541104210428,
0.0799101633969861,0.120042188031056,0.160349494010698,0.200700062460998,
0.240669149749349,0.281146928549081,0.321688268054021,0.361827692831356,
0.401937446250295,0.44191273333395,0.482224630789036,0.52301447823097,0.563360237938078,
0.603655558779622,0.623959945529193,0.644496878442225),.UNSPECIFIED.);
#1870=B_SPLINE_CURVE_WITH_KNOTS('',3,(#67498,#67499,#67500,#67501,#67502,
#67503,#67504,#67505,#67506,#67507,#67508,#67509,#67510,#67511,#67512,#67513,
#67514,#67515,#67516,#67517,#67518),.UNSPECIFIED.,.F.,.F.,(4,3,2,2,2,2,
2,2,2,4),(-5.39397368838195E-6,0.,0.0393075887039707,0.0794597964783887,
0.119850067157852,0.160325694985967,0.201138041009554,0.241798684361789,
0.282127159463835,0.322359660598591),.UNSPECIFIED.);
#1871=B_SPLINE_CURVE_WITH_KNOTS('',3,(#67524,#67525,#67526,#67527,#67528,
#67529,#67530,#67531,#67532,#67533,#67534,#67535,#67536,#67537,#67538,#67539,
#67540,#67541,#67542,#67543,#67544,#67545,#67546,#67547,#67548,#67549,#67550,
#67551,#67552,#67553,#67554,#67555,#67556,#67557),.UNSPECIFIED.,.T.,.F.,
(4,2,2,2,2,2,2,2,2,2,2,2,2,2,2,2,4),(-0.315593410768126,-0.29754747075378,
-0.277605746518463,-0.257690189723362,-0.237736453581343,-0.217652321280653,
-0.197942437206122,-0.178301549934773,-0.15872624759116,-0.139155513391519,
-0.119520099622689,-0.099798701851234,-0.080027130270589,-0.0598618542633545,
-0.0398484241333443,-0.0199251752696053,0.),.UNSPECIFIED.);
#1872=B_SPLINE_CURVE_WITH_KNOTS('',3,(#67561,#67562,#67563,#67564,#67565,
#67566,#67567,#67568,#67569,#67570,#67571,#67572,#67573,#67574,#67575,#67576,
#67577,#67578,#67579,#67580,#67581),.UNSPECIFIED.,.F.,.F.,(4,2,2,2,2,2,
2,2,3,4),(-0.300978142018712,-0.263914525329246,-0.226284750703183,-0.188545296544232,
-0.150403990415101,-0.111688584966917,-0.0737943243144371,-0.0366264406025384,
0.,8.00110665434538E-5),.UNSPECIFIED.);
#1873=B_SPLINE_CURVE_WITH_KNOTS('',3,(#67584,#67585,#67586,#67587,#67588,
#67589,#67590,#67591,#67592,#67593,#67594,#67595,#67596,#67597,#67598,#67599,
#67600,#67601,#67602,#67603,#67604,#67605,#67606,#67607,#67608,#67609,#67610,
#67611,#67612,#67613,#67614,#67615,#67616,#67617,#67618,#67619),
 .UNSPECIFIED.,.T.,.F.,(4,2,2,2,2,2,2,2,2,2,2,2,2,2,2,2,2,4),(0.,0.0355202696274643,
0.0730229242183205,0.109881947976405,0.147332215348248,0.185244244846206,
0.223245130798705,0.259644256135453,0.294838797496282,0.330228485388232,
0.366554345798093,0.404791218271537,0.442165216563109,0.480056587386566,
0.518291371402324,0.55254874302685,0.58852966834476,0.599949959139978),
 .UNSPECIFIED.);
#1874=B_SPLINE_CURVE_WITH_KNOTS('',3,(#67620,#67621,#67622,#67623,#67624,
#67625,#67626,#67627,#67628,#67629,#67630,#67631,#67632,#67633,#67634,#67635,
#67636,#67637,#67638,#67639),.UNSPECIFIED.,.F.,.F.,(4,2,2,2,2,2,2,2,2,4),
(8.00110665434538E-5,0.0353108547782378,0.0725312692972248,0.110518938547593,
0.149564323404323,0.188222355253345,0.226307975094044,0.264023560479495,
0.300970351665515,0.301144794938351),.UNSPECIFIED.);
#1875=B_SPLINE_CURVE_WITH_KNOTS('',3,(#67645,#67646,#67647,#67648,#67649,
#67650,#67651,#67652,#67653,#67654,#67655,#67656,#67657,#67658,#67659,#67660,
#67661,#67662,#67663,#67664,#67665,#67666,#67667,#67668,#67669,#67670,#67671,
#67672,#67673,#67674,#67675,#67676,#67677,#67678),.UNSPECIFIED.,.T.,.F.,
(4,2,2,2,2,2,2,2,2,2,2,2,2,2,2,2,4),(-0.31754678186458,-0.298854543535332,
-0.279132590217806,-0.25908366028776,-0.238869461524636,-0.218473096805952,
-0.198477657185613,-0.17884202633409,-0.159481005232111,-0.140133917139174,
-0.120526215304075,-0.100546056505587,-0.0800747095050212,-0.0596878946432227,
-0.0394856419211679,-0.019444442213569,0.),.UNSPECIFIED.);
#1876=B_SPLINE_CURVE_WITH_KNOTS('',3,(#67682,#67683,#67684,#67685,#67686,
#67687,#67688,#67689,#67690,#67691,#67692,#67693,#67694,#67695,#67696,#67697,
#67698,#67699),.UNSPECIFIED.,.F.,.F.,(4,2,2,2,2,2,2,2,4),(-0.322410599568958,
-0.282381736564621,-0.241782820187053,-0.201359211265473,-0.161045994561305,
-0.120443581321846,-0.0801730862382622,-0.0399924380800003,-6.45926737957721E-5),
 .UNSPECIFIED.);
#1877=B_SPLINE_CURVE_WITH_KNOTS('',3,(#67702,#67703,#67704,#67705,#67706,
#67707,#67708,#67709,#67710,#67711,#67712,#67713,#67714,#67715,#67716,#67717,
#67718,#67719,#67720,#67721,#67722,#67723,#67724,#67725,#67726,#67727,#67728,
#67729,#67730,#67731,#67732,#67733,#67734,#67735,#67736,#67737),
 .UNSPECIFIED.,.T.,.F.,(4,2,2,2,2,2,2,2,2,2,2,2,2,2,2,2,2,4),(0.,0.0399541104209861,
0.0799101633967313,0.120042188030496,0.160349494009841,0.200700062459914,
0.240669149747714,0.281146928546904,0.321688268051343,0.361827692828311,
0.401937446247057,0.441912733330249,0.482224630784895,0.523014478226398,
0.563360237933181,0.603655558774504,0.623959945523992,0.644496878437005),
 .UNSPECIFIED.);
#1878=B_SPLINE_CURVE_WITH_KNOTS('',3,(#67738,#67739,#67740,#67741,#67742,
#67743,#67744,#67745,#67746,#67747,#67748,#67749,#67750,#67751,#67752,#67753,
#67754,#67755,#67756,#67757,#67758,#67759,#67760),.UNSPECIFIED.,.F.,.F.,
(4,3,2,2,2,2,2,2,2,2,4),(-6.45926737957721E-5,0.,0.0390108812553356,0.0790243539467953,
0.119283184671902,0.159719989985786,0.200170808743092,0.241073441282928,
0.281478872292121,0.321809987466221,0.322307943731577),.UNSPECIFIED.);
#1879=B_SPLINE_CURVE_WITH_KNOTS('',3,(#67766,#67767,#67768,#67769,#67770,
#67771,#67772,#67773,#67774,#67775,#67776,#67777,#67778,#67779,#67780,#67781,
#67782,#67783,#67784,#67785,#67786,#67787,#67788,#67789,#67790,#67791,#67792,
#67793,#67794,#67795,#67796,#67797,#67798,#67799),.UNSPECIFIED.,.T.,.F.,
(4,2,2,2,2,2,2,2,2,2,2,2,2,2,2,2,4),(-0.31559325345182,-0.297317730854205,
-0.277323673584106,-0.257372580958333,-0.237457900008399,-0.217484430544864,
-0.197755119221471,-0.178067553902672,-0.158455097163848,-0.138887603657002,
-0.119294455824915,-0.0996233242918477,-0.0798789996652367,-0.0599063556623395,
-0.0398565846628778,-0.0199228180997341,0.),.UNSPECIFIED.);
#1880=B_SPLINE_CURVE_WITH_KNOTS('',3,(#67803,#67804,#67805,#67806,#67807,
#67808,#67809,#67810,#67811,#67812,#67813,#67814,#67815,#67816,#67817,#67818,
#67819,#67820,#67821,#67822,#67823,#67824,#67825),.UNSPECIFIED.,.F.,.F.,
(4,2,2,2,2,2,2,2,2,3,4),(-0.301050544014646,-0.300701045912431,-0.263849573346669,
-0.226560847894422,-0.188894701836328,-0.151018078542583,-0.112639483085741,
-0.0744561853366415,-0.0368753905065712,0.,7.74278383810611E-6),
 .UNSPECIFIED.);
#1881=B_SPLINE_CURVE_WITH_KNOTS('',3,(#67828,#67829,#67830,#67831,#67832,
#67833,#67834,#67835,#67836,#67837,#67838,#67839,#67840,#67841,#67842,#67843,
#67844,#67845,#67846,#67847,#67848,#67849,#67850,#67851,#67852,#67853,#67854,
#67855,#67856,#67857,#67858,#67859,#67860,#67861,#67862,#67863),
 .UNSPECIFIED.,.T.,.F.,(4,2,2,2,2,2,2,2,2,2,2,2,2,2,2,2,2,4),(0.,0.0355202696275411,
0.0730229242188105,0.10988194797803,0.147332215351439,0.185244244851336,
0.223245130806424,0.259644256145998,0.294838797510073,0.330228485405602,
0.366554345819332,0.404791218297467,0.442165216593924,0.480056587422867,
0.518291371444443,0.552548743074661,0.588529668399372,0.599949959195358),
 .UNSPECIFIED.);
#1882=B_SPLINE_CURVE_WITH_KNOTS('',3,(#67864,#67865,#67866,#67867,#67868,
#67869,#67870,#67871,#67872,#67873,#67874,#67875,#67876,#67877,#67878,#67879,
#67880,#67881),.UNSPECIFIED.,.F.,.F.,(4,2,2,2,2,2,2,2,4),(7.74278383810611E-6,
0.0358556004554429,0.0727165890303891,0.110307479935514,0.148690120729207,
0.187575552003323,0.225931327919466,0.263793633053924,0.301107698759479),
 .UNSPECIFIED.);
#1883=B_SPLINE_CURVE_WITH_KNOTS('',3,(#67887,#67888,#67889,#67890,#67891,
#67892,#67893,#67894,#67895,#67896,#67897,#67898,#67899,#67900,#67901,#67902,
#67903,#67904,#67905,#67906,#67907,#67908,#67909,#67910,#67911,#67912,#67913,
#67914,#67915,#67916,#67917,#67918,#67919,#67920),.UNSPECIFIED.,.T.,.F.,
(4,2,2,2,2,2,2,2,2,2,2,2,2,2,2,2,4),(-0.317562554188654,-0.298753170810319,
-0.279306735529762,-0.259305046894606,-0.239193146172324,-0.21890439655601,
-0.198468405269086,-0.178635579958314,-0.159150751579314,-0.139831347137531,
-0.120387634799293,-0.100604124620228,-0.0803902771831579,-0.0599545013953302,
-0.0396660633012328,-0.0195543258745943,0.),.UNSPECIFIED.);
#1884=B_SPLINE_CURVE_WITH_KNOTS('',3,(#67924,#67925,#67926,#67927,#67928,
#67929,#67930,#67931,#67932,#67933,#67934,#67935,#67936,#67937,#67938,#67939,
#67940,#67941),.UNSPECIFIED.,.F.,.F.,(4,2,2,2,2,2,2,2,4),(-0.322408809219383,
-0.282264936011648,-0.241770195002564,-0.201321774169933,-0.161005070722384,
-0.120554276389559,-0.0803107265542591,-0.0400757886480797,-8.3535166333862E-5),
 .UNSPECIFIED.);
#1885=B_SPLINE_CURVE_WITH_KNOTS('',3,(#67944,#67945,#67946,#67947,#67948,
#67949,#67950,#67951,#67952,#67953,#67954,#67955,#67956,#67957,#67958,#67959,
#67960,#67961,#67962,#67963,#67964,#67965,#67966,#67967,#67968,#67969,#67970,
#67971,#67972,#67973,#67974,#67975,#67976,#67977,#67978,#67979),
 .UNSPECIFIED.,.T.,.F.,(4,2,2,2,2,2,2,2,2,2,2,2,2,2,2,2,2,4),(0.,0.0399541104210371,
0.0799101633969276,0.120042188030811,0.160349494010247,0.200700062460135,
0.240669149748269,0.281146928547783,0.321688268052386,0.361827692829341,
0.401937446247806,0.441912733330861,0.48222463078534,0.5230144782264,0.563360237932858,
0.603655558773727,0.623959945523498,0.644496878436718),.UNSPECIFIED.);
#1886=B_SPLINE_CURVE_WITH_KNOTS('',3,(#67980,#67981,#67982,#67983,#67984,
#67985,#67986,#67987,#67988,#67989,#67990,#67991,#67992,#67993,#67994,#67995,
#67996,#67997,#67998,#67999,#68000,#68001,#68002),.UNSPECIFIED.,.F.,.F.,
(4,3,2,2,2,2,2,2,2,2,4),(-8.3535166333862E-5,0.,0.0393019758222067,0.0792300811977625,
0.119369024266062,0.159749636133907,0.200224937322439,0.241039083207198,
0.281753542603645,0.322095726126061,0.322313417546895),.UNSPECIFIED.);
#1887=B_SPLINE_CURVE_WITH_KNOTS('',3,(#68008,#68009,#68010,#68011,#68012,
#68013,#68014,#68015,#68016,#68017,#68018,#68019,#68020,#68021,#68022,#68023,
#68024,#68025,#68026,#68027,#68028,#68029,#68030,#68031,#68032,#68033,#68034,
#68035,#68036,#68037,#68038,#68039,#68040,#68041),.UNSPECIFIED.,.T.,.F.,
(4,2,2,2,2,2,2,2,2,2,2,2,2,2,2,2,4),(-0.315593216159719,-0.297386462000642,
-0.277445073116452,-0.257509675245072,-0.23759598204093,-0.217641702014589,
-0.197556079016382,-0.177846611841745,-0.158203876776851,-0.138626450407983,
-0.119055296324289,-0.0994213253944243,-0.0797018271356818,-0.0599314841789836,
-0.0399559588412318,-0.0199275817504349,0.),.UNSPECIFIED.);
#1888=B_SPLINE_CURVE_WITH_KNOTS('',3,(#68045,#68046,#68047,#68048,#68049,
#68050,#68051,#68052,#68053,#68054,#68055,#68056,#68057,#68058,#68059,#68060,
#68061,#68062),.UNSPECIFIED.,.F.,.F.,(4,2,2,2,2,2,2,2,4),(-0.301100921471536,
-0.264139472742094,-0.227310847047349,-0.18966289503287,-0.151936985647909,
-0.113847516176928,-0.0751904625710873,-0.0372387069697444,-4.04142026933364E-5),
 .UNSPECIFIED.);
#1889=B_SPLINE_CURVE_WITH_KNOTS('',3,(#68065,#68066,#68067,#68068,#68069,
#68070,#68071,#68072,#68073,#68074,#68075,#68076,#68077,#68078,#68079,#68080,
#68081,#68082,#68083,#68084,#68085,#68086,#68087,#68088,#68089,#68090,#68091,
#68092,#68093,#68094,#68095,#68096,#68097,#68098,#68099,#68100),
 .UNSPECIFIED.,.T.,.F.,(4,2,2,2,2,2,2,2,2,2,2,2,2,2,2,2,2,4),(0.,0.0355202696276432,
0.0730229242191987,0.10988194797855,0.14733221535206,0.185244244852172,
0.223245130807611,0.259644256147649,0.294838797512173,0.330228485408115,
0.366554345822225,0.404791218300779,0.442165216597644,0.48005658742687,
0.518291371448558,0.552548743079322,0.588529668404772,0.59994995920088),
 .UNSPECIFIED.);
#1890=B_SPLINE_CURVE_WITH_KNOTS('',3,(#68101,#68102,#68103,#68104,#68105,
#68106,#68107,#68108,#68109,#68110,#68111,#68112,#68113,#68114,#68115,#68116,
#68117,#68118,#68119,#68120,#68121,#68122,#68123),.UNSPECIFIED.,.F.,.F.,
(4,3,2,2,2,2,2,2,2,2,4),(-4.04142026933364E-5,0.,0.03615915200202,0.0727912610659081,
0.109971042269411,0.147916803776992,0.186554927423317,0.225238144277993,
0.263352588611955,0.301088646814997,0.301107134483528),.UNSPECIFIED.);
#1891=B_SPLINE_CURVE_WITH_KNOTS('',3,(#68129,#68130,#68131,#68132,#68133,
#68134,#68135,#68136,#68137,#68138,#68139,#68140,#68141,#68142,#68143,#68144,
#68145,#68146,#68147,#68148,#68149,#68150,#68151,#68152,#68153,#68154,#68155,
#68156,#68157,#68158,#68159,#68160,#68161,#68162),.UNSPECIFIED.,.T.,.F.,
(4,2,2,2,2,2,2,2,2,2,2,2,2,2,2,2,4),(-0.317584181788589,-0.298794557913286,
-0.279396413811771,-0.259685398425666,-0.239643320269254,-0.219448537685349,
-0.199071862622537,-0.179049482147542,-0.159380904563574,-0.140000463388759,
-0.120658150946535,-0.101075283083877,-0.0811229435079882,-0.0606564184644852,
-0.0402655107884883,-0.0200531994927753,0.),.UNSPECIFIED.);
#1892=B_SPLINE_CURVE_WITH_KNOTS('',3,(#68166,#68167,#68168,#68169,#68170,
#68171,#68172,#68173,#68174,#68175,#68176,#68177,#68178,#68179,#68180,#68181,
#68182,#68183),.UNSPECIFIED.,.F.,.F.,(4,2,2,2,2,2,2,2,4),(-0.322367453094563,
-0.282589671050591,-0.242222087757724,-0.201802504566437,-0.161472574115384,
-0.121132041451418,-0.0804114872777562,-0.0401588574067352,-6.49995567824529E-5),
 .UNSPECIFIED.);
#1893=B_SPLINE_CURVE_WITH_KNOTS('',3,(#68186,#68187,#68188,#68189,#68190,
#68191,#68192,#68193,#68194,#68195,#68196,#68197,#68198,#68199,#68200,#68201,
#68202,#68203,#68204,#68205,#68206,#68207,#68208,#68209,#68210,#68211,#68212,
#68213,#68214,#68215,#68216,#68217,#68218,#68219,#68220,#68221),
 .UNSPECIFIED.,.T.,.F.,(4,2,2,2,2,2,2,2,2,2,2,2,2,2,2,2,2,4),(0.,0.0399541104210577,
0.0799101633970396,0.120042188031162,0.160349494011025,0.200700062461786,
0.240669149750123,0.281146928549829,0.321688268054903,0.361827692832479,
0.401937446251727,0.441912733335557,0.482224630790908,0.523014478233397,
0.563360237941084,0.603655558783352,0.623959945533176,0.644496878446289),
 .UNSPECIFIED.);
#1894=B_SPLINE_CURVE_WITH_KNOTS('',3,(#68222,#68223,#68224,#68225,#68226,
#68227,#68228,#68229,#68230,#68231,#68232,#68233,#68234,#68235,#68236,#68237,
#68238,#68239,#68240,#68241,#68242,#68243,#68244),.UNSPECIFIED.,.F.,.F.,
(4,3,2,2,2,2,2,2,2,2,4),(-6.49995567824529E-5,0.,0.0390494216426324,0.0789385757792174,
0.118952328471186,0.159225359712887,0.199685658614001,0.240152451429887,
0.281286390433688,0.321830207846101,0.322355904221303),.UNSPECIFIED.);
#1895=B_SPLINE_CURVE_WITH_KNOTS('',3,(#68250,#68251,#68252,#68253,#68254,
#68255,#68256,#68257,#68258,#68259,#68260,#68261,#68262,#68263,#68264,#68265,
#68266,#68267,#68268,#68269,#68270,#68271,#68272,#68273,#68274,#68275,#68276,
#68277,#68278,#68279,#68280,#68281,#68282,#68283),.UNSPECIFIED.,.T.,.F.,
(4,2,2,2,2,2,2,2,2,2,2,2,2,2,2,2,4),(-0.315592124455107,-0.297184981883786,
-0.277286589738207,-0.257382966676634,-0.237485648421939,-0.217559378959289,
-0.19751848279024,-0.177796769809496,-0.158121997499943,-0.138520769293498,
-0.118957847887096,-0.0993605170780253,-0.0796782175625232,-0.0599216742760547,
-0.0401442832093851,-0.0199940413345806,0.),.UNSPECIFIED.);
#1896=B_SPLINE_CURVE_WITH_KNOTS('',3,(#68287,#68288,#68289,#68290,#68291,
#68292,#68293,#68294,#68295,#68296,#68297,#68298,#68299,#68300,#68301,#68302,
#68303,#68304),.UNSPECIFIED.,.F.,.F.,(4,2,2,2,2,2,2,2,4),(-0.301134002178748,
-0.264338890436258,-0.227452398713043,-0.190161791067931,-0.152441756292719,
-0.114634728995588,-0.0764184751015692,-0.0376670804260189,-7.69005437173066E-5),
 .UNSPECIFIED.);
#1897=B_SPLINE_CURVE_WITH_KNOTS('',3,(#68307,#68308,#68309,#68310,#68311,
#68312,#68313,#68314,#68315,#68316,#68317,#68318,#68319,#68320,#68321,#68322,
#68323,#68324,#68325,#68326,#68327,#68328,#68329,#68330,#68331,#68332,#68333,
#68334,#68335,#68336,#68337,#68338,#68339,#68340,#68341,#68342),
 .UNSPECIFIED.,.T.,.F.,(4,2,2,2,2,2,2,2,2,2,2,2,2,2,2,2,2,4),(0.,0.0355202696275121,
0.0730229242186736,0.109881947977543,0.147332215350511,0.185244244850115,
0.223245130804628,0.259644256143591,0.29483879750692,0.330228485401583,
0.366554345814411,0.404791218291486,0.442165216586747,0.480056587414318,
0.518291371434548,0.552548743063418,0.588529668386507,0.599949959182332),
 .UNSPECIFIED.);
#1898=B_SPLINE_CURVE_WITH_KNOTS('',3,(#68343,#68344,#68345,#68346,#68347,
#68348,#68349,#68350,#68351,#68352,#68353,#68354,#68355,#68356,#68357,#68358,
#68359,#68360,#68361,#68362,#68363,#68364,#68365),.UNSPECIFIED.,.F.,.F.,
(4,3,2,2,2,2,2,2,2,2,4),(-7.69005437173066E-5,0.,0.0360098100406934,0.0725977261367332,
0.109413926555899,0.146922956928712,0.185251849369556,0.224065827656858,
0.262360606682867,0.300207053497309,0.301127729713689),.UNSPECIFIED.);
#1899=B_SPLINE_CURVE_WITH_KNOTS('',3,(#68371,#68372,#68373,#68374,#68375,
#68376,#68377,#68378,#68379,#68380,#68381,#68382,#68383,#68384,#68385,#68386,
#68387,#68388,#68389,#68390,#68391,#68392,#68393,#68394,#68395,#68396,#68397,
#68398,#68399,#68400,#68401,#68402,#68403,#68404),.UNSPECIFIED.,.T.,.F.,
(4,2,2,2,2,2,2,2,2,2,2,2,2,2,2,2,4),(-0.317612772210092,-0.29817683215515,
-0.278761042396339,-0.259321595298189,-0.239494618350438,-0.219410736380407,
-0.199190916813444,-0.178820497886802,-0.158948070546673,-0.139427101945941,
-0.120094699680415,-0.100667107706439,-0.0809176240818496,-0.0607258855069793,
-0.0403404075805791,-0.0200982006130535,0.),.UNSPECIFIED.);
#1900=B_SPLINE_CURVE_WITH_KNOTS('',3,(#68408,#68409,#68410,#68411,#68412,
#68413,#68414,#68415,#68416,#68417,#68418,#68419,#68420,#68421,#68422,#68423,
#68424,#68425,#68426,#68427,#68428),.UNSPECIFIED.,.F.,.F.,(4,2,2,2,2,2,
2,2,3,4),(-0.322272493248835,-0.283311097305131,-0.242918471103494,-0.202337942338775,
-0.161792707575712,-0.121445031217079,-0.0810725197347086,-0.0402471007473572,
0.,8.22734960809895E-6),.UNSPECIFIED.);
#1901=B_SPLINE_CURVE_WITH_KNOTS('',3,(#68431,#68432,#68433,#68434,#68435,
#68436,#68437,#68438,#68439,#68440,#68441,#68442,#68443,#68444,#68445,#68446,
#68447,#68448,#68449,#68450,#68451,#68452,#68453,#68454,#68455,#68456,#68457,
#68458,#68459,#68460,#68461,#68462,#68463,#68464,#68465,#68466),
 .UNSPECIFIED.,.T.,.F.,(4,2,2,2,2,2,2,2,2,2,2,2,2,2,2,2,2,4),(0.,0.0399541104210513,
0.0799101633969759,0.120042188030928,0.160349494010625,0.200700062460617,
0.240669149748604,0.281146928548014,0.321688268052903,0.361827692830282,
0.401937446249133,0.441912733332665,0.482224630787743,0.523014478229303,
0.563360237936166,0.603655558777767,0.623959945527549,0.644496878440685),
 .UNSPECIFIED.);
#1902=B_SPLINE_CURVE_WITH_KNOTS('',3,(#68467,#68468,#68469,#68470,#68471,
#68472,#68473,#68474,#68475,#68476,#68477,#68478,#68479,#68480,#68481,#68482,
#68483,#68484,#68485,#68486),.UNSPECIFIED.,.F.,.F.,(4,2,2,2,2,2,2,2,2,4),
(8.22734960809895E-6,0.0388137442425556,0.0787567868575889,0.118683761763293,
0.158793716743972,0.19913884956911,0.239593065809621,0.280403847371113,
0.321081099617034,0.322446122896613),.UNSPECIFIED.);
#1903=B_SPLINE_CURVE_WITH_KNOTS('',3,(#68492,#68493,#68494,#68495,#68496,
#68497,#68498,#68499,#68500,#68501,#68502,#68503,#68504,#68505,#68506,#68507,
#68508,#68509,#68510,#68511,#68512,#68513,#68514,#68515,#68516,#68517,#68518,
#68519,#68520,#68521,#68522,#68523,#68524,#68525),.UNSPECIFIED.,.T.,.F.,
(4,2,2,2,2,2,2,2,2,2,2,2,2,2,2,2,4),(-0.315589991769754,-0.297543654155397,
-0.277607478676899,-0.257621899085537,-0.237642557654303,-0.21771469574947,
-0.197788689069841,-0.177759014798792,-0.158043966994748,-0.138388532458108,
-0.118799826628472,-0.0992263512383482,-0.0796005434512017,-0.0598945213917012,
-0.04013518410926,-0.0199929772862508,0.),.UNSPECIFIED.);
#1904=B_SPLINE_CURVE_WITH_KNOTS('',3,(#68529,#68530,#68531,#68532,#68533,
#68534,#68535,#68536,#68537,#68538,#68539,#68540,#68541,#68542,#68543,#68544,
#68545,#68546),.UNSPECIFIED.,.F.,.F.,(4,2,2,2,2,2,2,2,4),(-0.301156891144586,
-0.264547753021578,-0.226893649082149,-0.190048717511566,-0.152393534543418,
-0.114675560216569,-0.0766170892067709,-0.0379948570526523,-0.000119814599371271),
 .UNSPECIFIED.);
#1905=B_SPLINE_CURVE_WITH_KNOTS('',3,(#68549,#68550,#68551,#68552,#68553,
#68554,#68555,#68556,#68557,#68558,#68559,#68560,#68561,#68562,#68563,#68564,
#68565,#68566,#68567,#68568,#68569,#68570,#68571,#68572,#68573,#68574,#68575,
#68576,#68577,#68578,#68579,#68580,#68581,#68582,#68583,#68584),
 .UNSPECIFIED.,.T.,.F.,(4,2,2,2,2,2,2,2,2,2,2,2,2,2,2,2,2,4),(0.,0.0355202696278532,
0.0730229242199749,0.109881947980052,0.147332215354528,0.185244244855757,
0.223245130812486,0.259644256153658,0.294838797519483,0.330228485416982,
0.366554345832849,0.40479121831343,0.44216521661239,0.480056587444108,0.518291371468795,
0.552548743101786,0.588529668429641,0.599949959225988),.UNSPECIFIED.);
#1906=B_SPLINE_CURVE_WITH_KNOTS('',3,(#68585,#68586,#68587,#68588,#68589,
#68590,#68591,#68592,#68593,#68594,#68595,#68596,#68597,#68598,#68599,#68600,
#68601,#68602,#68603,#68604,#68605,#68606,#68607),.UNSPECIFIED.,.F.,.F.,
(4,3,2,2,2,2,2,2,2,2,4),(-0.000119814599371271,0.,0.0361408497492226,0.0728594924793139,
0.109485135803451,0.14661099959075,0.18449654911239,0.223091526309962,0.261828300698411,
0.299996368157121,0.301150010874056),.UNSPECIFIED.);
#1907=B_SPLINE_CURVE_WITH_KNOTS('',3,(#68613,#68614,#68615,#68616,#68617,
#68618,#68619,#68620,#68621,#68622,#68623,#68624,#68625,#68626,#68627,#68628,
#68629,#68630,#68631,#68632,#68633,#68634,#68635,#68636,#68637,#68638,#68639,
#68640,#68641,#68642,#68643,#68644,#68645,#68646),.UNSPECIFIED.,.T.,.F.,
(4,2,2,2,2,2,2,2,2,2,2,2,2,2,2,2,4),(-0.317634341816681,-0.298273465275683,
-0.278787654783001,-0.25938260516859,-0.239674569645085,-0.219635485556022,
-0.199447957928304,-0.179077235091592,-0.159038453352017,-0.139345729329634,
-0.119946990249479,-0.100601607582497,-0.0810308238562121,-0.06109602261861,
-0.0406271433249967,-0.0202254737216437,0.),.UNSPECIFIED.);
#1908=B_SPLINE_CURVE_WITH_KNOTS('',3,(#68650,#68651,#68652,#68653,#68654,
#68655,#68656,#68657,#68658,#68659,#68660,#68661,#68662,#68663,#68664,#68665,
#68666,#68667),.UNSPECIFIED.,.F.,.F.,(4,2,2,2,2,2,2,2,4),(-0.322263458289222,
-0.282900889548461,-0.242587226965438,-0.202121378962893,-0.161558213341175,
-0.121131727269642,-0.0808194109808987,-0.0402525098016497,-1.03876710068041E-5),
 .UNSPECIFIED.);
#1909=B_SPLINE_CURVE_WITH_KNOTS('',3,(#68670,#68671,#68672,#68673,#68674,
#68675,#68676,#68677,#68678,#68679,#68680,#68681,#68682,#68683,#68684,#68685,
#68686,#68687,#68688,#68689,#68690,#68691,#68692,#68693,#68694,#68695,#68696,
#68697,#68698,#68699,#68700,#68701,#68702,#68703,#68704,#68705),
 .UNSPECIFIED.,.T.,.F.,(4,2,2,2,2,2,2,2,2,2,2,2,2,2,2,2,2,4),(0.,0.0399541104210523,
0.0799101633969911,0.120042188030941,0.160349494010304,0.200700062459907,
0.240669149747547,0.281146928546813,0.321688268051475,0.361827692828482,
0.401937446246947,0.441912733330034,0.482224630784599,0.523014478226203,
0.563360237932926,0.603655558773891,0.623959945523787,0.644496878437038),
 .UNSPECIFIED.);
#1910=B_SPLINE_CURVE_WITH_KNOTS('',3,(#68706,#68707,#68708,#68709,#68710,
#68711,#68712,#68713,#68714,#68715,#68716,#68717,#68718,#68719,#68720,#68721,
#68722,#68723,#68724,#68725,#68726,#68727,#68728),.UNSPECIFIED.,.F.,.F.,
(4,3,2,2,2,2,2,2,2,2,4),(-1.03876710068041E-5,0.,0.0392625678077015,0.0792796756538265,
0.119187885161736,0.159187268402346,0.199422118099274,0.239844848466983,
0.280293454869346,0.321327404961611,0.322443487755003),.UNSPECIFIED.);
#1911=B_SPLINE_CURVE_WITH_KNOTS('',3,(#68734,#68735,#68736,#68737,#68738,
#68739,#68740,#68741,#68742,#68743,#68744,#68745,#68746,#68747,#68748,#68749,
#68750,#68751,#68752,#68753,#68754,#68755,#68756,#68757,#68758,#68759,#68760,
#68761,#68762,#68763,#68764,#68765,#68766,#68767),.UNSPECIFIED.,.T.,.F.,
(4,2,2,2,2,2,2,2,2,2,2,2,2,2,2,2,4),(-0.315584858250283,-0.297326864181455,
-0.27741097433004,-0.257461582863128,-0.237487701039889,-0.217544474680261,
-0.197628413501937,-0.177651504562011,-0.157929072796535,-0.138241416178837,
-0.118623507039874,-0.0990510100831163,-0.0794575655906757,-0.0597904016325671,
-0.0400512984940925,-0.0200862920905489,0.),.UNSPECIFIED.);
#1912=B_SPLINE_CURVE_WITH_KNOTS('',3,(#68771,#68772,#68773,#68774,#68775,
#68776,#68777,#68778,#68779,#68780,#68781,#68782,#68783,#68784,#68785,#68786,
#68787,#68788),.UNSPECIFIED.,.F.,.F.,(4,2,2,2,2,2,2,2,4),(-0.301172697629259,
-0.264933081927209,-0.227255014847489,-0.190345810670057,-0.152699661165205,
-0.115048750531758,-0.077207473536471,-0.0388798599000017,-0.000160983825265968),
 .UNSPECIFIED.);
#1913=B_SPLINE_CURVE_WITH_KNOTS('',3,(#68791,#68792,#68793,#68794,#68795,
#68796,#68797,#68798,#68799,#68800,#68801,#68802,#68803,#68804,#68805,#68806,
#68807,#68808,#68809,#68810,#68811,#68812,#68813,#68814,#68815,#68816,#68817,
#68818,#68819,#68820,#68821,#68822,#68823,#68824,#68825,#68826),
 .UNSPECIFIED.,.T.,.F.,(4,2,2,2,2,2,2,2,2,2,2,2,2,2,2,2,2,4),(0.,0.0355202696277295,
0.0730229242194867,0.109881947979006,0.147332215352552,0.185244244852634,
0.223245130807763,0.259644256147242,0.294838797511455,0.330228485407204,
0.366554345821095,0.404791218299421,0.44216521659611,0.480056587425235,
0.518291371446824,0.552548743077254,0.588529668402066,0.599949959198078),
 .UNSPECIFIED.);
#1914=B_SPLINE_CURVE_WITH_KNOTS('',3,(#68827,#68828,#68829,#68830,#68831,
#68832,#68833,#68834,#68835,#68836,#68837,#68838,#68839,#68840,#68841,#68842,
#68843,#68844,#68845,#68846,#68847,#68848,#68849),.UNSPECIFIED.,.F.,.F.,
(4,3,2,2,2,2,2,2,2,2,4),(-0.000160983825265968,0.,0.0358793027228612,0.0728886733477424,
0.10949360406576,0.14629244320943,0.183767821004726,0.2219434550389,0.260934846486396,
0.299438510889526,0.301156987828858),.UNSPECIFIED.);
#1915=B_SPLINE_CURVE_WITH_KNOTS('',3,(#68855,#68856,#68857,#68858,#68859,
#68860,#68861,#68862,#68863,#68864,#68865,#68866,#68867,#68868,#68869,#68870,
#68871,#68872,#68873,#68874,#68875,#68876,#68877,#68878,#68879,#68880,#68881,
#68882,#68883,#68884,#68885,#68886,#68887,#68888),.UNSPECIFIED.,.T.,.F.,
(4,2,2,2,2,2,2,2,2,2,2,2,2,2,2,2,4),(-0.317647719239506,-0.298200520794536,
-0.278596926941396,-0.25917026528438,-0.239726352873434,-0.21973739477608,
-0.199634745171728,-0.179348387513285,-0.158901547715117,-0.139020909227822,
-0.119487985266671,-0.100147621029955,-0.0807199456085233,-0.060975594285225,
-0.0408050752255367,-0.0203363613524164,0.),.UNSPECIFIED.);
#1916=B_SPLINE_CURVE_WITH_KNOTS('',3,(#68892,#68893,#68894,#68895,#68896,
#68897,#68898,#68899,#68900,#68901,#68902,#68903,#68904,#68905,#68906,#68907,
#68908,#68909),.UNSPECIFIED.,.F.,.F.,(4,2,2,2,2,2,2,2,4),(-0.322308096898006,
-0.283403399723437,-0.243105674074854,-0.202689452701646,-0.162028412209055,
-0.121388392100284,-0.0810028958206459,-0.0406912162856388,-6.69647710747405E-5),
 .UNSPECIFIED.);
#1917=B_SPLINE_CURVE_WITH_KNOTS('',3,(#68912,#68913,#68914,#68915,#68916,
#68917,#68918,#68919,#68920,#68921,#68922,#68923,#68924,#68925,#68926,#68927,
#68928,#68929,#68930,#68931,#68932,#68933,#68934,#68935,#68936,#68937,#68938,
#68939,#68940,#68941,#68942,#68943,#68944,#68945,#68946,#68947),
 .UNSPECIFIED.,.T.,.F.,(4,2,2,2,2,2,2,2,2,2,2,2,2,2,2,2,2,4),(0.,0.0399541104210872,
0.0799101633970701,0.120042188030963,0.160349494010509,0.200700062460821,
0.240669149749049,0.281146928548708,0.32168826805372,0.361827692831149,
0.401937446250155,0.441912733333774,0.482224630788839,0.523014478230791,
0.563360237937848,0.603655558779499,0.623959945529538,0.644496878442784),
 .UNSPECIFIED.);
#1918=B_SPLINE_CURVE_WITH_KNOTS('',3,(#68948,#68949,#68950,#68951,#68952,
#68953,#68954,#68955,#68956,#68957,#68958,#68959,#68960,#68961,#68962,#68963,
#68964,#68965,#68966,#68967,#68968,#68969,#68970),.UNSPECIFIED.,.F.,.F.,
(4,3,2,2,2,2,2,2,2,2,4),(-6.69647710747405E-5,0.,0.0389899751502963,0.0791272762346116,
0.119095234364202,0.159026497444346,0.199115825652264,0.239429199251524,
0.279858625606866,0.320661061518468,0.322378864463958),.UNSPECIFIED.);
#1919=B_SPLINE_CURVE_WITH_KNOTS('',3,(#68976,#68977,#68978,#68979,#68980,
#68981,#68982,#68983,#68984,#68985,#68986,#68987,#68988,#68989,#68990,#68991,
#68992,#68993,#68994,#68995,#68996,#68997,#68998,#68999,#69000,#69001,#69002,
#69003,#69004,#69005,#69006,#69007,#69008,#69009),.UNSPECIFIED.,.T.,.F.,
(4,2,2,2,2,2,2,2,2,2,2,2,2,2,2,2,4),(-0.315576748184792,-0.297053244765837,
-0.277151967701907,-0.257199189469323,-0.237571593074575,-0.217547892466614,
-0.197602911587109,-0.177701138303981,-0.157724828227981,-0.138006616652287,
-0.118340280590273,-0.0987405684270933,-0.079163582765697,-0.0595443936454144,
-0.0398513567435344,-0.0201041897531687,0.),.UNSPECIFIED.);
#1920=B_SPLINE_CURVE_WITH_KNOTS('',3,(#69013,#69014,#69015,#69016,#69017,
#69018,#69019,#69020,#69021,#69022,#69023,#69024,#69025,#69026,#69027,#69028,
#69029,#69030),.UNSPECIFIED.,.F.,.F.,(4,2,2,2,2,2,2,2,4),(-0.301120281951729,
-0.263576382922298,-0.225818802173902,-0.188754997605974,-0.151895401076345,
-0.114142761407066,-0.0764203504572131,-0.0384663620558447,-0.000147603040413052),
 .UNSPECIFIED.);
#1921=B_SPLINE_CURVE_WITH_KNOTS('',3,(#69033,#69034,#69035,#69036,#69037,
#69038,#69039,#69040,#69041,#69042,#69043,#69044,#69045,#69046,#69047,#69048,
#69049,#69050,#69051,#69052,#69053,#69054,#69055,#69056,#69057,#69058,#69059,
#69060,#69061,#69062,#69063,#69064,#69065,#69066,#69067,#69068),
 .UNSPECIFIED.,.T.,.F.,(4,2,2,2,2,2,2,2,2,2,2,2,2,2,2,2,2,4),(0.,0.0355202696276992,
0.0730229242193473,0.109881947978628,0.147332215351885,0.185244244851691,
0.223245130806753,0.259644256146375,0.294838797510505,0.330228485406038,
0.366554345819724,0.404791218297806,0.442165216594333,0.480056587423189,
0.518291371444511,0.552548743074586,0.588529668399033,0.599949959194981),
 .UNSPECIFIED.);
#1922=B_SPLINE_CURVE_WITH_KNOTS('',3,(#69069,#69070,#69071,#69072,#69073,
#69074,#69075,#69076,#69077,#69078,#69079,#69080,#69081,#69082,#69083,#69084,
#69085,#69086,#69087,#69088,#69089,#69090,#69091),.UNSPECIFIED.,.F.,.F.,
(4,3,2,2,2,2,2,2,2,2,4),(-0.000147603040413052,0.,0.0377539037831993,0.0751281221644984,
0.111887841210243,0.148520861419402,0.185616402493165,0.223453147294145,
0.262021736554917,0.300656505695179,0.301204822429525),.UNSPECIFIED.);
#1923=B_SPLINE_CURVE_WITH_KNOTS('',3,(#69097,#69098,#69099,#69100,#69101,
#69102,#69103,#69104,#69105,#69106,#69107,#69108,#69109,#69110,#69111,#69112,
#69113,#69114,#69115,#69116,#69117,#69118,#69119,#69120,#69121,#69122,#69123,
#69124,#69125,#69126,#69127,#69128,#69129,#69130),.UNSPECIFIED.,.T.,.F.,
(4,2,2,2,2,2,2,2,2,2,2,2,2,2,2,2,4),(-0.31764769122437,-0.298126594757583,
-0.278061059087757,-0.25855168614256,-0.239139946378455,-0.219621724224507,
-0.199578995246519,-0.179441223078379,-0.159144891999467,-0.138727517362643,
-0.119005202378359,-0.0995832877709888,-0.080234028709081,-0.060680702994594,
-0.0407740894175593,-0.0203443038622857,0.),.UNSPECIFIED.);
#1924=B_SPLINE_CURVE_WITH_KNOTS('',3,(#69134,#69135,#69136,#69137,#69138,
#69139,#69140,#69141,#69142,#69143,#69144,#69145,#69146,#69147,#69148,#69149,
#69150,#69151),.UNSPECIFIED.,.F.,.F.,(4,2,2,2,2,2,2,2,4),(-0.322294993083104,
-0.283085587582025,-0.242573319111423,-0.202265149720554,-0.161825459085777,
-0.121278611006667,-0.0808520831048596,-0.0405436064875047,-6.00049658257628E-5),
 .UNSPECIFIED.);
#1925=B_SPLINE_CURVE_WITH_KNOTS('',3,(#69154,#69155,#69156,#69157,#69158,
#69159,#69160,#69161,#69162,#69163,#69164,#69165,#69166,#69167,#69168,#69169,
#69170,#69171,#69172,#69173,#69174,#69175,#69176,#69177,#69178,#69179,#69180,
#69181,#69182,#69183,#69184,#69185,#69186,#69187,#69188,#69189),
 .UNSPECIFIED.,.T.,.F.,(4,2,2,2,2,2,2,2,2,2,2,2,2,2,2,2,2,4),(0.,0.0399541104211089,
0.0799101633971605,0.120042188031111,0.160349494010587,0.200700062460756,
0.240669149748765,0.281146928548236,0.321688268053059,0.361827692830262,
0.401937446248863,0.441912733332053,0.482224630786682,0.523014478228254,
0.563360237935002,0.603655558776195,0.623959945526125,0.644496878439372),
 .UNSPECIFIED.);
#1926=B_SPLINE_CURVE_WITH_KNOTS('',3,(#69190,#69191,#69192,#69193,#69194,
#69195,#69196,#69197,#69198,#69199,#69200,#69201,#69202,#69203,#69204,#69205,
#69206,#69207,#69208,#69209,#69210,#69211,#69212),.UNSPECIFIED.,.F.,.F.,
(4,3,2,2,2,2,2,2,2,2,4),(-6.00049658257628E-5,0.,0.0392897850588587,0.079479345871773,
0.119504351273332,0.159417323923056,0.199410327075563,0.239631683305099,
0.280043161873825,0.320485699897508,0.322364974673507),.UNSPECIFIED.);
#1927=B_SPLINE_CURVE_WITH_KNOTS('',3,(#69218,#69219,#69220,#69221,#69222,
#69223,#69224,#69225,#69226,#69227,#69228,#69229,#69230,#69231,#69232,#69233,
#69234,#69235,#69236,#69237,#69238,#69239,#69240,#69241,#69242,#69243,#69244,
#69245,#69246,#69247,#69248,#69249,#69250,#69251),.UNSPECIFIED.,.T.,.F.,
(4,2,2,2,2,2,2,2,2,2,2,2,2,2,2,2,4),(-0.315565835813836,-0.296977761293976,
-0.27700797437709,-0.257093427677873,-0.237151911102798,-0.217186116270328,
-0.197247154373207,-0.177332194059719,-0.157355502362145,-0.137638223444148,
-0.117952752060795,-0.098333751530719,-0.078758992743179,-0.0591645986628483,
-0.039498859894482,-0.0197630645862081,0.),.UNSPECIFIED.);
#1928=B_SPLINE_CURVE_WITH_KNOTS('',3,(#69255,#69256,#69257,#69258,#69259,
#69260,#69261,#69262,#69263,#69264,#69265,#69266,#69267,#69268,#69269,#69270,
#69271,#69272),.UNSPECIFIED.,.F.,.F.,(4,2,2,2,2,2,2,2,4),(-0.301047223106738,
-0.263578632733685,-0.225649522088337,-0.18795353439141,-0.151022848397426,
-0.113722078451354,-0.076039607899864,-0.0382349400305562,-9.66538702340807E-5),
 .UNSPECIFIED.);
#1929=B_SPLINE_CURVE_WITH_KNOTS('',3,(#69275,#69276,#69277,#69278,#69279,
#69280,#69281,#69282,#69283,#69284,#69285,#69286,#69287,#69288,#69289,#69290,
#69291,#69292,#69293,#69294,#69295,#69296,#69297,#69298,#69299,#69300,#69301,
#69302,#69303,#69304,#69305,#69306,#69307,#69308,#69309,#69310),
 .UNSPECIFIED.,.T.,.F.,(4,2,2,2,2,2,2,2,2,2,2,2,2,2,2,2,2,4),(0.,0.0355202696276597,
0.0730229242192084,0.109881947978522,0.147332215351905,0.185244244851805,
0.223245130806825,0.259644256146175,0.29483879750995,0.330228485405148,
0.366554345818643,0.404791218296623,0.442165216592673,0.480056587420968,
0.518291371441852,0.552548743071643,0.588529668395749,0.599949959191659),
 .UNSPECIFIED.);
#1930=B_SPLINE_CURVE_WITH_KNOTS('',3,(#69311,#69312,#69313,#69314,#69315,
#69316,#69317,#69318,#69319,#69320,#69321,#69322,#69323,#69324,#69325,#69326,
#69327,#69328,#69329,#69330,#69331,#69332,#69333),.UNSPECIFIED.,.F.,.F.,
(4,3,2,2,2,2,2,2,2,2,4),(-9.66538702340807E-5,0.,0.0375393633518907,0.0752835051296635,
0.112326473702278,0.148951470060482,0.18574314538863,0.223186825882593,
0.261324249138133,0.300258541488849,0.301234911690416),.UNSPECIFIED.);
#1931=B_SPLINE_CURVE_WITH_KNOTS('',3,(#69339,#69340,#69341,#69342,#69343,
#69344,#69345,#69346,#69347,#69348,#69349,#69350,#69351,#69352,#69353,#69354,
#69355,#69356,#69357,#69358,#69359,#69360,#69361,#69362,#69363,#69364,#69365,
#69366,#69367,#69368,#69369,#69370,#69371,#69372),.UNSPECIFIED.,.T.,.F.,
(4,2,2,2,2,2,2,2,2,2,2,2,2,2,2,2,4),(-0.317629464904961,-0.297714272038367,
-0.277577500901888,-0.257956254729707,-0.238517861015399,-0.219074978638032,
-0.199269307107419,-0.179183937587056,-0.158941321785611,-0.138538737217386,
-0.11863886681209,-0.099083234988701,-0.0797310797511626,-0.0603101816157416,
-0.0405879439157434,-0.0204362250140278,0.),.UNSPECIFIED.);
#1932=B_SPLINE_CURVE_WITH_KNOTS('',3,(#69376,#69377,#69378,#69379,#69380,
#69381,#69382,#69383,#69384,#69385,#69386,#69387,#69388,#69389,#69390,#69391,
#69392,#69393),.UNSPECIFIED.,.F.,.F.,(4,2,2,2,2,2,2,2,4),(-0.322273280496128,
-0.283164066278084,-0.242313649635905,-0.201927757921193,-0.161607273321421,
-0.121157355445028,-0.080708923195034,-0.0403897617268959,-4.12631041346659E-5),
 .UNSPECIFIED.);
#1933=B_SPLINE_CURVE_WITH_KNOTS('',3,(#69396,#69397,#69398,#69399,#69400,
#69401,#69402,#69403,#69404,#69405,#69406,#69407,#69408,#69409,#69410,#69411,
#69412,#69413,#69414,#69415,#69416,#69417,#69418,#69419,#69420,#69421,#69422,
#69423,#69424,#69425,#69426,#69427,#69428,#69429,#69430,#69431),
 .UNSPECIFIED.,.T.,.F.,(4,2,2,2,2,2,2,2,2,2,2,2,2,2,2,2,2,4),(0.,0.0399541104210812,
0.0799101633970315,0.120042188030822,0.160349494010275,0.200700062460568,
0.240669149748756,0.281146928548416,0.321688268053484,0.361827692830935,
0.401937446249939,0.441912733333782,0.482224630788817,0.523014478230698,
0.563360237937675,0.603655558779108,0.623959945529211,0.644496878442527),
 .UNSPECIFIED.);
#1934=B_SPLINE_CURVE_WITH_KNOTS('',3,(#69432,#69433,#69434,#69435,#69436,
#69437,#69438,#69439,#69440,#69441,#69442,#69443,#69444,#69445,#69446,#69447,
#69448,#69449,#69450,#69451,#69452,#69453,#69454),.UNSPECIFIED.,.F.,.F.,
(4,3,2,2,2,2,2,2,2,2,4),(-4.12631041346659E-5,0.,0.0399675679442238,0.0801897951235173,
0.120290688199724,0.160233372859482,0.200158067921408,0.240260671009271,
0.280600379519264,0.321053048499667,0.322354423090216),.UNSPECIFIED.);
#1935=B_SPLINE_CURVE_WITH_KNOTS('',3,(#69460,#69461,#69462,#69463,#69464,
#69465,#69466,#69467,#69468,#69469,#69470,#69471,#69472,#69473,#69474,#69475,
#69476,#69477,#69478,#69479,#69480,#69481,#69482,#69483,#69484,#69485,#69486,
#69487,#69488,#69489,#69490,#69491,#69492,#69493),.UNSPECIFIED.,.T.,.F.,
(4,2,2,2,2,2,2,2,2,2,2,2,2,2,2,2,4),(-0.315553268146494,-0.297304300154847,
-0.277232874841197,-0.257288395179118,-0.237380069391282,-0.217453712880523,
-0.197526993272217,-0.177618574645662,-0.157675821289914,-0.137607666323394,
-0.117904352341964,-0.0982559940572506,-0.0786687230926247,-0.0590935104011807,
-0.0394653656100249,-0.0197579638748003,0.),.UNSPECIFIED.);
#1936=B_SPLINE_CURVE_WITH_KNOTS('',3,(#69497,#69498,#69499,#69500,#69501,
#69502,#69503,#69504,#69505,#69506,#69507,#69508,#69509,#69510,#69511,#69512,
#69513,#69514),.UNSPECIFIED.,.F.,.F.,(4,2,2,2,2,2,2,2,4),(-0.301109175947192,
-0.262812042982321,-0.224724316953933,-0.186970956972154,-0.149886488164483,
-0.11301762842648,-0.0756285515230846,-0.0379138418272327,-0.000181832202353105),
 .UNSPECIFIED.);
#1937=B_SPLINE_CURVE_WITH_KNOTS('',3,(#69517,#69518,#69519,#69520,#69521,
#69522,#69523,#69524,#69525,#69526,#69527,#69528,#69529,#69530,#69531,#69532,
#69533,#69534,#69535,#69536,#69537,#69538,#69539,#69540,#69541,#69542,#69543,
#69544,#69545,#69546,#69547,#69548,#69549,#69550,#69551,#69552),
 .UNSPECIFIED.,.T.,.F.,(4,2,2,2,2,2,2,2,2,2,2,2,2,2,2,2,2,4),(0.,0.0355202696277283,
0.0730229242195419,0.109881947979107,0.147332215352648,0.185244244852912,
0.223245130808583,0.25964425614879,0.294838797513527,0.330228485409711,
0.366554345824243,0.404791218303629,0.442165216601193,0.480056587431119,
0.518291371453736,0.552548743085037,0.588529668410891,0.59994995920701),
 .UNSPECIFIED.);
#1938=B_SPLINE_CURVE_WITH_KNOTS('',3,(#69553,#69554,#69555,#69556,#69557,
#69558,#69559,#69560,#69561,#69562,#69563,#69564,#69565,#69566,#69567,#69568,
#69569,#69570,#69571,#69572,#69573,#69574,#69575,#69576,#69577),
 .UNSPECIFIED.,.F.,.F.,(4,3,2,2,2,2,2,2,2,2,2,4),(-0.000181832202353105,
0.,9.38366536167301E-5,0.0385047798493244,0.0765518818810497,0.113953342602953,
0.150737446188046,0.187371554731283,0.224440136490084,0.262235508831512,
0.300767100191795,0.301097788245665),.UNSPECIFIED.);
#1939=B_SPLINE_CURVE_WITH_KNOTS('',3,(#69583,#69584,#69585,#69586,#69587,
#69588,#69589,#69590,#69591,#69592,#69593,#69594,#69595,#69596,#69597,#69598,
#69599,#69600,#69601,#69602,#69603,#69604,#69605,#69606,#69607,#69608,#69609,
#69610,#69611,#69612,#69613,#69614,#69615,#69616),.UNSPECIFIED.,.T.,.F.,
(4,2,2,2,2,2,2,2,2,2,2,2,2,2,2,2,4),(-0.317594533089036,-0.297902075164115,
-0.277717583659871,-0.257653287417695,-0.238130426363534,-0.218714109872533,
-0.199204998726052,-0.179166112450341,-0.159044764786859,-0.138770672776784,
-0.118368847123579,-0.0986295682412476,-0.0791930104351003,-0.0598423732615011,
-0.0403036962525294,-0.0204206770504485,0.),.UNSPECIFIED.);
#1940=B_SPLINE_CURVE_WITH_KNOTS('',3,(#69620,#69621,#69622,#69623,#69624,
#69625,#69626,#69627,#69628,#69629,#69630,#69631,#69632,#69633,#69634,#69635,
#69636,#69637,#69638,#69639,#69640),.UNSPECIFIED.,.F.,.F.,(4,2,2,2,2,2,
2,2,3,4),(-0.322212451494843,-0.283737281153516,-0.242722123714327,-0.202268209971048,
-0.161970355596362,-0.121472143151954,-0.0808174241678842,-0.0403032184405623,
0.,3.41805086617603E-5),.UNSPECIFIED.);
#1941=B_SPLINE_CURVE_WITH_KNOTS('',3,(#69643,#69644,#69645,#69646,#69647,
#69648,#69649,#69650,#69651,#69652,#69653,#69654,#69655,#69656,#69657,#69658,
#69659,#69660,#69661,#69662,#69663,#69664,#69665,#69666,#69667,#69668,#69669,
#69670,#69671,#69672,#69673,#69674,#69675,#69676,#69677,#69678),
 .UNSPECIFIED.,.T.,.F.,(4,2,2,2,2,2,2,2,2,2,2,2,2,2,2,2,2,4),(0.,0.0399541104211557,
0.0799101633973391,0.120042188031283,0.160349494010752,0.200700062461029,
0.240669149749152,0.281146928548658,0.321688268053438,0.361827692830745,
0.401937446249819,0.441912733333285,0.482224630788115,0.523014478229936,
0.563360237936776,0.603655558778112,0.623959945528129,0.644496878441407),
 .UNSPECIFIED.);
#1942=B_SPLINE_CURVE_WITH_KNOTS('',3,(#69679,#69680,#69681,#69682,#69683,
#69684,#69685,#69686,#69687,#69688,#69689,#69690,#69691,#69692,#69693,#69694,
#69695,#69696,#69697,#69698),.UNSPECIFIED.,.F.,.F.,(4,2,2,2,2,2,2,2,2,4),
(3.41805086617603E-5,0.0394732086774792,0.079701088033428,0.119906369771394,
0.159959613748505,0.199889421771116,0.239872401764791,0.280061608671928,
0.320438058972153,0.32238398619812),.UNSPECIFIED.);
#1943=B_SPLINE_CURVE_WITH_KNOTS('',3,(#69704,#69705,#69706,#69707,#69708,
#69709,#69710,#69711,#69712,#69713,#69714,#69715,#69716,#69717,#69718,#69719,
#69720,#69721,#69722,#69723,#69724,#69725,#69726,#69727,#69728,#69729,#69730,
#69731,#69732,#69733,#69734,#69735,#69736,#69737),.UNSPECIFIED.,.T.,.F.,
(4,2,2,2,2,2,2,2,2,2,2,2,2,2,2,2,4),(-0.315539422451451,-0.29764665964427,
-0.277579650597126,-0.25764437253977,-0.237734954471469,-0.217762026234666,
-0.19774279120852,-0.17776218314531,-0.157848862492919,-0.137922119941295,
-0.117871746268506,-0.0981780349529489,-0.078545939200476,-0.0589630124018614,
-0.0393717766439356,-0.0197194318849499,0.),.UNSPECIFIED.);
#1944=B_SPLINE_CURVE_WITH_KNOTS('',3,(#69741,#69742,#69743,#69744,#69745,
#69746,#69747,#69748,#69749,#69750,#69751,#69752,#69753,#69754,#69755,#69756,
#69757,#69758),.UNSPECIFIED.,.F.,.F.,(4,2,2,2,2,2,2,2,4),(-0.301006762787625,
-0.264925988556105,-0.226376240130882,-0.188384262261974,-0.150702655161475,
-0.113069725454281,-0.0754287199925444,-0.0377927671943644,-6.79809902074358E-5),
 .UNSPECIFIED.);
#1945=B_SPLINE_CURVE_WITH_KNOTS('',3,(#69761,#69762,#69763,#69764,#69765,
#69766,#69767,#69768,#69769,#69770,#69771,#69772,#69773,#69774,#69775,#69776,
#69777,#69778,#69779,#69780,#69781,#69782,#69783,#69784,#69785,#69786,#69787,
#69788,#69789,#69790,#69791,#69792,#69793,#69794,#69795,#69796),
 .UNSPECIFIED.,.T.,.F.,(4,2,2,2,2,2,2,2,2,2,2,2,2,2,2,2,2,4),(0.,0.0355202696277629,
0.0730229242196933,0.109881947979405,0.147332215353019,0.185244244853643,
0.223245130809453,0.259644256149627,0.294838797514426,0.330228485410828,
0.366554345825704,0.404791218305273,0.442165216603097,0.480056587433275,
0.518291371456087,0.552548743087593,0.58852966841366,0.599949959209818),
 .UNSPECIFIED.);
#1946=B_SPLINE_CURVE_WITH_KNOTS('',3,(#69797,#69798,#69799,#69800,#69801,
#69802,#69803,#69804,#69805,#69806,#69807,#69808,#69809,#69810,#69811,#69812,
#69813,#69814,#69815,#69816,#69817,#69818,#69819),.UNSPECIFIED.,.F.,.F.,
(4,3,2,2,2,2,2,2,2,2,4),(-6.79809902074358E-5,0.,0.0356803651782013,0.0744612460975631,
0.112238318105394,0.14932462663091,0.185963804099021,0.222722923188193,
0.260104146420146,0.298186022335344,0.301109163651249),.UNSPECIFIED.);
#1947=B_SPLINE_CURVE_WITH_KNOTS('',3,(#69825,#69826,#69827,#69828,#69829,
#69830,#69831,#69832,#69833,#69834,#69835,#69836,#69837,#69838,#69839,#69840,
#69841,#69842,#69843,#69844,#69845,#69846,#69847,#69848,#69849,#69850,#69851,
#69852,#69853,#69854,#69855,#69856,#69857,#69858),.UNSPECIFIED.,.T.,.F.,
(4,2,2,2,2,2,2,2,2,2,2,2,2,2,2,2,4),(-0.317546919319209,-0.298237181118452,
-0.27788599623212,-0.257722699827236,-0.237703531338022,-0.218259701974539,
-0.198818616029039,-0.178839663119116,-0.158758082875245,-0.138499360197678,
-0.118073251856203,-0.0981722626108359,-0.0786104829396448,-0.0592550425800418,
-0.0398390935163074,-0.0201296135639513,0.),.UNSPECIFIED.);
#1948=B_SPLINE_CURVE_WITH_KNOTS('',3,(#69862,#69863,#69864,#69865,#69866,
#69867,#69868,#69869,#69870,#69871,#69872,#69873,#69874,#69875,#69876,#69877,
#69878,#69879),.UNSPECIFIED.,.F.,.F.,(4,2,2,2,2,2,2,2,4),(-0.322300981754088,
-0.28318251522055,-0.242774753788783,-0.201858981303984,-0.16144569609712,
-0.121144311498917,-0.0807322407035335,-0.0403094094323443,-4.72125003703735E-5),
 .UNSPECIFIED.);
#1949=B_SPLINE_CURVE_WITH_KNOTS('',3,(#69882,#69883,#69884,#69885,#69886,
#69887,#69888,#69889,#69890,#69891,#69892,#69893,#69894,#69895,#69896,#69897,
#69898,#69899,#69900,#69901,#69902,#69903,#69904,#69905,#69906,#69907,#69908,
#69909,#69910,#69911,#69912,#69913,#69914,#69915,#69916,#69917),
 .UNSPECIFIED.,.T.,.F.,(4,2,2,2,2,2,2,2,2,2,2,2,2,2,2,2,2,4),(0.,0.0399541104209768,
0.0799101633966359,0.120042188030262,0.160349494009563,0.200700062459491,
0.240669149747351,0.281146928546543,0.321688268050956,0.361827692827786,
0.401937446246216,0.441912733329095,0.482224630783251,0.523014478224417,
0.563360237930717,0.603655558771478,0.623959945521238,0.644496878434432),
 .UNSPECIFIED.);
#1950=B_SPLINE_CURVE_WITH_KNOTS('',3,(#69918,#69919,#69920,#69921,#69922,
#69923,#69924,#69925,#69926,#69927,#69928,#69929,#69930,#69931,#69932,#69933,
#69934,#69935,#69936,#69937,#69938,#69939,#69940),.UNSPECIFIED.,.F.,.F.,
(4,3,2,2,2,2,2,2,2,2,4),(-4.72125003703735E-5,0.,0.0401541608355253,0.0803379018857595,
0.120550355458553,0.160650987023366,0.200596462646156,0.2405175782139,0.280609074525696,
0.320937808358075,0.322266789344037),.UNSPECIFIED.);
#1951=B_SPLINE_CURVE_WITH_KNOTS('',3,(#69946,#69947,#69948,#69949,#69950,
#69951,#69952,#69953,#69954,#69955,#69956,#69957,#69958,#69959,#69960,#69961,
#69962,#69963,#69964,#69965,#69966,#69967,#69968,#69969,#69970,#69971,#69972,
#69973,#69974,#69975,#69976,#69977,#69978,#69979),.UNSPECIFIED.,.T.,.F.,
(4,2,2,2,2,2,2,2,2,2,2,2,2,2,2,2,4),(-0.31552451047958,-0.297280907827344,
-0.277523391905511,-0.257428902418356,-0.237473497248995,-0.217571624881194,
-0.197661500232289,-0.177749354472922,-0.157848485240125,-0.137907777204664,
-0.117838620146662,-0.09813907693786,-0.0784912592307547,-0.0589032081742604,
-0.0393286932776206,-0.0197035504924225,0.),.UNSPECIFIED.);
#1952=B_SPLINE_CURVE_WITH_KNOTS('',3,(#69983,#69984,#69985,#69986,#69987,
#69988,#69989,#69990,#69991,#69992,#69993,#69994,#69995,#69996,#69997,#69998,
#69999,#70000),.UNSPECIFIED.,.F.,.F.,(4,2,2,2,2,2,2,2,4),(-0.301015621190795,
-0.26464913614506,-0.225860948774485,-0.187630348606652,-0.149844101969181,
-0.112198999979826,-0.0753249907283473,-0.037674212913492,-9.15455865655557E-5),
 .UNSPECIFIED.);
#1953=B_SPLINE_CURVE_WITH_KNOTS('',3,(#70003,#70004,#70005,#70006,#70007,
#70008,#70009,#70010,#70011,#70012,#70013,#70014,#70015,#70016,#70017,#70018,
#70019,#70020,#70021,#70022,#70023,#70024,#70025,#70026,#70027,#70028,#70029,
#70030,#70031,#70032,#70033,#70034,#70035,#70036,#70037,#70038),
 .UNSPECIFIED.,.T.,.F.,(4,2,2,2,2,2,2,2,2,2,2,2,2,2,2,2,2,4),(0.,0.0355202696278056,
0.0730229242197536,0.109881947979361,0.147332215353219,0.185244244853985,
0.223245130809959,0.259644256150568,0.29483879751575,0.330228485412583,
0.366554345827937,0.404791218307693,0.442165216605726,0.48005658743653,
0.518291371460154,0.552548743092215,0.588529668419006,0.599949959215237),
 .UNSPECIFIED.);
#1954=B_SPLINE_CURVE_WITH_KNOTS('',3,(#70039,#70040,#70041,#70042,#70043,
#70044,#70045,#70046,#70047,#70048,#70049,#70050,#70051,#70052,#70053,#70054,
#70055,#70056,#70057,#70058,#70059,#70060,#70061),.UNSPECIFIED.,.F.,.F.,
(4,3,2,2,2,2,2,2,2,2,4),(-9.15455865655557E-5,0.,0.0367498513809987,0.0752209939176623,
0.113273329807805,0.15070796959203,0.187516731080181,0.224138077913942,
0.261156975549728,0.298894829763992,0.300991424502598),.UNSPECIFIED.);
#1955=B_SPLINE_CURVE_WITH_KNOTS('',3,(#70067,#70068,#70069,#70070,#70071,
#70072,#70073,#70074,#70075,#70076,#70077,#70078,#70079,#70080,#70081,#70082,
#70083,#70084,#70085,#70086,#70087,#70088,#70089,#70090,#70091,#70092,#70093,
#70094,#70095,#70096,#70097,#70098,#70099,#70100),.UNSPECIFIED.,.T.,.F.,
(4,2,2,2,2,2,2,2,2,2,2,2,2,2,2,2,4),(-0.317488428877463,-0.298036515488589,
-0.277628055879793,-0.25738424350405,-0.237308164390969,-0.21778572227554,
-0.198368809302504,-0.178862365231032,-0.158846741703291,-0.138701111469329,
-0.11837423341009,-0.0979264050779261,-0.078190697669169,-0.0587545592685796,
-0.0394060149601878,-0.0198735656069791,0.),.UNSPECIFIED.);
#1956=B_SPLINE_CURVE_WITH_KNOTS('',3,(#70104,#70105,#70106,#70107,#70108,
#70109,#70110,#70111,#70112,#70113,#70114,#70115,#70116,#70117,#70118,#70119,
#70120,#70121),.UNSPECIFIED.,.F.,.F.,(4,2,2,2,2,2,2,2,4),(-0.322341080919583,
-0.283397192137026,-0.242965114707,-0.202207166282649,-0.161620101984401,
-0.12131449207317,-0.0809262451179171,-0.0404192807283227,-7.52860376557503E-5),
 .UNSPECIFIED.);
#1957=B_SPLINE_CURVE_WITH_KNOTS('',3,(#70124,#70125,#70126,#70127,#70128,
#70129,#70130,#70131,#70132,#70133,#70134,#70135,#70136,#70137,#70138,#70139,
#70140,#70141,#70142,#70143,#70144,#70145,#70146,#70147,#70148,#70149,#70150,
#70151,#70152,#70153,#70154,#70155,#70156,#70157,#70158,#70159,#70160,#70161,
#70162,#70163,#70164,#70165,#70166,#70167,#70168,#70169,#70170,#70171),
 .UNSPECIFIED.,.T.,.F.,(4,2,2,2,2,2,2,2,2,2,2,2,2,2,2,2,2,2,2,2,2,2,2,4),
(0.,0.0335113392274846,0.0695662695919637,0.108091819664512,0.148791621535511,
0.188697016176582,0.228911969541493,0.248549485762229,0.261288477298313,
0.266974681879587,0.279405337299656,0.297653721121311,0.335724703623805,
0.370458461479632,0.40772209622371,0.447602408687505,0.488121713087397,
0.527106132404311,0.559214002352181,0.575561093124945,0.587383293115077,
0.599420863476123,0.616221156668834,0.644049639714414),.UNSPECIFIED.);
#1958=B_SPLINE_CURVE_WITH_KNOTS('',3,(#70172,#70173,#70174,#70175,#70176,
#70177,#70178,#70179,#70180,#70181,#70182,#70183,#70184,#70185,#70186,#70187,
#70188,#70189,#70190,#70191,#70192,#70193,#70194),.UNSPECIFIED.,.F.,.F.,
(4,3,2,2,2,2,2,2,2,2,4),(-7.52860376557503E-5,0.,0.0397392322804878,0.0802354008620384,
0.120447425093409,0.16063007506737,0.200664146488323,0.240582108771279,
0.280562031686767,0.320758571866905,0.322205986735066),.UNSPECIFIED.);
#1959=B_SPLINE_CURVE_WITH_KNOTS('',3,(#70200,#70201,#70202,#70203,#70204,
#70205,#70206,#70207,#70208,#70209,#70210,#70211,#70212,#70213,#70214,#70215,
#70216,#70217,#70218,#70219,#70220,#70221,#70222,#70223,#70224,#70225,#70226,
#70227,#70228,#70229,#70230,#70231,#70232,#70233),.UNSPECIFIED.,.T.,.F.,
(4,2,2,2,2,2,2,2,2,2,2,2,2,2,2,2,4),(-0.315511801736032,-0.297322926516652,
-0.277567954138442,-0.257424067681664,-0.237430365844225,-0.217516351887858,
-0.197593634790712,-0.177646959906082,-0.157717567973084,-0.137807467592321,
-0.117838533294104,-0.0981312561837001,-0.0784480093982619,-0.0588252961267834,
-0.0392478427160484,-0.0196569263325427,0.),.UNSPECIFIED.);
#1960=B_SPLINE_CURVE_WITH_KNOTS('',3,(#70237,#70238,#70239,#70240,#70241,
#70242,#70243,#70244,#70245,#70246,#70247,#70248,#70249,#70250,#70251,#70252,
#70253,#70254),.UNSPECIFIED.,.F.,.F.,(4,2,2,2,2,2,2,2,4),(-0.301008850825269,
-0.26442428051724,-0.225539555035701,-0.187129468600546,-0.14922300031385,
-0.111530253351743,-0.0745692246178906,-0.0377021715762848,-9.92896090334623E-5),
 .UNSPECIFIED.);
#1961=B_SPLINE_CURVE_WITH_KNOTS('',3,(#70257,#70258,#70259,#70260,#70261,
#70262,#70263,#70264,#70265,#70266,#70267,#70268,#70269,#70270,#70271,#70272,
#70273,#70274,#70275,#70276,#70277,#70278,#70279,#70280,#70281,#70282,#70283,
#70284,#70285,#70286,#70287,#70288,#70289,#70290,#70291,#70292),
 .UNSPECIFIED.,.T.,.F.,(4,2,2,2,2,2,2,2,2,2,2,2,2,2,2,2,2,4),(0.,0.0355202696276149,
0.0730229242189981,0.109881947977939,0.147332215351036,0.185244244850885,
0.223245130805628,0.259644256144758,0.294838797508318,0.330228485403177,
0.366554345816096,0.404791218293387,0.442165216588983,0.480056587416825,
0.51829137143723,0.552548743066467,0.588529668389975,0.599949959185819),
 .UNSPECIFIED.);
#1962=B_SPLINE_CURVE_WITH_KNOTS('',3,(#70293,#70294,#70295,#70296,#70297,
#70298,#70299,#70300,#70301,#70302,#70303,#70304,#70305,#70306,#70307,#70308,
#70309,#70310,#70311,#70312,#70313,#70314,#70315),.UNSPECIFIED.,.F.,.F.,
(4,3,2,2,2,2,2,2,2,2,4),(-9.92896090334623E-5,0.,0.0371215071931662,0.0751963489563421,
0.113814279468518,0.151609467281234,0.18872289670269,0.22537433686428,0.262116084041776,
0.299451874579786,0.3008946113259),.UNSPECIFIED.);
#1963=B_SPLINE_CURVE_WITH_KNOTS('',3,(#70321,#70322,#70323,#70324,#70325,
#70326,#70327,#70328,#70329,#70330,#70331,#70332,#70333,#70334,#70335,#70336,
#70337,#70338,#70339,#70340,#70341,#70342,#70343,#70344,#70345,#70346,#70347,
#70348,#70349,#70350,#70351,#70352,#70353,#70354),.UNSPECIFIED.,.T.,.F.,
(4,2,2,2,2,2,2,2,2,2,2,2,2,2,2,2,4),(-0.31742888296956,-0.297614680988988,
-0.277216006988426,-0.256943128376054,-0.236826826287557,-0.217180233857531,
-0.197728370920642,-0.178297477151747,-0.158518654238573,-0.138464191712988,
-0.118284269507906,-0.0979458955695503,-0.078023359766043,-0.0584366788244967,
-0.0390722257779513,-0.0196727140138107,0.),.UNSPECIFIED.);
#1964=B_SPLINE_CURVE_WITH_KNOTS('',3,(#70360,#70361,#70362,#70363,#70364,
#70365,#70366,#70367,#70368,#70369,#70370,#70371,#70372,#70373,#70374,#70375,
#70376,#70377,#70378,#70379,#70380,#70381,#70382,#70383,#70384,#70385,#70386,
#70387,#70388,#70389,#70390,#70391,#70392,#70393,#70394,#70395,#70396,#70397,
#70398,#70399,#70400,#70401,#70402,#70403),.UNSPECIFIED.,.T.,.F.,(4,2,2,
2,2,2,2,2,2,2,2,2,2,2,2,2,2,2,2,2,2,4),(0.,0.0127770956840893,0.0401769293152859,
0.0780448846179358,0.139821331639922,0.195108267791615,0.25352997178776,
0.31553240477771,0.376490923311257,0.438446166471974,0.474035280748466,
0.500390883434378,0.526892757452704,0.56201393628215,0.624036266196096,
0.678511078694792,0.736162275713911,0.797543466099766,0.858642911548674,
0.920080478592296,0.956389836746744,0.97628076565265),.UNSPECIFIED.);
#1965=B_SPLINE_CURVE_WITH_KNOTS('',3,(#70415,#70416,#70417,#70418,#70419,
#70420,#70421,#70422,#70423,#70424,#70425,#70426,#70427,#70428,#70429,#70430,
#70431,#70432,#70433,#70434,#70435,#70436,#70437,#70438,#70439,#70440,#70441,
#70442,#70443,#70444,#70445,#70446,#70447,#70448,#70449,#70450,#70451,#70452,
#70453,#70454,#70455,#70456,#70457,#70458,#70459,#70460),.UNSPECIFIED.,
 .T.,.F.,(4,2,2,2,2,2,2,2,2,2,2,2,2,2,2,2,2,2,2,2,2,2,4),(0.,0.00956491245687488,
0.030883344589073,0.0618829516961483,0.112184753046831,0.156999876022228,
0.204430459079411,0.254727738816217,0.304367474343013,0.353938489206773,
0.383699609227687,0.404561462882039,0.414031956382108,0.435291839053782,
0.466616523466818,0.517017233475614,0.561720661065273,0.609373928277655,
0.659517635087295,0.708833303469572,0.754032026996831,0.78008309963919,
0.793860837770021),.UNSPECIFIED.);
#1966=B_SPLINE_CURVE_WITH_KNOTS('',3,(#70470,#70471,#70472,#70473,#70474,
#70475,#70476,#70477,#70478,#70479,#70480,#70481,#70482,#70483,#70484,#70485,
#70486,#70487),.UNSPECIFIED.,.F.,.F.,(4,2,2,2,2,2,2,2,4),(-0.32228159478291,
-0.283799439738403,-0.243381635204158,-0.202597493718955,-0.161764444001045,
-0.121394670185239,-0.0810652882896529,-0.0405499785426211,-6.66314878022331E-6),
 .UNSPECIFIED.);
#1967=B_SPLINE_CURVE_WITH_KNOTS('',3,(#70490,#70491,#70492,#70493,#70494,
#70495,#70496,#70497,#70498,#70499,#70500,#70501,#70502,#70503,#70504,#70505,
#70506,#70507,#70508,#70509,#70510,#70511,#70512,#70513,#70514,#70515,#70516,
#70517,#70518,#70519,#70520,#70521,#70522,#70523,#70524,#70525,#70526,#70527,
#70528,#70529,#70530,#70531,#70532,#70533,#70534,#70535,#70536,#70537,#70538,
#70539,#70540,#70541),.UNSPECIFIED.,.T.,.F.,(4,2,2,2,2,2,2,2,2,2,2,2,2,
2,2,2,2,2,2,2,2,2,2,2,2,4),(0.,0.0282895937381302,0.0604612061645479,0.0955483414317913,
0.133156791658192,0.173259107140958,0.2138054447814,0.252451243352889,0.283476215783229,
0.297624487910025,0.307274542296832,0.311654955761004,0.321804811499666,
0.337921929043092,0.375015994336447,0.40903555725717,0.446013229785303,
0.486013466010895,0.526529373075068,0.564703570234459,0.599506180594163,
0.613229117562791,0.622237737759,0.626302999451298,0.635646637048587,0.644410107943693),
 .UNSPECIFIED.);
#1968=B_SPLINE_CURVE_WITH_KNOTS('',3,(#70542,#70543,#70544,#70545,#70546,
#70547,#70548,#70549,#70550,#70551,#70552,#70553,#70554,#70555,#70556,#70557,
#70558,#70559,#70560,#70561,#70562,#70563,#70564),.UNSPECIFIED.,.F.,.F.,
(4,3,2,2,2,2,2,2,2,2,4),(-6.66314878022331E-6,0.,0.0391495632548314,0.0794647813952141,
0.120127711159877,0.160348499619285,0.200480693554725,0.240456530427129,
0.280381832209827,0.32044609784586,0.322252227541039),.UNSPECIFIED.);
#1969=B_SPLINE_CURVE_WITH_KNOTS('',3,(#70570,#70571,#70572,#70573,#70574,
#70575,#70576,#70577,#70578,#70579,#70580,#70581,#70582,#70583,#70584,#70585,
#70586,#70587,#70588,#70589,#70590,#70591,#70592,#70593,#70594,#70595,#70596,
#70597,#70598,#70599,#70600,#70601,#70602,#70603),.UNSPECIFIED.,.T.,.F.,
(4,2,2,2,2,2,2,2,2,2,2,2,2,2,2,2,4),(-0.315502449039155,-0.297515748826024,
-0.277778880448211,-0.257824981175595,-0.237783331527644,-0.217855184230197,
-0.197937909351415,-0.177974799956127,-0.158002028094032,-0.138072732783704,
-0.118158524215663,-0.0981590114967407,-0.0784549137780755,-0.0587934272076247,
-0.0391924430371145,-0.0196151302800391,0.),.UNSPECIFIED.);
#1970=B_SPLINE_CURVE_WITH_KNOTS('',3,(#70607,#70608,#70609,#70610,#70611,
#70612,#70613,#70614,#70615,#70616,#70617,#70618,#70619,#70620,#70621,#70622,
#70623,#70624,#70625,#70626,#70627),.UNSPECIFIED.,.F.,.F.,(4,2,2,2,2,2,
2,2,3,4),(-0.300867269446679,-0.266056862620371,-0.227808585743502,-0.188962005203739,
-0.150665481576804,-0.11285491655002,-0.0752335214926206,-0.037614382743869,
0.,4.23225959967841E-5),.UNSPECIFIED.);
#1971=B_SPLINE_CURVE_WITH_KNOTS('',3,(#70630,#70631,#70632,#70633,#70634,
#70635,#70636,#70637,#70638,#70639,#70640,#70641,#70642,#70643,#70644,#70645,
#70646,#70647,#70648,#70649,#70650,#70651,#70652,#70653,#70654,#70655,#70656,
#70657,#70658,#70659,#70660,#70661,#70662,#70663,#70664,#70665,#70666,#70667,
#70668,#70669,#70670,#70671,#70672,#70673,#70674,#70675,#70676,#70677,#70678,
#70679,#70680,#70681,#70682,#70683),.UNSPECIFIED.,.T.,.F.,(4,2,2,2,2,2,
2,2,2,2,2,2,2,2,2,2,2,2,2,2,2,2,2,2,2,2,4),(0.,0.029081491771507,0.0612502674553373,
0.0961097574703367,0.133607299680108,0.171385053584874,0.206641008499803,
0.237112772984767,0.249042656047471,0.256728934232189,0.260169709018563,
0.267882879740654,0.279907399797955,0.312932772577639,0.343668137806066,
0.377290154421155,0.413624402754248,0.451812104238219,0.488740715671467,
0.523779739364488,0.54324113697516,0.552348398814064,0.556143993023423,
0.559504603731152,0.5668581250006,0.578100823004826,0.599543898462904),
 .UNSPECIFIED.);
#1972=B_SPLINE_CURVE_WITH_KNOTS('',3,(#70684,#70685,#70686,#70687,#70688,
#70689,#70690,#70691,#70692,#70693,#70694,#70695,#70696,#70697,#70698,#70699,
#70700,#70701,#70702,#70703),.UNSPECIFIED.,.F.,.F.,(4,2,2,2,2,2,2,2,2,4),
(4.23225959967841E-5,0.0357919825936412,0.0736951427824967,0.11213398720573,
0.150200682323832,0.187678724930752,0.224519795797413,0.261130708849028,
0.29809507630152,0.300954458020331),.UNSPECIFIED.);
#1973=B_SPLINE_CURVE_WITH_KNOTS('',3,(#70709,#70710,#70711,#70712,#70713,
#70714,#70715,#70716,#70717,#70718,#70719,#70720,#70721,#70722,#70723,#70724,
#70725,#70726,#70727,#70728,#70729,#70730,#70731,#70732,#70733,#70734,#70735,
#70736,#70737,#70738,#70739,#70740,#70741,#70742),.UNSPECIFIED.,.T.,.F.,
(4,2,2,2,2,2,2,2,2,2,2,2,2,2,2,2,4),(-0.317382584107991,-0.298404141251476,
-0.278172891490457,-0.257747654398373,-0.237483739094739,-0.217400881549399,
-0.197870634374672,-0.178454632462585,-0.158961383169832,-0.138962436628909,
-0.118826492452815,-0.0985020845516959,-0.0780507441744616,-0.0583017008699032,
-0.0388560211137377,-0.0195122248887286,0.),.UNSPECIFIED.);
#1974=B_SPLINE_CURVE_WITH_KNOTS('',3,(#70748,#70749,#70750,#70751,#70752,
#70753,#70754,#70755,#70756,#70757,#70758,#70759,#70760,#70761,#70762,#70763,
#70764,#70765,#70766,#70767,#70768,#70769,#70770,#70771,#70772,#70773,#70774,
#70775,#70776,#70777,#70778,#70779,#70780,#70781,#70782,#70783,#70784,#70785,
#70786,#70787,#70788,#70789,#70790,#70791,#70792,#70793,#70794,#70795),
 .UNSPECIFIED.,.T.,.F.,(4,2,2,2,2,2,2,2,2,2,2,2,2,2,2,2,2,2,2,2,2,2,2,4),
(0.,0.0282046675723413,0.0672171199264202,0.129041618802007,0.184527661316184,
0.24325253918707,0.304784892317842,0.365588080179233,0.423060617652659,
0.457593113565745,0.47215336749717,0.485219180055195,0.513137775499108,
0.551542455419591,0.613353262192266,0.66846001838336,0.726644630290134,
0.788438287740315,0.849529302645522,0.908974797531781,0.944754831213901,
0.959764451759562,0.967998471593533,0.976310474265571),.UNSPECIFIED.);
#1975=B_SPLINE_CURVE_WITH_KNOTS('',3,(#70807,#70808,#70809,#70810,#70811,
#70812,#70813,#70814,#70815,#70816,#70817,#70818,#70819,#70820,#70821,#70822,
#70823,#70824,#70825,#70826,#70827,#70828,#70829,#70830,#70831,#70832,#70833,
#70834,#70835,#70836,#70837,#70838,#70839,#70840,#70841,#70842,#70843,#70844,
#70845,#70846,#70847,#70848,#70849,#70850,#70851,#70852),.UNSPECIFIED.,
 .T.,.F.,(4,2,2,2,2,2,2,2,2,2,2,2,2,2,2,2,2,2,2,2,2,2,4),(0.,0.0111055104419066,
0.0368929406912385,0.074670643681405,0.125120054145412,0.171409106180065,
0.220390846274497,0.270537305216151,0.319819552908647,0.35954184970516,
0.386169475565741,0.397831092450577,0.408798696086061,0.434213522740755,
0.471993677197715,0.522392420649816,0.568316684839256,0.617007335876734,
0.66731342361697,0.716761752372739,0.755752478614718,0.782476626020418,
0.794702189516223),.UNSPECIFIED.);
#1976=B_SPLINE_CURVE_WITH_KNOTS('',3,(#70862,#70863,#70864,#70865,#70866,
#70867,#70868,#70869,#70870,#70871,#70872,#70873,#70874,#70875,#70876,#70877,
#70878,#70879,#70880,#70881,#70882),.UNSPECIFIED.,.F.,.F.,(4,2,2,2,2,2,
2,2,3,4),(-0.322218774969075,-0.28335234068869,-0.24295415460927,-0.202510991809381,
-0.161749409589793,-0.121051618638299,-0.0807274114131348,-0.0404085956102785,
0.,5.45605715912487E-5),.UNSPECIFIED.);
#1977=B_SPLINE_CURVE_WITH_KNOTS('',3,(#70885,#70886,#70887,#70888,#70889,
#70890,#70891,#70892,#70893,#70894,#70895,#70896,#70897,#70898,#70899,#70900,
#70901,#70902,#70903,#70904,#70905,#70906,#70907,#70908,#70909,#70910,#70911,
#70912,#70913,#70914,#70915,#70916,#70917,#70918,#70919,#70920,#70921,#70922,
#70923,#70924,#70925,#70926,#70927,#70928,#70929,#70930),.UNSPECIFIED.,
 .T.,.F.,(4,2,2,2,2,2,2,2,2,2,2,2,2,2,2,2,2,2,2,2,2,2,4),(0.,0.00873810502121739,
0.0297335652237157,0.0616990112040461,0.0970631346087308,0.134531567849255,
0.174349671243284,0.215481948596841,0.255760444392016,0.290213292281182,
0.312334523108192,0.321849300142609,0.33060135081765,0.350070743937972,
0.378009519424791,0.418839524570214,0.455810185569734,0.495264052732823,
0.536510600809825,0.576903924585634,0.610567503992075,0.632496660166461,
0.646225650111759),.UNSPECIFIED.);
#1978=B_SPLINE_CURVE_WITH_KNOTS('',3,(#70931,#70932,#70933,#70934,#70935,
#70936,#70937,#70938,#70939,#70940,#70941,#70942,#70943,#70944,#70945,#70946,
#70947,#70948,#70949,#70950),.UNSPECIFIED.,.F.,.F.,(4,2,2,2,2,2,2,2,2,4),
(5.45605715912487E-5,0.039878400931096,0.0801684025650735,0.120697106682991,
0.160900180797334,0.201072985262158,0.241099781645388,0.281010189203807,
0.320981648387607,0.322308412283677),.UNSPECIFIED.);
#1979=B_SPLINE_CURVE_WITH_KNOTS('',3,(#70956,#70957,#70958,#70959,#70960,
#70961,#70962,#70963,#70964,#70965,#70966,#70967,#70968,#70969,#70970,#70971,
#70972,#70973,#70974,#70975,#70976,#70977,#70978,#70979,#70980,#70981,#70982,
#70983,#70984,#70985,#70986,#70987,#70988,#70989),.UNSPECIFIED.,.T.,.F.,
(4,2,2,2,2,2,2,2,2,2,2,2,2,2,2,2,4),(-0.315496151749696,-0.297141575074231,
-0.277415457408466,-0.25765681663082,-0.237703025077304,-0.217662758313652,
-0.197739942938581,-0.177848166453009,-0.157949624971573,-0.138056146550069,
-0.118152621681464,-0.0981620045445807,-0.0784580509416342,-0.058779887561761,
-0.039162115708029,-0.0195886853957665,0.),.UNSPECIFIED.);
#1980=B_SPLINE_CURVE_WITH_KNOTS('',3,(#70993,#70994,#70995,#70996,#70997,
#70998,#70999,#71000,#71001,#71002,#71003,#71004,#71005,#71006,#71007,#71008,
#71009,#71010,#71011,#71012,#71013),.UNSPECIFIED.,.F.,.F.,(4,2,2,2,2,2,
2,2,3,4),(-0.300833207677732,-0.264750113783143,-0.226774592484691,-0.187880911782623,
-0.149445134550555,-0.111523025139705,-0.0738351531346529,-0.0368602858553398,
0.,4.89537572855928E-5),.UNSPECIFIED.);
#1981=B_SPLINE_CURVE_WITH_KNOTS('',3,(#71016,#71017,#71018,#71019,#71020,
#71021,#71022,#71023,#71024,#71025,#71026,#71027,#71028,#71029,#71030,#71031,
#71032,#71033,#71034,#71035,#71036,#71037,#71038,#71039,#71040,#71041,#71042,
#71043,#71044,#71045,#71046,#71047,#71048,#71049,#71050,#71051,#71052,#71053,
#71054,#71055,#71056,#71057,#71058,#71059,#71060,#71061,#71062,#71063,#71064,
#71065),.UNSPECIFIED.,.T.,.F.,(4,2,2,2,2,2,2,2,2,2,2,2,2,2,2,2,2,2,2,2,
2,2,2,2,4),(0.,0.0174902552738314,0.0550858062300793,0.0874413426616621,
0.122435820544715,0.160114672538892,0.198542604931461,0.235366820436462,
0.265053282103129,0.280633075883739,0.29213323641515,0.297515032600734,
0.310503863061896,0.331904262314661,0.369614127865018,0.402708235043435,
0.438605222741391,0.477283719499992,0.515058936087459,0.552237125762763,
0.571453983183572,0.583426564445621,0.588721291414423,0.593833968276376,
0.601312691951912),.UNSPECIFIED.);
#1982=B_SPLINE_CURVE_WITH_KNOTS('',3,(#71066,#71067,#71068,#71069,#71070,
#71071,#71072,#71073,#71074,#71075,#71076,#71077,#71078,#71079,#71080,#71081,
#71082,#71083,#71084,#71085),.UNSPECIFIED.,.F.,.F.,(4,2,2,2,2,2,2,2,2,4),
(4.89537572855928E-5,0.0370578863318484,0.0747718108286307,0.112802698338598,
0.151373421073754,0.189198820460287,0.226350822172125,0.263015487542908,
0.299729496728428,0.30092650203114),.UNSPECIFIED.);
#1983=B_SPLINE_CURVE_WITH_KNOTS('',3,(#71091,#71092,#71093,#71094,#71095,
#71096,#71097,#71098,#71099,#71100,#71101,#71102,#71103,#71104,#71105,#71106,
#71107,#71108,#71109,#71110,#71111,#71112,#71113,#71114,#71115,#71116,#71117,
#71118,#71119,#71120,#71121,#71122,#71123,#71124),.UNSPECIFIED.,.T.,.F.,
(4,2,2,2,2,2,2,2,2,2,2,2,2,2,2,2,4),(-0.317346030989117,-0.297995934362178,
-0.277928934514266,-0.25753190568753,-0.237254031147267,-0.217134005118395,
-0.197471893982024,-0.178012846903565,-0.158589272536198,-0.138829010197109,
-0.118785798049446,-0.0986237170224576,-0.0783022451151404,-0.0583630651928147,
-0.0387567340203183,-0.0193856473349845,0.),.UNSPECIFIED.);
#1984=B_SPLINE_CURVE_WITH_KNOTS('',3,(#71130,#71131,#71132,#71133,#71134,
#71135,#71136,#71137,#71138,#71139,#71140,#71141,#71142,#71143,#71144,#71145,
#71146,#71147,#71148,#71149,#71150,#71151,#71152,#71153,#71154,#71155,#71156,
#71157,#71158,#71159,#71160,#71161,#71162,#71163,#71164,#71165,#71166,#71167,
#71168,#71169,#71170,#71171,#71172,#71173,#71174,#71175,#71176,#71177),
 .UNSPECIFIED.,.T.,.F.,(4,2,2,2,2,2,2,2,2,2,2,2,2,2,2,2,2,2,2,2,2,2,2,4),
(0.,0.0228087393460127,0.0549366750067231,0.105316123466778,0.150464710355334,
0.198392767561193,0.248535673308152,0.297889317955252,0.342588836115512,
0.369689349930825,0.38118255907791,0.391575762926861,0.41409606552552,0.445762906742391,
0.49601844873358,0.540990902106172,0.5885466312523,0.639053432053313,0.688811270073417,
0.738067260149195,0.767321634856702,0.778057915095754,0.786088157672185,
0.794230570233434),.UNSPECIFIED.);
#1985=B_SPLINE_CURVE_WITH_KNOTS('',3,(#71187,#71188,#71189,#71190,#71191,
#71192,#71193,#71194,#71195,#71196,#71197,#71198,#71199,#71200,#71201,#71202,
#71203,#71204),.UNSPECIFIED.,.F.,.F.,(4,2,2,2,2,2,2,2,4),(-0.322324642448947,
-0.283170110480757,-0.242893701651131,-0.20248068587249,-0.162079642170941,
-0.121214233737345,-0.0808314172024501,-0.0405092858788416,-5.16185884715199E-5),
 .UNSPECIFIED.);
#1986=B_SPLINE_CURVE_WITH_KNOTS('',3,(#71207,#71208,#71209,#71210,#71211,
#71212,#71213,#71214,#71215,#71216,#71217,#71218,#71219,#71220,#71221,#71222,
#71223,#71224,#71225,#71226,#71227,#71228,#71229,#71230,#71231,#71232,#71233,
#71234,#71235,#71236,#71237,#71238,#71239,#71240,#71241,#71242,#71243,#71244,
#71245,#71246,#71247,#71248,#71249,#71250,#71251,#71252),.UNSPECIFIED.,
 .T.,.F.,(4,2,2,2,2,2,2,2,2,2,2,2,2,2,2,2,2,2,2,2,2,2,4),(0.,0.0199662620991212,
0.0456036708902883,0.0866788818107017,0.123725228190072,0.163049723108265,
0.204263320607153,0.244685065062753,0.282205616781563,0.306135095944507,
0.316400114302969,0.325778046773526,0.346228604908454,0.374648057812432,
0.415526278856,0.452824745585227,0.492421691123166,0.533724430707627,0.574202604793491,
0.609288763055298,0.632836882279711,0.639650492487668,0.646612817989489),
 .UNSPECIFIED.);
#1987=B_SPLINE_CURVE_WITH_KNOTS('',3,(#71253,#71254,#71255,#71256,#71257,
#71258,#71259,#71260,#71261,#71262,#71263,#71264,#71265,#71266,#71267,#71268,
#71269,#71270,#71271,#71272,#71273,#71274,#71275),.UNSPECIFIED.,.F.,.F.,
(4,3,2,2,2,2,2,2,2,2,4),(-5.16185884715199E-5,0.,0.0397076196931033,0.0800974819415304,
0.12040505293073,0.161034734354159,0.201254995785147,0.241394874061776,
0.281378594841956,0.321302725625809,0.322201573923194),.UNSPECIFIED.);
#1988=B_SPLINE_CURVE_WITH_KNOTS('',3,(#71281,#71282,#71283,#71284,#71285,
#71286,#71287,#71288,#71289,#71290,#71291,#71292,#71293,#71294,#71295,#71296,
#71297,#71298,#71299,#71300,#71301,#71302,#71303,#71304,#71305,#71306,#71307,
#71308,#71309,#71310,#71311,#71312,#71313,#71314),.UNSPECIFIED.,.T.,.F.,
(4,2,2,2,2,2,2,2,2,2,2,2,2,2,2,2,4),(-0.315495812936942,-0.297578610010775,
-0.277904381048878,-0.25817151629882,-0.238219344577973,-0.218169621207347,
-0.198238419757734,-0.17832335818959,-0.158361527849011,-0.138384955393027,
-0.11845118141045,-0.0985400198722068,-0.0785529006156278,-0.0588481937293625,
-0.0391823435752262,-0.0195772166611429,0.),.UNSPECIFIED.);
#1989=B_SPLINE_CURVE_WITH_KNOTS('',3,(#71318,#71319,#71320,#71321,#71322,
#71323,#71324,#71325,#71326,#71327,#71328,#71329,#71330,#71331,#71332,#71333,
#71334,#71335,#71336,#71337,#71338),.UNSPECIFIED.,.F.,.F.,(4,2,2,2,2,2,
2,2,3,4),(-0.300885931061383,-0.266181870099638,-0.228550611403087,-0.190322958570215,
-0.151381013671441,-0.112981195344573,-0.0751269286008902,-0.0375398082342578,
0.,1.71168970408003E-6),.UNSPECIFIED.);
#1990=B_SPLINE_CURVE_WITH_KNOTS('',3,(#71341,#71342,#71343,#71344,#71345,
#71346,#71347,#71348,#71349,#71350,#71351,#71352,#71353,#71354,#71355,#71356,
#71357,#71358,#71359,#71360,#71361,#71362,#71363,#71364,#71365,#71366,#71367,
#71368,#71369,#71370,#71371,#71372,#71373,#71374,#71375,#71376,#71377,#71378,
#71379,#71380,#71381,#71382,#71383,#71384),.UNSPECIFIED.,.T.,.F.,(4,2,2,
2,2,2,2,2,2,2,2,2,2,2,2,2,2,2,2,2,2,4),(0.,0.0203990498424528,0.0469460048503852,
0.0848738261531423,0.120105716086176,0.157717798457702,0.196702634118489,
0.234570083384929,0.26706804740395,0.289415373886137,0.299224543866209,
0.308435731691215,0.329423643581651,0.359480802783041,0.392724216440543,
0.428045328293282,0.465901370645603,0.504950277233587,0.542785883592349,
0.572721848192345,0.594147464046836,0.603455879224188),.UNSPECIFIED.);
#1991=B_SPLINE_CURVE_WITH_KNOTS('',3,(#71385,#71386,#71387,#71388,#71389,
#71390,#71391,#71392,#71393,#71394,#71395,#71396,#71397,#71398,#71399,#71400,
#71401,#71402,#71403,#71404),.UNSPECIFIED.,.F.,.F.,(4,2,2,2,2,2,2,2,2,4),
(1.71168970408003E-6,0.03560475636088,0.0732078587183183,0.111112077341659,
0.149581682513832,0.187656524414964,0.225160409956919,0.262020719057387,
0.298624458310984,0.300851400504656),.UNSPECIFIED.);
#1992=B_SPLINE_CURVE_WITH_KNOTS('',3,(#71410,#71411,#71412,#71413,#71414,
#71415,#71416,#71417,#71418,#71419,#71420,#71421,#71422,#71423,#71424,#71425,
#71426,#71427,#71428,#71429,#71430,#71431,#71432,#71433,#71434,#71435,#71436,
#71437,#71438,#71439,#71440,#71441,#71442,#71443),.UNSPECIFIED.,.T.,.F.,
(4,2,2,2,2,2,2,2,2,2,2,2,2,2,2,2,4),(-0.317333830607944,-0.299024107107697,
-0.279222039008183,-0.259023226107041,-0.238552477892511,-0.218235524773687,
-0.198127155821481,-0.178585612581037,-0.15916910395986,-0.139501687049666,
-0.119527020809853,-0.0993901227013666,-0.0790439448424767,-0.0585635571160489,
-0.0387971326001783,-0.0193396977379661,0.),.UNSPECIFIED.);
#1993=B_SPLINE_CURVE_WITH_KNOTS('',3,(#71449,#71450,#71451,#71452,#71453,
#71454,#71455,#71456,#71457,#71458,#71459,#71460,#71461,#71462,#71463,#71464,
#71465,#71466,#71467,#71468,#71469,#71470,#71471,#71472,#71473,#71474,#71475,
#71476,#71477,#71478,#71479,#71480,#71481,#71482,#71483,#71484,#71485,#71486,
#71487,#71488,#71489,#71490,#71491,#71492,#71493,#71494,#71495,#71496,#71497,
#71498),.UNSPECIFIED.,.T.,.F.,(4,2,2,2,2,2,2,2,2,2,2,2,2,2,2,2,2,2,2,2,
2,2,2,2,4),(0.,0.015737764201583,0.0227091894460013,0.0379800462074193,
0.0610465319914851,0.109245059961081,0.151423734853957,0.196523645677437,
0.244746836023321,0.294515239039496,0.343325882195566,0.373646972099584,
0.391245029174184,0.398851690056153,0.40592016688941,0.42227530229542,0.447514818143624,
0.497644663183851,0.54189375504281,0.588933970108545,0.63880092723784,0.688513444191969,
0.736651553710438,0.778315039794088,0.793270637567377),.UNSPECIFIED.);
#1994=B_SPLINE_CURVE_WITH_KNOTS('',3,(#71508,#71509,#71510,#71511,#71512,
#71513,#71514,#71515,#71516,#71517,#71518,#71519,#71520,#71521,#71522,#71523,
#71524,#71525,#71526,#71527,#71528),.UNSPECIFIED.,.F.,.F.,(4,2,2,2,2,2,
2,2,3,4),(-0.322273947232433,-0.283099340074154,-0.242930612661278,-0.202553329014119,
-0.162116370789489,-0.121350728416329,-0.0806718074596314,-0.0403491998561452,
0.,4.9818029130011E-6),.UNSPECIFIED.);
#1995=B_SPLINE_CURVE_WITH_KNOTS('',3,(#71531,#71532,#71533,#71534,#71535,
#71536,#71537,#71538,#71539,#71540,#71541,#71542,#71543,#71544,#71545,#71546,
#71547,#71548,#71549,#71550,#71551,#71552,#71553,#71554,#71555,#71556,#71557,
#71558,#71559,#71560,#71561,#71562,#71563,#71564,#71565,#71566,#71567,#71568,
#71569,#71570,#71571,#71572,#71573,#71574,#71575,#71576,#71577,#71578),
 .UNSPECIFIED.,.T.,.F.,(4,2,2,2,2,2,2,2,2,2,2,2,2,2,2,2,2,2,2,2,2,2,2,4),
(0.,0.00669853431147558,0.012713180910249,0.0259817703783651,0.0457978017341711,
0.0862472748334269,0.121364061808267,0.159062921898553,0.19950502707867,
0.239781234850052,0.279191609031118,0.303790559229149,0.318543386024955,
0.331106263508047,0.345588545654211,0.368909480379511,0.409771179994493,
0.445823314050088,0.48429238576702,0.525273376653319,0.565632394938103,
0.604062186616965,0.630829326260229,0.644914916016497),.UNSPECIFIED.);
#1996=B_SPLINE_CURVE_WITH_KNOTS('',3,(#71579,#71580,#71581,#71582,#71583,
#71584,#71585,#71586,#71587,#71588,#71589,#71590,#71591,#71592,#71593,#71594,
#71595,#71596,#71597,#71598),.UNSPECIFIED.,.F.,.F.,(4,2,2,2,2,2,2,2,2,4),
(4.9818029130011E-6,0.0399314412331601,0.0803482982070822,0.12064699164969,
0.161109119663353,0.201310573704939,0.241498999732639,0.28154854111158,
0.3214703171836,0.322256971972009),.UNSPECIFIED.);
#1997=B_SPLINE_CURVE_WITH_KNOTS('',3,(#71604,#71605,#71606,#71607,#71608,
#71609,#71610,#71611,#71612,#71613,#71614,#71615,#71616,#71617,#71618,#71619,
#71620,#71621,#71622,#71623,#71624,#71625,#71626,#71627,#71628,#71629,#71630,
#71631,#71632,#71633,#71634,#71635,#71636,#71637),.UNSPECIFIED.,.T.,.F.,
(4,2,2,2,2,2,2,2,2,2,2,2,2,2,2,2,4),(-0.315499076058523,-0.2972402057324,
-0.277597963621351,-0.257882336638775,-0.238128502172578,-0.21817417918185,
-0.198149453137237,-0.178227840344242,-0.15831825446875,-0.1383881085649,
-0.118467083477265,-0.0985607662514616,-0.0785988845860134,-0.0588944188066577,
-0.0392078558436279,-0.0195791697313611,0.),.UNSPECIFIED.);
#1998=B_SPLINE_CURVE_WITH_KNOTS('',3,(#71641,#71642,#71643,#71644,#71645,
#71646,#71647,#71648,#71649,#71650,#71651,#71652,#71653,#71654,#71655,#71656,
#71657,#71658),.UNSPECIFIED.,.F.,.F.,(4,2,2,2,2,2,2,2,4),(-0.300918316190137,
-0.265745760462606,-0.228515752189276,-0.190575887865076,-0.151992690861013,
-0.113365511833562,-0.0753078026554617,-0.0376144696996458,-2.55858819131527E-5),
 .UNSPECIFIED.);
#1999=B_SPLINE_CURVE_WITH_KNOTS('',3,(#71661,#71662,#71663,#71664,#71665,
#71666,#71667,#71668,#71669,#71670,#71671,#71672,#71673,#71674,#71675,#71676,
#71677,#71678,#71679,#71680,#71681,#71682,#71683,#71684,#71685,#71686,#71687,
#71688,#71689,#71690,#71691,#71692,#71693,#71694,#71695,#71696,#71697,#71698,
#71699,#71700,#71701,#71702,#71703,#71704,#71705,#71706),.UNSPECIFIED.,
 .T.,.F.,(4,2,2,2,2,2,2,2,2,2,2,2,2,2,2,2,2,2,2,2,2,2,4),(0.,0.00760469797038185,
0.0225312774191947,0.0419560879026201,0.0780731809945311,0.111552300436574,
0.147532803522562,0.185950797597975,0.223692437106523,0.260678361683232,
0.284505934676511,0.300664678877027,0.307944044053357,0.323797732599743,
0.34634348054576,0.384453328157906,0.418674376842058,0.455279169648842,
0.4942078035792,0.531921981089708,0.568780963126567,0.59189655980923,0.602188976422285),
 .UNSPECIFIED.);
#2000=B_SPLINE_CURVE_WITH_KNOTS('',3,(#71707,#71708,#71709,#71710,#71711,
#71712,#71713,#71714,#71715,#71716,#71717,#71718,#71719,#71720,#71721,#71722,
#71723,#71724,#71725,#71726,#71727,#71728,#71729),.UNSPECIFIED.,.F.,.F.,
(4,3,2,2,2,2,2,2,2,2,4),(-2.55858819131527E-5,0.,0.035530362708851,0.0731447096843527,
0.110848045581484,0.148930238186376,0.187583389005476,0.22544323105114,
0.262636684542578,0.299315223853983,0.300828949622202),.UNSPECIFIED.);
#2001=B_SPLINE_CURVE_WITH_KNOTS('',3,(#71735,#71736,#71737,#71738,#71739,
#71740,#71741,#71742,#71743,#71744,#71745,#71746,#71747,#71748,#71749,#71750,
#71751,#71752,#71753,#71754,#71755,#71756,#71757,#71758,#71759,#71760,#71761,
#71762,#71763,#71764,#71765,#71766,#71767,#71768),.UNSPECIFIED.,.T.,.F.,
(4,2,2,2,2,2,2,2,2,2,2,2,2,2,2,2,4),(-0.317339667561293,-0.298795703489905,
-0.279184279507441,-0.259230080396284,-0.238777447832178,-0.218410892308438,
-0.198226466872123,-0.17819786279233,-0.158733004447799,-0.139311936420403,
-0.119571300281915,-0.0995322929494558,-0.0793315274247309,-0.0589518315551108,
-0.0389982306107753,-0.0193762192206639,0.),.UNSPECIFIED.);
#2002=B_SPLINE_CURVE_WITH_KNOTS('',3,(#71772,#71773,#71774,#71775,#71776,
#71777,#71778,#71779,#71780,#71781,#71782,#71783,#71784,#71785,#71786,#71787,
#71788,#71789,#71790,#71791,#71792),.UNSPECIFIED.,.F.,.F.,(4,2,2,2,2,2,
2,2,3,4),(-0.322274258494419,-0.282879524331831,-0.242837204088746,-0.202563596153524,
-0.162140589147018,-0.121726321036062,-0.0807483977258747,-0.0403043194683415,
0.,1.88449534006124E-5),.UNSPECIFIED.);
#2003=B_SPLINE_CURVE_WITH_KNOTS('',3,(#71795,#71796,#71797,#71798,#71799,
#71800,#71801,#71802,#71803,#71804,#71805,#71806,#71807,#71808,#71809,#71810,
#71811,#71812,#71813,#71814,#71815,#71816,#71817,#71818,#71819,#71820,#71821,
#71822,#71823,#71824,#71825,#71826,#71827,#71828,#71829,#71830,#71831,#71832,
#71833,#71834,#71835,#71836,#71837,#71838,#71839,#71840,#71841,#71842,#71843,
#71844,#71845,#71846),.UNSPECIFIED.,.T.,.F.,(4,2,2,2,2,2,2,2,2,2,2,2,2,
2,2,2,2,2,2,2,2,2,2,2,2,4),(0.,0.0269134229306956,0.0409782021484428,0.0467989934801527,
0.0519956902626756,0.0634124484114814,0.0804691074750597,0.117157819874466,
0.151328717625095,0.188057436113526,0.227289028229523,0.267875360744782,
0.307235789391439,0.342887885734985,0.359578238118146,0.370976269015013,
0.376151692845378,0.388053248420623,0.406799989243721,0.44617600536186,
0.481057576445251,0.518571261952553,0.558803877079373,0.59508754338857,
0.616643521243479,0.643958608562694),.UNSPECIFIED.);
#2004=B_SPLINE_CURVE_WITH_KNOTS('',3,(#71847,#71848,#71849,#71850,#71851,
#71852,#71853,#71854,#71855,#71856,#71857,#71858,#71859,#71860,#71861,#71862,
#71863,#71864,#71865,#71866),.UNSPECIFIED.,.F.,.F.,(4,2,2,2,2,2,2,2,2,4),
(1.88449534006124E-5,0.0395684033320943,0.0800690626690298,0.120435494836762,
0.160752649183436,0.201406338324787,0.241624765872817,0.281764951499659,
0.321747064678894,0.322268162535351),.UNSPECIFIED.);
#2005=B_SPLINE_CURVE_WITH_KNOTS('',3,(#71872,#71873,#71874,#71875,#71876,
#71877,#71878,#71879,#71880,#71881,#71882,#71883,#71884,#71885,#71886,#71887,
#71888,#71889,#71890,#71891,#71892,#71893,#71894,#71895,#71896,#71897,#71898,
#71899,#71900,#71901,#71902,#71903,#71904,#71905),.UNSPECIFIED.,.T.,.F.,
(4,2,2,2,2,2,2,2,2,2,2,2,2,2,2,2,4),(-0.315507475062968,-0.297429255241995,
-0.27782589295879,-0.258150653180531,-0.238413338898343,-0.218658308519064,
-0.198562599760213,-0.178604336309516,-0.158695105820558,-0.138763144550359,
-0.118818027328735,-0.0988989879663173,-0.0789817611557068,-0.0589745295578617,
-0.0392695744228467,-0.0196038790058241,0.),.UNSPECIFIED.);
#2006=B_SPLINE_CURVE_WITH_KNOTS('',3,(#71909,#71910,#71911,#71912,#71913,
#71914,#71915,#71916,#71917,#71918,#71919,#71920,#71921,#71922,#71923,#71924,
#71925,#71926),.UNSPECIFIED.,.F.,.F.,(4,2,2,2,2,2,2,2,4),(-0.300983756064892,
-0.265266012119335,-0.228384761090753,-0.190829162479439,-0.152502737010859,
-0.113726790690218,-0.0754803593170012,-0.0376768011524792,-5.89284099797474E-5),
 .UNSPECIFIED.);
#2007=B_SPLINE_CURVE_WITH_KNOTS('',3,(#71929,#71930,#71931,#71932,#71933,
#71934,#71935,#71936,#71937,#71938,#71939,#71940,#71941,#71942,#71943,#71944,
#71945,#71946,#71947,#71948,#71949,#71950,#71951,#71952,#71953,#71954,#71955,
#71956,#71957,#71958,#71959,#71960,#71961,#71962,#71963,#71964,#71965,#71966,
#71967,#71968,#71969,#71970,#71971,#71972,#71973,#71974,#71975,#71976,#71977,
#71978,#71979,#71980,#71981,#71982,#71983,#71984),.UNSPECIFIED.,.T.,.F.,
(4,2,2,2,2,2,2,2,2,2,2,2,2,2,2,2,2,2,2,2,2,2,2,2,2,2,2,4),(0.,0.0195543842904808,
0.027312393989098,0.0324982300196665,0.0348519738504469,0.0403876189278208,
0.0496853599646738,0.082443001531438,0.112274367628169,0.145234456597813,
0.180889844249304,0.219274867422076,0.256429259960666,0.288239963951727,
0.314854389628641,0.324153776360445,0.329896973336055,0.332440267879227,
0.338012281194982,0.34657211619618,0.37067856846271,0.39932757792812,0.431417294726784,
0.466348706046538,0.50396323936281,0.542162628101251,0.565650967054169,
0.599691088329776),.UNSPECIFIED.);
#2008=B_SPLINE_CURVE_WITH_KNOTS('',3,(#71985,#71986,#71987,#71988,#71989,
#71990,#71991,#71992,#71993,#71994,#71995,#71996,#71997,#71998,#71999,#72000,
#72001,#72002,#72003,#72004,#72005,#72006,#72007),.UNSPECIFIED.,.F.,.F.,
(4,3,2,2,2,2,2,2,2,2,4),(-5.89284099797474E-5,0.,0.0356142768925199,0.072932941351032,
0.110609867053781,0.148407439096288,0.186642520710408,0.225409711009659,
0.2629940508189,0.299916704084242,0.300810914179693),.UNSPECIFIED.);
#2009=B_SPLINE_CURVE_WITH_KNOTS('',3,(#72013,#72014,#72015,#72016,#72017,
#72018,#72019,#72020,#72021,#72022,#72023,#72024,#72025,#72026,#72027,#72028,
#72029,#72030,#72031,#72032,#72033,#72034,#72035,#72036,#72037,#72038,#72039,
#72040,#72041,#72042,#72043,#72044,#72045,#72046),.UNSPECIFIED.,.T.,.F.,
(4,2,2,2,2,2,2,2,2,2,2,2,2,2,2,2,4),(-0.317367226772087,-0.29856007747775,
-0.279107507122395,-0.259344623570977,-0.239162101406073,-0.218785432411179,
-0.198555314522819,-0.178473874575583,-0.15889896570101,-0.139474421591269,
-0.120014537391426,-0.100004403392165,-0.0799235976831349,-0.0596943289774754,
-0.0393180790414062,-0.0194978929382608,0.),.UNSPECIFIED.);
#2010=B_SPLINE_CURVE_WITH_KNOTS('',3,(#72050,#72051,#72052,#72053,#72054,
#72055,#72056,#72057,#72058,#72059,#72060,#72061,#72062,#72063,#72064,#72065,
#72066,#72067,#72068,#72069,#72070),.UNSPECIFIED.,.F.,.F.,(4,2,2,2,2,2,
2,2,3,4),(-0.322235936119025,-0.282555513840953,-0.242603866140275,-0.202466099519466,
-0.162118431397947,-0.121692507545716,-0.0809194365641546,-0.0403047888943224,
0.,8.24103542715754E-5),.UNSPECIFIED.);
#2011=B_SPLINE_CURVE_WITH_KNOTS('',3,(#72073,#72074,#72075,#72076,#72077,
#72078,#72079,#72080,#72081,#72082,#72083,#72084,#72085,#72086,#72087,#72088,
#72089,#72090,#72091,#72092,#72093,#72094,#72095,#72096,#72097,#72098,#72099,
#72100,#72101,#72102,#72103,#72104,#72105,#72106,#72107,#72108),
 .UNSPECIFIED.,.T.,.F.,(4,2,2,2,2,2,2,2,2,2,2,2,2,2,2,2,2,4),(0.,0.0399541104210797,
0.0799101633971029,0.120042188031122,0.160349494010668,0.200700062460712,
0.24066914974901,0.281146928548852,0.321688268053878,0.361827692831203,
0.401937446249913,0.441912733333203,0.482224630787991,0.523014478229367,
0.563360237936025,0.603655558777084,0.623959945526864,0.644496878440061),
 .UNSPECIFIED.);
#2012=B_SPLINE_CURVE_WITH_KNOTS('',3,(#72109,#72110,#72111,#72112,#72113,
#72114,#72115,#72116,#72117,#72118,#72119,#72120,#72121,#72122,#72123,#72124,
#72125,#72126,#72127,#72128),.UNSPECIFIED.,.F.,.F.,(4,2,2,2,2,2,2,2,2,4),
(8.24103542715754E-5,0.0391110548112336,0.0796930627605846,0.12022456504364,
0.160555221999647,0.200926013596631,0.241765756700222,0.281979900518358,
0.322064242067825,0.322325169710773),.UNSPECIFIED.);
#2013=B_SPLINE_CURVE_WITH_KNOTS('',3,(#72134,#72135,#72136,#72137,#72138,
#72139,#72140,#72141,#72142,#72143,#72144,#72145,#72146,#72147,#72148,#72149,
#72150,#72151,#72152,#72153,#72154,#72155,#72156,#72157,#72158,#72159,#72160,
#72161,#72162,#72163,#72164,#72165,#72166,#72167),.UNSPECIFIED.,.T.,.F.,
(4,2,2,2,2,2,2,2,2,2,2,2,2,2,2,2,4),(-0.315519596162171,-0.297809213750164,
-0.278229052184091,-0.258601131851469,-0.238901505305988,-0.219155579631688,
-0.19901849790277,-0.179030986117222,-0.15911985913336,-0.139182788191571,
-0.11919620309571,-0.0992213413463237,-0.0793002802766647,-0.0593770243920267,
-0.0393451090122846,-0.0196454507796741,0.),.UNSPECIFIED.);
#2014=B_SPLINE_CURVE_WITH_KNOTS('',3,(#72171,#72172,#72173,#72174,#72175,
#72176,#72177,#72178,#72179,#72180,#72181,#72182,#72183,#72184,#72185,#72186,
#72187,#72188),.UNSPECIFIED.,.F.,.F.,(4,2,2,2,2,2,2,2,4),(-0.300994263979636,
-0.264790681083084,-0.228121553138037,-0.190934646109778,-0.153029416903194,
-0.114459349502728,-0.0758034579641479,-0.0377146753865591,-9.89973092749212E-6),
 .UNSPECIFIED.);
#2015=B_SPLINE_CURVE_WITH_KNOTS('',3,(#72191,#72192,#72193,#72194,#72195,
#72196,#72197,#72198,#72199,#72200,#72201,#72202,#72203,#72204,#72205,#72206,
#72207,#72208,#72209,#72210,#72211,#72212,#72213,#72214,#72215,#72216,#72217,
#72218,#72219,#72220,#72221,#72222,#72223,#72224,#72225,#72226,#72227,#72228,
#72229,#72230,#72231,#72232,#72233,#72234,#72235,#72236,#72237,#72238,#72239,
#72240),.UNSPECIFIED.,.T.,.F.,(4,2,2,2,2,2,2,2,2,2,2,2,2,2,2,2,2,2,2,2,
2,2,2,2,4),(0.,0.0307690129943918,0.0457737289117332,0.0564496066162463,
0.067013357847641,0.0815094903801632,0.112271321654035,0.143533118871858,
0.177384865979269,0.213742800882818,0.251861559810511,0.288869905007967,
0.326261511254301,0.342991018079337,0.354087677704956,0.359080348486155,
0.370267767881213,0.38720643207021,0.422871977549177,0.455142045306466,
0.489970533764269,0.527422511009619,0.559321254860859,0.577641902721842,
0.599527726299083),.UNSPECIFIED.);
#2016=B_SPLINE_CURVE_WITH_KNOTS('',3,(#72241,#72242,#72243,#72244,#72245,
#72246,#72247,#72248,#72249,#72250,#72251,#72252,#72253,#72254,#72255,#72256,
#72257,#72258,#72259,#72260,#72261,#72262,#72263),.UNSPECIFIED.,.F.,.F.,
(4,3,2,2,2,2,2,2,2,2,4),(-9.89973092749212E-6,0.,0.0355811345666444,0.073230471527062,
0.110862998883392,0.148561283179237,0.186608826750277,0.225220645754983,
0.263129936848216,0.300376106774349,0.300875213706327),.UNSPECIFIED.);
#2017=B_SPLINE_CURVE_WITH_KNOTS('',3,(#72269,#72270,#72271,#72272,#72273,
#72274,#72275,#72276,#72277,#72278,#72279,#72280,#72281,#72282,#72283,#72284,
#72285,#72286,#72287,#72288,#72289,#72290,#72291,#72292,#72293,#72294,#72295,
#72296,#72297,#72298,#72299,#72300,#72301,#72302),.UNSPECIFIED.,.T.,.F.,
(4,2,2,2,2,2,2,2,2,2,2,2,2,2,2,2,4),(-0.317410329630175,-0.298796136347515,
-0.279435032432556,-0.259850090267512,-0.239920497281374,-0.219468774491086,
-0.199092484550111,-0.178893042770457,-0.158849925953669,-0.139369604600803,
-0.119951222078813,-0.100224265505886,-0.0801908841414913,-0.0600071079341823,
-0.0396435087199044,-0.0196564465565322,0.),.UNSPECIFIED.);
#2018=B_SPLINE_CURVE_WITH_KNOTS('',3,(#72306,#72307,#72308,#72309,#72310,
#72311,#72312,#72313,#72314,#72315,#72316,#72317,#72318,#72319,#72320,#72321,
#72322,#72323,#72324,#72325,#72326),.UNSPECIFIED.,.F.,.F.,(4,2,2,2,2,2,
2,2,3,4),(-0.322296005070645,-0.282691705710254,-0.242785602353315,-0.202757253805612,
-0.162487760230491,-0.122052055744033,-0.0816187550391033,-0.0405188529317101,
0.,6.19087250895434E-5),.UNSPECIFIED.);
#2019=B_SPLINE_CURVE_WITH_KNOTS('',3,(#72329,#72330,#72331,#72332,#72333,
#72334,#72335,#72336,#72337,#72338,#72339,#72340,#72341,#72342,#72343,#72344,
#72345,#72346,#72347,#72348,#72349,#72350,#72351,#72352,#72353,#72354,#72355,
#72356,#72357,#72358,#72359,#72360,#72361,#72362,#72363,#72364),
 .UNSPECIFIED.,.T.,.F.,(4,2,2,2,2,2,2,2,2,2,2,2,2,2,2,2,2,4),(0.,0.0399541104210688,
0.079910163397041,0.120042188031002,0.160349494010565,0.200700062460793,
0.240669149749168,0.281146928548791,0.321688268053567,0.361827692830774,
0.401937446249555,0.441912733332932,0.482224630787771,0.52301447822922,
0.563360237936112,0.603655558777431,0.623959945527353,0.644496878440584),
 .UNSPECIFIED.);
#2020=B_SPLINE_CURVE_WITH_KNOTS('',3,(#72365,#72366,#72367,#72368,#72369,
#72370,#72371,#72372,#72373,#72374,#72375,#72376,#72377,#72378,#72379,#72380,
#72381,#72382,#72383,#72384),.UNSPECIFIED.,.F.,.F.,(4,2,2,2,2,2,2,2,2,4),
(6.19087250895434E-5,0.0393985606342027,0.0797735668134333,0.120209511040999,
0.160547540179541,0.200870649931096,0.241547367613034,0.281769090282563,
0.321913645565474,0.322291378416777),.UNSPECIFIED.);
#2021=B_SPLINE_CURVE_WITH_KNOTS('',3,(#72390,#72391,#72392,#72393,#72394,
#72395,#72396,#72397,#72398,#72399,#72400,#72401,#72402,#72403,#72404,#72405,
#72406,#72407,#72408,#72409,#72410,#72411,#72412,#72413,#72414,#72415,#72416,
#72417,#72418,#72419,#72420,#72421,#72422,#72423),.UNSPECIFIED.,.T.,.F.,
(4,2,2,2,2,2,2,2,2,2,2,2,2,2,2,2,4),(-0.315533165774014,-0.297436528606874,
-0.277865413070616,-0.258265642221209,-0.238590196427937,-0.218847406594884,
-0.199084884742368,-0.178940376230227,-0.158949603464515,-0.139041131952,
-0.119136887716367,-0.0992245788045587,-0.0793233934924771,-0.0594023812818215,
-0.0393747941743775,-0.0196670977017911,0.),.UNSPECIFIED.);
#2022=B_SPLINE_CURVE_WITH_KNOTS('',3,(#72427,#72428,#72429,#72430,#72431,
#72432,#72433,#72434,#72435,#72436,#72437,#72438,#72439,#72440,#72441,#72442,
#72443,#72444,#72445,#72446,#72447),.UNSPECIFIED.,.F.,.F.,(4,2,2,2,2,2,
2,2,3,4),(-0.30096860817143,-0.264198560924269,-0.227582862782118,-0.19073044092391,
-0.153208886894111,-0.115042102447996,-0.0761891983612259,-0.0378539075755994,
0.,0.000101239354754264),.UNSPECIFIED.);
#2023=B_SPLINE_CURVE_WITH_KNOTS('',3,(#72450,#72451,#72452,#72453,#72454,
#72455,#72456,#72457,#72458,#72459,#72460,#72461,#72462,#72463,#72464,#72465,
#72466,#72467,#72468,#72469,#72470,#72471,#72472,#72473,#72474,#72475,#72476,
#72477,#72478,#72479,#72480,#72481,#72482,#72483,#72484,#72485),
 .UNSPECIFIED.,.T.,.F.,(4,2,2,2,2,2,2,2,2,2,2,2,2,2,2,2,2,4),(0.,0.0355202696275906,
0.0730229242189133,0.109881947977843,0.147332215350788,0.185244244850189,
0.223245130804677,0.259644256143498,0.29483879750671,0.330228485401298,
0.366554345813953,0.404791218290754,0.442165216585822,0.480056587413159,
0.518291371432835,0.552548743061451,0.588529668384299,0.599949959180055),
 .UNSPECIFIED.);
#2024=B_SPLINE_CURVE_WITH_KNOTS('',3,(#72486,#72487,#72488,#72489,#72490,
#72491,#72492,#72493,#72494,#72495,#72496,#72497,#72498,#72499,#72500,#72501,
#72502,#72503,#72504,#72505),.UNSPECIFIED.,.F.,.F.,(4,2,2,2,2,2,2,2,2,4),
(0.000101239354754264,0.036436712581457,0.0733520329498323,0.110663930226565,
0.14833558961367,0.186139232912933,0.224385561227797,0.263172520415901,
0.300809097706522,0.30100062624167),.UNSPECIFIED.);
#2025=B_SPLINE_CURVE_WITH_KNOTS('',3,(#72511,#72512,#72513,#72514,#72515,
#72516,#72517,#72518,#72519,#72520,#72521,#72522,#72523,#72524,#72525,#72526,
#72527,#72528,#72529,#72530,#72531,#72532,#72533,#72534,#72535,#72536,#72537,
#72538,#72539,#72540,#72541,#72542,#72543,#72544),.UNSPECIFIED.,.T.,.F.,
(4,2,2,2,2,2,2,2,2,2,2,2,2,2,2,2,4),(-0.317465401521424,-0.298534881991798,
-0.279185985931209,-0.259748990694432,-0.24000764059935,-0.219844234330012,
-0.199433889771009,-0.179162910845198,-0.159055689337048,-0.13946094284028,
-0.120029518902961,-0.100576113834194,-0.0805716695602433,-0.060486845933592,
-0.0402456000833756,-0.0198516982892401,0.),.UNSPECIFIED.);
#2026=B_SPLINE_CURVE_WITH_KNOTS('',3,(#72548,#72549,#72550,#72551,#72552,
#72553,#72554,#72555,#72556,#72557,#72558,#72559,#72560,#72561,#72562,#72563,
#72564,#72565,#72566,#72567),.UNSPECIFIED.,.F.,.F.,(4,2,2,2,2,2,2,2,2,4),
(-0.32240779513704,-0.322309948170045,-0.282207124514264,-0.242258251398018,
-0.202316548946315,-0.162196977851497,-0.121858894724617,-0.0814269356067834,
-0.0406404219381981,-1.19643287557059E-5),.UNSPECIFIED.);
#2027=B_SPLINE_CURVE_WITH_KNOTS('',3,(#72570,#72571,#72572,#72573,#72574,
#72575,#72576,#72577,#72578,#72579,#72580,#72581,#72582,#72583,#72584,#72585,
#72586,#72587,#72588,#72589,#72590,#72591,#72592,#72593,#72594,#72595,#72596,
#72597,#72598,#72599,#72600,#72601,#72602,#72603,#72604,#72605),
 .UNSPECIFIED.,.T.,.F.,(4,2,2,2,2,2,2,2,2,2,2,2,2,2,2,2,2,4),(0.,0.0399541104211151,
0.0799101633971823,0.120042188031122,0.160349494010512,0.200700062460637,
0.240669149748722,0.281146928548262,0.321688268053098,0.361827692830207,
0.401937446248661,0.441912733331772,0.482224630786321,0.523014478227461,
0.563360237933615,0.603655558774151,0.623959945524341,0.64449687843778),
 .UNSPECIFIED.);
#2028=B_SPLINE_CURVE_WITH_KNOTS('',3,(#72606,#72607,#72608,#72609,#72610,
#72611,#72612,#72613,#72614,#72615,#72616,#72617,#72618,#72619,#72620,#72621,
#72622,#72623,#72624,#72625,#72626),.UNSPECIFIED.,.F.,.F.,(4,3,2,2,2,2,
2,2,2,4),(-1.19643287557059E-5,0.,0.0390447294337543,0.0794373447788432,
0.120030120161568,0.160589432579093,0.200937759073155,0.241289481748733,
0.282079104740989,0.322210485893345),.UNSPECIFIED.);
#2029=B_SPLINE_CURVE_WITH_KNOTS('',3,(#72632,#72633,#72634,#72635,#72636,
#72637,#72638,#72639,#72640,#72641,#72642,#72643,#72644,#72645,#72646,#72647,
#72648,#72649,#72650,#72651,#72652,#72653,#72654,#72655,#72656,#72657,#72658,
#72659,#72660,#72661,#72662,#72663,#72664,#72665),.UNSPECIFIED.,.T.,.F.,
(4,2,2,2,2,2,2,2,2,2,2,2,2,2,2,2,4),(-0.315548571684421,-0.297773351174838,
-0.278176003062129,-0.258598189537295,-0.238976726468293,-0.219281852001301,
-0.199535221016545,-0.179391819962517,-0.159399197996224,-0.139486889367128,
-0.11954902226534,-0.0995560164366063,-0.0795697129165012,-0.059641377251603,
-0.0397234123798072,-0.0197072139785503,0.),.UNSPECIFIED.);
#2030=B_SPLINE_CURVE_WITH_KNOTS('',3,(#72669,#72670,#72671,#72672,#72673,
#72674,#72675,#72676,#72677,#72678,#72679,#72680,#72681,#72682,#72683,#72684,
#72685,#72686,#72687,#72688,#72689,#72690,#72691),.UNSPECIFIED.,.F.,.F.,
(4,2,2,2,2,2,2,2,2,3,4),(-0.301044807969637,-0.301018227949179,-0.263705218785146,
-0.226969493307541,-0.190315888874966,-0.153176105293676,-0.115309971137163,
-0.0767479418711244,-0.0380966018702412,0.,0.000121343267829525),
 .UNSPECIFIED.);
#2031=B_SPLINE_CURVE_WITH_KNOTS('',3,(#72694,#72695,#72696,#72697,#72698,
#72699,#72700,#72701,#72702,#72703,#72704,#72705,#72706,#72707,#72708,#72709,
#72710,#72711,#72712,#72713,#72714,#72715,#72716,#72717,#72718,#72719,#72720,
#72721,#72722,#72723,#72724,#72725,#72726,#72727,#72728,#72729),
 .UNSPECIFIED.,.T.,.F.,(4,2,2,2,2,2,2,2,2,2,2,2,2,2,2,2,2,4),(0.,0.035520269627724,
0.0730229242195072,0.109881947979195,0.147332215353038,0.185244244853688,
0.223245130809801,0.259644256150227,0.294838797515063,0.330228485411425,
0.366554345826138,0.404791218305404,0.442165216602898,0.480056587432884,
0.518291371455665,0.55254874308709,0.588529668413202,0.599949959209379),
 .UNSPECIFIED.);
#2032=B_SPLINE_CURVE_WITH_KNOTS('',3,(#72730,#72731,#72732,#72733,#72734,
#72735,#72736,#72737,#72738,#72739,#72740,#72741,#72742,#72743,#72744,#72745,
#72746,#72747),.UNSPECIFIED.,.F.,.F.,(4,2,2,2,2,2,2,2,4),(0.000121343267829525,
0.0366203311667738,0.0742978920120693,0.111163641608319,0.148850930352528,
0.186555371217545,0.224549916816768,0.263085201813925,0.301031791575559),
 .UNSPECIFIED.);
#2033=B_SPLINE_CURVE_WITH_KNOTS('',3,(#72753,#72754,#72755,#72756,#72757,
#72758,#72759,#72760,#72761,#72762,#72763,#72764,#72765,#72766,#72767,#72768,
#72769,#72770,#72771,#72772,#72773,#72774,#72775,#72776,#72777,#72778,#72779,
#72780,#72781,#72782,#72783,#72784,#72785,#72786),.UNSPECIFIED.,.T.,.F.,
(4,2,2,2,2,2,2,2,2,2,2,2,2,2,2,2,4),(-0.317520789214244,-0.298884746791165,
-0.279463280388508,-0.260109693987934,-0.240554297200441,-0.220653647372428,
-0.200213118904547,-0.179844668128175,-0.159642952730947,-0.139584427087022,
-0.120082689424148,-0.100665871473826,-0.0809522571001296,-0.0609189321719877,
-0.0407632761903409,-0.0204362576967705,0.),.UNSPECIFIED.);
#2034=B_SPLINE_CURVE_WITH_KNOTS('',3,(#72790,#72791,#72792,#72793,#72794,
#72795,#72796,#72797,#72798,#72799,#72800,#72801,#72802,#72803,#72804,#72805,
#72806,#72807,#72808,#72809,#72810,#72811,#72812),.UNSPECIFIED.,.F.,.F.,
(4,2,2,2,2,2,2,2,2,3,4),(-0.322425076967677,-0.32231349089565,-0.282145629075095,
-0.242145113385566,-0.202238999895162,-0.162228469192213,-0.121978668171416,
-0.0815481694877585,-0.0411040729638831,0.,7.74523776212593E-6),
 .UNSPECIFIED.);
#2035=B_SPLINE_CURVE_WITH_KNOTS('',3,(#72815,#72816,#72817,#72818,#72819,
#72820,#72821,#72822,#72823,#72824,#72825,#72826,#72827,#72828,#72829,#72830,
#72831,#72832,#72833,#72834,#72835,#72836,#72837,#72838,#72839,#72840,#72841,
#72842,#72843,#72844,#72845,#72846,#72847,#72848,#72849,#72850),
 .UNSPECIFIED.,.T.,.F.,(4,2,2,2,2,2,2,2,2,2,2,2,2,2,2,2,2,4),(0.,0.0399541104210824,
0.0799101633971159,0.120042188031233,0.160349494011014,0.200700062461302,
0.240669149749529,0.281146928549236,0.321688268054275,0.361827692831736,
0.401937446250701,0.441912733334188,0.482224630789035,0.523014478230616,
0.56336023793752,0.603655558779058,0.623959945529218,0.644496878442553),
 .UNSPECIFIED.);
#2036=B_SPLINE_CURVE_WITH_KNOTS('',3,(#72851,#72852,#72853,#72854,#72855,
#72856,#72857,#72858,#72859,#72860,#72861,#72862,#72863,#72864,#72865,#72866,
#72867,#72868),.UNSPECIFIED.,.F.,.F.,(4,2,2,2,2,2,2,2,4),(7.74523776212593E-6,
0.0396065933934371,0.0799124406986436,0.120313242028674,0.160793977016685,
0.201168607760791,0.24148430748624,0.282102424584037,0.322225812953619),
 .UNSPECIFIED.);
#2037=B_SPLINE_CURVE_WITH_KNOTS('',3,(#72874,#72875,#72876,#72877,#72878,
#72879,#72880,#72881,#72882,#72883,#72884,#72885,#72886,#72887,#72888,#72889,
#72890,#72891,#72892,#72893,#72894,#72895,#72896,#72897,#72898,#72899,#72900,
#72901,#72902,#72903,#72904,#72905,#72906,#72907),.UNSPECIFIED.,.T.,.F.,
(4,2,2,2,2,2,2,2,2,2,2,2,2,2,2,2,4),(-0.315562181390567,-0.297399338673171,
-0.277783079139259,-0.258210583754242,-0.238617327429595,-0.218950639127311,
-0.19921201502306,-0.179446456268321,-0.159308096556667,-0.139319421594417,
-0.119405860207257,-0.0994866391650725,-0.0795530415751003,-0.0596365801854092,
-0.0397191192000682,-0.0197147983578177,0.),.UNSPECIFIED.);
#2038=B_SPLINE_CURVE_WITH_KNOTS('',3,(#72911,#72912,#72913,#72914,#72915,
#72916,#72917,#72918,#72919,#72920,#72921,#72922,#72923,#72924,#72925,#72926,
#72927,#72928,#72929,#72930,#72931),.UNSPECIFIED.,.F.,.F.,(4,2,2,2,2,2,
2,2,3,4),(-0.301143817833422,-0.263550055241862,-0.226554857552283,-0.189938047509704,
-0.153112323520037,-0.115617591452942,-0.0774492295109371,-0.0384767409856328,
0.,0.000115639545563484),.UNSPECIFIED.);
#2039=B_SPLINE_CURVE_WITH_KNOTS('',3,(#72934,#72935,#72936,#72937,#72938,
#72939,#72940,#72941,#72942,#72943,#72944,#72945,#72946,#72947,#72948,#72949,
#72950,#72951,#72952,#72953,#72954,#72955,#72956,#72957,#72958,#72959,#72960,
#72961,#72962,#72963,#72964,#72965,#72966,#72967,#72968,#72969),
 .UNSPECIFIED.,.T.,.F.,(4,2,2,2,2,2,2,2,2,2,2,2,2,2,2,2,2,4),(0.,0.0355202696276797,
0.0730229242192678,0.109881947978633,0.147332215352278,0.185244244852624,
0.223245130807942,0.259644256147764,0.294838797512181,0.330228485408057,
0.366554345822135,0.404791218300789,0.442165216597746,0.480056587427034,
0.518291371449068,0.552548743079712,0.588529668404829,0.599949959200832),
 .UNSPECIFIED.);
#2040=B_SPLINE_CURVE_WITH_KNOTS('',3,(#72970,#72971,#72972,#72973,#72974,
#72975,#72976,#72977,#72978,#72979,#72980,#72981,#72982,#72983,#72984,#72985,
#72986,#72987,#72988,#72989),.UNSPECIFIED.,.F.,.F.,(4,2,2,2,2,2,2,2,2,4),
(0.000115639545563484,0.0353759396023698,0.0730488697140438,0.110680865125456,
0.14831820650525,0.185958002516291,0.223780919085869,0.262084290340789,
0.300943211829805,0.301033737001698),.UNSPECIFIED.);
#2041=B_SPLINE_CURVE_WITH_KNOTS('',3,(#72995,#72996,#72997,#72998,#72999,
#73000,#73001,#73002,#73003,#73004,#73005,#73006,#73007,#73008,#73009,#73010,
#73011,#73012,#73013,#73014,#73015,#73016,#73017,#73018,#73019,#73020,#73021,
#73022,#73023,#73024,#73025,#73026,#73027,#73028),.UNSPECIFIED.,.T.,.F.,
(4,2,2,2,2,2,2,2,2,2,2,2,2,2,2,2,4),(-0.317575567098843,-0.298445182096447,
-0.278896806076191,-0.259545627203428,-0.240120965983672,-0.220394138326682,
-0.200247246637959,-0.179781459930513,-0.159442591673954,-0.13929341444518,
-0.11968545437467,-0.100250205219309,-0.080800551891539,-0.0608164077051777,
-0.0407200069083776,-0.020440667324873,0.),.UNSPECIFIED.);
#2042=B_SPLINE_CURVE_WITH_KNOTS('',3,(#73032,#73033,#73034,#73035,#73036,
#73037,#73038,#73039,#73040,#73041,#73042,#73043,#73044,#73045,#73046,#73047,
#73048,#73049,#73050,#73051,#73052,#73053,#73054),.UNSPECIFIED.,.F.,.F.,
(4,2,2,2,2,2,2,2,2,3,4),(-0.301177822624064,-0.30086554318467,-0.262823177269621,
-0.225437092346638,-0.188664030260345,-0.152025487199693,-0.114937899685909,
-0.0771209266757964,-0.0385646913814458,0.,0.000147036074768649),
 .UNSPECIFIED.);
#2043=B_SPLINE_CURVE_WITH_KNOTS('',3,(#73057,#73058,#73059,#73060,#73061,
#73062,#73063,#73064,#73065,#73066,#73067,#73068,#73069,#73070,#73071,#73072,
#73073,#73074,#73075,#73076,#73077,#73078,#73079,#73080,#73081,#73082,#73083,
#73084,#73085,#73086,#73087,#73088,#73089,#73090,#73091,#73092),
 .UNSPECIFIED.,.T.,.F.,(4,2,2,2,2,2,2,2,2,2,2,2,2,2,2,2,2,4),(0.,0.0355202696277128,
0.0730229242193518,0.109881947978684,0.147332215352392,0.185244244852654,
0.223245130808227,0.259644256148146,0.294838797512514,0.330228485408397,
0.366554345822571,0.404791218301228,0.442165216598115,0.480056587427485,
0.518291371449575,0.552548743080241,0.588529668405412,0.599949959201459),
 .UNSPECIFIED.);
#2044=B_SPLINE_CURVE_WITH_KNOTS('',3,(#73093,#73094,#73095,#73096,#73097,
#73098,#73099,#73100,#73101,#73102,#73103,#73104,#73105,#73106,#73107,#73108,
#73109,#73110,#73111,#73112),.UNSPECIFIED.,.F.,.F.,(4,2,2,2,2,2,2,2,2,4),
(0.000147036074768649,0.0002632003303773,0.0382957067158387,0.076039995313587,
0.11311569401633,0.149980240799155,0.1873806962898,0.225106586749685,0.26300984239388,
0.301085178106991),.UNSPECIFIED.);
#2045=B_SPLINE_CURVE_WITH_KNOTS('',3,(#73118,#73119,#73120,#73121,#73122,
#73123,#73124,#73125,#73126,#73127,#73128,#73129,#73130,#73131,#73132,#73133,
#73134,#73135,#73136,#73137,#73138,#73139,#73140,#73141,#73142,#73143,#73144,
#73145,#73146,#73147,#73148,#73149,#73150,#73151),.UNSPECIFIED.,.T.,.F.,
(4,2,2,2,2,2,2,2,2,2,2,2,2,2,2,2,4),(-0.317617838667146,-0.297749119122409,
-0.27801232301177,-0.25857847777276,-0.239227863669495,-0.219685791919498,
-0.199797683321152,-0.179390605497121,-0.159080534568315,-0.138922841472281,
-0.118864173739561,-0.0993487487947275,-0.0799339791397019,-0.0604183948867128,
-0.0403723235572229,-0.0202583353081762,0.),.UNSPECIFIED.);
#2046=B_SPLINE_CURVE_WITH_KNOTS('',3,(#73155,#73156,#73157,#73158,#73159,
#73160,#73161,#73162,#73163,#73164,#73165,#73166,#73167,#73168,#73169,#73170,
#73171,#73172,#73173,#73174,#73175,#73176,#73177),.UNSPECIFIED.,.F.,.F.,
(4,2,2,2,2,2,2,2,2,3,4),(-0.322386353128523,-0.321924747431815,-0.281676040704693,
-0.241548845237877,-0.201587824271888,-0.16165494878838,-0.121556749590579,
-0.081233967950947,-0.0408003840156776,0.,6.67458284606265E-5),
 .UNSPECIFIED.);
#2047=B_SPLINE_CURVE_WITH_KNOTS('',3,(#73180,#73181,#73182,#73183,#73184,
#73185,#73186,#73187,#73188,#73189,#73190,#73191,#73192,#73193,#73194,#73195,
#73196,#73197,#73198,#73199,#73200,#73201,#73202,#73203,#73204,#73205,#73206,
#73207,#73208,#73209,#73210,#73211,#73212,#73213,#73214,#73215),
 .UNSPECIFIED.,.T.,.F.,(4,2,2,2,2,2,2,2,2,2,2,2,2,2,2,2,2,4),(0.,0.0399541104211141,
0.0799101633971717,0.120042188031049,0.160349494010557,0.200700062460784,
0.240669149748917,0.281146928548468,0.321688268053327,0.361827692830636,
0.401937446249474,0.441912733332744,0.482224630787451,0.523014478229153,
0.56336023793604,0.603655558777477,0.623959945527602,0.644496878440942),
 .UNSPECIFIED.);
#2048=B_SPLINE_CURVE_WITH_KNOTS('',3,(#73216,#73217,#73218,#73219,#73220,
#73221,#73222,#73223,#73224,#73225,#73226,#73227,#73228,#73229,#73230,#73231,
#73232,#73233),.UNSPECIFIED.,.F.,.F.,(4,2,2,2,2,2,2,2,4),(6.67458284606265E-5,
0.0393826488471203,0.0796914813289635,0.120093624542018,0.160725370013617,
0.201339688030563,0.24171722174321,0.282040571557513,0.322293513905308),
 .UNSPECIFIED.);
#2049=B_SPLINE_CURVE_WITH_KNOTS('',3,(#73239,#73240,#73241,#73242,#73243,
#73244,#73245,#73246,#73247,#73248,#73249,#73250,#73251,#73252,#73253,#73254,
#73255,#73256,#73257,#73258,#73259,#73260,#73261,#73262,#73263,#73264,#73265,
#73266,#73267,#73268,#73269,#73270,#73271,#73272),.UNSPECIFIED.,.T.,.F.,
(4,2,2,2,2,2,2,2,2,2,2,2,2,2,2,2,4),(-0.315575068397107,-0.297725501979271,
-0.278054313638465,-0.258450452345541,-0.238874557421568,-0.219261153221667,
-0.199573893731351,-0.179829007564642,-0.159694178352794,-0.139711485464633,
-0.119804488965712,-0.0998605425660636,-0.0798476482302862,-0.0598364031986145,
-0.0398950310581945,-0.0199874120120488,0.),.UNSPECIFIED.);
#2050=B_SPLINE_CURVE_WITH_KNOTS('',3,(#73375,#73376,#73377,#73378,#73379,
#73380,#73381,#73382,#73383,#73384,#73385,#73386,#73387,#73388,#73389,#73390,
#73391,#73392,#73393,#73394,#73395,#73396,#73397,#73398,#73399),
 .UNSPECIFIED.,.F.,.F.,(4,2,2,2,3,2,2,2,2,2,2,4),(-0.163168148872215,-0.149527097306421,
-0.099418871001962,-0.0495338134349146,0.,0.0181167695460887,0.0672138706813057,
0.116111680955948,0.165495495020991,0.211936470057348,0.257662170504295,
0.287380385163945),.UNSPECIFIED.);
#2051=B_SPLINE_CURVE_WITH_KNOTS('',3,(#73402,#73403,#73404,#73405,#73406,
#73407,#73408,#73409),.UNSPECIFIED.,.F.,.F.,(4,2,2,4),(-0.287435863143152,
-0.242415728675084,-0.196766145639793,-0.163168148872215),.UNSPECIFIED.);
#2052=B_SPLINE_CURVE_WITH_KNOTS('',3,(#73518,#73519,#73520,#73521,#73522,
#73523,#73524,#73525,#73526,#73527,#73528,#73529,#73530,#73531,#73532,#73533,
#73534,#73535,#73536,#73537,#73538,#73539,#73540),.UNSPECIFIED.,.F.,.F.,
(4,2,2,3,2,2,2,2,2,2,4),(-0.136734216111625,-0.0994188710018493,-0.0495338134348796,
0.,0.0181167695462525,0.0672138706826966,0.11611168095846,0.165495495024581,
0.211936470061975,0.257662170509725,0.287380385169817),.UNSPECIFIED.);
#2053=B_SPLINE_CURVE_WITH_KNOTS('',3,(#73543,#73544,#73545,#73546,#73547,
#73548,#73549,#73550,#73551,#73552),.UNSPECIFIED.,.F.,.F.,(4,2,2,2,4),(-0.287435863144066,
-0.242415728675624,-0.196766145640031,-0.149527097306449,-0.136734216111625),
 .UNSPECIFIED.);
#2054=B_SPLINE_CURVE_WITH_KNOTS('',3,(#73649,#73650,#73651,#73652,#73653,
#73654,#73655,#73656,#73657,#73658,#73659,#73660,#73661,#73662,#73663,#73664,
#73665,#73666,#73667,#73668,#73669,#73670,#73671),.UNSPECIFIED.,.F.,.F.,
(4,2,2,3,2,2,2,2,2,2,4),(-0.110237651798014,-0.0994188710015688,-0.0495338134348444,
0.,0.018116769546061,0.0672138706809179,0.116111680955262,0.165495495019963,
0.21193647005629,0.257662170503162,0.287380385162707),.UNSPECIFIED.);
#2055=B_SPLINE_CURVE_WITH_KNOTS('',3,(#73674,#73675,#73676,#73677,#73678,
#73679,#73680,#73681,#73682,#73683),.UNSPECIFIED.,.F.,.F.,(4,2,2,2,4),(-0.287435863141549,
-0.242415728673738,-0.196766145638641,-0.149527097305494,-0.110237651798014),
 .UNSPECIFIED.);
#2056=B_SPLINE_CURVE_WITH_KNOTS('',3,(#73792,#73793,#73794,#73795,#73796,
#73797,#73798,#73799,#73800,#73801,#73802,#73803,#73804,#73805,#73806,#73807,
#73808,#73809,#73810,#73811,#73812),.UNSPECIFIED.,.F.,.F.,(4,2,3,2,2,2,
2,2,2,4),(-0.0838008711994917,-0.0495338134349723,0.,0.0181167695463933,
0.0672138706835067,0.116111680959761,0.165495495026224,0.211936470064241,
0.25766217051282,0.287380385173364),.UNSPECIFIED.);
#2057=B_SPLINE_CURVE_WITH_KNOTS('',3,(#73815,#73816,#73817,#73818,#73819,
#73820,#73821,#73822,#73823,#73824,#73825,#73826),.UNSPECIFIED.,.F.,.F.,
(4,2,2,2,2,4),(-0.28743586314397,-0.242415728675305,-0.196766145639633,
-0.149527097306083,-0.0994188710019063,-0.0838008711994917),
 .UNSPECIFIED.);
#2058=B_SPLINE_CURVE_WITH_KNOTS('',3,(#73935,#73936,#73937,#73938,#73939,
#73940,#73941,#73942,#73943,#73944,#73945,#73946,#73947,#73948,#73949,#73950,
#73951,#73952,#73953,#73954,#73955),.UNSPECIFIED.,.F.,.F.,(4,2,3,2,2,2,
2,2,2,4),(-0.0573096617767208,-0.0495338134349582,0.,0.0181167695464065,
0.067213870683422,0.11611168095957,0.165495495026031,0.211936470063854,
0.257662170511938,0.287380385172065),.UNSPECIFIED.);
#2059=B_SPLINE_CURVE_WITH_KNOTS('',3,(#73958,#73959,#73960,#73961,#73962,
#73963,#73964,#73965,#73966,#73967,#73968,#73969),.UNSPECIFIED.,.F.,.F.,
(4,2,2,2,2,4),(-0.287435863144792,-0.24241572867618,-0.196766145640472,
-0.149527097306765,-0.0994188710021029,-0.0573096617767208),
 .UNSPECIFIED.);
#2060=B_SPLINE_CURVE_WITH_KNOTS('',3,(#74078,#74079,#74080,#74081,#74082,
#74083,#74084,#74085,#74086,#74087,#74088,#74089,#74090,#74091,#74092,#74093,
#74094,#74095,#74096),.UNSPECIFIED.,.F.,.F.,(4,3,2,2,2,2,2,2,4),(-0.030871330269263,
0.,0.0181167695458699,0.0672138706791213,0.116111680952223,0.165495495015657,
0.211936470050785,0.257662170496474,0.287380385155237),.UNSPECIFIED.);
#2061=B_SPLINE_CURVE_WITH_KNOTS('',3,(#74099,#74100,#74101,#74102,#74103,
#74104,#74105,#74106,#74107,#74108,#74109,#74110,#74111,#74112),
 .UNSPECIFIED.,.F.,.F.,(4,2,2,2,2,2,4),(-0.287435863140128,-0.242415728672749,
-0.196766145638088,-0.149527097305286,-0.0994188710013708,-0.0495338134347677,
-0.030871330269263),.UNSPECIFIED.);
#2062=B_SPLINE_CURVE_WITH_KNOTS('',3,(#74221,#74222,#74223,#74224,#74225,
#74226,#74227,#74228,#74229,#74230,#74231,#74232,#74233,#74234,#74235,#74236,
#74237,#74238,#74239),.UNSPECIFIED.,.F.,.F.,(4,3,2,2,2,2,2,2,4),(-0.0043909955767957,
0.,0.0181167695464896,0.0672138706846621,0.116111680961959,0.165495495029324,
0.211936470068035,0.257662170516974,0.287380385177773),.UNSPECIFIED.);
#2063=B_SPLINE_CURVE_WITH_KNOTS('',3,(#74242,#74243,#74244,#74245,#74246,
#74247,#74248,#74249,#74250,#74251,#74252,#74253,#74254,#74255),
 .UNSPECIFIED.,.F.,.F.,(4,2,2,2,2,2,4),(-0.287435863146267,-0.242415728677103,
-0.196766145640964,-0.149527097306892,-0.0994188710022298,-0.0495338134350148,
-0.0043909955767957),.UNSPECIFIED.);
#2064=B_SPLINE_CURVE_WITH_KNOTS('',3,(#74352,#74353,#74354,#74355,#74356,
#74357,#74358,#74359,#74360,#74361,#74362,#74363,#74364,#74365),
 .UNSPECIFIED.,.F.,.F.,(4,2,2,2,2,2,4),(0.0219992412523513,0.0672138706833701,
0.116111680959517,0.165495495025897,0.211936470063604,0.257662170511581,
0.287380385171759),.UNSPECIFIED.);
#2065=B_SPLINE_CURVE_WITH_KNOTS('',3,(#74368,#74369,#74370,#74371,#74372,
#74373,#74374,#74375,#74376,#74377,#74378,#74379,#74380,#74381,#74382,#74383,
#74384,#74385,#74386),.UNSPECIFIED.,.F.,.F.,(4,2,2,2,2,2,3,2,4),(-0.287435863143863,
-0.242415728675397,-0.196766145639793,-0.149527097306269,-0.0994188710018298,
-0.0495338134348875,0.,0.0181167695463815,0.0219992412523513),
 .UNSPECIFIED.);
#2066=B_SPLINE_CURVE_WITH_KNOTS('',3,(#74495,#74496,#74497,#74498,#74499,
#74500,#74501,#74502,#74503,#74504,#74505,#74506,#74507,#74508),
 .UNSPECIFIED.,.F.,.F.,(4,2,2,2,2,2,4),(0.0484769366691737,0.0672138706802703,
0.116111680953911,0.165495495018043,0.211936470053924,0.2576621705003,0.287380385159541),
 .UNSPECIFIED.);
#2067=B_SPLINE_CURVE_WITH_KNOTS('',3,(#74511,#74512,#74513,#74514,#74515,
#74516,#74517,#74518,#74519,#74520,#74521,#74522,#74523,#74524,#74525,#74526,
#74527,#74528,#74529),.UNSPECIFIED.,.F.,.F.,(4,2,2,2,2,2,3,2,4),(-0.28743586314069,
-0.242415728673121,-0.196766145638307,-0.149527097305332,-0.0994188710013639,
-0.0495338134347652,0.,0.0181167695459964,0.0484769366691737),
 .UNSPECIFIED.);
#2068=B_SPLINE_CURVE_WITH_KNOTS('',3,(#74638,#74639,#74640,#74641,#74642,
#74643,#74644,#74645,#74646,#74647,#74648,#74649),.UNSPECIFIED.,.F.,.F.,
(4,2,2,2,2,4),(0.074915383377095,0.116111680950963,0.165495495013905,0.211936470048695,
0.257662170494074,0.287380385152742),.UNSPECIFIED.);
#2069=B_SPLINE_CURVE_WITH_KNOTS('',3,(#74652,#74653,#74654,#74655,#74656,
#74657,#74658,#74659,#74660,#74661,#74662,#74663,#74664,#74665,#74666,#74667,
#74668,#74669,#74670,#74671,#74672),.UNSPECIFIED.,.F.,.F.,(4,2,2,2,2,2,
3,2,2,4),(-0.287435863139544,-0.242415728672318,-0.196766145637718,-0.149527097305004,
-0.099418871001249,-0.0495338134347465,0.,0.0181167695457953,0.067213870678527,
0.074915383377095),.UNSPECIFIED.);
#2070=B_SPLINE_CURVE_WITH_KNOTS('',3,(#74781,#74782,#74783,#74784,#74785,
#74786,#74787,#74788,#74789,#74790,#74791,#74792),.UNSPECIFIED.,.F.,.F.,
(4,2,2,2,2,4),(0.101402925040076,0.116111680956364,0.165495495021304,0.211936470057817,
0.257662170504839,0.287380385164579),.UNSPECIFIED.);
#2071=B_SPLINE_CURVE_WITH_KNOTS('',3,(#74795,#74796,#74797,#74798,#74799,
#74800,#74801,#74802,#74803,#74804,#74805,#74806,#74807,#74808,#74809,#74810,
#74811,#74812,#74813,#74814,#74815),.UNSPECIFIED.,.F.,.F.,(4,2,2,2,2,2,
3,2,2,4),(-0.28743586314205,-0.242415728673942,-0.196766145638722,-0.14952709730564,
-0.0994188710015697,-0.0495338134348303,0.,0.0181167695460824,0.0672138706815053,
0.101402925040076),.UNSPECIFIED.);
#2072=B_SPLINE_CURVE_WITH_KNOTS('',3,(#74924,#74925,#74926,#74927,#74928,
#74929,#74930,#74931,#74932,#74933),.UNSPECIFIED.,.F.,.F.,(4,2,2,2,4),(0.127838203298608,
0.165495495016154,0.211936470051326,0.257662170497038,0.287380385156003),
 .UNSPECIFIED.);
#2073=B_SPLINE_CURVE_WITH_KNOTS('',3,(#74936,#74937,#74938,#74939,#74940,
#74941,#74942,#74943,#74944,#74945,#74946,#74947,#74948,#74949,#74950,#74951,
#74952,#74953,#74954,#74955,#74956,#74957,#74958),.UNSPECIFIED.,.F.,.F.,
(4,2,2,2,2,2,3,2,2,2,4),(-0.287435863140559,-0.242415728672966,-0.196766145638107,
-0.149527097305205,-0.0994188710012938,-0.0495338134347454,0.,0.0181167695458621,
0.0672138706792296,0.116111680952409,0.127838203298608),.UNSPECIFIED.);
#2074=B_SPLINE_CURVE_WITH_KNOTS('',3,(#75055,#75056,#75057,#75058,#75059,
#75060,#75061,#75062,#75063,#75064),.UNSPECIFIED.,.F.,.F.,(4,2,2,2,4),(0.154331148598444,
0.165495495019413,0.211936470055537,0.257662170502203,0.287380385161736),
 .UNSPECIFIED.);
#2075=B_SPLINE_CURVE_WITH_KNOTS('',3,(#75067,#75068,#75069,#75070,#75071,
#75072,#75073,#75074,#75075,#75076,#75077,#75078,#75079,#75080,#75081,#75082,
#75083,#75084,#75085,#75086,#75087,#75088,#75089),.UNSPECIFIED.,.F.,.F.,
(4,2,2,2,2,2,3,2,2,2,4),(-0.2874358631423,-0.242415728674201,-0.196766145638911,
-0.149527097305732,-0.0994188710014949,-0.0495338134347817,0.,0.018116769546075,
0.0672138706808332,0.116111680954877,0.154331148598444),.UNSPECIFIED.);
#2076=B_SPLINE_CURVE_WITH_KNOTS('',3,(#75198,#75199,#75200,#75201,#75202,
#75203,#75204,#75205),.UNSPECIFIED.,.F.,.F.,(4,2,2,4),(0.180763661414687,
0.211936470057055,0.257662170504015,0.287380385163549),.UNSPECIFIED.);
#2077=B_SPLINE_CURVE_WITH_KNOTS('',3,(#75208,#75209,#75210,#75211,#75212,
#75213,#75214,#75215,#75216,#75217,#75218,#75219,#75220,#75221,#75222,#75223,
#75224,#75225,#75226,#75227,#75228,#75229,#75230,#75231,#75232),
 .UNSPECIFIED.,.F.,.F.,(4,2,2,2,2,2,3,2,2,2,2,4),(-0.287435863142792,-0.242415728674566,
-0.196766145639177,-0.149527097305729,-0.0994188710016275,-0.0495338134348599,
0.,0.0181167695461263,0.0672138706812888,0.116111680955793,0.165495495020501,
0.180763661414687),.UNSPECIFIED.);
#2078=B_SPLINE_CURVE_WITH_KNOTS('',3,(#75341,#75342,#75343,#75344,#75345,
#75346,#75347,#75348),.UNSPECIFIED.,.F.,.F.,(4,2,2,4),(0.20723494990689,
0.211936470059604,0.25766217050719,0.28738038516735),.UNSPECIFIED.);
#2079=B_SPLINE_CURVE_WITH_KNOTS('',3,(#75351,#75352,#75353,#75354,#75355,
#75356,#75357,#75358,#75359,#75360,#75361,#75362,#75363,#75364,#75365,#75366,
#75367,#75368,#75369,#75370,#75371,#75372,#75373,#75374,#75375),
 .UNSPECIFIED.,.F.,.F.,(4,2,2,2,2,2,3,2,2,2,2,4),(-0.287435863143056,-0.242415728674689,
-0.196766145639263,-0.14952709730598,-0.099418871001769,-0.0495338134348932,
0.,0.0181167695462657,0.0672138706821976,0.116111680957489,0.165495495022889,
0.20723494990689),.UNSPECIFIED.);
#2080=B_SPLINE_CURVE_WITH_KNOTS('',3,(#75484,#75485,#75486,#75487,#75488,
#75489),.UNSPECIFIED.,.F.,.F.,(4,2,4),(0.233673284093007,0.257662170504296,
0.287380385164373),.UNSPECIFIED.);
#2081=B_SPLINE_CURVE_WITH_KNOTS('',3,(#75492,#75493,#75494,#75495,#75496,
#75497,#75498,#75499,#75500,#75501,#75502,#75503,#75504,#75505,#75506,#75507,
#75508,#75509,#75510,#75511,#75512,#75513,#75514,#75515,#75516,#75517,#75518),
 .UNSPECIFIED.,.F.,.F.,(4,2,2,2,2,2,3,2,2,2,2,2,4),(-0.287435863141504,
-0.242415728674061,-0.196766145638992,-0.149527097305872,-0.0994188710018303,
-0.0495338134349093,0.,0.0181167695460408,0.0672138706811696,0.116111680955736,
0.165495495020723,0.211936470057386,0.233673284093007),.UNSPECIFIED.);
#2082=B_SPLINE_CURVE_WITH_KNOTS('',3,(#75627,#75628,#75629,#75630),
 .UNSPECIFIED.,.F.,.F.,(4,4),(0.260117487351587,0.287380385169054),
 .UNSPECIFIED.);
#2083=B_SPLINE_CURVE_WITH_KNOTS('',3,(#75633,#75634,#75635,#75636,#75637,
#75638,#75639,#75640,#75641,#75642,#75643,#75644,#75645,#75646,#75647,#75648,
#75649,#75650,#75651,#75652,#75653,#75654,#75655,#75656,#75657,#75658,#75659,
#75660,#75661),.UNSPECIFIED.,.F.,.F.,(4,2,2,2,2,2,3,2,2,2,2,2,2,4),(-0.287435863143853,
-0.242415728675398,-0.19676614563975,-0.149527097306065,-0.0994188710017117,
-0.0495338134348613,0.,0.0181167695462665,0.0672138706825982,0.116111680958237,
0.165495495023962,0.211936470061099,0.257662170508858,0.260117487351587),
 .UNSPECIFIED.);
#2084=B_SPLINE_CURVE_WITH_KNOTS('',3,(#75758,#75759,#75760,#75761),
 .UNSPECIFIED.,.F.,.F.,(4,4),(0.286585728945047,0.287380385163699),
 .UNSPECIFIED.);
#2085=B_SPLINE_CURVE_WITH_KNOTS('',3,(#75764,#75765,#75766,#75767,#75768,
#75769,#75770,#75771,#75772,#75773,#75774,#75775,#75776,#75777,#75778,#75779,
#75780,#75781,#75782,#75783,#75784,#75785,#75786,#75787,#75788,#75789,#75790,
#75791,#75792),.UNSPECIFIED.,.F.,.F.,(4,2,2,2,2,2,3,2,2,2,2,2,2,4),(-0.287435863142645,
-0.242415728674694,-0.196766145639482,-0.149527097306091,-0.099418871001846,
-0.0495338134349094,0.,0.0181167695460932,0.0672138706811363,0.116111680955706,
0.165495495020644,0.211936470057252,0.257662170504159,0.286585728945047),
 .UNSPECIFIED.);
#2086=B_SPLINE_CURVE_WITH_KNOTS('',3,(#75903,#75904,#75905,#75906,#75907,
#75908,#75909,#75910,#75911,#75912,#75913,#75914,#75915,#75916,#75917,#75918,
#75919,#75920,#75921,#75922,#75923,#75924,#75925,#75926,#75927,#75928,#75929,
#75930,#75931),.UNSPECIFIED.,.F.,.F.,(4,2,2,2,2,2,2,3,2,2,2,2,2,4),(0.50632031739344,
0.53603853205329,0.581764232500794,0.628205207537996,0.677589021603566,
0.726486831878774,0.775583933014714,0.793700702560937,0.843234515995651,
0.893119573562134,0.94322779986628,0.990466848199578,1.0361164312349,1.08113656570317),
 .UNSPECIFIED.);
#2087=B_SPLINE_CURVE_WITH_KNOTS('',3,(#76031,#76032,#76033,#76034,#76035,
#76036,#76037,#76038,#76039,#76040,#76041,#76042),.UNSPECIFIED.,.F.,.F.,
(4,2,2,2,2,4),(0.,0.0190658252712468,0.0452304041939831,0.0568941639977528,
0.0817283147450615,0.110084577318765),.UNSPECIFIED.);
#2088=B_SPLINE_CURVE_WITH_KNOTS('',3,(#76058,#76059,#76060,#76061,#76062,
#76063,#76064,#76065,#76066,#76067,#76068,#76069,#76070,#76071,#76072,#76073,
#76074,#76075,#76076,#76077,#76078,#76079,#76080,#76081,#76082,#76083,#76084,
#76085,#76086,#76087,#76088,#76089,#76090,#76091,#76092,#76093),
 .UNSPECIFIED.,.F.,.F.,(4,2,2,2,2,2,2,2,2,2,2,2,2,2,2,2,2,4),(0.,0.0308101291271131,
0.0585102160249069,0.107376034221475,0.153242377810569,0.196274905402532,
0.246470222643019,0.271920550681864,0.288008391296742,0.294995460635489,
0.310418509414427,0.333264464530267,0.381330610566836,0.423929647067707,
0.469249423768235,0.517202341943224,0.551749790166704,0.59009865246996),
 .UNSPECIFIED.);
#2089=B_SPLINE_CURVE_WITH_KNOTS('',3,(#76181,#76182,#76183,#76184,#76185,
#76186,#76187,#76188,#76189,#76190,#76191,#76192,#76193,#76194),
 .UNSPECIFIED.,.F.,.F.,(4,2,2,2,2,2,4),(0.,0.0755351073398052,0.117972466547439,
0.150106900517715,0.182308953145744,0.22500423988959,0.300408947780656),
 .UNSPECIFIED.);
#2090=B_SPLINE_CURVE_WITH_KNOTS('',3,(#76366,#76367,#76368,#76369,#76370,
#76371,#76372,#76373,#76374,#76375,#76376,#76377,#76378,#76379,#76380,#76381,
#76382,#76383,#76384,#76385,#76386,#76387,#76388,#76389),.UNSPECIFIED.,
 .F.,.F.,(4,2,2,2,2,2,2,2,2,2,2,4),(0.,0.0432252777893914,0.0917875128943153,
0.153562045824851,0.189491598602029,0.215103697999651,0.226790580176592,
0.253342417228272,0.292964110987221,0.354939922037077,0.394370298538859,
0.430153691883516),.UNSPECIFIED.);
#2091=B_SPLINE_CURVE_WITH_KNOTS('',3,(#76597,#76598,#76599,#76600,#76601,
#76602,#76603,#76604,#76605,#76606),.UNSPECIFIED.,.F.,.F.,(4,2,2,2,4),(0.115471253326685,
0.14952709730731,0.196766145641448,0.242415728677503,0.287435863146423),
 .UNSPECIFIED.);
#2092=B_SPLINE_CURVE_WITH_KNOTS('',3,(#76608,#76609,#76610,#76611,#76612,
#76613,#76614,#76615,#76616,#76617,#76618,#76619,#76620,#76621,#76622,#76623,
#76624,#76625,#76626,#76627,#76628,#76629,#76630,#76631,#76632,#76633,#76634,
#76635),.UNSPECIFIED.,.F.,.F.,(4,2,2,2,2,2,2,2,2,2,2,2,2,4),(0.,0.0337497043514118,
0.064125244377998,0.112622372775232,0.158167577684873,0.200871358502125,
0.246447408502993,0.269509078364172,0.2859826603936,0.293562975218655,0.311533142617737,
0.3405100735619,0.374412159077522,0.401781469644215),.UNSPECIFIED.);
#2093=B_SPLINE_CURVE_WITH_KNOTS('',3,(#76747,#76748,#76749,#76750,#76751,
#76752,#76753,#76754,#76755,#76756,#76757,#76758,#76759,#76760,#76761,#76762,
#76763,#76764,#76765,#76766,#76767,#76768,#76769,#76770,#76771,#76772,#76773,
#76774,#76775),.UNSPECIFIED.,.F.,.F.,(4,2,2,2,2,2,2,3,2,2,2,2,2,4),(0.506320317396995,
0.536038532057083,0.581764232504992,0.628205207542535,0.677589021608681,
0.726486831884498,0.775583933021264,0.793700702567583,0.843234516002442,
0.893119573569278,0.943227799873571,0.990466848207139,1.03611643124272,
1.08113656571108),.UNSPECIFIED.);
#2094=B_SPLINE_CURVE_WITH_KNOTS('',3,(#76885,#76886,#76887,#76888,#76889,
#76890,#76891,#76892,#76893,#76894,#76895,#76896,#76897,#76898,#76899,#76900,
#76901,#76902,#76903,#76904,#76905,#76906,#76907,#76908,#76909,#76910,#76911,
#76912,#76913),.UNSPECIFIED.,.F.,.F.,(4,2,2,2,2,2,3,2,2,2,2,2,2,4),(-0.268990399052299,
-0.242415728673278,-0.196766145638393,-0.149527097305505,-0.0994188710015041,
-0.0495338134348189,0.,0.0181167695460229,0.0672138706805404,0.116111680954595,
0.165495495019033,0.211936470055113,0.257662170501655,0.287380385160891),
 .UNSPECIFIED.);
#2095=B_SPLINE_CURVE_WITH_KNOTS('',3,(#76916,#76917,#76918,#76919),
 .UNSPECIFIED.,.F.,.F.,(4,4),(-0.287435863140965,-0.268990399052299),
 .UNSPECIFIED.);
#2096=B_SPLINE_CURVE_WITH_KNOTS('',3,(#77016,#77017,#77018,#77019,#77020,
#77021,#77022,#77023,#77024,#77025,#77026,#77027,#77028,#77029,#77030,#77031,
#77032,#77033,#77034,#77035,#77036,#77037,#77038,#77039,#77040,#77041,#77042,
#77043,#77044),.UNSPECIFIED.,.F.,.F.,(4,2,2,2,2,2,3,2,2,2,2,2,2,4),(-0.242533959473534,
-0.242415728674442,-0.196766145639165,-0.149527097305957,-0.099418871001771,
-0.0495338134348831,0.,0.0181167695462372,0.067213870681872,0.116111680956732,
0.165495495021875,0.211936470058645,0.257662170505937,0.287380385164999),
 .UNSPECIFIED.);
#2097=B_SPLINE_CURVE_WITH_KNOTS('',3,(#77047,#77048,#77049,#77050),
 .UNSPECIFIED.,.F.,.F.,(4,4),(-0.287435863143146,-0.242533959473534),
 .UNSPECIFIED.);
#2098=B_SPLINE_CURVE_WITH_KNOTS('',3,(#77159,#77160,#77161,#77162,#77163,
#77164,#77165,#77166,#77167,#77168,#77169,#77170,#77171,#77172,#77173,#77174,
#77175,#77176,#77177,#77178,#77179,#77180,#77181,#77182,#77183,#77184,#77185),
 .UNSPECIFIED.,.F.,.F.,(4,2,2,2,2,3,2,2,2,2,2,2,4),(-0.216081250737383,
-0.196766145639079,-0.149527097305844,-0.0994188710017439,-0.0495338134348963,
0.,0.0181167695460728,0.067213870681023,0.116111680955563,0.165495495020394,
0.211936470056958,0.25766217050386,0.287380385163262),.UNSPECIFIED.);
#2099=B_SPLINE_CURVE_WITH_KNOTS('',3,(#77188,#77189,#77190,#77191,#77192,
#77193),.UNSPECIFIED.,.F.,.F.,(4,2,4),(-0.287435863142567,-0.242415728674427,
-0.216081250737383),.UNSPECIFIED.);
#2100=B_SPLINE_CURVE_WITH_KNOTS('',3,(#77302,#77303,#77304,#77305,#77306,
#77307,#77308,#77309,#77310,#77311,#77312,#77313,#77314,#77315,#77316,#77317,
#77318,#77319,#77320,#77321,#77322,#77323,#77324,#77325,#77326),
 .UNSPECIFIED.,.F.,.F.,(4,2,2,2,3,2,2,2,2,2,2,4),(-0.189647450541698,-0.149527097305893,
-0.0994188710016985,-0.0495338134348624,0.,0.0181167695462411,0.0672138706819809,
0.11611168095712,0.165495495022401,0.211936470059391,0.25766217050701,0.287380385166855),
 .UNSPECIFIED.);
#2101=B_SPLINE_CURVE_WITH_KNOTS('',3,(#77329,#77330,#77331,#77332,#77333,
#77334,#77335,#77336),.UNSPECIFIED.,.F.,.F.,(4,2,2,4),(-0.287435863142678,
-0.242415728674601,-0.19676614563926,-0.189647450541698),.UNSPECIFIED.);
#2102=B_SPLINE_CURVE_WITH_KNOTS('',3,(#77403,#77404,#77405,#77406,#77407,
#77408,#77409,#77410,#77411,#77412,#77413,#77414,#77415,#77416,#77417,#77418,
#77419,#77420,#77421,#77422,#77423,#77424,#77425),.UNSPECIFIED.,.F.,.F.,
(4,2,2,2,2,2,3,2,2,2,4),(0.46489444415617,0.482224630787222,0.523014478228721,
0.563360237935425,0.603655558776688,0.623959945526705,0.644496878439993,
0.684450988861052,0.72440704183694,0.76453906647082,0.78715174771853),
 .UNSPECIFIED.);
#2103=B_SPLINE_CURVE_WITH_KNOTS('',3,(#77426,#77427,#77428,#77429,#77430,
#77431,#77432,#77433,#77434,#77435,#77436,#77437,#77438,#77439,#77440,#77441,
#77442,#77443,#77444,#77445),.UNSPECIFIED.,.F.,.F.,(4,2,2,2,2,2,2,2,2,4),
(0.78715174771853,0.804846372450503,0.845196940900909,0.88516602818916,
0.925643806988713,0.96618514649351,1.00632457127068,1.04643432468934,1.08640961177265,
1.10939132259616),.UNSPECIFIED.);
#2104=B_SPLINE_CURVE_WITH_KNOTS('',3,(#77453,#77454,#77455,#77456),
 .UNSPECIFIED.,.F.,.F.,(4,4),(0.,0.000964377926953999),.UNSPECIFIED.);
#2105=B_SPLINE_CURVE_WITH_KNOTS('',3,(#77458,#77459,#77460,#77461),
 .UNSPECIFIED.,.F.,.F.,(4,4),(0.000964426268463036,0.0153569489639517),
 .UNSPECIFIED.);
#2106=B_SPLINE_CURVE_WITH_KNOTS('',3,(#77463,#77464,#77465,#77466,#77467,
#77468,#77469,#77470,#77471,#77472,#77473,#77474,#77475,#77476,#77477,#77478,
#77479,#77480,#77481,#77482,#77483,#77484,#77485,#77486,#77487,#77488,#77489,
#77490,#77491,#77492,#77493,#77494,#77495,#77496,#77497,#77498,#77499,#77500,
#77501,#77502,#77503,#77504,#77505,#77506,#77507,#77508,#77509,#77510,#77511,
#77512,#77513,#77514,#77515,#77516,#77517,#77518,#77519,#77520,#77521,#77522,
#77523,#77524,#77525,#77526,#77527,#77528,#77529,#77530,#77531,#77532,#77533,
#77534,#77535,#77536,#77537,#77538,#77539,#77540,#77541,#77542,#77543,#77544,
#77545,#77546,#77547,#77548,#77549,#77550,#77551,#77552,#77553,#77554,#77555,
#77556,#77557,#77558,#77559,#77560,#77561,#77562,#77563,#77564,#77565,#77566,
#77567,#77568,#77569,#77570,#77571,#77572,#77573,#77574,#77575,#77576,#77577,
#77578,#77579,#77580,#77581,#77582,#77583,#77584,#77585,#77586,#77587,#77588,
#77589,#77590,#77591,#77592,#77593,#77594,#77595,#77596,#77597,#77598,#77599,
#77600,#77601,#77602,#77603,#77604,#77605,#77606,#77607,#77608,#77609,#77610,
#77611,#77612,#77613,#77614,#77615,#77616,#77617,#77618,#77619,#77620,#77621,
#77622),.UNSPECIFIED.,.F.,.F.,(4,3,3,3,3,3,3,3,3,3,3,3,3,3,3,3,3,3,3,3,
3,3,3,3,3,3,3,3,3,3,3,3,3,3,3,3,3,3,3,3,3,3,3,3,3,3,3,3,3,3,3,3,3,4),(0.0153569489639517,
0.0219282083148865,0.0294333381847798,0.0381269700773983,0.0456471396536513,
0.0550333230967721,0.0644194943084723,0.0738056535444641,0.0831918010597966,
0.0925779371097566,0.101964061949826,0.111350175835289,0.120736279021378,
0.130122371763683,0.139508454317902,0.148894526938201,0.158280589880695,
0.167666643401077,0.177052687754107,0.186438723195174,0.196237513095298,
0.205730090811043,0.21511647703801,0.224502831755281,0.233889155984714,
0.243275450747821,0.252661717066159,0.262047955961215,0.271434168454673,
0.280820355568032,0.290206518322942,0.29959265774067,0.308978774842652,
0.318364870650084,0.327750946184637,0.337137002467656,0.346523040520444,
0.356115350487863,0.365501714783882,0.374888018497213,0.384274265714455,
0.39366046052189,0.403046607005449,0.412432709250706,0.42181877134353,0.431591424925482,
0.440977743225469,0.450363950600201,0.459750063393973,0.469064457894216,
0.47842434354882,0.48778780374317,0.497151365244305,0.499999999999145),
 .UNSPECIFIED.);
#2107=B_SPLINE_CURVE_WITH_KNOTS('',3,(#77624,#77625,#77626,#77627,#77628,
#77629,#77630,#77631,#77632,#77633,#77634,#77635,#77636,#77637,#77638,#77639,
#77640,#77641,#77642,#77643,#77644,#77645,#77646,#77647,#77648,#77649,#77650,
#77651,#77652,#77653,#77654,#77655,#77656,#77657,#77658,#77659,#77660,#77661,
#77662,#77663,#77664,#77665,#77666,#77667,#77668,#77669,#77670,#77671,#77672,
#77673,#77674,#77675,#77676,#77677,#77678,#77679,#77680,#77681,#77682,#77683,
#77684,#77685,#77686,#77687,#77688,#77689,#77690,#77691,#77692,#77693,#77694,
#77695,#77696,#77697,#77698,#77699,#77700,#77701,#77702,#77703,#77704,#77705,
#77706,#77707,#77708,#77709,#77710,#77711,#77712,#77713,#77714,#77715,#77716,
#77717,#77718,#77719,#77720,#77721,#77722,#77723,#77724,#77725,#77726,#77727,
#77728,#77729,#77730,#77731,#77732,#77733,#77734,#77735,#77736,#77737,#77738,
#77739,#77740,#77741,#77742,#77743,#77744,#77745,#77746,#77747,#77748,#77749,
#77750,#77751,#77752,#77753,#77754,#77755,#77756,#77757,#77758,#77759,#77760,
#77761,#77762,#77763,#77764,#77765,#77766,#77767,#77768,#77769,#77770,#77771,
#77772,#77773,#77774,#77775,#77776,#77777,#77778,#77779,#77780,#77781,#77782,
#77783),.UNSPECIFIED.,.F.,.F.,(4,3,3,3,3,3,3,3,3,3,3,3,3,3,3,3,3,3,3,3,
3,3,3,3,3,3,3,3,3,3,3,3,3,3,3,3,3,3,3,3,3,3,3,3,3,3,3,3,3,3,3,3,3,4),(0.499999999999145,
0.509363634815052,0.518727213283903,0.528087636608761,0.537479514573638,
0.546865650705078,0.556251775624736,0.565637889587881,0.575023992849933,
0.584410085666254,0.593796168292422,0.60318224098332,0.612568303994555,
0.621954357581328,0.631340401999322,0.64072643750358,0.650527332785632,
0.66002195009012,0.669408336532774,0.678794691458984,0.688181015890325,
0.697567310848398,0.706953577354932,0.716339816431409,0.725726029099394,
0.735112216380421,0.744498379295462,0.753884518867239,0.763270636116398,
0.772656732063998,0.78204280773193,0.791428864141412,0.800814902313632,
0.810411163827108,0.819797528518683,0.829183832601694,0.838570080162811,
0.847956275288611,0.857342422064618,0.866728524576365,0.876114586909905,
0.885894649362323,0.895280968320628,0.904667176263448,0.914053289534979,
0.923439324478087,0.932825563338133,0.942211619595582,0.951597722715543,
0.954355086529251,0.963248944870356,0.971455195139771,0.978625769560708,
0.984645425631258),.UNSPECIFIED.);
#2108=B_SPLINE_CURVE_WITH_KNOTS('',3,(#77785,#77786,#77787,#77788),
 .UNSPECIFIED.,.F.,.F.,(4,4),(0.984645425631258,0.999035201896067),
 .UNSPECIFIED.);
#2109=B_SPLINE_CURVE_WITH_KNOTS('',3,(#77790,#77791,#77792,#77793),
 .UNSPECIFIED.,.F.,.F.,(4,4),(0.999035250238492,1.),.UNSPECIFIED.);
#2110=B_SPLINE_CURVE_WITH_KNOTS('',3,(#77818,#77819,#77820,#77821,#77822,
#77823,#77824,#77825,#77826,#77827),.UNSPECIFIED.,.F.,.F.,(4,2,2,2,4),(0.,
0.221863776616433,0.443727553232867,0.6655913298493,0.887455106465734),
 .UNSPECIFIED.);
#2111=B_SPLINE_CURVE_WITH_KNOTS('',3,(#77830,#77831,#77832,#77833,#77834,
#77835,#77836,#77837,#77838,#77839),.UNSPECIFIED.,.F.,.F.,(4,2,2,2,4),(0.,
0.22177646038554,0.443552920771081,0.665329381156621,0.887105841542162),
 .UNSPECIFIED.);
#2112=B_SPLINE_CURVE_WITH_KNOTS('',3,(#77861,#77862,#77863,#77864,#77865,
#77866,#77867,#77868,#77869,#77870,#77871,#77872,#77873,#77874,#77875,#77876,
#77877,#77878,#77879,#77880,#77881,#77882,#77883,#77884,#77885,#77886,#77887,
#77888,#77889,#77890,#77891),.UNSPECIFIED.,.F.,.F.,(4,3,3,3,3,3,3,3,3,3,
4),(0.0219302008781805,0.110889998370047,0.208167498777535,0.309406295627344,
0.422707248982262,0.5,0.625,0.72740110002725,0.823316949159066,0.912880322251734,
1.),.UNSPECIFIED.);
#2113=B_SPLINE_CURVE_WITH_KNOTS('',3,(#77908,#77909,#77910,#77911,#77912,
#77913,#77914,#77915,#77916,#77917,#77918,#77919,#77920,#77921,#77922,#77923,
#77924,#77925,#77926,#77927,#77928,#77929,#77930,#77931,#77932,#77933,#77934,
#77935,#77936,#77937,#77938,#77939,#77940,#77941),.UNSPECIFIED.,.T.,.F.,
(4,2,2,2,2,2,2,2,2,2,2,2,2,2,2,2,4),(-0.315583874891462,-0.29738266229352,
-0.27768463654161,-0.258053667090507,-0.238476218724991,-0.218890293083453,
-0.199237519662791,-0.179509847947857,-0.159745824539116,-0.139647939264777,
-0.119687705010333,-0.0997724646185103,-0.0798173438841853,-0.0598300512340101,
-0.0398741605185745,-0.0199587807235321,0.),.UNSPECIFIED.);
#2114=B_SPLINE_CURVE_WITH_KNOTS('',3,(#77945,#77946,#77947,#77948,#77949,
#77950,#77951,#77952,#77953,#77954,#77955,#77956,#77957,#77958,#77959,#77960,
#77961,#77962,#77963,#77964,#77965,#77966,#77967),.UNSPECIFIED.,.F.,.F.,
(4,2,2,2,2,2,2,2,2,3,4),(-0.322394442933457,-0.321463867844831,-0.281213098456134,
-0.241013349314738,-0.200984471704924,-0.161071936773251,-0.121080015185152,
-0.080858754962794,-0.0404461452144988,0.,6.19698534856371E-5),
 .UNSPECIFIED.);
#2115=B_SPLINE_CURVE_WITH_KNOTS('',3,(#77969,#77970,#77971,#77972,#77973,
#77974,#77975,#77976,#77977,#77978,#77979,#77980,#77981,#77982,#77983,#77984,
#77985,#77986),.UNSPECIFIED.,.F.,.F.,(4,2,2,2,2,2,2,2,4),(6.19698534856371E-5,
0.04009610250426,0.0805804917540971,0.120891813402526,0.161364748502932,
0.201955855009439,0.242412218648003,0.282721308068169,0.322308248865181),
 .UNSPECIFIED.);
#2116=B_SPLINE_CURVE_WITH_KNOTS('',3,(#78006,#78007,#78008,#78009,#78010,
#78011,#78012,#78013,#78014,#78015,#78016,#78017,#78018,#78019,#78020,#78021,
#78022,#78023,#78024,#78025,#78026,#78027),.UNSPECIFIED.,.F.,.F.,(4,3,3,
3,3,3,3,4),(0.000407408283309958,0.00497275683192009,0.005742565261487,
0.00594626923060788,0.00861384760452239,0.00871569970425684,0.0108497382981234,
0.0114851301779058),.UNSPECIFIED.);
#2117=B_SPLINE_CURVE_WITH_KNOTS('',3,(#78031,#78032,#78033,#78034,#78035,
#78036,#78037,#78038),.UNSPECIFIED.,.F.,.F.,(4,2,2,4),(-0.0450504263378443,
-0.043734901660658,-0.0225288176281075,0.),.UNSPECIFIED.);
#2118=B_SPLINE_CURVE_WITH_KNOTS('',3,(#78047,#78048,#78049,#78050,#78051,
#78052,#78053,#78054,#78055,#78056,#78057,#78058,#78059,#78060,#78061,#78062,
#78063,#78064,#78065,#78066,#78067,#78068),.UNSPECIFIED.,.F.,.F.,(4,3,3,
3,3,3,3,4),(2.91329505494903E-9,0.000660163016541207,0.00123543637619839,
0.0017900655732896,0.00185315456429469,0.00211503954798182,0.00237836381180336,
0.00247087275239099),.UNSPECIFIED.);
#2119=B_SPLINE_CURVE_WITH_KNOTS('',3,(#78072,#78073,#78074,#78075,#78076,
#78077,#78078,#78079,#78080,#78081,#78082,#78083,#78084,#78085,#78086,#78087,
#78088,#78089),.UNSPECIFIED.,.F.,.F.,(4,2,2,2,2,2,2,2,4),(-0.31597704258338,
-0.275100125004532,-0.244154449549492,-0.223290285080556,-0.213738196895435,
-0.192181551009235,-0.15769667845806,-0.0892749983694439,-1.39001374278569E-6),
 .UNSPECIFIED.);
#2120=B_SPLINE_CURVE_WITH_KNOTS('',3,(#78105,#78106,#78107,#78108,#78109,
#78110),.UNSPECIFIED.,.F.,.F.,(4,2,4),(1.13372962259874E-5,0.075979708245961,
0.132752016386919),.UNSPECIFIED.);
#2121=B_SPLINE_CURVE_WITH_KNOTS('',3,(#78116,#78117,#78118,#78119,#78120,
#78121,#78122,#78123,#78124,#78125,#78126,#78127,#78128,#78129,#78130,#78131,
#78132,#78133,#78134),.UNSPECIFIED.,.F.,.F.,(4,3,3,3,3,3,4),(0.,0.00276943641060585,
0.00281960538769298,0.00553887282121171,0.00570812155224864,0.0103685864131738,
0.0110777456424234),.UNSPECIFIED.);
#2122=B_SPLINE_CURVE_WITH_KNOTS('',3,(#78136,#78137,#78138,#78139,#78140,
#78141,#78142,#78143,#78144,#78145),.UNSPECIFIED.,.F.,.F.,(4,3,3,4),(5.53618044130801E-9,
0.000299661069992586,0.000432086313124671,0.000450310767172612),
 .UNSPECIFIED.);
#2123=B_SPLINE_CURVE_WITH_KNOTS('',3,(#78171,#78172,#78173,#78174,#78175,
#78176,#78177,#78178,#78179,#78180,#78181,#78182,#78183),.UNSPECIFIED.,
 .F.,.F.,(4,3,3,3,4),(2.55408693138011E-10,0.000328350173161266,0.00065542770044065,
0.000980575591406873,0.00121964937926107),.UNSPECIFIED.);
#2124=B_SPLINE_CURVE_WITH_KNOTS('',3,(#78191,#78192,#78193,#78194,#78195,
#78196),.UNSPECIFIED.,.F.,.F.,(4,2,4),(-0.12344151138567,-0.0612593453644722,
-1.69855123624801E-5),.UNSPECIFIED.);
#2125=B_SPLINE_CURVE_WITH_KNOTS('',3,(#78197,#78198,#78199,#78200,#78201,
#78202,#78203,#78204,#78205,#78206,#78207,#78208,#78209,#78210,#78211,#78212,
#78213,#78214,#78215,#78216,#78217,#78218,#78219,#78220,#78221,#78222,#78223,
#78224,#78225,#78226,#78227,#78228,#78229,#78230,#78231,#78232,#78233,#78234,
#78235,#78236,#78237,#78238,#78239,#78240,#78241,#78242,#78243,#78244,#78245,
#78246,#78247,#78248,#78249,#78250,#78251,#78252,#78253,#78254,#78255,#78256,
#78257,#78258,#78259,#78260,#78261,#78262,#78263,#78264,#78265,#78266,#78267,
#78268,#78269,#78270,#78271,#78272,#78273,#78274,#78275,#78276,#78277,#78278,
#78279,#78280,#78281,#78282,#78283,#78284,#78285,#78286,#78287,#78288,#78289,
#78290,#78291,#78292,#78293),.UNSPECIFIED.,.F.,.F.,(4,3,3,3,3,3,3,3,3,3,
3,3,3,3,3,3,3,3,3,3,3,3,3,3,3,3,3,3,3,3,3,3,4),(0.00488558905517301,0.0051934316125717,
0.00550131709313176,0.0056266698314079,0.00611648667187354,0.00636775060764279,
0.00686005421483842,0.00735498318747559,0.00784991216011275,0.00819113275196426,
0.00853283329082221,0.00859099293634774,0.00908351642592215,0.00933207371258273,
0.00982197624572552,0.0103181057553891,0.0108142352650527,0.0113008118805492,
0.0117986043490359,0.0122963968175226,0.0127889568608241,0.0130374775937576,
0.0133803810095318,0.0137227757530312,0.0137785583699925,0.0142670392354198,
0.0147638795789411,0.0152607199224624,0.0157505715721473,0.0160018006986973,
0.0163098524339766,0.016617784004579,0.016742881472115),.UNSPECIFIED.);
#2126=B_SPLINE_CURVE_WITH_KNOTS('',3,(#78306,#78307,#78308,#78309,#78310,
#78311,#78312,#78313,#78314,#78315,#78316,#78317,#78318,#78319,#78320,#78321,
#78322,#78323),.UNSPECIFIED.,.F.,.F.,(4,2,2,2,2,2,2,2,4),(-0.314107268919085,
-0.223401463457807,-0.156175714250431,-0.122651406592743,-0.10167412033179,
-0.092313374585261,-0.0715343781050509,-0.0401556420432856,-1.88820737717577E-5),
 .UNSPECIFIED.);
#2127=B_SPLINE_CURVE_WITH_KNOTS('',3,(#78357,#78358,#78359,#78360),
 .UNSPECIFIED.,.F.,.F.,(4,4),(0.,0.000407408044724523),.UNSPECIFIED.);
#2128=B_SPLINE_CURVE_WITH_KNOTS('',3,(#78363,#78364,#78365,#78366,#78367,
#78368,#78369,#78370,#78371,#78372,#78373,#78374,#78375,#78376,#78377,#78378,
#78379,#78380,#78381,#78382,#78383,#78384,#78385,#78386,#78387,#78388,#78389,
#78390,#78391,#78392,#78393,#78394,#78395,#78396,#78397,#78398,#78399,#78400,
#78401,#78402,#78403,#78404,#78405,#78406,#78407,#78408),.UNSPECIFIED.,
 .F.,.F.,(4,3,3,3,3,3,3,3,3,3,3,3,3,3,3,4),(1.47097541858838E-9,0.000771492196635795,
0.00152729150168422,0.00226483520945305,0.00286070517058098,0.00360261249656041,
0.00434678131828715,0.0050965673029855,0.00572141034116197,0.00654881697400354,
0.00740654146015019,0.00829947330035251,0.00925690323311813,0.010261775897808,
0.0113497658956453,0.0114428206823239),.UNSPECIFIED.);
#2129=B_SPLINE_CURVE_WITH_KNOTS('',3,(#78562,#78563,#78564,#78565,#78566,
#78567,#78568,#78569,#78570,#78571,#78572,#78573,#78574,#78575,#78576,#78577,
#78578,#78579,#78580,#78581,#78582,#78583,#78584,#78585,#78586,#78587,#78588,
#78589,#78590,#78591,#78592,#78593,#78594,#78595,#78596,#78597,#78598,#78599,
#78600,#78601,#78602,#78603,#78604,#78605,#78606,#78607,#78608,#78609,#78610,
#78611,#78612,#78613,#78614,#78615,#78616,#78617,#78618,#78619,#78620,#78621,
#78622,#78623,#78624,#78625,#78626,#78627,#78628,#78629,#78630,#78631,#78632,
#78633,#78634,#78635,#78636,#78637,#78638,#78639,#78640,#78641,#78642,#78643,
#78644,#78645,#78646,#78647,#78648,#78649,#78650,#78651,#78652,#78653,#78654,
#78655,#78656,#78657,#78658,#78659,#78660,#78661,#78662,#78663,#78664,#78665,
#78666,#78667,#78668,#78669,#78670,#78671,#78672,#78673,#78674,#78675,#78676,
#78677,#78678,#78679,#78680,#78681,#78682,#78683,#78684,#78685,#78686,#78687,
#78688,#78689,#78690,#78691,#78692,#78693,#78694,#78695,#78696,#78697,#78698,
#78699,#78700,#78701,#78702,#78703,#78704,#78705,#78706,#78707,#78708,#78709,
#78710,#78711,#78712,#78713,#78714,#78715,#78716,#78717,#78718,#78719,#78720,
#78721,#78722,#78723,#78724,#78725,#78726,#78727,#78728,#78729,#78730,#78731,
#78732,#78733,#78734,#78735,#78736,#78737,#78738,#78739),.UNSPECIFIED.,
 .F.,.F.,(4,3,3,3,3,3,3,3,3,3,3,3,3,3,3,3,3,3,3,3,3,3,3,3,3,3,3,3,3,3,3,
3,3,3,3,3,3,3,3,3,3,3,3,3,3,3,3,3,3,3,3,3,3,3,3,3,3,3,3,4),(0.,0.000926416342889362,
0.00173634802732097,0.00175238767688987,0.00260794610843211,0.00262858151533464,
0.00340413825758895,0.00348157049108613,0.00350477535377941,0.00497295805954557,
0.00523349326742887,0.00525716303066868,0.00611135611184734,0.0069897893210327,
0.00700955070755794,0.00850723651272925,0.00874742345145967,0.0087619383844472,
0.00962649083989963,0.00963813222289174,0.0105052986518987,0.0105143260613363,
0.0113839108634704,0.0113905198997808,0.0122624548555008,0.0122667137382254,
0.0135264537493205,0.0140191014151145,0.014019137693761,0.0148952952535591,
0.014897467492945,0.0157714890920036,0.0157758871470558,0.0169878014714307,
0.0175238767688928,0.0175330131040703,0.0184000706073373,0.0184119417422983,
0.0192762644457819,0.0192908621262671,0.0201524582842264,0.0201697828683268,
0.0208826521471334,0.0210286521226709,0.0210487131721851,0.0221316423632042,
0.02278103979956,0.0228048120482523,0.0236572336380045,0.0236815439919199,
0.024533427476449,0.0245569736992918,0.0257675221065015,0.0262858151533381,
0.0263020749158942,0.0267918500587691,0.0271620089917824,0.0275476169326534,
0.0279235134160577,0.0280382028302268),.UNSPECIFIED.);
#2130=B_SPLINE_CURVE_WITH_KNOTS('',3,(#78740,#78741,#78742,#78743,#78744,
#78745,#78746,#78747,#78748,#78749,#78750,#78751,#78752,#78753,#78754,#78755,
#78756,#78757,#78758,#78759,#78760,#78761,#78762,#78763,#78764,#78765,#78766,
#78767,#78768,#78769,#78770,#78771,#78772,#78773,#78774,#78775,#78776,#78777,
#78778,#78779,#78780,#78781,#78782,#78783,#78784,#78785,#78786,#78787,#78788,
#78789,#78790,#78791,#78792,#78793,#78794,#78795,#78796,#78797,#78798,#78799,
#78800,#78801,#78802,#78803,#78804,#78805,#78806,#78807,#78808,#78809,#78810,
#78811,#78812,#78813,#78814,#78815,#78816,#78817,#78818,#78819,#78820,#78821,
#78822,#78823,#78824,#78825,#78826,#78827,#78828,#78829,#78830,#78831,#78832,
#78833,#78834,#78835,#78836,#78837,#78838,#78839,#78840,#78841,#78842,#78843,
#78844,#78845,#78846,#78847,#78848,#78849,#78850,#78851,#78852,#78853,#78854,
#78855,#78856,#78857,#78858,#78859,#78860,#78861,#78862,#78863,#78864,#78865,
#78866,#78867,#78868,#78869,#78870,#78871,#78872,#78873,#78874,#78875,#78876,
#78877,#78878,#78879,#78880,#78881,#78882,#78883,#78884,#78885,#78886,#78887,
#78888,#78889,#78890,#78891,#78892,#78893,#78894,#78895,#78896,#78897,#78898,
#78899,#78900,#78901,#78902),.UNSPECIFIED.,.F.,.F.,(4,3,3,3,3,3,3,3,3,3,
3,3,3,3,3,3,3,3,3,3,3,3,3,3,3,3,3,3,3,3,3,3,3,3,3,3,3,3,3,3,3,3,3,3,3,3,
3,3,3,3,3,3,3,3,4),(0.,0.000368128432020981,0.000744995308322254,0.000832257560475207,
0.0013051293478806,0.00166426378958133,0.00166451512095041,0.00296289381169945,
0.00332903024190082,0.00333012447958715,0.00416335856250361,0.00499354536285123,
0.00499658605666537,0.00656887393213025,0.00665806048380164,0.00666253488292151,
0.00749031804427697,0.00749514135964159,0.0083225756047523,0.00832744533043317,
0.00915483316522763,0.0091594350159297,0.00998709072570296,0.00999111303251047,
0.0116516058466535,0.0116538603965027,0.0124838634071288,0.0124849548202084,
0.0133160095344897,0.0133161209676041,0.0148710898848926,0.0149782215041487,
0.0149806360885546,0.0158094588117832,0.0158128936490299,0.0166409414709503,
0.0166451512095052,0.0174726683061663,0.0174774087699804,0.0183046496274646,
0.0183096663304557,0.0199695592386629,0.0199741814514062,0.0208024587002455,
0.021635565418514,0.0216386965723568,0.0231473042510861,0.0233019830100467,
0.0233032116933073,0.0241350880431039,0.0241354692537826,0.0249677268142579,
0.0249679138728332,0.0260382453062477,0.0266322419352084),.UNSPECIFIED.);
#2131=B_SPLINE_CURVE_WITH_KNOTS('',3,(#78933,#78934,#78935,#78936,#78937,
#78938,#78939,#78940,#78941,#78942,#78943,#78944,#78945,#78946,#78947,#78948,
#78949,#78950,#78951,#78952,#78953,#78954,#78955,#78956,#78957,#78958,#78959,
#78960,#78961,#78962,#78963,#78964,#78965,#78966,#78967,#78968,#78969,#78970,
#78971,#78972,#78973,#78974,#78975,#78976,#78977,#78978),.UNSPECIFIED.,
 .F.,.F.,(4,3,3,3,3,3,3,3,3,3,3,3,3,3,3,4),(0.,0.00106719154926921,0.00206281499229115,
0.00297783614552313,0.00385877869507663,0.00471036156803993,0.00552671449927665,
0.00572149247899258,0.00647690763549953,0.00722797363372799,0.00797355695846304,
0.00858223871848886,0.00932082492988301,0.0100699874777538,0.0108423688248513,
0.0114429849579852),.UNSPECIFIED.);
#2132=B_SPLINE_CURVE_WITH_KNOTS('',3,(#78979,#78980,#78981,#78982),
 .UNSPECIFIED.,.F.,.F.,(4,4),(0.011077745885897,0.0114851542376453),
 .UNSPECIFIED.);
#2133=B_SPLINE_CURVE_WITH_KNOTS('',3,(#78988,#78989,#78990,#78991,#78992,
#78993,#78994,#78995,#78996,#78997,#78998,#78999,#79000,#79001,#79002,#79003,
#79004,#79005,#79006,#79007,#79008,#79009,#79010,#79011,#79012,#79013,#79014,
#79015,#79016,#79017,#79018,#79019,#79020,#79021,#79022,#79023,#79024,#79025,
#79026,#79027,#79028,#79029,#79030,#79031,#79032,#79033,#79034,#79035,#79036,
#79037,#79038,#79039,#79040,#79041,#79042,#79043,#79044,#79045,#79046,#79047,
#79048,#79049,#79050,#79051,#79052,#79053,#79054,#79055,#79056,#79057,#79058,
#79059,#79060),.UNSPECIFIED.,.F.,.F.,(4,3,3,3,3,3,3,3,3,3,3,3,3,3,3,3,3,
3,3,3,3,3,3,3,4),(0.00723577310341842,0.00746729739937353,0.00813249812078954,
0.00829755964440309,0.00874410725636207,0.00949827503482505,0.00995736819421411,
0.010252442813288,0.0113395003728997,0.0116156878478535,0.011760778370214,
0.0124443236839924,0.0132691139271399,0.0132728091843271,0.0147774494840659,
0.0149301313935435,0.0155316172625289,0.0157589738467299,0.0162857850409919,
0.0165883666173337,0.0177941205979179,0.0182480168910559,0.018548288376381,
0.0191055922868745,0.0193024561548439),.UNSPECIFIED.);
#2134=B_SPLINE_CURVE_WITH_KNOTS('',3,(#79076,#79077,#79078,#79079),
 .UNSPECIFIED.,.F.,.F.,(4,4),(0.,0.00312907272408999),.UNSPECIFIED.);
#2135=B_SPLINE_CURVE_WITH_KNOTS('',3,(#79082,#79083,#79084,#79085),
 .UNSPECIFIED.,.F.,.F.,(4,4),(0.,1.),.UNSPECIFIED.);
#2136=B_SPLINE_CURVE_WITH_KNOTS('',3,(#79204,#79205,#79206,#79207,#79208,
#79209,#79210,#79211,#79212,#79213,#79214,#79215,#79216,#79217,#79218,#79219,
#79220,#79221,#79222,#79223,#79224,#79225,#79226,#79227,#79228),
 .UNSPECIFIED.,.F.,.F.,(4,3,3,3,3,3,3,3,4),(0.,0.125,0.25,0.258487929334817,
0.437367182643581,0.5,0.562763102241527,0.867038912738001,0.999999776819451),
 .UNSPECIFIED.);
#2137=B_SPLINE_CURVE_WITH_KNOTS('',3,(#79230,#79231,#79232,#79233,#79234,
#79235,#79236,#79237,#79238,#79239,#79240,#79241,#79242,#79243,#79244,#79245,
#79246,#79247,#79248,#79249,#79250,#79251,#79252,#79253,#79254,#79255,#79256,
#79257,#79258,#79259,#79260,#79261,#79262,#79263,#79264,#79265,#79266,#79267,
#79268,#79269,#79270,#79271,#79272,#79273,#79274,#79275,#79276,#79277,#79278,
#79279,#79280,#79281,#79282,#79283,#79284,#79285,#79286,#79287,#79288,#79289,
#79290,#79291,#79292,#79293,#79294,#79295,#79296,#79297,#79298,#79299),
 .UNSPECIFIED.,.F.,.F.,(4,3,3,3,3,3,3,3,3,3,3,3,3,3,3,3,3,3,3,3,3,3,3,4),
(0.,0.0141557809778879,0.0625000000000003,0.0746323172226332,0.125000000000001,
0.13511093095757,0.250000000000001,0.256066251541517,0.375000000000001,
0.3770215763065,0.487187056529488,0.497976862476372,0.500000000000001,0.558454572926683,
0.562500000000001,0.618932222315836,0.625000000000001,0.739887548974724,
0.750000000000001,0.860842875279398,0.875,0.941938525686023,0.981797501825127,
0.999999999378131),.UNSPECIFIED.);
#2138=B_SPLINE_CURVE_WITH_KNOTS('',3,(#79300,#79301,#79302,#79303,#79304,
#79305,#79306,#79307,#79308,#79309,#79310,#79311,#79312,#79313,#79314,#79315,
#79316,#79317,#79318,#79319,#79320,#79321),.UNSPECIFIED.,.F.,.F.,(4,3,3,
3,3,3,3,4),(1.32021523337872E-9,0.130874672952653,0.432343443865136,0.500000000000005,
0.733812423852511,0.750000000000002,0.964531007757503,0.999999999999006),
 .UNSPECIFIED.);
#2139=B_SPLINE_CURVE_WITH_KNOTS('',3,(#79322,#79323,#79324,#79325,#79326,
#79327,#79328,#79329,#79330,#79331,#79332,#79333,#79334,#79335,#79336,#79337,
#79338,#79339,#79340,#79341,#79342,#79343,#79344,#79345,#79346,#79347,#79348,
#79349,#79350,#79351,#79352,#79353,#79354,#79355,#79356,#79357,#79358,#79359,
#79360,#79361,#79362,#79363,#79364,#79365,#79366,#79367,#79368,#79369,#79370,
#79371,#79372,#79373,#79374,#79375,#79376,#79377,#79378,#79379,#79380,#79381,
#79382,#79383,#79384,#79385,#79386,#79387,#79388,#79389,#79390,#79391,#79392,
#79393,#79394,#79395,#79396,#79397,#79398,#79399,#79400,#79401,#79402,#79403,
#79404,#79405,#79406,#79407,#79408,#79409,#79410,#79411,#79412,#79413,#79414,
#79415,#79416,#79417,#79418,#79419,#79420,#79421,#79422,#79423,#79424,#79425,
#79426,#79427,#79428,#79429,#79430,#79431,#79432,#79433,#79434,#79435,#79436,
#79437,#79438,#79439,#79440,#79441,#79442,#79443,#79444,#79445,#79446,#79447,
#79448,#79449,#79450,#79451,#79452,#79453,#79454,#79455,#79456,#79457,#79458,
#79459,#79460,#79461,#79462,#79463,#79464,#79465,#79466,#79467,#79468,#79469,
#79470,#79471,#79472,#79473,#79474,#79475,#79476,#79477,#79478,#79479,#79480,
#79481),.UNSPECIFIED.,.F.,.F.,(4,3,3,3,3,3,3,3,3,3,3,3,3,3,3,3,3,3,3,3,
3,3,3,3,3,3,3,3,3,3,3,3,3,3,3,3,3,3,3,3,3,3,3,3,3,3,3,3,3,3,3,3,3,4),(2.91264979220492E-15,
0.00300575703219071,0.00458596257778495,0.00462972345140002,0.00757533490906404,
0.00918741237741677,0.00925944690279713,0.0126379912408766,0.0138046411776548,
0.0138891703541942,0.0172144086662736,0.0184304802702438,0.0185188938055914,
0.0219135792309688,0.023059852717408,0.0231486172569885,0.026176380485865,
0.0276962761650712,0.0277783407083856,0.0309338119603887,0.0323414639693572,
0.0324080641597827,0.0344028998389768,0.0346670786726838,0.0347229258854812,
0.0365283926285558,0.036993641415406,0.0370377876111798,0.040278050293859,
0.041644475594072,0.0416675110625769,0.0449242871498441,0.0462888090190751,
0.046297234513974,0.0493505573314523,0.0509248440873743,0.0509269579653712,
0.0532400429443998,0.0532418196910697,0.0555542205796149,0.0555566814167682,
0.0588514339459642,0.0601819075336434,0.0601864048681651,0.0640737496238627,
0.0648116186367275,0.064816128319562,0.0689095202840357,0.0694454977932579,
0.0694458517709589,0.0709188654315961,0.0723842403891683,0.0737814416001958,
0.0740755752223558),.UNSPECIFIED.);
#2140=B_SPLINE_CURVE_WITH_KNOTS('',3,(#79494,#79495,#79496,#79497,#79498,
#79499,#79500),.UNSPECIFIED.,.F.,.F.,(4,3,4),(0.,0.00276685003849761,0.00458363052137194),
 .UNSPECIFIED.);
#2141=B_SPLINE_CURVE_WITH_KNOTS('',3,(#79515,#79516,#79517,#79518),
 .UNSPECIFIED.,.F.,.F.,(4,4),(0.,1.),.UNSPECIFIED.);
#2142=B_SPLINE_CURVE_WITH_KNOTS('',3,(#79519,#79520,#79521,#79522),
 .UNSPECIFIED.,.F.,.F.,(4,4),(0.,0.00312895336538498),.UNSPECIFIED.);
#2143=B_SPLINE_CURVE_WITH_KNOTS('',3,(#79535,#79536,#79537,#79538,#79539,
#79540,#79541),.UNSPECIFIED.,.F.,.F.,(4,3,4),(5.87409092738369E-11,0.00293217098656389,
0.00458274107704695),.UNSPECIFIED.);
#2144=B_SPLINE_CURVE_WITH_KNOTS('',3,(#79570,#79571,#79572,#79573,#79574,
#79575,#79576,#79577,#79578,#79579,#79580,#79581,#79582,#79583,#79584,#79585),
 .UNSPECIFIED.,.F.,.F.,(4,3,3,3,3,4),(0.,0.000314760444717577,0.000629520889435155,
0.000835315943262965,0.00104717886106664,0.00125904177887031),
 .UNSPECIFIED.);
#2145=B_SPLINE_CURVE_WITH_KNOTS('',3,(#79619,#79620,#79621,#79622,#79623,
#79624,#79625,#79626,#79627,#79628,#79629,#79630,#79631,#79632,#79633,#79634),
 .UNSPECIFIED.,.F.,.F.,(4,3,3,3,3,4),(0.,0.000314760444717579,0.000629520889435158,
0.000835315943339465,0.00104717886110491,0.00125904177887035),
 .UNSPECIFIED.);
#2146=B_SPLINE_CURVE_WITH_KNOTS('',3,(#79661,#79662,#79663,#79664,#79665,
#79666,#79667,#79668,#79669,#79670,#79671,#79672,#79673,#79674,#79675,#79676),
 .UNSPECIFIED.,.F.,.F.,(4,3,3,3,3,4),(0.,0.000314760444717591,0.000629520889435182,
0.000835315943223551,0.00104717886104696,0.00125904177887036),
 .UNSPECIFIED.);
#2147=B_SPLINE_CURVE_WITH_KNOTS('',3,(#79708,#79709,#79710,#79711,#79712,
#79713,#79714,#79715,#79716,#79717,#79718,#79719,#79720,#79721,#79722,#79723),
 .UNSPECIFIED.,.F.,.F.,(4,3,3,3,3,4),(0.,0.000314760444717582,0.000629520889435164,
0.000835315943184375,0.00104717886102734,0.0012590417788703),
 .UNSPECIFIED.);
#2148=B_SPLINE_CURVE_WITH_KNOTS('',3,(#79767,#79768,#79769,#79770,#79771,
#79772,#79773,#79774,#79775,#79776,#79777,#79778,#79779,#79780,#79781,#79782,
#79783,#79784,#79785,#79786,#79787,#79788,#79789,#79790,#79791,#79792,#79793,
#79794,#79795,#79796,#79797,#79798,#79799,#79800,#79801,#79802,#79803,#79804,
#79805,#79806,#79807,#79808,#79809,#79810,#79811,#79812,#79813,#79814,#79815),
 .UNSPECIFIED.,.F.,.F.,(4,3,3,3,3,3,3,3,3,3,3,3,3,3,3,3,4),(6.4247391107438E-15,
0.0672804347847839,0.137054964536528,0.212077380895502,0.227495036868895,
0.298907893425271,0.372169120979542,0.447629859322508,0.454990073737789,
0.529338104220492,0.605911607413588,0.6782088495798,0.682485110606684,0.757595417712821,
0.829409200582694,0.897759011016633,0.909980147475578),.UNSPECIFIED.);
#2149=B_SPLINE_CURVE_WITH_KNOTS('',3,(#79816,#79817,#79818,#79819,#79820,
#79821,#79822,#79823,#79824,#79825,#79826,#79827,#79828,#79829,#79830,#79831,
#79832,#79833,#79834,#79835,#79836,#79837),.UNSPECIFIED.,.F.,.F.,(4,3,3,
3,3,3,3,4),(0.,0.000855980888566154,0.00166641330334462,0.00241857507887524,
0.00314395788179104,0.00384525579784931,0.00451678851924274,0.0046334773523488),
 .UNSPECIFIED.);
#2150=B_SPLINE_CURVE_WITH_KNOTS('',3,(#79882,#79883,#79884,#79885,#79886,
#79887,#79888,#79889,#79890,#79891,#79892,#79893,#79894,#79895,#79896,#79897,
#79898,#79899,#79900,#79901,#79902,#79903,#79904,#79905,#79906),
 .UNSPECIFIED.,.F.,.F.,(4,3,3,3,3,3,3,3,4),(-6.00000001243266E-8,0.000118874083410464,
0.00026625895319811,0.000560941736381697,0.00114958238230934,0.00232100875268056,
0.00261300899752845,0.003820437717179,0.00463423520310888),
 .UNSPECIFIED.);
#2151=B_SPLINE_CURVE_WITH_KNOTS('',3,(#79909,#79910,#79911,#79912,#79913,
#79914),.UNSPECIFIED.,.F.,.F.,(4,2,4),(0.00373703492180183,0.0175573755935873,
0.0313777749446053),.UNSPECIFIED.);
#2152=B_SPLINE_CURVE_WITH_KNOTS('',3,(#79916,#79917,#79918,#79919,#79920,
#79921,#79922),.UNSPECIFIED.,.F.,.F.,(4,3,4),(0.,0.00190419423264558,0.00234423638057238),
 .UNSPECIFIED.);
#2153=B_SPLINE_CURVE_WITH_KNOTS('',3,(#79926,#79927,#79928,#79929),
 .UNSPECIFIED.,.F.,.F.,(4,4),(0.,0.00234424630178264),.UNSPECIFIED.);
#2154=B_SPLINE_CURVE_WITH_KNOTS('',3,(#79930,#79931,#79932,#79933,#79934,
#79935),.UNSPECIFIED.,.F.,.F.,(4,2,4),(0.00236563017817001,0.0161860243951214,
0.0300063042511233),.UNSPECIFIED.);
#2155=B_SPLINE_CURVE_WITH_KNOTS('',3,(#80015,#80016,#80017,#80018,#80019,
#80020,#80021,#80022,#80023,#80024,#80025,#80026,#80027,#80028,#80029,#80030,
#80031,#80032,#80033,#80034,#80035,#80036,#80037,#80038,#80039,#80040,#80041,
#80042,#80043,#80044,#80045,#80046,#80047,#80048,#80049,#80050,#80051,#80052,
#80053,#80054,#80055,#80056,#80057,#80058,#80059,#80060,#80061,#80062,#80063,
#80064,#80065,#80066,#80067,#80068,#80069,#80070,#80071,#80072,#80073,#80074,
#80075,#80076,#80077,#80078,#80079,#80080,#80081,#80082,#80083,#80084,#80085,
#80086,#80087,#80088,#80089,#80090,#80091,#80092,#80093,#80094,#80095,#80096,
#80097,#80098,#80099,#80100,#80101,#80102,#80103,#80104,#80105,#80106,#80107,
#80108,#80109,#80110,#80111,#80112,#80113,#80114,#80115,#80116,#80117,#80118,
#80119,#80120,#80121,#80122,#80123,#80124,#80125,#80126,#80127,#80128,#80129),
 .UNSPECIFIED.,.F.,.F.,(4,3,3,3,3,3,3,3,3,3,3,3,3,3,3,3,3,3,3,3,3,3,3,3,
3,3,3,3,3,3,3,3,3,3,3,3,3,3,4),(0.00311905352256314,0.0053801116275994,
0.00602984295399501,0.00807521049387905,0.00859175969223719,0.0109929812518547,
0.0120513367482218,0.0140644658619112,0.0165539281004915,0.0180279533176651,
0.0195371720315853,0.0213524177914092,0.0222735251164223,0.0239416797884228,
0.0250098782012593,0.0268439228031144,0.0286311930298163,0.0297781443204118,
0.0304825843709334,0.0326614314275284,0.0332189374557705,0.0342821935385057,
0.0345871139981891,0.0355175999826488,0.0359552905406078,0.0371490638991439,
0.03834283725768,0.0394975346329774,0.0406635361544574,0.0411512932950454,
0.0414279967102819,0.0423661024051587,0.0433094733853823,0.0439784633754719,
0.0441643497951191,0.0449939343403188,0.0457876834631741,0.0465442361737627,
0.0469007028799563),.UNSPECIFIED.);
#2156=B_SPLINE_CURVE_WITH_KNOTS('',3,(#80131,#80132,#80133,#80134,#80135,
#80136,#80137,#80138,#80139,#80140,#80141,#80142,#80143,#80144,#80145,#80146,
#80147,#80148,#80149,#80150,#80151,#80152,#80153,#80154,#80155,#80156,#80157,
#80158,#80159,#80160,#80161,#80162,#80163,#80164,#80165,#80166,#80167,#80168,
#80169,#80170,#80171,#80172,#80173,#80174,#80175,#80176,#80177,#80178,#80179,
#80180,#80181,#80182,#80183,#80184,#80185,#80186,#80187,#80188,#80189,#80190,
#80191,#80192,#80193,#80194,#80195,#80196,#80197,#80198,#80199,#80200,#80201,
#80202,#80203,#80204,#80205,#80206,#80207,#80208,#80209,#80210,#80211,#80212,
#80213,#80214,#80215,#80216,#80217,#80218,#80219,#80220,#80221,#80222,#80223,
#80224,#80225,#80226,#80227,#80228,#80229,#80230,#80231,#80232,#80233,#80234,
#80235,#80236,#80237,#80238,#80239,#80240,#80241,#80242,#80243,#80244,#80245,
#80246,#80247,#80248,#80249,#80250,#80251,#80252,#80253,#80254,#80255,#80256,
#80257),.UNSPECIFIED.,.F.,.F.,(4,3,3,3,3,3,3,3,3,3,3,3,3,3,3,3,3,3,3,3,
3,3,3,3,3,3,3,3,3,3,3,3,3,3,3,3,3,3,3,3,3,3,4),(0.,0.000768003065203817,
0.00156145589592255,0.00241145844771756,0.00290679751418499,0.00294209519057979,
0.00392936817884266,0.0049005686379947,0.00578940001938904,0.00581359502836999,
0.00691978270676153,0.00802064641753534,0.00861020326582181,0.00872039254255498,
0.00999358199255706,0.011283185442689,0.0114371426134103,0.01162719005674,
0.0129550959660898,0.0142810553350758,0.0157391861777158,0.0171489834289433,
0.01744078508511,0.0191831843701593,0.0210590838955528,0.0229349834209464,
0.0232543801134799,0.0252635651010464,0.0273699950355587,0.028769893630631,
0.0290679751418499,0.0320087732834693,0.0346366633260412,0.0348815701702199,
0.0373829744484225,0.0398598781887525,0.0405367165403877,0.0406951651985899,
0.0429951987229959,0.0435089813873852,0.0436019627127749,0.0450961502804854,
0.0465087602269599),.UNSPECIFIED.);
#2157=B_SPLINE_CURVE_WITH_KNOTS('',3,(#80332,#80333,#80334,#80335,#80336,
#80337,#80338,#80339,#80340,#80341,#80342,#80343,#80344,#80345,#80346,#80347,
#80348,#80349,#80350,#80351,#80352,#80353,#80354,#80355,#80356,#80357,#80358,
#80359,#80360,#80361,#80362,#80363,#80364,#80365,#80366,#80367,#80368,#80369,
#80370,#80371,#80372,#80373,#80374,#80375,#80376,#80377,#80378,#80379,#80380,
#80381,#80382,#80383,#80384,#80385,#80386,#80387,#80388,#80389,#80390,#80391,
#80392,#80393,#80394,#80395,#80396,#80397,#80398,#80399,#80400,#80401,#80402,
#80403,#80404,#80405,#80406,#80407,#80408,#80409,#80410,#80411,#80412,#80413,
#80414,#80415,#80416,#80417,#80418,#80419,#80420,#80421,#80422,#80423,#80424,
#80425,#80426,#80427,#80428,#80429,#80430,#80431,#80432,#80433,#80434,#80435,
#80436,#80437,#80438,#80439,#80440,#80441,#80442,#80443,#80444,#80445,#80446,
#80447,#80448,#80449),.UNSPECIFIED.,.F.,.F.,(4,3,3,3,3,3,3,3,3,3,3,3,3,
3,3,3,3,3,3,3,3,3,3,3,3,3,3,3,3,3,3,3,3,3,3,3,3,3,3,4),(0.,0.000726143059507885,
0.00147913467854374,0.00229201659693578,0.00272869752028247,0.00289529540141928,
0.00384720949917479,0.00478654822520129,0.00545739504056494,0.00570254014808291,
0.00675424881063688,0.00778705433857549,0.00818609256084741,0.00849911281909295,
0.00934447282246815,0.00955044132098881,0.0104584755543277,0.0109147900811302,
0.0113219360486972,0.0135942089848239,0.0157324884413447,0.0163721851216964,
0.0170495208719571,0.0188101707222918,0.0206158981728578,0.0218295801622627,
0.0228747183578681,0.0245582776825458,0.0263139312909912,0.0272869752028289,
0.02877680882973,0.0313209150461057,0.032744370243395,0.0347410550859414,
0.037138016640503,0.0382017652839612,0.0403769928727384,0.0407493932180728,
0.0431136999609109,0.0436591603245274),.UNSPECIFIED.);
#2158=B_SPLINE_CURVE_WITH_KNOTS('',3,(#80452,#80453,#80454,#80455,#80456,
#80457,#80458,#80459,#80460,#80461,#80462,#80463,#80464,#80465,#80466,#80467,
#80468,#80469,#80470,#80471,#80472,#80473,#80474,#80475,#80476,#80477,#80478,
#80479,#80480,#80481,#80482,#80483,#80484,#80485,#80486,#80487,#80488,#80489,
#80490,#80491,#80492,#80493,#80494,#80495,#80496,#80497,#80498,#80499,#80500,
#80501,#80502,#80503,#80504,#80505,#80506,#80507,#80508,#80509,#80510,#80511,
#80512,#80513,#80514,#80515,#80516,#80517,#80518,#80519,#80520,#80521,#80522,
#80523,#80524,#80525,#80526,#80527,#80528,#80529,#80530,#80531,#80532,#80533,
#80534,#80535,#80536,#80537,#80538,#80539,#80540,#80541,#80542,#80543,#80544,
#80545,#80546,#80547,#80548,#80549,#80550,#80551,#80552,#80553,#80554,#80555,
#80556,#80557,#80558,#80559,#80560,#80561,#80562,#80563,#80564,#80565,#80566,
#80567,#80568,#80569,#80570,#80571,#80572,#80573,#80574,#80575,#80576,#80577,
#80578,#80579,#80580,#80581),.UNSPECIFIED.,.F.,.F.,(4,3,3,3,3,3,3,3,3,3,
3,3,3,3,3,3,3,3,3,3,3,3,3,3,3,3,3,3,3,3,3,3,3,3,3,3,3,3,3,3,3,3,3,4),(0.,
0.0014880631106233,0.00289325796053988,0.00298895696726662,0.00546149369419472,
0.00578651592107976,0.00595032476225151,0.00839147043197193,0.0108596509061964,
0.0115730318421595,0.0118288390287403,0.014754677083364,0.0173595477632393,
0.0176745278189992,0.0196969647367931,0.0216224066731238,0.0231460636843191,
0.0234885065984452,0.0252834612916259,0.0271080204485124,0.0287938721334718,
0.0289325796053988,0.0292532769261303,0.030987394920195,0.0326942847566698,
0.0343658661896815,0.0347190955264786,0.034944203878361,0.035728171147985,
0.0361657245067487,0.0376123534870188,0.0377582145051172,0.0387818159471292,
0.0398198044369845,0.0405056114475593,0.0405598044644439,0.0415184848666389,
0.0425122980456137,0.0433815323903777,0.0433988694080998,0.0442301226091971,
0.0450135032249515,0.0457477991098854,0.0462921273686404),.UNSPECIFIED.);
#2159=B_SPLINE_CURVE_WITH_KNOTS('',3,(#80715,#80716,#80717,#80718,#80719,
#80720,#80721,#80722,#80723,#80724,#80725,#80726,#80727,#80728,#80729,#80730,
#80731,#80732,#80733,#80734,#80735,#80736,#80737,#80738,#80739,#80740,#80741,
#80742,#80743,#80744,#80745,#80746,#80747,#80748,#80749,#80750,#80751,#80752,
#80753,#80754,#80755,#80756,#80757,#80758,#80759,#80760,#80761,#80762,#80763,
#80764,#80765,#80766,#80767,#80768,#80769,#80770,#80771,#80772,#80773,#80774,
#80775,#80776,#80777,#80778,#80779,#80780,#80781,#80782,#80783,#80784,#80785,
#80786,#80787,#80788,#80789,#80790,#80791,#80792,#80793,#80794,#80795,#80796,
#80797,#80798,#80799,#80800,#80801,#80802,#80803,#80804,#80805,#80806,#80807,
#80808,#80809,#80810,#80811,#80812,#80813,#80814,#80815,#80816,#80817,#80818,
#80819,#80820,#80821,#80822,#80823,#80824,#80825,#80826,#80827,#80828,#80829,
#80830,#80831,#80832,#80833,#80834,#80835,#80836,#80837,#80838,#80839,#80840,
#80841,#80842,#80843,#80844,#80845,#80846,#80847,#80848,#80849,#80850,#80851,
#80852,#80853,#80854,#80855,#80856,#80857,#80858,#80859,#80860,#80861,#80862,
#80863,#80864,#80865,#80866,#80867,#80868,#80869,#80870,#80871,#80872,#80873,
#80874,#80875,#80876,#80877,#80878,#80879,#80880,#80881,#80882,#80883,#80884,
#80885,#80886,#80887,#80888,#80889,#80890,#80891,#80892,#80893,#80894,#80895,
#80896,#80897,#80898,#80899,#80900,#80901,#80902,#80903,#80904,#80905,#80906,
#80907,#80908,#80909,#80910,#80911,#80912,#80913),.UNSPECIFIED.,.F.,.F.,
(4,3,3,3,3,3,3,3,3,3,3,3,3,3,3,3,3,3,3,3,3,3,3,3,3,3,3,3,3,3,3,3,3,3,3,
3,3,3,3,3,3,3,3,3,3,3,3,3,3,3,3,3,3,3,3,3,3,3,3,3,3,3,3,3,3,3,4),(-5.59795119973968E-8,
3.77153166948725E-5,5.42420177488181E-5,0.000132553837957507,0.000150709093707369,
0.000302142533558002,0.000604345067115865,0.000786478784293366,0.0012087501342316,
0.00205947175303894,0.00241756026846307,0.00432788328869313,0.00460569556319153,
0.00483518053692602,0.00765167798628207,0.0096704210738519,0.00968212413977662,
0.0121986817239082,0.0147309548882147,0.0172905697838751,0.0193409021477037,
0.0197246627808341,0.0225497079721102,0.0254165723872828,0.0283511952458422,
0.0290113832215555,0.0296334023415766,0.032598479695546,0.0356401719954766,
0.0384990492010592,0.0386818642954072,0.0394311552495718,0.0420390225446679,
0.0435171048323331,0.0442854463712337,0.0465596741328543,0.048352345369259,
0.0491025292327438,0.0511450575694643,0.0530508480161911,0.0531875859061849,
0.0538733380029565,0.0557095849073245,0.0575121872200063,0.0580228264431107,
0.0585879878559654,0.0604404467115735,0.0609228364106318,0.0616492568458051,
0.0628580669800366,0.0632453611893526,0.0645539017016228,0.0658671302108557,
0.0671869467768509,0.0676933075169628,0.0678750498154547,0.0692097954598117,
0.0705855751610864,0.0720100465266797,0.0725285480538889,0.0725479710459296,
0.0738436643829537,0.0749312406649937,0.0749461683223518,0.0759822319304995,
0.0769769212816998,0.0773637885908147),.UNSPECIFIED.);
#2160=B_SPLINE_CURVE_WITH_KNOTS('',3,(#81049,#81050,#81051,#81052,#81053,
#81054,#81055,#81056,#81057,#81058,#81059,#81060,#81061,#81062,#81063,#81064,
#81065,#81066,#81067,#81068,#81069,#81070,#81071,#81072,#81073,#81074,#81075,
#81076,#81077,#81078,#81079,#81080,#81081,#81082,#81083,#81084,#81085,#81086,
#81087,#81088),.UNSPECIFIED.,.F.,.F.,(4,2,2,2,2,2,2,2,2,2,2,2,2,2,2,2,2,
2,2,4),(0.,0.00488270447985229,0.00732405671977861,0.00976540895970492,
0.0146481134395579,0.0170894656794843,0.0183101417994474,0.0195308179194105,
0.0244135223992626,0.0292962268791146,0.0341789313589667,0.0390616358388187,
0.0488270447985229,0.058592453758227,0.0683578627179311,0.073240567197783,
0.0756819194377091,0.0769025955576723,0.0775129336176539,0.0781232716776354),
 .UNSPECIFIED.);
#2161=B_SPLINE_CURVE_WITH_KNOTS('',3,(#81092,#81093,#81094,#81095,#81096,
#81097,#81098,#81099,#81100,#81101,#81102,#81103,#81104,#81105,#81106,#81107,
#81108,#81109,#81110,#81111,#81112,#81113,#81114,#81115,#81116,#81117,#81118,
#81119,#81120,#81121,#81122,#81123,#81124,#81125,#81126,#81127,#81128,#81129,
#81130,#81131,#81132,#81133,#81134,#81135,#81136,#81137,#81138,#81139,#81140,
#81141,#81142,#81143,#81144,#81145,#81146,#81147,#81148,#81149,#81150,#81151,
#81152,#81153,#81154,#81155,#81156,#81157,#81158,#81159,#81160,#81161,#81162,
#81163,#81164,#81165,#81166,#81167,#81168,#81169,#81170,#81171,#81172,#81173,
#81174,#81175,#81176,#81177,#81178,#81179,#81180,#81181,#81182,#81183,#81184,
#81185,#81186,#81187,#81188,#81189,#81190,#81191,#81192,#81193,#81194,#81195,
#81196,#81197,#81198,#81199,#81200,#81201,#81202,#81203,#81204,#81205,#81206,
#81207,#81208,#81209,#81210,#81211,#81212,#81213,#81214,#81215,#81216,#81217,
#81218,#81219,#81220,#81221,#81222,#81223,#81224,#81225,#81226,#81227,#81228,
#81229,#81230,#81231,#81232,#81233,#81234,#81235,#81236,#81237,#81238,#81239,
#81240,#81241,#81242,#81243,#81244,#81245,#81246,#81247,#81248,#81249,#81250,
#81251,#81252,#81253,#81254,#81255,#81256,#81257,#81258,#81259,#81260,#81261,
#81262,#81263,#81264,#81265,#81266,#81267,#81268,#81269,#81270,#81271,#81272,
#81273,#81274,#81275,#81276,#81277,#81278,#81279,#81280,#81281,#81282,#81283,
#81284,#81285,#81286,#81287,#81288,#81289,#81290,#81291,#81292,#81293,#81294,
#81295,#81296,#81297,#81298,#81299,#81300,#81301,#81302,#81303,#81304,#81305,
#81306,#81307,#81308,#81309,#81310,#81311,#81312,#81313,#81314,#81315,#81316,
#81317,#81318,#81319,#81320,#81321,#81322,#81323,#81324,#81325,#81326,#81327,
#81328,#81329,#81330,#81331,#81332,#81333,#81334,#81335),.UNSPECIFIED.,
 .F.,.F.,(4,3,3,3,3,3,3,3,3,3,3,3,3,3,3,3,3,3,3,3,3,3,3,3,3,3,3,3,3,3,3,
3,3,3,3,3,3,3,3,3,3,3,3,3,3,3,3,3,3,3,3,3,3,3,3,3,3,3,3,3,3,3,3,3,3,3,3,
3,3,3,3,3,3,3,3,3,3,3,3,3,3,4),(0.0138213625150584,0.0153557252057815,0.016967809312913,
0.0186005460987653,0.0203100782662155,0.0218040616343076,0.0236391782065667,
0.0256135223282299,0.0278020457228518,0.0297867607535567,0.0324211420232949,
0.0346222226998159,0.0366314376259851,0.0385183080194414,0.0402765202164955,
0.0419783697096923,0.0436039474387354,0.0449779475927287,0.0457521589920549,
0.0471616940402511,0.0485724556204019,0.0499853340506432,0.0513995226194317,
0.0528159415151625,0.0537348581113041,0.0551463951926526,0.0565385724899381,
0.0577262076709287,0.0590012271883266,0.060299813065953,0.0613266973480848,
0.0617175572305534,0.0633557013899515,0.0649958419736401,0.0666385396463259,
0.0682825571558663,0.0699276823934046,0.0715737010877966,0.0732206481682718,
0.0748679134463574,0.0765153305568312,0.0776771708855837,0.0776829554690519,
0.0798220465852468,0.0820269821662078,0.0841070044248161,0.0856656545883011,
0.0875503928177031,0.0892804802057929,0.0909480261844515,0.0925357499280549,
0.0936483537075503,0.0940287551521221,0.095402302693789,0.0968005776623906,
0.0982387635443414,0.0997005647312465,0.10119455705148,0.1016310528268,
0.103158876473257,0.10470000813583,0.105775168386768,0.10731195168399,0.107618077166237,
0.108766337718664,0.109613751946049,0.110371017456633,0.112612002482226,
0.11491420298544,0.117283745588801,0.119769286762534,0.122334997043814,
0.125039715440694,0.125579150184548,0.128267344839129,0.129570499744172,
0.131236775216371,0.132915090511205,0.133561849303797,0.136328208654542,
0.139188103873677,0.14154453702431),.UNSPECIFIED.);
#2162=B_SPLINE_CURVE_WITH_KNOTS('',3,(#81614,#81615,#81616,#81617),
 .UNSPECIFIED.,.F.,.F.,(4,4),(0.,0.00229184701740597),.UNSPECIFIED.);
#2163=B_SPLINE_CURVE_WITH_KNOTS('',3,(#81619,#81620,#81621,#81622,#81623,
#81624,#81625),.UNSPECIFIED.,.F.,.F.,(4,3,4),(-5.9999999698125E-8,0.00114592679117705,
0.0022919135823538),.UNSPECIFIED.);
#2164=B_SPLINE_CURVE_WITH_KNOTS('',3,(#81627,#81628,#81629,#81630,#81631,
#81632,#81633,#81634,#81635,#81636,#81637,#81638,#81639,#81640,#81641,#81642,
#81643,#81644,#81645,#81646,#81647,#81648,#81649,#81650,#81651,#81652,#81653,
#81654,#81655,#81656,#81657,#81658,#81659,#81660,#81661,#81662,#81663,#81664,
#81665,#81666,#81667,#81668,#81669,#81670,#81671,#81672,#81673,#81674,#81675,
#81676,#81677,#81678,#81679,#81680,#81681,#81682,#81683,#81684,#81685,#81686,
#81687,#81688,#81689,#81690,#81691,#81692,#81693,#81694,#81695,#81696,#81697,
#81698,#81699,#81700,#81701,#81702,#81703,#81704,#81705,#81706,#81707,#81708,
#81709,#81710,#81711,#81712,#81713,#81714,#81715,#81716,#81717,#81718,#81719,
#81720,#81721,#81722,#81723,#81724,#81725,#81726,#81727,#81728,#81729,#81730,
#81731,#81732,#81733,#81734,#81735,#81736,#81737,#81738,#81739,#81740,#81741,
#81742,#81743,#81744,#81745,#81746,#81747,#81748,#81749,#81750,#81751,#81752,
#81753,#81754,#81755,#81756,#81757,#81758,#81759,#81760,#81761,#81762,#81763,
#81764,#81765,#81766,#81767,#81768,#81769,#81770,#81771,#81772,#81773,#81774,
#81775,#81776,#81777),.UNSPECIFIED.,.F.,.F.,(4,3,3,3,3,3,3,3,3,3,3,3,3,
3,3,3,3,3,3,3,3,3,3,3,3,3,3,3,3,3,3,3,3,3,3,3,3,3,3,3,3,3,3,3,3,3,3,3,3,
3,4),(0.,0.00254964314673973,0.00496070222628838,0.00501980874154407,0.00826545197487785,
0.00992140445257675,0.0100311925058059,0.0136136254161935,0.0174983629157502,
0.0198428089051537,0.0200323843653405,0.0251558497217403,0.0297642133577307,
0.0300168623559456,0.0348512400831266,0.0388899647682047,0.0396856178103077,
0.0399877547963082,0.0442724564177337,0.0446463200365963,0.044965125921608,
0.0478278095482398,0.0496070222628849,0.0499357590496292,0.0522517417694013,
0.0543924576210147,0.0545677244891735,0.0548913186057754,0.0568663425859277,
0.0587651627048331,0.0595284267154621,0.0598185736751817,0.0612486302751543,
0.0620087778286062,0.0622677632564443,0.0638697876314808,0.0644891289417504,
0.0647077384064401,0.0662847719523633,0.0678876752602966,0.0694498311680387,
0.0695699086585862,0.0710966014883998,0.0719301822811829,0.0720034895600447,
0.0734239213479113,0.074410533394327,0.0744472360436,0.0763835183275585,
0.077890280957556,0.079371235620615),.UNSPECIFIED.);
#2165=B_SPLINE_CURVE_WITH_KNOTS('',5,(#81779,#81780,#81781,#81782,#81783,
#81784,#81785,#81786,#81787,#81788,#81789,#81790,#81791,#81792,#81793,#81794,
#81795,#81796,#81797),.UNSPECIFIED.,.F.,.F.,(6,1,2,3,3,3,1,6),(0.026904580241564,
0.0624999999998681,0.124999999999887,0.249999999999925,0.500000000000001,
0.750000000000077,0.875000000000115,0.97309541975779),.UNSPECIFIED.);
#2166=B_SPLINE_CURVE_WITH_KNOTS('',3,(#81798,#81799,#81800,#81801,#81802,
#81803,#81804,#81805,#81806,#81807,#81808,#81809,#81810,#81811,#81812,#81813,
#81814,#81815,#81816,#81817,#81818,#81819,#81820,#81821,#81822,#81823,#81824,
#81825,#81826,#81827,#81828,#81829,#81830,#81831,#81832,#81833,#81834,#81835,
#81836,#81837,#81838,#81839,#81840,#81841,#81842,#81843,#81844,#81845,#81846,
#81847,#81848,#81849,#81850,#81851,#81852,#81853,#81854,#81855,#81856,#81857,
#81858,#81859,#81860,#81861,#81862,#81863,#81864,#81865,#81866,#81867,#81868,
#81869,#81870,#81871,#81872,#81873,#81874,#81875,#81876,#81877,#81878,#81879,
#81880,#81881,#81882,#81883,#81884,#81885,#81886,#81887,#81888,#81889,#81890,
#81891,#81892,#81893,#81894,#81895,#81896,#81897,#81898,#81899,#81900,#81901,
#81902,#81903,#81904,#81905,#81906,#81907,#81908,#81909,#81910,#81911,#81912,
#81913,#81914,#81915,#81916,#81917,#81918,#81919,#81920,#81921,#81922,#81923,
#81924,#81925,#81926,#81927,#81928,#81929,#81930,#81931,#81932,#81933,#81934,
#81935,#81936,#81937,#81938,#81939,#81940,#81941,#81942,#81943,#81944,#81945,
#81946,#81947,#81948,#81949,#81950,#81951,#81952,#81953,#81954,#81955,#81956,
#81957,#81958,#81959,#81960),.UNSPECIFIED.,.F.,.F.,(4,3,3,3,3,3,3,3,3,3,
3,3,3,3,3,3,3,3,3,3,3,3,3,3,3,3,3,3,3,3,3,3,3,3,3,3,3,3,3,3,3,3,3,3,3,3,
3,3,3,3,3,3,3,3,4),(0.,0.00140947603978418,0.0024756341357668,0.00248033423984031,
0.00401846206250739,0.00494329357891454,0.00495126827153361,0.00676698994228475,
0.00838410792447671,0.00982709094185986,0.00990253654306755,0.0114864206850264,
0.0130928099150335,0.0146991991450405,0.0148538048146015,0.0167010364617009,
0.0171457642489763,0.0173294389503683,0.0194739265126486,0.0196023111933348,
0.0198050730861351,0.0217052560346576,0.0236804462177422,0.0245443401511237,
0.0247563413576684,0.0269124535382796,0.0291847695784314,0.0295139096563174,
0.0297076096292018,0.0325507544885065,0.034497823346557,0.0346588779007351,
0.0378033430080754,0.0394883310170963,0.0396101461722684,0.0429789048814282,
0.0468219392681408,0.049498571171444,0.0495126827153351,0.0556179629347513,
0.0594152192584017,0.0595245880574298,0.0637007112342887,0.0643664875299352,
0.0666105083933754,0.0686940084843271,0.0693177558014686,0.0695562768533866,
0.0719529892403943,0.0742690240730021,0.0746112540765943,0.0771545039955694,
0.0784302024647239,0.0790690551790372,0.0792202923445355),.UNSPECIFIED.);
#2167=B_SPLINE_CURVE_WITH_KNOTS('',3,(#81962,#81963,#81964,#81965,#81966,
#81967,#81968,#81969,#81970,#81971,#81972,#81973,#81974,#81975,#81976,#81977,
#81978,#81979,#81980,#81981,#81982,#81983,#81984,#81985,#81986,#81987,#81988,
#81989,#81990,#81991,#81992,#81993,#81994,#81995,#81996,#81997,#81998),
 .UNSPECIFIED.,.F.,.F.,(4,3,3,3,3,3,3,3,3,3,3,3,4),(0.,0.0797408492149254,
0.161855164948292,0.248717931187981,0.338623906203558,0.432533374925927,
0.5,0.594371835892723,0.686236776709294,0.772607332273767,0.856209295506246,
0.93626015886546,1.),.UNSPECIFIED.);
#2168=B_SPLINE_CURVE_WITH_KNOTS('',3,(#82012,#82013,#82014,#82015,#82016,
#82017,#82018,#82019,#82020,#82021,#82022,#82023,#82024,#82025,#82026,#82027,
#82028,#82029,#82030,#82031,#82032,#82033,#82034,#82035,#82036,#82037,#82038,
#82039,#82040,#82041,#82042,#82043,#82044,#82045,#82046,#82047,#82048),
 .UNSPECIFIED.,.F.,.F.,(4,3,3,3,3,3,3,3,3,3,3,3,4),(0.,0.0797761540364943,
0.161934993682177,0.248863688029891,0.338853887792259,0.432867845144356,
0.5,0.594694033641728,0.686818625637526,0.773322404313094,0.857008887365513,
0.937104727272101,1.),.UNSPECIFIED.);
#2169=B_SPLINE_CURVE_WITH_KNOTS('',3,(#82147,#82148,#82149,#82150),
 .UNSPECIFIED.,.F.,.F.,(4,4),(0.,0.0994990093838759),.UNSPECIFIED.);
#2170=B_SPLINE_CURVE_WITH_KNOTS('',3,(#82151,#82152,#82153,#82154,#82155,
#82156,#82157),.UNSPECIFIED.,.F.,.F.,(4,3,4),(0.000501749122919644,0.0788687616003136,
0.100000758506779),.UNSPECIFIED.);
#2171=B_SPLINE_CURVE_WITH_KNOTS('',3,(#82285,#82286,#82287,#82288,#82289,
#82290,#82291,#82292,#82293,#82294,#82295,#82296,#82297,#82298,#82299,#82300,
#82301,#82302,#82303,#82304,#82305,#82306,#82307,#82308,#82309,#82310,#82311,
#82312,#82313,#82314,#82315,#82316,#82317,#82318,#82319,#82320,#82321),
 .UNSPECIFIED.,.F.,.F.,(4,3,3,3,3,3,3,3,3,3,3,3,4),(0.,0.0798162266516071,
0.161952526089989,0.248677675875237,0.338294947140869,0.431635010482063,
0.5,0.593343691841967,0.684478682447239,0.770593179237603,0.854107271329051,
0.934207928070758,1.),.UNSPECIFIED.);
#2172=B_SPLINE_CURVE_WITH_KNOTS('',3,(#82346,#82347,#82348,#82349),
 .UNSPECIFIED.,.F.,.F.,(4,4),(0.000501748999621204,0.100000733467173),
 .UNSPECIFIED.);
#2173=B_SPLINE_CURVE_WITH_KNOTS('',3,(#82350,#82351,#82352,#82353,#82354,
#82355,#82356),.UNSPECIFIED.,.F.,.F.,(4,3,4),(0.,0.0156807264631829,0.0994990093838759),
 .UNSPECIFIED.);
#2174=B_SPLINE_CURVE_WITH_KNOTS('',3,(#82370,#82371,#82372,#82373),
 .UNSPECIFIED.,.F.,.F.,(4,4),(0.000501749122919617,0.100000758506779),
 .UNSPECIFIED.);
#2175=B_SPLINE_CURVE_WITH_KNOTS('',3,(#82374,#82375,#82376,#82377),
 .UNSPECIFIED.,.F.,.F.,(4,4),(0.,0.0994989844675695),.UNSPECIFIED.);
#2176=B_SPLINE_CURVE_WITH_KNOTS('',3,(#82390,#82391,#82392,#82393),
 .UNSPECIFIED.,.F.,.F.,(4,4),(0.000501748999621204,0.100000733467173),
 .UNSPECIFIED.);
#2177=B_SPLINE_CURVE_WITH_KNOTS('',3,(#82406,#82407,#82408,#82409),
 .UNSPECIFIED.,.F.,.F.,(4,4),(0.,0.0994989844675695),.UNSPECIFIED.);
#2178=B_SPLINE_CURVE_WITH_KNOTS('',3,(#82475,#82476,#82477,#82478,#82479,
#82480,#82481,#82482,#82483,#82484,#82485,#82486,#82487,#82488,#82489,#82490,
#82491,#82492,#82493,#82494,#82495,#82496,#82497,#82498,#82499,#82500,#82501,
#82502,#82503,#82504,#82505,#82506,#82507,#82508,#82509,#82510,#82511,#82512,
#82513,#82514,#82515,#82516,#82517,#82518,#82519,#82520,#82521,#82522,#82523,
#82524,#82525,#82526,#82527,#82528,#82529,#82530,#82531,#82532,#82533,#82534,
#82535,#82536,#82537,#82538,#82539,#82540,#82541,#82542,#82543,#82544,#82545,
#82546,#82547,#82548,#82549,#82550,#82551,#82552,#82553,#82554,#82555,#82556,
#82557,#82558,#82559,#82560,#82561,#82562,#82563,#82564,#82565,#82566,#82567,
#82568,#82569,#82570,#82571,#82572,#82573,#82574,#82575,#82576,#82577,#82578,
#82579,#82580,#82581,#82582,#82583,#82584,#82585,#82586,#82587,#82588,#82589,
#82590,#82591,#82592,#82593,#82594,#82595,#82596,#82597,#82598,#82599,#82600,
#82601,#82602,#82603,#82604,#82605,#82606,#82607,#82608,#82609,#82610,#82611,
#82612,#82613,#82614,#82615,#82616,#82617,#82618,#82619,#82620,#82621,#82622,
#82623,#82624,#82625,#82626,#82627,#82628,#82629,#82630,#82631,#82632,#82633,
#82634,#82635,#82636,#82637,#82638,#82639,#82640,#82641,#82642,#82643,#82644,
#82645,#82646,#82647,#82648,#82649,#82650,#82651,#82652,#82653,#82654,#82655,
#82656,#82657,#82658,#82659,#82660,#82661),.UNSPECIFIED.,.F.,.F.,(4,3,3,
3,3,3,3,3,3,3,3,3,3,3,3,3,3,3,3,3,3,3,3,3,3,3,3,3,3,3,3,3,3,3,3,3,3,3,3,
3,3,3,3,3,3,3,3,3,3,3,3,3,3,3,3,3,3,3,3,3,3,3,4),(0.,0.00129806474652078,
0.00173826111454353,0.00175748537690092,0.00253439280672143,0.00260848340217944,
0.00263622806535153,0.00347971001178824,0.00351497075380215,0.00459045036182651,
0.00522713955700752,0.00527245613070368,0.00593919936703502,0.00610334028621381,
0.00615119881915445,0.00698136154947715,0.00702994150760521,0.00761773897739526,
0.00790868419605598,0.00836503337917805,0.00874285200622063,0.00878742688450675,
0.0102952263202082,0.0105106640972962,0.0105449122614081,0.0113430190056926,
0.0113966380311906,0.0114236549498588,0.0122838726044989,0.0123023976383095,
0.0140595560052317,0.0140598830152109,0.014764174565025,0.0149386257036616,
0.0149478752944383,0.0158173683921124,0.0158357198344066,0.0169081214885754,
0.0175748537690138,0.0176088189027247,0.0187941931735089,0.0193323391459153,
0.0193769020438058,0.0202110818343661,0.020258524249687,0.0209265199003004,
0.021089824522817,0.0211384645734138,0.0221119423053973,0.0228473098997184,
0.022892870910804,0.0236593526447152,0.0237260525881691,0.0237673174050347,
0.0246047952766199,0.0246402836506722,0.0258895920454538,0.0263622806535216,
0.0263820780204341,0.0268115506812034,0.0272410233419727,0.0276803946861982,
0.0281197660304237),.UNSPECIFIED.);
#2179=B_SPLINE_CURVE_WITH_KNOTS('',3,(#82776,#82777,#82778,#82779,#82780,
#82781,#82782,#82783,#82784,#82785,#82786,#82787,#82788,#82789,#82790,#82791,
#82792,#82793,#82794,#82795,#82796,#82797,#82798,#82799,#82800,#82801,#82802,
#82803,#82804,#82805,#82806,#82807,#82808,#82809,#82810,#82811,#82812,#82813),
 .UNSPECIFIED.,.F.,.F.,(4,2,2,2,2,2,2,2,2,2,2,2,2,2,2,2,2,2,4),(1.69183768239892E-7,
0.0048773097517895,0.00975461950357901,0.0146319292553685,0.019509239007158,
0.0219478938830527,0.0243865487589474,0.0292638585107367,0.034141168262526,
0.0390184780143152,0.0414571328902099,0.0438957877661045,0.0487730975178938,
0.0536504072696831,0.0585277170214724,0.0634050267732618,0.0682823365250511,
0.0731596462768404,0.078036786716835),.UNSPECIFIED.);
#2180=B_SPLINE_CURVE_WITH_KNOTS('',3,(#83066,#83067,#83068,#83069,#83070,
#83071,#83072,#83073,#83074,#83075,#83076,#83077,#83078,#83079,#83080,#83081,
#83082,#83083,#83084,#83085,#83086,#83087,#83088,#83089,#83090),
 .UNSPECIFIED.,.F.,.F.,(4,3,3,3,3,3,3,3,4),(0.0299184616875247,0.0303501458310297,
0.0337269825420159,0.0352479488762528,0.037103821794114,0.0379126924706169,
0.0387922400745739,0.0404806582791753,0.0405774360649809),.UNSPECIFIED.);
#2181=B_SPLINE_CURVE_WITH_KNOTS('',3,(#83091,#83092,#83093,#83094,#83095,
#83096,#83097,#83098,#83099,#83100,#83101,#83102,#83103,#83104,#83105,#83106),
 .UNSPECIFIED.,.F.,.F.,(4,3,3,3,3,4),(0.0170041804055748,0.0202196292169069,
0.0221201639002461,0.0235964706859312,0.0269733085854605,0.0272361473949173),
 .UNSPECIFIED.);
#2182=B_SPLINE_CURVE_WITH_KNOTS('',3,(#83107,#83108,#83109,#83110,#83111,
#83112,#83113,#83114,#83115,#83116,#83117,#83118,#83119,#83120,#83121,#83122,
#83123,#83124,#83125,#83126,#83127,#83128,#83129,#83130,#83131,#83132,#83133,
#83134,#83135,#83136,#83137,#83138,#83139,#83140,#83141,#83142,#83143,#83144,
#83145,#83146,#83147,#83148,#83149,#83150,#83151,#83152,#83153,#83154,#83155,
#83156,#83157,#83158,#83159,#83160,#83161,#83162,#83163,#83164,#83165,#83166,
#83167,#83168,#83169,#83170,#83171,#83172,#83173,#83174,#83175,#83176),
 .UNSPECIFIED.,.F.,.F.,(4,3,3,3,3,3,3,3,3,3,3,3,3,3,3,3,3,3,3,3,3,3,3,4),
(0.0019251675425492,0.00334378906625673,0.00447186156832812,0.00493983969368741,
0.00502452477533919,0.00586801927215848,0.00644718237437487,0.00671228437311717,
0.00755649345598186,0.00795452505506233,0.00840082127134725,0.00882308249445703,
0.00924513359857515,0.00946186773574978,0.00966686202115364,0.0100888830220607,
0.0108460286904892,0.0109333300155275,0.0109692104164372,0.0117775399721665,
0.0124765530971247,0.0126217496304117,0.0134659578750993,0.0139838957778122),
 .UNSPECIFIED.);
#2183=B_SPLINE_CURVE_WITH_KNOTS('',3,(#83177,#83178,#83179,#83180,#83181,
#83182,#83183,#83184,#83185,#83186,#83187,#83188,#83189,#83190,#83191,#83192,
#83193,#83194,#83195,#83196,#83197,#83198,#83199,#83200,#83201,#83202,#83203,
#83204,#83205,#83206,#83207,#83208,#83209,#83210,#83211,#83212,#83213,#83214,
#83215,#83216,#83217,#83218,#83219,#83220,#83221,#83222,#83223,#83224,#83225,
#83226,#83227,#83228,#83229,#83230,#83231,#83232,#83233,#83234,#83235,#83236,
#83237,#83238,#83239,#83240,#83241,#83242,#83243,#83244,#83245,#83246,#83247,
#83248,#83249,#83250,#83251,#83252,#83253,#83254,#83255,#83256,#83257,#83258,
#83259,#83260,#83261,#83262,#83263,#83264,#83265,#83266,#83267,#83268,#83269,
#83270,#83271,#83272,#83273,#83274,#83275,#83276,#83277,#83278,#83279,#83280,
#83281,#83282,#83283,#83284,#83285,#83286,#83287,#83288,#83289,#83290,#83291,
#83292,#83293,#83294,#83295,#83296,#83297,#83298,#83299,#83300,#83301,#83302,
#83303,#83304,#83305,#83306,#83307,#83308,#83309,#83310,#83311,#83312,#83313,
#83314,#83315,#83316,#83317,#83318,#83319,#83320,#83321,#83322,#83323,#83324,
#83325,#83326,#83327,#83328,#83329,#83330,#83331,#83332,#83333,#83334,#83335,
#83336,#83337,#83338,#83339,#83340,#83341,#83342,#83343,#83344,#83345,#83346,
#83347,#83348,#83349,#83350,#83351,#83352,#83353,#83354,#83355,#83356,#83357,
#83358,#83359,#83360,#83361,#83362,#83363,#83364,#83365,#83366,#83367,#83368,
#83369,#83370,#83371,#83372,#83373,#83374,#83375,#83376,#83377,#83378,#83379,
#83380,#83381,#83382,#83383,#83384,#83385,#83386,#83387,#83388,#83389,#83390,
#83391,#83392,#83393,#83394,#83395,#83396,#83397,#83398,#83399,#83400,#83401,
#83402,#83403,#83404,#83405,#83406,#83407,#83408,#83409,#83410,#83411,#83412,
#83413,#83414,#83415,#83416,#83417,#83418,#83419,#83420,#83421,#83422,#83423,
#83424,#83425,#83426,#83427,#83428,#83429,#83430,#83431,#83432),
 .UNSPECIFIED.,.F.,.F.,(4,3,3,3,3,3,3,3,3,3,3,3,3,3,3,3,3,3,3,3,3,3,3,3,
3,3,3,3,3,3,3,3,3,3,3,3,3,3,3,3,3,3,3,3,3,3,3,3,3,3,3,3,3,3,3,3,3,3,3,3,
3,3,3,3,3,3,3,3,3,3,3,3,3,3,3,3,3,3,3,3,3,3,3,3,3,4),(0.,0.000671271444715106,
0.00133573398492509,0.00199656612730211,0.00267564160261107,0.00334004269519932,
0.00402645536186862,0.00471286802853793,0.00547920794335988,0.00628429962118388,
0.00716079437273603,0.00808586384770316,0.00908883320141247,0.00942573605707585,
0.0104652026191,0.0115317045578357,0.0126000266263672,0.013666613817005,
0.0141386040856138,0.0151515096840178,0.0161699677133158,0.0171934455273772,
0.018228269718743,0.0188514721141517,0.0197328956913815,0.0206287034168766,
0.0212079061284207,0.0222544789108859,0.0233470560080171,0.0235643401426896,
0.0246626218613768,0.0258454200191195,0.0271492080637942,0.0282772081712275,
0.0296408732222399,0.030981969144124,0.0322417032554741,0.0329900761997653,
0.0341682932068998,0.0352934947584113,0.0363996004210637,0.0374869166232296,
0.0377029442283032,0.0378307562325676,0.0389450672375698,0.0400593782425721,
0.0410084966162602,0.0419734390593707,0.0424158122568411,0.0436667633990814,
0.0449613146661833,0.046274937431326,0.0471286802853789,0.048395788287793,
0.0495938760100985,0.0507177121620077,0.0518415483139168,0.0529519305126435,
0.0540079497098051,0.0550392316356208,0.0560406255956614,0.0565544163424547,
0.0575733034733135,0.0585697691399218,0.0589108503567236,0.0597776382715151,
0.0606400134853726,0.0612672843709925,0.0623243005149662,0.0633870339544853,
0.0644492360151451,0.0654931261235198,0.0659801523995304,0.0669869888480002,
0.0679134967430172,0.0687682851712823,0.0695816398702095,0.0703432939240617,
0.0706930204280682,0.0713654965182033,0.0720302304898885,0.0726900854517225,
0.0733690266256629,0.0740291640074781,0.074717507077481,0.0754058501474839),
 .UNSPECIFIED.);
#2184=B_SPLINE_CURVE_WITH_KNOTS('',3,(#83433,#83434,#83435,#83436,#83437,
#83438,#83439,#83440,#83441,#83442,#83443,#83444,#83445,#83446,#83447,#83448,
#83449,#83450,#83451,#83452,#83453,#83454),.UNSPECIFIED.,.F.,.F.,(4,3,3,
3,3,3,3,4),(0.0477477555525722,0.0480785186018883,0.0489227697563253,0.0493078116841327,
0.0506111708367689,0.0508678770957731,0.0522995954683137,0.0539880079190539),
 .UNSPECIFIED.);
#2185=B_SPLINE_CURVE_WITH_KNOTS('',3,(#83455,#83456,#83457,#83458,#83459,
#83460,#83461,#83462,#83463,#83464,#83465,#83466,#83467,#83468,#83469,#83470,
#83471,#83472,#83473,#83474,#83475,#83476,#83477,#83478,#83479,#83480,#83481,
#83482,#83483,#83484,#83485,#83486,#83487,#83488),.UNSPECIFIED.,.F.,.F.,
(4,3,3,3,3,3,3,3,3,3,3,4),(0.0416412057894145,0.0421690766487205,0.0427185744702001,
0.0430132854152916,0.0437959431509857,0.0438574958856639,0.0442796014294634,
0.0447017045928652,0.0448733118317713,0.0451238084081384,0.0455459138152578,
0.0459506805125569),.UNSPECIFIED.);
#2908=ORIENTED_CLOSED_SHELL('',*,#45449,.F.);
#2909=ORIENTED_CLOSED_SHELL('',*,#45450,.F.);
#2912=ELLIPSE('',#45570,8.34154176961301,8.30313896599411);
#2913=ELLIPSE('',#45577,8.31271199747688,8.30313896599411);
#2914=ELLIPSE('',#45578,8.3415417696134,8.3031389659941);
#2915=ELLIPSE('',#47457,8.31271199747759,8.3031389659941);
#2916=ELLIPSE('',#47528,19.6143071532144,16.9851908864685);
#2917=ELLIPSE('',#47529,19.614307153188,16.9851908864196);
#2918=BREP_WITH_VOIDS('Body1',#45451,(#2908,#2909));
#2921=SHAPE_REPRESENTATION_RELATIONSHIP('SRR','None',#130943,#2929);
#2929=ADVANCED_BREP_SHAPE_REPRESENTATION('',(#2918),#130903);
#2937=STYLED_ITEM('',(#130991),#2918);
#2952=PLANE('',#45569);
#2953=PLANE('',#45571);
#2954=PLANE('',#45574);
#2955=PLANE('',#45575);
#2956=PLANE('',#45579);
#2957=PLANE('',#45580);
#2958=PLANE('',#45581);
#2959=PLANE('',#47448);
#2960=PLANE('',#47450);
#2961=PLANE('',#47461);
#2962=PLANE('',#47462);
#2963=PLANE('',#47465);
#2964=PLANE('',#47472);
#2965=PLANE('',#47525);
#2966=PLANE('',#47526);
#2967=PLANE('',#47527);
#2968=PLANE('',#47531);
#2969=PLANE('',#47532);
#2970=PLANE('',#47535);
#2971=PLANE('',#47536);
#2972=PLANE('',#47538);
#2973=PLANE('',#47539);
#2974=PLANE('',#47540);
#2975=PLANE('',#47541);
#2976=PLANE('',#47542);
#2977=PLANE('',#47543);
#2978=PLANE('',#47544);
#2979=PLANE('',#47545);
#2980=PLANE('',#47546);
#2981=PLANE('',#47547);
#2982=PLANE('',#47548);
#2983=PLANE('',#47549);
#2984=PLANE('',#47550);
#2985=PLANE('',#47551);
#2986=PLANE('',#47552);
#2987=PLANE('',#47553);
#2988=PLANE('',#47554);
#2989=PLANE('',#47555);
#2990=PLANE('',#47556);
#2991=PLANE('',#47557);
#2992=PLANE('',#47558);
#2993=PLANE('',#47559);
#2994=PLANE('',#47560);
#2995=PLANE('',#47561);
#2996=PLANE('',#47562);
#2997=PLANE('',#47563);
#2998=PLANE('',#47564);
#2999=PLANE('',#47565);
#3000=PLANE('',#47566);
#3001=PLANE('',#47567);
#3002=PLANE('',#47568);
#3003=PLANE('',#47569);
#3004=PLANE('',#47570);
#3005=PLANE('',#47571);
#3006=PLANE('',#47572);
#3007=PLANE('',#47573);
#3008=PLANE('',#47574);
#3009=PLANE('',#47575);
#3010=PLANE('',#47576);
#3011=PLANE('',#47577);
#3012=PLANE('',#47578);
#3013=PLANE('',#47579);
#3014=PLANE('',#47580);
#3015=PLANE('',#47581);
#3016=PLANE('',#47582);
#3017=PLANE('',#47583);
#3018=PLANE('',#47584);
#3019=PLANE('',#47585);
#3020=PLANE('',#47586);
#3021=PLANE('',#47587);
#3022=PLANE('',#47588);
#3023=PLANE('',#47589);
#3024=PLANE('',#47590);
#3025=PLANE('',#47591);
#3026=PLANE('',#47592);
#3027=PLANE('',#47593);
#3028=PLANE('',#47594);
#3029=PLANE('',#47595);
#3030=PLANE('',#47596);
#3031=PLANE('',#47597);
#3032=PLANE('',#47598);
#3033=PLANE('',#47599);
#3034=PLANE('',#47600);
#3035=PLANE('',#47601);
#3036=PLANE('',#47602);
#3037=PLANE('',#47603);
#3038=PLANE('',#47604);
#3039=PLANE('',#47605);
#3040=PLANE('',#47606);
#3041=PLANE('',#47607);
#3042=PLANE('',#47608);
#3043=PLANE('',#47609);
#3044=PLANE('',#47610);
#3045=PLANE('',#47611);
#3046=PLANE('',#47612);
#3047=PLANE('',#47613);
#3048=PLANE('',#47614);
#3049=PLANE('',#47615);
#3050=PLANE('',#47616);
#3051=PLANE('',#47617);
#3052=PLANE('',#47618);
#3053=PLANE('',#47619);
#3054=PLANE('',#47620);
#3055=PLANE('',#47621);
#3056=PLANE('',#47622);
#3057=PLANE('',#47623);
#3058=PLANE('',#47624);
#3059=PLANE('',#47625);
#3060=PLANE('',#47626);
#3061=PLANE('',#47627);
#3062=PLANE('',#47628);
#3063=PLANE('',#47629);
#3064=PLANE('',#47630);
#3065=PLANE('',#47631);
#3066=PLANE('',#47632);
#3067=PLANE('',#47633);
#3068=PLANE('',#47634);
#3069=PLANE('',#47635);
#3070=PLANE('',#47636);
#3071=PLANE('',#47637);
#3072=PLANE('',#47638);
#3073=PLANE('',#47639);
#3074=PLANE('',#47640);
#3075=PLANE('',#47641);
#3076=PLANE('',#47642);
#3077=PLANE('',#47643);
#3078=PLANE('',#47644);
#3079=PLANE('',#47645);
#3080=PLANE('',#47646);
#3081=PLANE('',#47647);
#3082=PLANE('',#47648);
#3083=PLANE('',#47649);
#3084=PLANE('',#47650);
#3085=PLANE('',#47651);
#3086=PLANE('',#47652);
#3087=PLANE('',#47653);
#3088=PLANE('',#47654);
#3089=PLANE('',#47655);
#3090=PLANE('',#47656);
#3091=PLANE('',#47657);
#3092=PLANE('',#47658);
#3093=PLANE('',#47659);
#3094=PLANE('',#47660);
#3095=PLANE('',#47661);
#3096=PLANE('',#47662);
#3097=PLANE('',#47663);
#3098=PLANE('',#47664);
#3099=PLANE('',#47665);
#3100=PLANE('',#47666);
#3101=PLANE('',#47667);
#3102=PLANE('',#47668);
#3103=PLANE('',#47669);
#3104=PLANE('',#47670);
#3105=PLANE('',#47671);
#3106=PLANE('',#47672);
#3107=PLANE('',#47673);
#3108=PLANE('',#47674);
#3109=PLANE('',#47675);
#3110=PLANE('',#47676);
#3111=PLANE('',#47677);
#3112=PLANE('',#47678);
#3113=PLANE('',#47679);
#3114=PLANE('',#47680);
#3115=PLANE('',#47681);
#3116=PLANE('',#47682);
#3117=PLANE('',#47683);
#3118=PLANE('',#47684);
#3119=PLANE('',#47685);
#3120=PLANE('',#47686);
#3121=PLANE('',#47687);
#3122=PLANE('',#47688);
#3123=PLANE('',#47689);
#3124=PLANE('',#47690);
#3125=PLANE('',#47691);
#3126=PLANE('',#47692);
#3127=PLANE('',#47693);
#3128=PLANE('',#47694);
#3129=PLANE('',#47695);
#3130=PLANE('',#47696);
#3131=PLANE('',#47697);
#3132=PLANE('',#47698);
#3133=PLANE('',#47699);
#3134=PLANE('',#47700);
#3135=PLANE('',#47701);
#3136=PLANE('',#47702);
#3137=PLANE('',#47703);
#3138=PLANE('',#47704);
#3139=PLANE('',#47705);
#3140=PLANE('',#47706);
#3141=PLANE('',#47707);
#3142=PLANE('',#47708);
#3143=PLANE('',#47709);
#3144=PLANE('',#47710);
#3145=PLANE('',#47711);
#3146=PLANE('',#47712);
#3147=PLANE('',#47713);
#3148=PLANE('',#47714);
#3149=PLANE('',#47715);
#3150=PLANE('',#47716);
#3151=PLANE('',#47717);
#3152=PLANE('',#47718);
#3153=PLANE('',#47719);
#3154=PLANE('',#47720);
#3155=PLANE('',#47721);
#3156=PLANE('',#47722);
#3157=PLANE('',#47723);
#3158=PLANE('',#47724);
#3159=PLANE('',#47725);
#3160=PLANE('',#47726);
#3161=PLANE('',#47727);
#3162=PLANE('',#47728);
#3163=PLANE('',#47729);
#3164=PLANE('',#47730);
#3165=PLANE('',#47731);
#3166=PLANE('',#47732);
#3167=PLANE('',#47733);
#3168=PLANE('',#47734);
#3169=PLANE('',#47735);
#3170=PLANE('',#47736);
#3171=PLANE('',#47737);
#3172=PLANE('',#47738);
#3173=PLANE('',#47739);
#3174=PLANE('',#47740);
#3175=PLANE('',#47741);
#3176=PLANE('',#47742);
#3177=PLANE('',#47743);
#3178=PLANE('',#47744);
#3179=PLANE('',#47745);
#3180=PLANE('',#47746);
#3181=PLANE('',#47747);
#3182=PLANE('',#47748);
#3183=PLANE('',#47749);
#3184=PLANE('',#47750);
#3185=PLANE('',#47751);
#3186=PLANE('',#47752);
#3187=PLANE('',#47753);
#3188=PLANE('',#47754);
#3189=PLANE('',#47755);
#3190=PLANE('',#47756);
#3191=PLANE('',#47757);
#3192=PLANE('',#47758);
#3193=PLANE('',#47759);
#3194=PLANE('',#47760);
#3195=PLANE('',#47761);
#3196=PLANE('',#47762);
#3197=PLANE('',#47763);
#3198=PLANE('',#47764);
#3199=PLANE('',#47765);
#3200=PLANE('',#47766);
#3201=PLANE('',#47767);
#3202=PLANE('',#47768);
#3203=PLANE('',#47769);
#3204=PLANE('',#47770);
#3205=PLANE('',#47771);
#3206=PLANE('',#47772);
#3207=PLANE('',#47773);
#3208=PLANE('',#47774);
#3209=PLANE('',#47775);
#3210=PLANE('',#47776);
#3211=PLANE('',#47777);
#3212=PLANE('',#47778);
#3213=PLANE('',#47779);
#3214=PLANE('',#47780);
#3215=PLANE('',#47781);
#3216=PLANE('',#47782);
#3217=PLANE('',#47783);
#3218=PLANE('',#47784);
#3219=PLANE('',#47785);
#3220=PLANE('',#47786);
#3221=PLANE('',#47787);
#3222=PLANE('',#47788);
#3223=PLANE('',#47789);
#3224=PLANE('',#47790);
#3225=PLANE('',#47791);
#3226=PLANE('',#47792);
#3227=PLANE('',#47793);
#3228=PLANE('',#47794);
#3229=PLANE('',#47795);
#3230=PLANE('',#47796);
#3231=PLANE('',#47797);
#3232=PLANE('',#47798);
#3233=PLANE('',#47799);
#3234=PLANE('',#47800);
#3235=PLANE('',#47801);
#3236=PLANE('',#47802);
#3237=PLANE('',#47803);
#3238=PLANE('',#47804);
#3239=PLANE('',#47805);
#3240=PLANE('',#47806);
#3241=PLANE('',#47807);
#3242=PLANE('',#47808);
#3243=PLANE('',#47809);
#3244=PLANE('',#47810);
#3245=PLANE('',#47811);
#3246=PLANE('',#47812);
#3247=PLANE('',#47813);
#3248=PLANE('',#47814);
#3249=PLANE('',#47815);
#3250=PLANE('',#47816);
#3251=PLANE('',#47817);
#3252=PLANE('',#47818);
#3253=PLANE('',#47819);
#3254=PLANE('',#47820);
#3255=PLANE('',#47821);
#3256=PLANE('',#47822);
#3257=PLANE('',#47823);
#3258=PLANE('',#47824);
#3259=PLANE('',#47825);
#3260=PLANE('',#47826);
#3261=PLANE('',#47827);
#3262=PLANE('',#47828);
#3263=PLANE('',#47829);
#3264=PLANE('',#47830);
#3265=PLANE('',#47831);
#3266=PLANE('',#47832);
#3267=PLANE('',#47833);
#3268=PLANE('',#47834);
#3269=PLANE('',#47835);
#3270=PLANE('',#47836);
#3271=PLANE('',#47837);
#3272=PLANE('',#47838);
#3273=PLANE('',#47839);
#3274=PLANE('',#47840);
#3275=PLANE('',#47841);
#3276=PLANE('',#47842);
#3277=PLANE('',#47843);
#3278=PLANE('',#47844);
#3279=PLANE('',#47845);
#3280=PLANE('',#47846);
#3281=PLANE('',#47847);
#3282=PLANE('',#47848);
#3283=PLANE('',#47849);
#3284=PLANE('',#47850);
#3285=PLANE('',#47851);
#3286=PLANE('',#47852);
#3287=PLANE('',#47853);
#3288=PLANE('',#47854);
#3289=PLANE('',#47855);
#3290=PLANE('',#47856);
#3291=PLANE('',#47857);
#3292=PLANE('',#47858);
#3293=PLANE('',#47859);
#3294=PLANE('',#47860);
#3295=PLANE('',#47861);
#3296=PLANE('',#47862);
#3297=PLANE('',#47863);
#3298=PLANE('',#47864);
#3299=PLANE('',#47865);
#3300=PLANE('',#47866);
#3301=PLANE('',#47867);
#3302=PLANE('',#47868);
#3303=PLANE('',#47869);
#3304=PLANE('',#47870);
#3305=PLANE('',#47871);
#3306=PLANE('',#47872);
#3307=PLANE('',#47873);
#3308=PLANE('',#47874);
#3309=PLANE('',#47875);
#3310=PLANE('',#47876);
#3311=PLANE('',#47877);
#3312=PLANE('',#47878);
#3313=PLANE('',#47879);
#3314=PLANE('',#47880);
#3315=PLANE('',#47881);
#3316=PLANE('',#47882);
#3317=PLANE('',#47883);
#3318=PLANE('',#47884);
#3319=PLANE('',#47885);
#3320=PLANE('',#47886);
#3321=PLANE('',#47887);
#3322=PLANE('',#47888);
#3323=PLANE('',#47889);
#3324=PLANE('',#47890);
#3325=PLANE('',#47891);
#3326=PLANE('',#47892);
#3327=PLANE('',#47893);
#3328=PLANE('',#47894);
#3329=PLANE('',#47895);
#3330=PLANE('',#47896);
#3331=PLANE('',#47897);
#3332=PLANE('',#47898);
#3333=PLANE('',#47899);
#3334=PLANE('',#47900);
#3335=PLANE('',#47901);
#3336=PLANE('',#47902);
#3337=PLANE('',#47903);
#3338=PLANE('',#47904);
#3339=PLANE('',#47905);
#3340=PLANE('',#47906);
#3341=PLANE('',#47907);
#3342=PLANE('',#47908);
#3343=PLANE('',#47909);
#3344=PLANE('',#47910);
#3345=PLANE('',#47911);
#3346=PLANE('',#47912);
#3347=PLANE('',#47913);
#3348=PLANE('',#47914);
#3349=PLANE('',#47915);
#3350=PLANE('',#47916);
#3351=PLANE('',#47917);
#3352=PLANE('',#47918);
#3353=PLANE('',#47919);
#3354=PLANE('',#47920);
#3355=PLANE('',#47921);
#3356=PLANE('',#47922);
#3357=PLANE('',#47923);
#3358=PLANE('',#47924);
#3359=PLANE('',#47925);
#3360=PLANE('',#47926);
#3361=PLANE('',#47927);
#3362=PLANE('',#47928);
#3363=PLANE('',#47929);
#3364=PLANE('',#47930);
#3365=PLANE('',#47931);
#3366=PLANE('',#47932);
#3367=PLANE('',#47933);
#3368=PLANE('',#47934);
#3369=PLANE('',#47935);
#3370=PLANE('',#47936);
#3371=PLANE('',#47937);
#3372=PLANE('',#47938);
#3373=PLANE('',#47939);
#3374=PLANE('',#47940);
#3375=PLANE('',#47941);
#3376=PLANE('',#47942);
#3377=PLANE('',#47943);
#3378=PLANE('',#47944);
#3379=PLANE('',#47945);
#3380=PLANE('',#47946);
#3381=PLANE('',#47947);
#3382=PLANE('',#47948);
#3383=PLANE('',#47949);
#3384=PLANE('',#47950);
#3385=PLANE('',#47951);
#3386=PLANE('',#47952);
#3387=PLANE('',#47953);
#3388=PLANE('',#47954);
#3389=PLANE('',#47955);
#3390=PLANE('',#47956);
#3391=PLANE('',#47957);
#3392=PLANE('',#47958);
#3393=PLANE('',#47959);
#3394=PLANE('',#47960);
#3395=PLANE('',#47961);
#3396=PLANE('',#47962);
#3397=PLANE('',#47963);
#3398=PLANE('',#47964);
#3399=PLANE('',#47965);
#3400=PLANE('',#47966);
#3401=PLANE('',#47967);
#3402=PLANE('',#47968);
#3403=PLANE('',#47969);
#3404=PLANE('',#47970);
#3405=PLANE('',#47971);
#3406=PLANE('',#47972);
#3407=PLANE('',#47973);
#3408=PLANE('',#47974);
#3409=PLANE('',#47975);
#3410=PLANE('',#47976);
#3411=PLANE('',#47977);
#3412=PLANE('',#47978);
#3413=PLANE('',#47979);
#3414=PLANE('',#47980);
#3415=PLANE('',#47981);
#3416=PLANE('',#47982);
#3417=PLANE('',#47983);
#3418=PLANE('',#47984);
#3419=PLANE('',#47985);
#3420=PLANE('',#47986);
#3421=PLANE('',#47987);
#3422=PLANE('',#47988);
#3423=PLANE('',#47989);
#3424=PLANE('',#47990);
#3425=PLANE('',#47991);
#3426=PLANE('',#47992);
#3427=PLANE('',#47993);
#3428=PLANE('',#47994);
#3429=PLANE('',#47995);
#3430=PLANE('',#47996);
#3431=PLANE('',#47997);
#3432=PLANE('',#47998);
#3433=PLANE('',#47999);
#3434=PLANE('',#48000);
#3435=PLANE('',#48001);
#3436=PLANE('',#48002);
#3437=PLANE('',#48003);
#3438=PLANE('',#48004);
#3439=PLANE('',#48005);
#3440=PLANE('',#48006);
#3441=PLANE('',#48007);
#3442=PLANE('',#48008);
#3443=PLANE('',#48009);
#3444=PLANE('',#48010);
#3445=PLANE('',#48011);
#3446=PLANE('',#48012);
#3447=PLANE('',#48013);
#3448=PLANE('',#48014);
#3449=PLANE('',#48015);
#3450=PLANE('',#48016);
#3451=PLANE('',#48017);
#3452=PLANE('',#48018);
#3453=PLANE('',#48019);
#3454=PLANE('',#48020);
#3455=PLANE('',#48021);
#3456=PLANE('',#48022);
#3457=PLANE('',#48023);
#3458=PLANE('',#48024);
#3459=PLANE('',#48025);
#3460=PLANE('',#48026);
#3461=PLANE('',#48027);
#3462=PLANE('',#48028);
#3463=PLANE('',#48029);
#3464=PLANE('',#48030);
#3465=PLANE('',#48031);
#3466=PLANE('',#48032);
#3467=PLANE('',#48033);
#3468=PLANE('',#48034);
#3469=PLANE('',#48035);
#3470=PLANE('',#48036);
#3471=PLANE('',#48037);
#3472=PLANE('',#48038);
#3473=PLANE('',#48039);
#3474=PLANE('',#48040);
#3475=PLANE('',#48041);
#3476=PLANE('',#48042);
#3477=PLANE('',#48043);
#3478=PLANE('',#48044);
#3479=PLANE('',#48045);
#3480=PLANE('',#48046);
#3481=PLANE('',#48047);
#3482=PLANE('',#48048);
#3483=PLANE('',#48049);
#3484=PLANE('',#48050);
#3485=PLANE('',#48051);
#3486=PLANE('',#48052);
#3487=PLANE('',#48053);
#3488=PLANE('',#48054);
#3489=PLANE('',#48055);
#3490=PLANE('',#48056);
#3491=PLANE('',#48057);
#3492=PLANE('',#48058);
#3493=PLANE('',#48059);
#3494=PLANE('',#48060);
#3495=PLANE('',#48061);
#3496=PLANE('',#48062);
#3497=PLANE('',#48063);
#3498=PLANE('',#48064);
#3499=PLANE('',#48065);
#3500=PLANE('',#48066);
#3501=PLANE('',#48067);
#3502=PLANE('',#48068);
#3503=PLANE('',#48069);
#3504=PLANE('',#48070);
#3505=PLANE('',#48071);
#3506=PLANE('',#48072);
#3507=PLANE('',#48073);
#3508=PLANE('',#48074);
#3509=PLANE('',#48075);
#3510=PLANE('',#48076);
#3511=PLANE('',#48077);
#3512=PLANE('',#48078);
#3513=PLANE('',#48079);
#3514=PLANE('',#48080);
#3515=PLANE('',#48081);
#3516=PLANE('',#48082);
#3517=PLANE('',#48083);
#3518=PLANE('',#48084);
#3519=PLANE('',#48085);
#3520=PLANE('',#48086);
#3521=PLANE('',#48087);
#3522=PLANE('',#48088);
#3523=PLANE('',#48089);
#3524=PLANE('',#48090);
#3525=PLANE('',#48091);
#3526=PLANE('',#48092);
#3527=PLANE('',#48093);
#3528=PLANE('',#48094);
#3529=PLANE('',#48095);
#3530=PLANE('',#48096);
#3531=PLANE('',#48097);
#3532=PLANE('',#48098);
#3533=PLANE('',#48099);
#3534=PLANE('',#48100);
#3535=PLANE('',#48101);
#3536=PLANE('',#48102);
#3537=PLANE('',#48103);
#3538=PLANE('',#48104);
#3539=PLANE('',#48105);
#3540=PLANE('',#48106);
#3541=PLANE('',#48107);
#3542=PLANE('',#48108);
#3543=PLANE('',#48109);
#3544=PLANE('',#48110);
#3545=PLANE('',#48111);
#3546=PLANE('',#48112);
#3547=PLANE('',#48113);
#3548=PLANE('',#48114);
#3549=PLANE('',#48115);
#3550=PLANE('',#48116);
#3551=PLANE('',#48117);
#3552=PLANE('',#48118);
#3553=PLANE('',#48119);
#3554=PLANE('',#48120);
#3555=PLANE('',#48121);
#3556=PLANE('',#48122);
#3557=PLANE('',#48123);
#3558=PLANE('',#48124);
#3559=PLANE('',#48125);
#3560=PLANE('',#48126);
#3561=PLANE('',#48127);
#3562=PLANE('',#48128);
#3563=PLANE('',#48129);
#3564=PLANE('',#48130);
#3565=PLANE('',#48131);
#3566=PLANE('',#48132);
#3567=PLANE('',#48133);
#3568=PLANE('',#48134);
#3569=PLANE('',#48135);
#3570=PLANE('',#48136);
#4315=LINE('',#65513,#6089);
#4316=LINE('',#65517,#6090);
#4317=LINE('',#65518,#6091);
#4318=LINE('',#65521,#6092);
#4319=LINE('',#65524,#6093);
#4320=LINE('',#65526,#6094);
#4321=LINE('',#65527,#6095);
#4322=LINE('',#65533,#6096);
#4323=LINE('',#65537,#6097);
#4324=LINE('',#65541,#6098);
#4325=LINE('',#65542,#6099);
#4326=LINE('',#65545,#6100);
#4327=LINE('',#65546,#6101);
#4328=LINE('',#65554,#6102);
#4329=LINE('',#65560,#6103);
#4330=LINE('',#65566,#6104);
#4331=LINE('',#65572,#6105);
#4332=LINE('',#65578,#6106);
#4333=LINE('',#65584,#6107);
#4334=LINE('',#65590,#6108);
#4335=LINE('',#65596,#6109);
#4336=LINE('',#65602,#6110);
#4337=LINE('',#65608,#6111);
#4338=LINE('',#65614,#6112);
#4339=LINE('',#65620,#6113);
#4340=LINE('',#65647,#6114);
#4341=LINE('',#65708,#6115);
#4342=LINE('',#65767,#6116);
#4343=LINE('',#65829,#6117);
#4344=LINE('',#65891,#6118);
#4345=LINE('',#65950,#6119);
#4346=LINE('',#66009,#6120);
#4347=LINE('',#66071,#6121);
#4348=LINE('',#66133,#6122);
#4349=LINE('',#66192,#6123);
#4350=LINE('',#66254,#6124);
#4351=LINE('',#66313,#6125);
#4352=LINE('',#66375,#6126);
#4353=LINE('',#66434,#6127);
#4354=LINE('',#66496,#6128);
#4355=LINE('',#66555,#6129);
#4356=LINE('',#66617,#6130);
#4357=LINE('',#66676,#6131);
#4358=LINE('',#66738,#6132);
#4359=LINE('',#66797,#6133);
#4360=LINE('',#66856,#6134);
#4361=LINE('',#66918,#6135);
#4362=LINE('',#66977,#6136);
#4363=LINE('',#67039,#6137);
#4364=LINE('',#67098,#6138);
#4365=LINE('',#67160,#6139);
#4366=LINE('',#67219,#6140);
#4367=LINE('',#67281,#6141);
#4368=LINE('',#67340,#6142);
#4369=LINE('',#67402,#6143);
#4370=LINE('',#67461,#6144);
#4371=LINE('',#67523,#6145);
#4372=LINE('',#67583,#6146);
#4373=LINE('',#67644,#6147);
#4374=LINE('',#67701,#6148);
#4375=LINE('',#67765,#6149);
#4376=LINE('',#67827,#6150);
#4377=LINE('',#67886,#6151);
#4378=LINE('',#67943,#6152);
#4379=LINE('',#68007,#6153);
#4380=LINE('',#68064,#6154);
#4381=LINE('',#68128,#6155);
#4382=LINE('',#68185,#6156);
#4383=LINE('',#68249,#6157);
#4384=LINE('',#68306,#6158);
#4385=LINE('',#68370,#6159);
#4386=LINE('',#68430,#6160);
#4387=LINE('',#68491,#6161);
#4388=LINE('',#68548,#6162);
#4389=LINE('',#68612,#6163);
#4390=LINE('',#68669,#6164);
#4391=LINE('',#68733,#6165);
#4392=LINE('',#68790,#6166);
#4393=LINE('',#68854,#6167);
#4394=LINE('',#68911,#6168);
#4395=LINE('',#68975,#6169);
#4396=LINE('',#69032,#6170);
#4397=LINE('',#69096,#6171);
#4398=LINE('',#69153,#6172);
#4399=LINE('',#69217,#6173);
#4400=LINE('',#69274,#6174);
#4401=LINE('',#69338,#6175);
#4402=LINE('',#69395,#6176);
#4403=LINE('',#69459,#6177);
#4404=LINE('',#69516,#6178);
#4405=LINE('',#69582,#6179);
#4406=LINE('',#69642,#6180);
#4407=LINE('',#69703,#6181);
#4408=LINE('',#69760,#6182);
#4409=LINE('',#69824,#6183);
#4410=LINE('',#69881,#6184);
#4411=LINE('',#69945,#6185);
#4412=LINE('',#70002,#6186);
#4413=LINE('',#70066,#6187);
#4414=LINE('',#70123,#6188);
#4415=LINE('',#70199,#6189);
#4416=LINE('',#70256,#6190);
#4417=LINE('',#70320,#6191);
#4418=LINE('',#70359,#6192);
#4419=LINE('',#70408,#6193);
#4420=LINE('',#70414,#6194);
#4421=LINE('',#70465,#6195);
#4422=LINE('',#70489,#6196);
#4423=LINE('',#70569,#6197);
#4424=LINE('',#70629,#6198);
#4425=LINE('',#70708,#6199);
#4426=LINE('',#70747,#6200);
#4427=LINE('',#70800,#6201);
#4428=LINE('',#70806,#6202);
#4429=LINE('',#70857,#6203);
#4430=LINE('',#70884,#6204);
#4431=LINE('',#70955,#6205);
#4432=LINE('',#71015,#6206);
#4433=LINE('',#71090,#6207);
#4434=LINE('',#71129,#6208);
#4435=LINE('',#71182,#6209);
#4436=LINE('',#71206,#6210);
#4437=LINE('',#71280,#6211);
#4438=LINE('',#71340,#6212);
#4439=LINE('',#71409,#6213);
#4440=LINE('',#71448,#6214);
#4441=LINE('',#71503,#6215);
#4442=LINE('',#71530,#6216);
#4443=LINE('',#71603,#6217);
#4444=LINE('',#71660,#6218);
#4445=LINE('',#71734,#6219);
#4446=LINE('',#71794,#6220);
#4447=LINE('',#71871,#6221);
#4448=LINE('',#71928,#6222);
#4449=LINE('',#72012,#6223);
#4450=LINE('',#72072,#6224);
#4451=LINE('',#72133,#6225);
#4452=LINE('',#72190,#6226);
#4453=LINE('',#72268,#6227);
#4454=LINE('',#72328,#6228);
#4455=LINE('',#72389,#6229);
#4456=LINE('',#72449,#6230);
#4457=LINE('',#72510,#6231);
#4458=LINE('',#72569,#6232);
#4459=LINE('',#72631,#6233);
#4460=LINE('',#72693,#6234);
#4461=LINE('',#72752,#6235);
#4462=LINE('',#72814,#6236);
#4463=LINE('',#72873,#6237);
#4464=LINE('',#72933,#6238);
#4465=LINE('',#72994,#6239);
#4466=LINE('',#73056,#6240);
#4467=LINE('',#73117,#6241);
#4468=LINE('',#73179,#6242);
#4469=LINE('',#73238,#6243);
#4470=LINE('',#73277,#6244);
#4471=LINE('',#73283,#6245);
#4472=LINE('',#73289,#6246);
#4473=LINE('',#73295,#6247);
#4474=LINE('',#73301,#6248);
#4475=LINE('',#73307,#6249);
#4476=LINE('',#73313,#6250);
#4477=LINE('',#73319,#6251);
#4478=LINE('',#73325,#6252);
#4479=LINE('',#73331,#6253);
#4480=LINE('',#73337,#6254);
#4481=LINE('',#73343,#6255);
#4482=LINE('',#73349,#6256);
#4483=LINE('',#73355,#6257);
#4484=LINE('',#73361,#6258);
#4485=LINE('',#73367,#6259);
#4486=LINE('',#73373,#6260);
#4487=LINE('',#73414,#6261);
#4488=LINE('',#73420,#6262);
#4489=LINE('',#73426,#6263);
#4490=LINE('',#73432,#6264);
#4491=LINE('',#73438,#6265);
#4492=LINE('',#73444,#6266);
#4493=LINE('',#73450,#6267);
#4494=LINE('',#73456,#6268);
#4495=LINE('',#73462,#6269);
#4496=LINE('',#73468,#6270);
#4497=LINE('',#73474,#6271);
#4498=LINE('',#73480,#6272);
#4499=LINE('',#73486,#6273);
#4500=LINE('',#73492,#6274);
#4501=LINE('',#73498,#6275);
#4502=LINE('',#73504,#6276);
#4503=LINE('',#73510,#6277);
#4504=LINE('',#73516,#6278);
#4505=LINE('',#73557,#6279);
#4506=LINE('',#73563,#6280);
#4507=LINE('',#73569,#6281);
#4508=LINE('',#73575,#6282);
#4509=LINE('',#73581,#6283);
#4510=LINE('',#73587,#6284);
#4511=LINE('',#73593,#6285);
#4512=LINE('',#73599,#6286);
#4513=LINE('',#73605,#6287);
#4514=LINE('',#73611,#6288);
#4515=LINE('',#73617,#6289);
#4516=LINE('',#73623,#6290);
#4517=LINE('',#73629,#6291);
#4518=LINE('',#73635,#6292);
#4519=LINE('',#73641,#6293);
#4520=LINE('',#73647,#6294);
#4521=LINE('',#73688,#6295);
#4522=LINE('',#73694,#6296);
#4523=LINE('',#73700,#6297);
#4524=LINE('',#73706,#6298);
#4525=LINE('',#73712,#6299);
#4526=LINE('',#73718,#6300);
#4527=LINE('',#73724,#6301);
#4528=LINE('',#73730,#6302);
#4529=LINE('',#73736,#6303);
#4530=LINE('',#73742,#6304);
#4531=LINE('',#73748,#6305);
#4532=LINE('',#73754,#6306);
#4533=LINE('',#73760,#6307);
#4534=LINE('',#73766,#6308);
#4535=LINE('',#73772,#6309);
#4536=LINE('',#73778,#6310);
#4537=LINE('',#73784,#6311);
#4538=LINE('',#73790,#6312);
#4539=LINE('',#73831,#6313);
#4540=LINE('',#73837,#6314);
#4541=LINE('',#73843,#6315);
#4542=LINE('',#73849,#6316);
#4543=LINE('',#73855,#6317);
#4544=LINE('',#73861,#6318);
#4545=LINE('',#73867,#6319);
#4546=LINE('',#73873,#6320);
#4547=LINE('',#73879,#6321);
#4548=LINE('',#73885,#6322);
#4549=LINE('',#73891,#6323);
#4550=LINE('',#73897,#6324);
#4551=LINE('',#73903,#6325);
#4552=LINE('',#73909,#6326);
#4553=LINE('',#73915,#6327);
#4554=LINE('',#73921,#6328);
#4555=LINE('',#73927,#6329);
#4556=LINE('',#73933,#6330);
#4557=LINE('',#73974,#6331);
#4558=LINE('',#73980,#6332);
#4559=LINE('',#73986,#6333);
#4560=LINE('',#73992,#6334);
#4561=LINE('',#73998,#6335);
#4562=LINE('',#74004,#6336);
#4563=LINE('',#74010,#6337);
#4564=LINE('',#74016,#6338);
#4565=LINE('',#74022,#6339);
#4566=LINE('',#74028,#6340);
#4567=LINE('',#74034,#6341);
#4568=LINE('',#74040,#6342);
#4569=LINE('',#74046,#6343);
#4570=LINE('',#74052,#6344);
#4571=LINE('',#74058,#6345);
#4572=LINE('',#74064,#6346);
#4573=LINE('',#74070,#6347);
#4574=LINE('',#74076,#6348);
#4575=LINE('',#74117,#6349);
#4576=LINE('',#74123,#6350);
#4577=LINE('',#74129,#6351);
#4578=LINE('',#74135,#6352);
#4579=LINE('',#74141,#6353);
#4580=LINE('',#74147,#6354);
#4581=LINE('',#74153,#6355);
#4582=LINE('',#74159,#6356);
#4583=LINE('',#74165,#6357);
#4584=LINE('',#74171,#6358);
#4585=LINE('',#74177,#6359);
#4586=LINE('',#74183,#6360);
#4587=LINE('',#74189,#6361);
#4588=LINE('',#74195,#6362);
#4589=LINE('',#74201,#6363);
#4590=LINE('',#74207,#6364);
#4591=LINE('',#74213,#6365);
#4592=LINE('',#74219,#6366);
#4593=LINE('',#74260,#6367);
#4594=LINE('',#74266,#6368);
#4595=LINE('',#74272,#6369);
#4596=LINE('',#74278,#6370);
#4597=LINE('',#74284,#6371);
#4598=LINE('',#74290,#6372);
#4599=LINE('',#74296,#6373);
#4600=LINE('',#74302,#6374);
#4601=LINE('',#74308,#6375);
#4602=LINE('',#74314,#6376);
#4603=LINE('',#74320,#6377);
#4604=LINE('',#74326,#6378);
#4605=LINE('',#74332,#6379);
#4606=LINE('',#74338,#6380);
#4607=LINE('',#74344,#6381);
#4608=LINE('',#74350,#6382);
#4609=LINE('',#74391,#6383);
#4610=LINE('',#74397,#6384);
#4611=LINE('',#74403,#6385);
#4612=LINE('',#74409,#6386);
#4613=LINE('',#74415,#6387);
#4614=LINE('',#74421,#6388);
#4615=LINE('',#74427,#6389);
#4616=LINE('',#74433,#6390);
#4617=LINE('',#74439,#6391);
#4618=LINE('',#74445,#6392);
#4619=LINE('',#74451,#6393);
#4620=LINE('',#74457,#6394);
#4621=LINE('',#74463,#6395);
#4622=LINE('',#74469,#6396);
#4623=LINE('',#74475,#6397);
#4624=LINE('',#74481,#6398);
#4625=LINE('',#74487,#6399);
#4626=LINE('',#74493,#6400);
#4627=LINE('',#74534,#6401);
#4628=LINE('',#74540,#6402);
#4629=LINE('',#74546,#6403);
#4630=LINE('',#74552,#6404);
#4631=LINE('',#74558,#6405);
#4632=LINE('',#74564,#6406);
#4633=LINE('',#74570,#6407);
#4634=LINE('',#74576,#6408);
#4635=LINE('',#74582,#6409);
#4636=LINE('',#74588,#6410);
#4637=LINE('',#74594,#6411);
#4638=LINE('',#74600,#6412);
#4639=LINE('',#74606,#6413);
#4640=LINE('',#74612,#6414);
#4641=LINE('',#74618,#6415);
#4642=LINE('',#74624,#6416);
#4643=LINE('',#74630,#6417);
#4644=LINE('',#74636,#6418);
#4645=LINE('',#74677,#6419);
#4646=LINE('',#74683,#6420);
#4647=LINE('',#74689,#6421);
#4648=LINE('',#74695,#6422);
#4649=LINE('',#74701,#6423);
#4650=LINE('',#74707,#6424);
#4651=LINE('',#74713,#6425);
#4652=LINE('',#74719,#6426);
#4653=LINE('',#74725,#6427);
#4654=LINE('',#74731,#6428);
#4655=LINE('',#74737,#6429);
#4656=LINE('',#74743,#6430);
#4657=LINE('',#74749,#6431);
#4658=LINE('',#74755,#6432);
#4659=LINE('',#74761,#6433);
#4660=LINE('',#74767,#6434);
#4661=LINE('',#74773,#6435);
#4662=LINE('',#74779,#6436);
#4663=LINE('',#74820,#6437);
#4664=LINE('',#74826,#6438);
#4665=LINE('',#74832,#6439);
#4666=LINE('',#74838,#6440);
#4667=LINE('',#74844,#6441);
#4668=LINE('',#74850,#6442);
#4669=LINE('',#74856,#6443);
#4670=LINE('',#74862,#6444);
#4671=LINE('',#74868,#6445);
#4672=LINE('',#74874,#6446);
#4673=LINE('',#74880,#6447);
#4674=LINE('',#74886,#6448);
#4675=LINE('',#74892,#6449);
#4676=LINE('',#74898,#6450);
#4677=LINE('',#74904,#6451);
#4678=LINE('',#74910,#6452);
#4679=LINE('',#74916,#6453);
#4680=LINE('',#74922,#6454);
#4681=LINE('',#74963,#6455);
#4682=LINE('',#74969,#6456);
#4683=LINE('',#74975,#6457);
#4684=LINE('',#74981,#6458);
#4685=LINE('',#74987,#6459);
#4686=LINE('',#74993,#6460);
#4687=LINE('',#74999,#6461);
#4688=LINE('',#75005,#6462);
#4689=LINE('',#75011,#6463);
#4690=LINE('',#75017,#6464);
#4691=LINE('',#75023,#6465);
#4692=LINE('',#75029,#6466);
#4693=LINE('',#75035,#6467);
#4694=LINE('',#75041,#6468);
#4695=LINE('',#75047,#6469);
#4696=LINE('',#75053,#6470);
#4697=LINE('',#75094,#6471);
#4698=LINE('',#75100,#6472);
#4699=LINE('',#75106,#6473);
#4700=LINE('',#75112,#6474);
#4701=LINE('',#75118,#6475);
#4702=LINE('',#75124,#6476);
#4703=LINE('',#75130,#6477);
#4704=LINE('',#75136,#6478);
#4705=LINE('',#75142,#6479);
#4706=LINE('',#75148,#6480);
#4707=LINE('',#75154,#6481);
#4708=LINE('',#75160,#6482);
#4709=LINE('',#75166,#6483);
#4710=LINE('',#75172,#6484);
#4711=LINE('',#75178,#6485);
#4712=LINE('',#75184,#6486);
#4713=LINE('',#75190,#6487);
#4714=LINE('',#75196,#6488);
#4715=LINE('',#75237,#6489);
#4716=LINE('',#75243,#6490);
#4717=LINE('',#75249,#6491);
#4718=LINE('',#75255,#6492);
#4719=LINE('',#75261,#6493);
#4720=LINE('',#75267,#6494);
#4721=LINE('',#75273,#6495);
#4722=LINE('',#75279,#6496);
#4723=LINE('',#75285,#6497);
#4724=LINE('',#75291,#6498);
#4725=LINE('',#75297,#6499);
#4726=LINE('',#75303,#6500);
#4727=LINE('',#75309,#6501);
#4728=LINE('',#75315,#6502);
#4729=LINE('',#75321,#6503);
#4730=LINE('',#75327,#6504);
#4731=LINE('',#75333,#6505);
#4732=LINE('',#75339,#6506);
#4733=LINE('',#75380,#6507);
#4734=LINE('',#75386,#6508);
#4735=LINE('',#75392,#6509);
#4736=LINE('',#75398,#6510);
#4737=LINE('',#75404,#6511);
#4738=LINE('',#75410,#6512);
#4739=LINE('',#75416,#6513);
#4740=LINE('',#75422,#6514);
#4741=LINE('',#75428,#6515);
#4742=LINE('',#75434,#6516);
#4743=LINE('',#75440,#6517);
#4744=LINE('',#75446,#6518);
#4745=LINE('',#75452,#6519);
#4746=LINE('',#75458,#6520);
#4747=LINE('',#75464,#6521);
#4748=LINE('',#75470,#6522);
#4749=LINE('',#75476,#6523);
#4750=LINE('',#75482,#6524);
#4751=LINE('',#75523,#6525);
#4752=LINE('',#75529,#6526);
#4753=LINE('',#75535,#6527);
#4754=LINE('',#75541,#6528);
#4755=LINE('',#75547,#6529);
#4756=LINE('',#75553,#6530);
#4757=LINE('',#75559,#6531);
#4758=LINE('',#75565,#6532);
#4759=LINE('',#75571,#6533);
#4760=LINE('',#75577,#6534);
#4761=LINE('',#75583,#6535);
#4762=LINE('',#75589,#6536);
#4763=LINE('',#75595,#6537);
#4764=LINE('',#75601,#6538);
#4765=LINE('',#75607,#6539);
#4766=LINE('',#75613,#6540);
#4767=LINE('',#75619,#6541);
#4768=LINE('',#75625,#6542);
#4769=LINE('',#75666,#6543);
#4770=LINE('',#75672,#6544);
#4771=LINE('',#75678,#6545);
#4772=LINE('',#75684,#6546);
#4773=LINE('',#75690,#6547);
#4774=LINE('',#75696,#6548);
#4775=LINE('',#75702,#6549);
#4776=LINE('',#75708,#6550);
#4777=LINE('',#75714,#6551);
#4778=LINE('',#75720,#6552);
#4779=LINE('',#75726,#6553);
#4780=LINE('',#75732,#6554);
#4781=LINE('',#75738,#6555);
#4782=LINE('',#75744,#6556);
#4783=LINE('',#75750,#6557);
#4784=LINE('',#75756,#6558);
#4785=LINE('',#75797,#6559);
#4786=LINE('',#75803,#6560);
#4787=LINE('',#75809,#6561);
#4788=LINE('',#75815,#6562);
#4789=LINE('',#75821,#6563);
#4790=LINE('',#75827,#6564);
#4791=LINE('',#75833,#6565);
#4792=LINE('',#75839,#6566);
#4793=LINE('',#75845,#6567);
#4794=LINE('',#75851,#6568);
#4795=LINE('',#75857,#6569);
#4796=LINE('',#75863,#6570);
#4797=LINE('',#75869,#6571);
#4798=LINE('',#75875,#6572);
#4799=LINE('',#75881,#6573);
#4800=LINE('',#75887,#6574);
#4801=LINE('',#75893,#6575);
#4802=LINE('',#75899,#6576);
#4803=LINE('',#75937,#6577);
#4804=LINE('',#75943,#6578);
#4805=LINE('',#75949,#6579);
#4806=LINE('',#75955,#6580);
#4807=LINE('',#75961,#6581);
#4808=LINE('',#75967,#6582);
#4809=LINE('',#75973,#6583);
#4810=LINE('',#75979,#6584);
#4811=LINE('',#75985,#6585);
#4812=LINE('',#75991,#6586);
#4813=LINE('',#75997,#6587);
#4814=LINE('',#76003,#6588);
#4815=LINE('',#76009,#6589);
#4816=LINE('',#76015,#6590);
#4817=LINE('',#76021,#6591);
#4818=LINE('',#76027,#6592);
#4819=LINE('',#76048,#6593);
#4820=LINE('',#76054,#6594);
#4821=LINE('',#76099,#6595);
#4822=LINE('',#76105,#6596);
#4823=LINE('',#76111,#6597);
#4824=LINE('',#76117,#6598);
#4825=LINE('',#76123,#6599);
#4826=LINE('',#76129,#6600);
#4827=LINE('',#76135,#6601);
#4828=LINE('',#76141,#6602);
#4829=LINE('',#76147,#6603);
#4830=LINE('',#76153,#6604);
#4831=LINE('',#76159,#6605);
#4832=LINE('',#76165,#6606);
#4833=LINE('',#76171,#6607);
#4834=LINE('',#76177,#6608);
#4835=LINE('',#76200,#6609);
#4836=LINE('',#76206,#6610);
#4837=LINE('',#76212,#6611);
#4838=LINE('',#76218,#6612);
#4839=LINE('',#76224,#6613);
#4840=LINE('',#76230,#6614);
#4841=LINE('',#76236,#6615);
#4842=LINE('',#76242,#6616);
#4843=LINE('',#76248,#6617);
#4844=LINE('',#76254,#6618);
#4845=LINE('',#76260,#6619);
#4846=LINE('',#76266,#6620);
#4847=LINE('',#76272,#6621);
#4848=LINE('',#76278,#6622);
#4849=LINE('',#76284,#6623);
#4850=LINE('',#76290,#6624);
#4851=LINE('',#76296,#6625);
#4852=LINE('',#76302,#6626);
#4853=LINE('',#76308,#6627);
#4854=LINE('',#76314,#6628);
#4855=LINE('',#76320,#6629);
#4856=LINE('',#76326,#6630);
#4857=LINE('',#76332,#6631);
#4858=LINE('',#76338,#6632);
#4859=LINE('',#76344,#6633);
#4860=LINE('',#76350,#6634);
#4861=LINE('',#76356,#6635);
#4862=LINE('',#76362,#6636);
#4863=LINE('',#76395,#6637);
#4864=LINE('',#76401,#6638);
#4865=LINE('',#76407,#6639);
#4866=LINE('',#76413,#6640);
#4867=LINE('',#76419,#6641);
#4868=LINE('',#76425,#6642);
#4869=LINE('',#76431,#6643);
#4870=LINE('',#76437,#6644);
#4871=LINE('',#76443,#6645);
#4872=LINE('',#76449,#6646);
#4873=LINE('',#76455,#6647);
#4874=LINE('',#76461,#6648);
#4875=LINE('',#76467,#6649);
#4876=LINE('',#76473,#6650);
#4877=LINE('',#76479,#6651);
#4878=LINE('',#76485,#6652);
#4879=LINE('',#76491,#6653);
#4880=LINE('',#76497,#6654);
#4881=LINE('',#76503,#6655);
#4882=LINE('',#76509,#6656);
#4883=LINE('',#76515,#6657);
#4884=LINE('',#76521,#6658);
#4885=LINE('',#76527,#6659);
#4886=LINE('',#76533,#6660);
#4887=LINE('',#76539,#6661);
#4888=LINE('',#76545,#6662);
#4889=LINE('',#76551,#6663);
#4890=LINE('',#76557,#6664);
#4891=LINE('',#76563,#6665);
#4892=LINE('',#76569,#6666);
#4893=LINE('',#76575,#6667);
#4894=LINE('',#76581,#6668);
#4895=LINE('',#76587,#6669);
#4896=LINE('',#76593,#6670);
#4897=LINE('',#76641,#6671);
#4898=LINE('',#76647,#6672);
#4899=LINE('',#76653,#6673);
#4900=LINE('',#76659,#6674);
#4901=LINE('',#76665,#6675);
#4902=LINE('',#76671,#6676);
#4903=LINE('',#76677,#6677);
#4904=LINE('',#76683,#6678);
#4905=LINE('',#76689,#6679);
#4906=LINE('',#76695,#6680);
#4907=LINE('',#76701,#6681);
#4908=LINE('',#76707,#6682);
#4909=LINE('',#76713,#6683);
#4910=LINE('',#76719,#6684);
#4911=LINE('',#76725,#6685);
#4912=LINE('',#76731,#6686);
#4913=LINE('',#76737,#6687);
#4914=LINE('',#76743,#6688);
#4915=LINE('',#76781,#6689);
#4916=LINE('',#76787,#6690);
#4917=LINE('',#76793,#6691);
#4918=LINE('',#76799,#6692);
#4919=LINE('',#76805,#6693);
#4920=LINE('',#76811,#6694);
#4921=LINE('',#76817,#6695);
#4922=LINE('',#76823,#6696);
#4923=LINE('',#76829,#6697);
#4924=LINE('',#76835,#6698);
#4925=LINE('',#76841,#6699);
#4926=LINE('',#76847,#6700);
#4927=LINE('',#76853,#6701);
#4928=LINE('',#76859,#6702);
#4929=LINE('',#76865,#6703);
#4930=LINE('',#76871,#6704);
#4931=LINE('',#76877,#6705);
#4932=LINE('',#76883,#6706);
#4933=LINE('',#76924,#6707);
#4934=LINE('',#76930,#6708);
#4935=LINE('',#76936,#6709);
#4936=LINE('',#76942,#6710);
#4937=LINE('',#76948,#6711);
#4938=LINE('',#76954,#6712);
#4939=LINE('',#76960,#6713);
#4940=LINE('',#76966,#6714);
#4941=LINE('',#76972,#6715);
#4942=LINE('',#76978,#6716);
#4943=LINE('',#76984,#6717);
#4944=LINE('',#76990,#6718);
#4945=LINE('',#76996,#6719);
#4946=LINE('',#77002,#6720);
#4947=LINE('',#77008,#6721);
#4948=LINE('',#77014,#6722);
#4949=LINE('',#77055,#6723);
#4950=LINE('',#77061,#6724);
#4951=LINE('',#77067,#6725);
#4952=LINE('',#77073,#6726);
#4953=LINE('',#77079,#6727);
#4954=LINE('',#77085,#6728);
#4955=LINE('',#77091,#6729);
#4956=LINE('',#77097,#6730);
#4957=LINE('',#77103,#6731);
#4958=LINE('',#77109,#6732);
#4959=LINE('',#77115,#6733);
#4960=LINE('',#77121,#6734);
#4961=LINE('',#77127,#6735);
#4962=LINE('',#77133,#6736);
#4963=LINE('',#77139,#6737);
#4964=LINE('',#77145,#6738);
#4965=LINE('',#77151,#6739);
#4966=LINE('',#77157,#6740);
#4967=LINE('',#77198,#6741);
#4968=LINE('',#77204,#6742);
#4969=LINE('',#77210,#6743);
#4970=LINE('',#77216,#6744);
#4971=LINE('',#77222,#6745);
#4972=LINE('',#77228,#6746);
#4973=LINE('',#77234,#6747);
#4974=LINE('',#77240,#6748);
#4975=LINE('',#77246,#6749);
#4976=LINE('',#77252,#6750);
#4977=LINE('',#77258,#6751);
#4978=LINE('',#77264,#6752);
#4979=LINE('',#77270,#6753);
#4980=LINE('',#77276,#6754);
#4981=LINE('',#77282,#6755);
#4982=LINE('',#77288,#6756);
#4983=LINE('',#77294,#6757);
#4984=LINE('',#77300,#6758);
#4985=LINE('',#77341,#6759);
#4986=LINE('',#77800,#6760);
#4987=LINE('',#77856,#6761);
#4988=LINE('',#77859,#6762);
#4989=LINE('',#77897,#6763);
#4990=LINE('',#77907,#6764);
#4991=LINE('',#77968,#6765);
#4992=LINE('',#78004,#6766);
#4993=LINE('',#78029,#6767);
#4994=LINE('',#78040,#6768);
#4995=LINE('',#78041,#6769);
#4996=LINE('',#78069,#6770);
#4997=LINE('',#78096,#6771);
#4998=LINE('',#78099,#6772);
#4999=LINE('',#78102,#6773);
#5000=LINE('',#78115,#6774);
#5001=LINE('',#78135,#6775);
#5002=LINE('',#78149,#6776);
#5003=LINE('',#78153,#6777);
#5004=LINE('',#78158,#6778);
#5005=LINE('',#78160,#6779);
#5006=LINE('',#78161,#6780);
#5007=LINE('',#78162,#6781);
#5008=LINE('',#78166,#6782);
#5009=LINE('',#78187,#6783);
#5010=LINE('',#78295,#6784);
#5011=LINE('',#78296,#6785);
#5012=LINE('',#78906,#6786);
#5013=LINE('',#78986,#6787);
#5014=LINE('',#79681,#6788);
#5015=LINE('',#79682,#6789);
#5016=LINE('',#80914,#6790);
#5017=LINE('',#81048,#6791);
#5018=LINE('',#83692,#6792);
#5019=LINE('',#83694,#6793);
#6089=VECTOR('',#51646,1000.);
#6090=VECTOR('',#51649,1000.);
#6091=VECTOR('',#51650,1000.);
#6092=VECTOR('',#51653,1000.);
#6093=VECTOR('',#51656,1000.);
#6094=VECTOR('',#51659,1000.);
#6095=VECTOR('',#51660,1000.);
#6096=VECTOR('',#51667,1000.);
#6097=VECTOR('',#51670,1000.);
#6098=VECTOR('',#51675,1000.);
#6099=VECTOR('',#51676,1000.);
#6100=VECTOR('',#51679,1000.);
#6101=VECTOR('',#51680,1000.);
#6102=VECTOR('',#51691,0.500000000000054);
#6103=VECTOR('',#51698,1.81285717707168);
#6104=VECTOR('',#51705,0.500000000000054);
#6105=VECTOR('',#51712,1.81285717707167);
#6106=VECTOR('',#51719,0.500000000000054);
#6107=VECTOR('',#51726,1.81285717707166);
#6108=VECTOR('',#51733,0.499999999999939);
#6109=VECTOR('',#51740,1.81285717707156);
#6110=VECTOR('',#51747,0.499999999999935);
#6111=VECTOR('',#51754,1.81285717707156);
#6112=VECTOR('',#51761,0.499999999999944);
#6113=VECTOR('',#51768,1.81285717707167);
#6114=VECTOR('',#51773,0.948084450180161);
#6115=VECTOR('',#51778,0.500000000000054);
#6116=VECTOR('',#51781,1.02140828085145);
#6117=VECTOR('',#51786,0.500000000000054);
#6118=VECTOR('',#51789,0.948084450180157);
#6119=VECTOR('',#51794,0.500000000000054);
#6120=VECTOR('',#51797,1.02140828085145);
#6121=VECTOR('',#51802,0.500000000000054);
#6122=VECTOR('',#51805,0.948084450180157);
#6123=VECTOR('',#51810,0.500000000000054);
#6124=VECTOR('',#51813,1.02140828085145);
#6125=VECTOR('',#51818,0.499999999999944);
#6126=VECTOR('',#51821,0.948084450180161);
#6127=VECTOR('',#51826,0.499999999999944);
#6128=VECTOR('',#51829,1.02140828085144);
#6129=VECTOR('',#51834,0.500000000000058);
#6130=VECTOR('',#51837,0.948084450180162);
#6131=VECTOR('',#51842,0.500000000000058);
#6132=VECTOR('',#51845,1.02140828085145);
#6133=VECTOR('',#51850,0.500000000000058);
#6134=VECTOR('',#51853,0.948084450180161);
#6135=VECTOR('',#51858,0.500000000000172);
#6136=VECTOR('',#51861,1.02140828085157);
#6137=VECTOR('',#51866,0.499999999999935);
#6138=VECTOR('',#51869,0.948084450180161);
#6139=VECTOR('',#51874,0.500000000000058);
#6140=VECTOR('',#51877,1.02140828085134);
#6141=VECTOR('',#51882,0.499999999999935);
#6142=VECTOR('',#51885,0.948084450180275);
#6143=VECTOR('',#51890,0.500000000000058);
#6144=VECTOR('',#51893,1.02140828085134);
#6145=VECTOR('',#51898,0.500000000000058);
#6146=VECTOR('',#51901,0.948084450180152);
#6147=VECTOR('',#51906,0.499999999999944);
#6148=VECTOR('',#51909,1.02140828085157);
#6149=VECTOR('',#51914,0.500000000000067);
#6150=VECTOR('',#51917,0.948084450180047);
#6151=VECTOR('',#51922,0.499999999999935);
#6152=VECTOR('',#51925,1.02140828085145);
#6153=VECTOR('',#51930,0.499999999999935);
#6154=VECTOR('',#51933,0.94808445018017);
#6155=VECTOR('',#51938,0.500000000000058);
#6156=VECTOR('',#51941,1.02140828085121);
#6157=VECTOR('',#51946,0.499999999999944);
#6158=VECTOR('',#51949,0.948084450180161);
#6159=VECTOR('',#51954,0.499999999999944);
#6160=VECTOR('',#51957,1.02140828085145);
#6161=VECTOR('',#51962,0.499999999999939);
#6162=VECTOR('',#51965,0.948084450180161);
#6163=VECTOR('',#51970,0.500000000000167);
#6164=VECTOR('',#51973,1.02140828085134);
#6165=VECTOR('',#51978,0.499999999999944);
#6166=VECTOR('',#51981,0.948084450180275);
#6167=VECTOR('',#51986,0.500000000000054);
#6168=VECTOR('',#51989,1.02140828085134);
#6169=VECTOR('',#51994,0.49999999999994);
#6170=VECTOR('',#51997,0.948084450180161);
#6171=VECTOR('',#52002,0.500000000000054);
#6172=VECTOR('',#52005,1.02140828085145);
#6173=VECTOR('',#52010,0.500000000000054);
#6174=VECTOR('',#52013,0.948084450180157);
#6175=VECTOR('',#52018,0.500000000000049);
#6176=VECTOR('',#52021,1.02140828085145);
#6177=VECTOR('',#52026,0.500000000000054);
#6178=VECTOR('',#52029,0.948084450180157);
#6179=VECTOR('',#52034,0.500000000000054);
#6180=VECTOR('',#52037,1.02140828085134);
#6181=VECTOR('',#52042,0.500000000000049);
#6182=VECTOR('',#52045,0.948084450180157);
#6183=VECTOR('',#52050,0.500000000000049);
#6184=VECTOR('',#52053,1.02140828085145);
#6185=VECTOR('',#52058,0.500000000000058);
#6186=VECTOR('',#52061,0.948084450180161);
#6187=VECTOR('',#52066,0.499999999999944);
#6188=VECTOR('',#52069,1.02140828085133);
#6189=VECTOR('',#52074,0.499999999999935);
#6190=VECTOR('',#52077,0.948084450180047);
#6191=VECTOR('',#52082,0.499999999999944);
#6192=VECTOR('',#52087,1.54967110260237);
#6193=VECTOR('',#52092,0.49999999999994);
#6194=VECTOR('',#52099,1.25936103546568);
#6195=VECTOR('',#52104,0.500000000000049);
#6196=VECTOR('',#52109,1.02140828085145);
#6197=VECTOR('',#52114,0.49999999999994);
#6198=VECTOR('',#52117,0.948084450179934);
#6199=VECTOR('',#52122,0.49999999999994);
#6200=VECTOR('',#52127,1.54967110260249);
#6201=VECTOR('',#52132,0.499999999999944);
#6202=VECTOR('',#52139,1.25936103546569);
#6203=VECTOR('',#52144,0.500000000000058);
#6204=VECTOR('',#52149,1.02140828085145);
#6205=VECTOR('',#52154,0.500000000000058);
#6206=VECTOR('',#52157,0.948084450180166);
#6207=VECTOR('',#52162,0.500000000000054);
#6208=VECTOR('',#52167,1.25936103546568);
#6209=VECTOR('',#52172,0.500000000000054);
#6210=VECTOR('',#52177,1.02140828085145);
#6211=VECTOR('',#52182,0.500000000000058);
#6212=VECTOR('',#52185,0.948084450180275);
#6213=VECTOR('',#52190,0.500000000000058);
#6214=VECTOR('',#52195,1.25936103546568);
#6215=VECTOR('',#52200,0.49999999999994);
#6216=VECTOR('',#52205,1.02140828085145);
#6217=VECTOR('',#52210,0.500000000000058);
#6218=VECTOR('',#52213,0.948084450180162);
#6219=VECTOR('',#52218,0.49999999999994);
#6220=VECTOR('',#52221,1.02140828085133);
#6221=VECTOR('',#52226,0.499999999999944);
#6222=VECTOR('',#52229,0.948084450180166);
#6223=VECTOR('',#52234,0.499999999999944);
#6224=VECTOR('',#52237,1.02140828085146);
#6225=VECTOR('',#52242,0.500000000000058);
#6226=VECTOR('',#52245,0.948084450180161);
#6227=VECTOR('',#52250,0.500000000000054);
#6228=VECTOR('',#52253,1.02140828085144);
#6229=VECTOR('',#52258,0.499999999999944);
#6230=VECTOR('',#52261,0.948084450180157);
#6231=VECTOR('',#52266,0.500000000000063);
#6232=VECTOR('',#52269,1.02140828085156);
#6233=VECTOR('',#52274,0.49999999999994);
#6234=VECTOR('',#52277,0.948084450180161);
#6235=VECTOR('',#52282,0.500000000000054);
#6236=VECTOR('',#52285,1.02140828085134);
#6237=VECTOR('',#52290,0.500000000000054);
#6238=VECTOR('',#52293,0.948084450180157);
#6239=VECTOR('',#52298,0.49999999999994);
#6240=VECTOR('',#52301,0.948084450180161);
#6241=VECTOR('',#52306,0.500000000000054);
#6242=VECTOR('',#52309,1.02140828085134);
#6243=VECTOR('',#52314,0.499999999999944);
#6244=VECTOR('',#52319,1.0588834746273);
#6245=VECTOR('',#52326,0.500000000000054);
#6246=VECTOR('',#52333,1.29583333162394);
#6247=VECTOR('',#52340,0.500000000000054);
#6248=VECTOR('',#52347,1.60653900437062);
#6249=VECTOR('',#52354,0.500000000000054);
#6250=VECTOR('',#52361,1.82809807486272);
#6251=VECTOR('',#52368,0.499999999999944);
#6252=VECTOR('',#52375,1.85841829658605);
#6253=VECTOR('',#52382,0.500000000000054);
#6254=VECTOR('',#52389,1.81285717707166);
#6255=VECTOR('',#52396,0.500000000000054);
#6256=VECTOR('',#52403,1.91146602029503);
#6257=VECTOR('',#52410,0.500000000000054);
#6258=VECTOR('',#52417,1.54967110260249);
#6259=VECTOR('',#52424,0.499999999999944);
#6260=VECTOR('',#52431,1.25936103546568);
#6261=VECTOR('',#52438,0.500000000000054);
#6262=VECTOR('',#52445,1.0588834746273);
#6263=VECTOR('',#52452,0.500000000000054);
#6264=VECTOR('',#52459,1.29583333162394);
#6265=VECTOR('',#52466,0.499999999999944);
#6266=VECTOR('',#52473,1.60653900437062);
#6267=VECTOR('',#52480,0.500000000000054);
#6268=VECTOR('',#52487,1.82809807486272);
#6269=VECTOR('',#52494,0.499999999999944);
#6270=VECTOR('',#52501,1.85841829658605);
#6271=VECTOR('',#52508,0.499999999999944);
#6272=VECTOR('',#52515,1.81285717707166);
#6273=VECTOR('',#52522,0.499999999999944);
#6274=VECTOR('',#52529,1.91146602029502);
#6275=VECTOR('',#52536,0.500000000000054);
#6276=VECTOR('',#52543,1.54967110260249);
#6277=VECTOR('',#52550,0.499999999999944);
#6278=VECTOR('',#52557,1.25936103546569);
#6279=VECTOR('',#52564,0.500000000000054);
#6280=VECTOR('',#52571,1.0588834746273);
#6281=VECTOR('',#52578,0.499999999999935);
#6282=VECTOR('',#52585,1.29583333162394);
#6283=VECTOR('',#52592,0.500000000000054);
#6284=VECTOR('',#52599,1.60653900437051);
#6285=VECTOR('',#52606,0.499999999999935);
#6286=VECTOR('',#52613,1.82809807486262);
#6287=VECTOR('',#52620,0.500000000000049);
#6288=VECTOR('',#52627,1.85841829658605);
#6289=VECTOR('',#52634,0.500000000000054);
#6290=VECTOR('',#52641,1.91146602029503);
#6291=VECTOR('',#52648,0.500000000000049);
#6292=VECTOR('',#52655,1.54967110260249);
#6293=VECTOR('',#52662,0.500000000000058);
#6294=VECTOR('',#52669,1.25936103546568);
#6295=VECTOR('',#52676,0.500000000000049);
#6296=VECTOR('',#52683,1.05888347462729);
#6297=VECTOR('',#52690,0.500000000000049);
#6298=VECTOR('',#52697,1.29583333162383);
#6299=VECTOR('',#52704,0.499999999999826);
#6300=VECTOR('',#52711,1.60653900437051);
#6301=VECTOR('',#52718,0.500000000000054);
#6302=VECTOR('',#52725,1.82809807486273);
#6303=VECTOR('',#52732,0.500000000000049);
#6304=VECTOR('',#52739,1.85841829658606);
#6305=VECTOR('',#52746,0.500000000000049);
#6306=VECTOR('',#52753,1.81285717707167);
#6307=VECTOR('',#52760,0.499999999999944);
#6308=VECTOR('',#52767,1.91146602029503);
#6309=VECTOR('',#52774,0.500000000000058);
#6310=VECTOR('',#52781,1.5496711026026);
#6311=VECTOR('',#52788,0.500000000000058);
#6312=VECTOR('',#52795,1.25936103546569);
#6313=VECTOR('',#52802,0.500000000000049);
#6314=VECTOR('',#52809,1.05888347462741);
#6315=VECTOR('',#52816,0.500000000000054);
#6316=VECTOR('',#52823,1.29583333162417);
#6317=VECTOR('',#52830,0.500000000000177);
#6318=VECTOR('',#52837,1.60653900437062);
#6319=VECTOR('',#52844,0.500000000000063);
#6320=VECTOR('',#52851,1.82809807486272);
#6321=VECTOR('',#52858,0.500000000000054);
#6322=VECTOR('',#52865,1.85841829658605);
#6323=VECTOR('',#52872,0.499999999999935);
#6324=VECTOR('',#52879,1.81285717707167);
#6325=VECTOR('',#52886,0.499999999999944);
#6326=VECTOR('',#52893,1.91146602029502);
#6327=VECTOR('',#52900,0.499999999999935);
#6328=VECTOR('',#52907,1.54967110260249);
#6329=VECTOR('',#52914,0.499999999999935);
#6330=VECTOR('',#52921,1.25936103546568);
#6331=VECTOR('',#52928,0.500000000000058);
#6332=VECTOR('',#52935,1.05888347462741);
#6333=VECTOR('',#52942,0.500000000000054);
#6334=VECTOR('',#52949,1.29583333162394);
#6335=VECTOR('',#52956,0.49999999999994);
#6336=VECTOR('',#52963,1.60653900437051);
#6337=VECTOR('',#52970,0.49999999999994);
#6338=VECTOR('',#52977,1.82809807486272);
#6339=VECTOR('',#52984,0.499999999999935);
#6340=VECTOR('',#52991,1.85841829658605);
#6341=VECTOR('',#52998,0.500000000000049);
#6342=VECTOR('',#53005,1.81285717707144);
#6343=VECTOR('',#53012,0.499999999999821);
#6344=VECTOR('',#53019,1.9114660202949);
#6345=VECTOR('',#53026,0.499999999999935);
#6346=VECTOR('',#53033,1.54967110260237);
#6347=VECTOR('',#53040,0.500000000000049);
#6348=VECTOR('',#53047,1.25936103546556);
#6349=VECTOR('',#53054,0.499999999999821);
#6350=VECTOR('',#53061,1.0588834746273);
#6351=VECTOR('',#53068,0.500000000000058);
#6352=VECTOR('',#53075,1.29583333162394);
#6353=VECTOR('',#53082,0.500000000000058);
#6354=VECTOR('',#53089,1.60653900437062);
#6355=VECTOR('',#53096,0.499999999999944);
#6356=VECTOR('',#53103,1.82809807486284);
#6357=VECTOR('',#53110,0.500000000000172);
#6358=VECTOR('',#53117,1.85841829658605);
#6359=VECTOR('',#53124,0.500000000000058);
#6360=VECTOR('',#53131,1.81285717707155);
#6361=VECTOR('',#53138,0.500000000000058);
#6362=VECTOR('',#53145,1.91146602029503);
#6363=VECTOR('',#53152,0.499999999999944);
#6364=VECTOR('',#53159,1.5496711026025);
#6365=VECTOR('',#53166,0.499999999999944);
#6366=VECTOR('',#53173,1.2593610354658);
#6367=VECTOR('',#53180,0.500000000000172);
#6368=VECTOR('',#53187,1.0588834746273);
#6369=VECTOR('',#53194,0.49999999999994);
#6370=VECTOR('',#53201,1.29583333162394);
#6371=VECTOR('',#53208,0.499999999999944);
#6372=VECTOR('',#53215,1.60653900437051);
#6373=VECTOR('',#53222,0.499999999999944);
#6374=VECTOR('',#53229,1.82809807486261);
#6375=VECTOR('',#53236,0.49999999999994);
#6376=VECTOR('',#53243,1.85841829658593);
#6377=VECTOR('',#53250,0.49999999999994);
#6378=VECTOR('',#53257,1.91146602029514);
#6379=VECTOR('',#53264,0.500000000000058);
#6380=VECTOR('',#53271,1.54967110260249);
#6381=VECTOR('',#53278,0.499999999999935);
#6382=VECTOR('',#53285,1.25936103546568);
#6383=VECTOR('',#53292,0.499999999999944);
#6384=VECTOR('',#53299,1.05888347462741);
#6385=VECTOR('',#53306,0.500000000000058);
#6386=VECTOR('',#53313,1.29583333162394);
#6387=VECTOR('',#53320,0.49999999999994);
#6388=VECTOR('',#53327,1.60653900437051);
#6389=VECTOR('',#53334,0.500000000000058);
#6390=VECTOR('',#53341,1.82809807486273);
#6391=VECTOR('',#53348,0.500000000000058);
#6392=VECTOR('',#53355,1.85841829658593);
#6393=VECTOR('',#53362,0.500000000000058);
#6394=VECTOR('',#53369,1.81285717707167);
#6395=VECTOR('',#53376,0.500000000000058);
#6396=VECTOR('',#53383,1.91146602029491);
#6397=VECTOR('',#53390,0.499999999999944);
#6398=VECTOR('',#53397,1.54967110260237);
#6399=VECTOR('',#53404,0.499999999999935);
#6400=VECTOR('',#53411,1.25936103546569);
#6401=VECTOR('',#53418,0.500000000000058);
#6402=VECTOR('',#53425,1.05888347462741);
#6403=VECTOR('',#53432,0.500000000000054);
#6404=VECTOR('',#53439,1.29583333162383);
#6405=VECTOR('',#53446,0.500000000000054);
#6406=VECTOR('',#53453,1.60653900437062);
#6407=VECTOR('',#53460,0.499999999999935);
#6408=VECTOR('',#53467,1.82809807486272);
#6409=VECTOR('',#53474,0.499999999999935);
#6410=VECTOR('',#53481,1.85841829658616);
#6411=VECTOR('',#53488,0.500000000000054);
#6412=VECTOR('',#53495,1.81285717707168);
#6413=VECTOR('',#53502,0.500000000000054);
#6414=VECTOR('',#53509,1.91146602029514);
#6415=VECTOR('',#53516,0.500000000000054);
#6416=VECTOR('',#53523,1.5496711026025);
#6417=VECTOR('',#53530,0.500000000000049);
#6418=VECTOR('',#53537,1.25936103546568);
#6419=VECTOR('',#53544,0.500000000000049);
#6420=VECTOR('',#53551,1.05888347462729);
#6421=VECTOR('',#53558,0.500000000000058);
#6422=VECTOR('',#53565,1.29583333162394);
#6423=VECTOR('',#53572,0.49999999999994);
#6424=VECTOR('',#53579,1.60653900437051);
#6425=VECTOR('',#53586,0.49999999999994);
#6426=VECTOR('',#53593,1.82809807486273);
#6427=VECTOR('',#53600,0.49999999999994);
#6428=VECTOR('',#53607,1.85841829658616);
#6429=VECTOR('',#53614,0.500000000000054);
#6430=VECTOR('',#53621,1.81285717707166);
#6431=VECTOR('',#53628,0.499999999999821);
#6432=VECTOR('',#53635,1.91146602029503);
#6433=VECTOR('',#53642,0.499999999999821);
#6434=VECTOR('',#53649,1.54967110260249);
#6435=VECTOR('',#53656,0.500000000000054);
#6436=VECTOR('',#53663,1.25936103546579);
#6437=VECTOR('',#53670,0.500000000000058);
#6438=VECTOR('',#53677,1.0588834746273);
#6439=VECTOR('',#53684,0.500000000000058);
#6440=VECTOR('',#53691,1.29583333162395);
#6441=VECTOR('',#53698,0.499999999999935);
#6442=VECTOR('',#53705,1.60653900437051);
#6443=VECTOR('',#53712,0.500000000000054);
#6444=VECTOR('',#53719,1.82809807486273);
#6445=VECTOR('',#53726,0.500000000000063);
#6446=VECTOR('',#53733,1.85841829658605);
#6447=VECTOR('',#53740,0.499999999999821);
#6448=VECTOR('',#53747,1.81285717707144);
#6449=VECTOR('',#53754,0.499999999999821);
#6450=VECTOR('',#53761,1.91146602029503);
#6451=VECTOR('',#53768,0.500000000000054);
#6452=VECTOR('',#53775,1.54967110260249);
#6453=VECTOR('',#53782,0.499999999999944);
#6454=VECTOR('',#53789,1.25936103546568);
#6455=VECTOR('',#53796,0.499999999999944);
#6456=VECTOR('',#53803,1.0588834746273);
#6457=VECTOR('',#53810,0.500000000000054);
#6458=VECTOR('',#53817,1.29583333162382);
#6459=VECTOR('',#53824,0.499999999999826);
#6460=VECTOR('',#53831,1.60653900437062);
#6461=VECTOR('',#53838,0.500000000000058);
#6462=VECTOR('',#53845,1.82809807486272);
#6463=VECTOR('',#53852,0.499999999999944);
#6464=VECTOR('',#53859,1.85841829658605);
#6465=VECTOR('',#53866,0.49999999999994);
#6466=VECTOR('',#53873,1.9114660202949);
#6467=VECTOR('',#53880,0.499999999999821);
#6468=VECTOR('',#53887,1.54967110260249);
#6469=VECTOR('',#53894,0.500000000000054);
#6470=VECTOR('',#53901,1.25936103546569);
#6471=VECTOR('',#53908,0.49999999999994);
#6472=VECTOR('',#53915,1.05888347462729);
#6473=VECTOR('',#53922,0.500000000000054);
#6474=VECTOR('',#53929,1.29583333162371);
#6475=VECTOR('',#53936,0.499999999999935);
#6476=VECTOR('',#53943,1.60653900437051);
#6477=VECTOR('',#53950,0.499999999999944);
#6478=VECTOR('',#53957,1.82809807486262);
#6479=VECTOR('',#53964,0.500000000000058);
#6480=VECTOR('',#53971,1.85841829658605);
#6481=VECTOR('',#53978,0.499999999999944);
#6482=VECTOR('',#53985,1.81285717707166);
#6483=VECTOR('',#53992,0.499999999999944);
#6484=VECTOR('',#53999,1.91146602029514);
#6485=VECTOR('',#54006,0.500000000000054);
#6486=VECTOR('',#54013,1.54967110260238);
#6487=VECTOR('',#54020,0.499999999999935);
#6488=VECTOR('',#54027,1.25936103546568);
#6489=VECTOR('',#54034,0.49999999999994);
#6490=VECTOR('',#54041,1.0588834746273);
#6491=VECTOR('',#54048,0.499999999999944);
#6492=VECTOR('',#54055,1.29583333162395);
#6493=VECTOR('',#54062,0.500000000000054);
#6494=VECTOR('',#54069,1.60653900437063);
#6495=VECTOR('',#54076,0.500000000000054);
#6496=VECTOR('',#54083,1.82809807486273);
#6497=VECTOR('',#54090,0.500000000000058);
#6498=VECTOR('',#54097,1.85841829658594);
#6499=VECTOR('',#54104,0.49999999999994);
#6500=VECTOR('',#54111,1.81285717707156);
#6501=VECTOR('',#54118,0.500000000000058);
#6502=VECTOR('',#54125,1.91146602029491);
#6503=VECTOR('',#54132,0.500000000000054);
#6504=VECTOR('',#54139,1.54967110260249);
#6505=VECTOR('',#54146,0.499999999999944);
#6506=VECTOR('',#54153,1.25936103546568);
#6507=VECTOR('',#54160,0.500000000000058);
#6508=VECTOR('',#54167,1.0588834746273);
#6509=VECTOR('',#54174,0.500000000000054);
#6510=VECTOR('',#54181,1.29583333162394);
#6511=VECTOR('',#54188,0.500000000000054);
#6512=VECTOR('',#54195,1.60653900437062);
#6513=VECTOR('',#54202,0.500000000000054);
#6514=VECTOR('',#54209,1.82809807486272);
#6515=VECTOR('',#54216,0.499999999999944);
#6516=VECTOR('',#54223,1.85841829658605);
#6517=VECTOR('',#54230,0.500000000000054);
#6518=VECTOR('',#54237,1.81285717707167);
#6519=VECTOR('',#54244,0.500000000000054);
#6520=VECTOR('',#54251,1.91146602029503);
#6521=VECTOR('',#54258,0.500000000000049);
#6522=VECTOR('',#54265,1.54967110260249);
#6523=VECTOR('',#54272,0.499999999999944);
#6524=VECTOR('',#54279,1.25936103546569);
#6525=VECTOR('',#54286,0.500000000000054);
#6526=VECTOR('',#54293,1.0588834746274);
#6527=VECTOR('',#54300,0.499999999999944);
#6528=VECTOR('',#54307,1.29583333162394);
#6529=VECTOR('',#54314,0.500000000000054);
#6530=VECTOR('',#54321,1.60653900437062);
#6531=VECTOR('',#54328,0.500000000000054);
#6532=VECTOR('',#54335,1.82809807486272);
#6533=VECTOR('',#54342,0.500000000000054);
#6534=VECTOR('',#54349,1.85841829658605);
#6535=VECTOR('',#54356,0.500000000000049);
#6536=VECTOR('',#54363,1.81285717707167);
#6537=VECTOR('',#54370,0.500000000000054);
#6538=VECTOR('',#54377,1.91146602029502);
#6539=VECTOR('',#54384,0.500000000000054);
#6540=VECTOR('',#54391,1.54967110260249);
#6541=VECTOR('',#54398,0.500000000000054);
#6542=VECTOR('',#54405,1.25936103546568);
#6543=VECTOR('',#54412,0.499999999999944);
#6544=VECTOR('',#54419,1.05888347462741);
#6545=VECTOR('',#54426,0.500000000000054);
#6546=VECTOR('',#54433,1.29583333162394);
#6547=VECTOR('',#54440,0.500000000000054);
#6548=VECTOR('',#54447,1.60653900437062);
#6549=VECTOR('',#54454,0.500000000000054);
#6550=VECTOR('',#54461,1.82809807486261);
#6551=VECTOR('',#54468,0.49999999999994);
#6552=VECTOR('',#54475,1.85841829658605);
#6553=VECTOR('',#54482,0.500000000000054);
#6554=VECTOR('',#54489,1.91146602029503);
#6555=VECTOR('',#54496,0.500000000000054);
#6556=VECTOR('',#54503,1.54967110260249);
#6557=VECTOR('',#54510,0.500000000000054);
#6558=VECTOR('',#54517,1.25936103546568);
#6559=VECTOR('',#54524,0.500000000000054);
#6560=VECTOR('',#54531,1.05888347462729);
#6561=VECTOR('',#54538,0.499999999999935);
#6562=VECTOR('',#54545,1.29583333162395);
#6563=VECTOR('',#54552,0.500000000000063);
#6564=VECTOR('',#54559,1.60653900437062);
#6565=VECTOR('',#54566,0.500000000000054);
#6566=VECTOR('',#54573,1.82809807486273);
#6567=VECTOR('',#54580,0.500000000000058);
#6568=VECTOR('',#54587,1.85841829658605);
#6569=VECTOR('',#54594,0.49999999999994);
#6570=VECTOR('',#54601,1.81285717707167);
#6571=VECTOR('',#54608,0.49999999999994);
#6572=VECTOR('',#54615,1.91146602029491);
#6573=VECTOR('',#54622,0.499999999999826);
#6574=VECTOR('',#54629,1.54967110260249);
#6575=VECTOR('',#54636,0.500000000000054);
#6576=VECTOR('',#54643,1.2593610354658);
#6577=VECTOR('',#54652,0.500000000000058);
#6578=VECTOR('',#54659,1.0588834746273);
#6579=VECTOR('',#54666,0.499999999999935);
#6580=VECTOR('',#54673,1.29583333162395);
#6581=VECTOR('',#54680,0.500000000000054);
#6582=VECTOR('',#54687,1.60653900437074);
#6583=VECTOR('',#54694,0.500000000000058);
#6584=VECTOR('',#54701,1.82809807486272);
#6585=VECTOR('',#54708,0.500000000000054);
#6586=VECTOR('',#54715,1.85841829658616);
#6587=VECTOR('',#54722,0.500000000000167);
#6588=VECTOR('',#54729,1.81285717707155);
#6589=VECTOR('',#54736,0.499999999999935);
#6590=VECTOR('',#54743,1.91146602029503);
#6591=VECTOR('',#54750,0.500000000000054);
#6592=VECTOR('',#54757,1.54967110260249);
#6593=VECTOR('',#54766,0.49999999999994);
#6594=VECTOR('',#54773,1.25936103546556);
#6595=VECTOR('',#54782,0.499999999999821);
#6596=VECTOR('',#54789,1.05888347462729);
#6597=VECTOR('',#54796,0.500000000000058);
#6598=VECTOR('',#54803,1.29583333162382);
#6599=VECTOR('',#54810,0.500000000000054);
#6600=VECTOR('',#54817,1.60653900437074);
#6601=VECTOR('',#54824,0.500000000000063);
#6602=VECTOR('',#54831,1.82809807486272);
#6603=VECTOR('',#54838,0.500000000000054);
#6604=VECTOR('',#54845,1.85841829658605);
#6605=VECTOR('',#54852,0.500000000000049);
#6606=VECTOR('',#54859,1.81285717707166);
#6607=VECTOR('',#54866,0.500000000000049);
#6608=VECTOR('',#54873,1.91146602029503);
#6609=VECTOR('',#54882,0.500000000000054);
#6610=VECTOR('',#54889,1.0588834746273);
#6611=VECTOR('',#54896,0.500000000000058);
#6612=VECTOR('',#54903,1.29583333162395);
#6613=VECTOR('',#54910,0.500000000000058);
#6614=VECTOR('',#54917,1.60653900437063);
#6615=VECTOR('',#54924,0.500000000000058);
#6616=VECTOR('',#54931,1.82809807486273);
#6617=VECTOR('',#54938,0.49999999999994);
#6618=VECTOR('',#54945,1.85841829658605);
#6619=VECTOR('',#54952,0.499999999999935);
#6620=VECTOR('',#54959,1.81285717707167);
#6621=VECTOR('',#54966,0.499999999999944);
#6622=VECTOR('',#54973,1.91146602029503);
#6623=VECTOR('',#54980,0.500000000000167);
#6624=VECTOR('',#54987,1.0588834746273);
#6625=VECTOR('',#54994,0.499999999999944);
#6626=VECTOR('',#55001,1.29583333162394);
#6627=VECTOR('',#55008,0.500000000000054);
#6628=VECTOR('',#55015,1.60653900437062);
#6629=VECTOR('',#55022,0.499999999999944);
#6630=VECTOR('',#55029,1.82809807486273);
#6631=VECTOR('',#55036,0.499999999999944);
#6632=VECTOR('',#55043,1.85841829658605);
#6633=VECTOR('',#55050,0.499999999999944);
#6634=VECTOR('',#55057,1.91146602029503);
#6635=VECTOR('',#55064,0.500000000000058);
#6636=VECTOR('',#55071,1.54967110260249);
#6637=VECTOR('',#55080,0.49999999999994);
#6638=VECTOR('',#55087,1.05888347462741);
#6639=VECTOR('',#55094,0.49999999999994);
#6640=VECTOR('',#55101,1.29583333162394);
#6641=VECTOR('',#55108,0.49999999999994);
#6642=VECTOR('',#55115,1.60653900437063);
#6643=VECTOR('',#55122,0.500000000000058);
#6644=VECTOR('',#55129,1.82809807486273);
#6645=VECTOR('',#55136,0.500000000000058);
#6646=VECTOR('',#55143,1.85841829658593);
#6647=VECTOR('',#55150,0.49999999999994);
#6648=VECTOR('',#55157,1.81285717707155);
#6649=VECTOR('',#55164,0.49999999999994);
#6650=VECTOR('',#55171,1.91146602029503);
#6651=VECTOR('',#55178,0.49999999999994);
#6652=VECTOR('',#55185,1.54967110260237);
#6653=VECTOR('',#55192,0.49999999999994);
#6654=VECTOR('',#55199,1.05888347462729);
#6655=VECTOR('',#55206,0.500000000000054);
#6656=VECTOR('',#55213,1.29583333162383);
#6657=VECTOR('',#55220,0.500000000000054);
#6658=VECTOR('',#55227,1.60653900437051);
#6659=VECTOR('',#55234,0.499999999999935);
#6660=VECTOR('',#55241,1.82809807486262);
#6661=VECTOR('',#55248,0.500000000000063);
#6662=VECTOR('',#55255,1.85841829658605);
#6663=VECTOR('',#55262,0.500000000000054);
#6664=VECTOR('',#55269,1.81285717707166);
#6665=VECTOR('',#55276,0.499999999999935);
#6666=VECTOR('',#55283,1.9114660202949);
#6667=VECTOR('',#55290,0.499999999999935);
#6668=VECTOR('',#55297,1.54967110260238);
#6669=VECTOR('',#55304,0.499999999999935);
#6670=VECTOR('',#55311,1.25936103546556);
#6671=VECTOR('',#55320,0.499999999999935);
#6672=VECTOR('',#55327,1.05888347462741);
#6673=VECTOR('',#55334,0.500000000000058);
#6674=VECTOR('',#55341,1.29583333162406);
#6675=VECTOR('',#55348,0.49999999999994);
#6676=VECTOR('',#55355,1.60653900437063);
#6677=VECTOR('',#55362,0.500000000000058);
#6678=VECTOR('',#55369,1.82809807486262);
#6679=VECTOR('',#55376,0.49999999999994);
#6680=VECTOR('',#55383,1.85841829658593);
#6681=VECTOR('',#55390,0.49999999999994);
#6682=VECTOR('',#55397,1.81285717707179);
#6683=VECTOR('',#55404,0.49999999999994);
#6684=VECTOR('',#55411,1.91146602029502);
#6685=VECTOR('',#55418,0.49999999999994);
#6686=VECTOR('',#55425,1.54967110260249);
#6687=VECTOR('',#55432,0.500000000000058);
#6688=VECTOR('',#55439,1.25936103546569);
#6689=VECTOR('',#55448,0.499999999999935);
#6690=VECTOR('',#55455,1.0588834746273);
#6691=VECTOR('',#55462,0.500000000000054);
#6692=VECTOR('',#55469,1.29583333162406);
#6693=VECTOR('',#55476,0.500000000000177);
#6694=VECTOR('',#55483,1.60653900437051);
#6695=VECTOR('',#55490,0.49999999999994);
#6696=VECTOR('',#55497,1.82809807486261);
#6697=VECTOR('',#55504,0.499999999999944);
#6698=VECTOR('',#55511,1.85841829658594);
#6699=VECTOR('',#55518,0.49999999999994);
#6700=VECTOR('',#55525,1.81285717707156);
#6701=VECTOR('',#55532,0.499999999999944);
#6702=VECTOR('',#55539,1.91146602029503);
#6703=VECTOR('',#55546,0.500000000000054);
#6704=VECTOR('',#55553,1.5496711026026);
#6705=VECTOR('',#55560,0.500000000000058);
#6706=VECTOR('',#55567,1.2593610354658);
#6707=VECTOR('',#55574,0.500000000000063);
#6708=VECTOR('',#55581,1.05888347462741);
#6709=VECTOR('',#55588,0.49999999999994);
#6710=VECTOR('',#55595,1.29583333162395);
#6711=VECTOR('',#55602,0.500000000000054);
#6712=VECTOR('',#55609,1.60653900437063);
#6713=VECTOR('',#55616,0.500000000000167);
#6714=VECTOR('',#55623,1.82809807486262);
#6715=VECTOR('',#55630,0.499999999999944);
#6716=VECTOR('',#55637,1.85841829658605);
#6717=VECTOR('',#55644,0.499999999999944);
#6718=VECTOR('',#55651,1.91146602029502);
#6719=VECTOR('',#55658,0.499999999999944);
#6720=VECTOR('',#55665,1.5496711026026);
#6721=VECTOR('',#55672,0.500000000000054);
#6722=VECTOR('',#55679,1.25936103546567);
#6723=VECTOR('',#55686,0.49999999999994);
#6724=VECTOR('',#55693,1.05888347462741);
#6725=VECTOR('',#55700,0.500000000000054);
#6726=VECTOR('',#55707,1.29583333162394);
#6727=VECTOR('',#55714,0.49999999999994);
#6728=VECTOR('',#55721,1.6065390043705);
#6729=VECTOR('',#55728,0.49999999999994);
#6730=VECTOR('',#55735,1.82809807486261);
#6731=VECTOR('',#55742,0.500000000000054);
#6732=VECTOR('',#55749,1.85841829658593);
#6733=VECTOR('',#55756,0.49999999999994);
#6734=VECTOR('',#55763,1.81285717707167);
#6735=VECTOR('',#55770,0.500000000000058);
#6736=VECTOR('',#55777,1.91146602029503);
#6737=VECTOR('',#55784,0.500000000000054);
#6738=VECTOR('',#55791,1.54967110260249);
#6739=VECTOR('',#55798,0.500000000000058);
#6740=VECTOR('',#55805,1.25936103546568);
#6741=VECTOR('',#55812,0.49999999999994);
#6742=VECTOR('',#55819,1.0588834746273);
#6743=VECTOR('',#55826,0.500000000000054);
#6744=VECTOR('',#55833,1.29583333162383);
#6745=VECTOR('',#55840,0.499999999999935);
#6746=VECTOR('',#55847,1.60653900437062);
#6747=VECTOR('',#55854,0.500000000000058);
#6748=VECTOR('',#55861,1.82809807486272);
#6749=VECTOR('',#55868,0.500000000000058);
#6750=VECTOR('',#55875,1.85841829658594);
#6751=VECTOR('',#55882,0.499999999999826);
#6752=VECTOR('',#55889,1.81285717707156);
#6753=VECTOR('',#55896,0.499999999999944);
#6754=VECTOR('',#55903,1.91146602029502);
#6755=VECTOR('',#55910,0.499999999999935);
#6756=VECTOR('',#55917,1.54967110260249);
#6757=VECTOR('',#55924,0.500000000000054);
#6758=VECTOR('',#55931,1.25936103546568);
#6759=VECTOR('',#55938,0.500000000000054);
#6760=VECTOR('',#56009,8.99091713639496);
#6761=VECTOR('',#56050,1000.);
#6762=VECTOR('',#56053,1000.);
#6763=VECTOR('',#56062,8.99091713639503);
#6764=VECTOR('',#56075,0.500000000000054);
#6765=VECTOR('',#56078,1.02140828085145);
#6766=VECTOR('',#56085,1000.);
#6767=VECTOR('',#56086,10.);
#6768=VECTOR('',#56087,1000.);
#6769=VECTOR('',#56088,1000.);
#6770=VECTOR('',#56093,1000.);
#6771=VECTOR('',#56102,1000.);
#6772=VECTOR('',#56105,1000.);
#6773=VECTOR('',#56108,1000.);
#6774=VECTOR('',#56115,10.);
#6775=VECTOR('',#56116,1000.);
#6776=VECTOR('',#56119,1000.);
#6777=VECTOR('',#56122,1000.);
#6778=VECTOR('',#56127,1000.);
#6779=VECTOR('',#56128,1000.);
#6780=VECTOR('',#56129,1000.);
#6781=VECTOR('',#56130,1000.);
#6782=VECTOR('',#56133,1000.);
#6783=VECTOR('',#56142,1000.);
#6784=VECTOR('',#56147,1000.);
#6785=VECTOR('',#56148,1000.);
#6786=VECTOR('',#56189,10.);
#6787=VECTOR('',#56196,10.);
#6788=VECTOR('',#56229,1000.);
#6789=VECTOR('',#56230,1000.);
#6790=VECTOR('',#56243,10.);
#6791=VECTOR('',#56244,10.);
#6792=VECTOR('',#56281,1000.);
#6793=VECTOR('',#56284,1000.);
#7863=CYLINDRICAL_SURFACE('',#45573,8.3031389659941);
#7864=CYLINDRICAL_SURFACE('',#45576,8.3031389659941);
#7865=CYLINDRICAL_SURFACE('',#45583,8.3031389659941);
#7866=CYLINDRICAL_SURFACE('',#45584,0.500000000000054);
#7867=CYLINDRICAL_SURFACE('',#45587,1.81285717707168);
#7868=CYLINDRICAL_SURFACE('',#45590,0.500000000000054);
#7869=CYLINDRICAL_SURFACE('',#45593,1.81285717707167);
#7870=CYLINDRICAL_SURFACE('',#45596,0.500000000000054);
#7871=CYLINDRICAL_SURFACE('',#45599,1.81285717707166);
#7872=CYLINDRICAL_SURFACE('',#45602,0.499999999999939);
#7873=CYLINDRICAL_SURFACE('',#45605,1.81285717707156);
#7874=CYLINDRICAL_SURFACE('',#45608,0.499999999999935);
#7875=CYLINDRICAL_SURFACE('',#45611,1.81285717707156);
#7876=CYLINDRICAL_SURFACE('',#45614,0.499999999999944);
#7877=CYLINDRICAL_SURFACE('',#45617,1.81285717707167);
#7878=CYLINDRICAL_SURFACE('',#45620,0.948084450180161);
#7879=CYLINDRICAL_SURFACE('',#45621,0.500000000000054);
#7880=CYLINDRICAL_SURFACE('',#45623,1.02140828085145);
#7881=CYLINDRICAL_SURFACE('',#45624,0.500000000000054);
#7882=CYLINDRICAL_SURFACE('',#45626,0.948084450180157);
#7883=CYLINDRICAL_SURFACE('',#45627,0.500000000000054);
#7884=CYLINDRICAL_SURFACE('',#45629,1.02140828085145);
#7885=CYLINDRICAL_SURFACE('',#45630,0.500000000000054);
#7886=CYLINDRICAL_SURFACE('',#45632,0.948084450180157);
#7887=CYLINDRICAL_SURFACE('',#45633,0.500000000000054);
#7888=CYLINDRICAL_SURFACE('',#45635,1.02140828085145);
#7889=CYLINDRICAL_SURFACE('',#45636,0.499999999999944);
#7890=CYLINDRICAL_SURFACE('',#45638,0.948084450180161);
#7891=CYLINDRICAL_SURFACE('',#45639,0.499999999999944);
#7892=CYLINDRICAL_SURFACE('',#45641,1.02140828085144);
#7893=CYLINDRICAL_SURFACE('',#45642,0.500000000000058);
#7894=CYLINDRICAL_SURFACE('',#45644,0.948084450180161);
#7895=CYLINDRICAL_SURFACE('',#45645,0.500000000000058);
#7896=CYLINDRICAL_SURFACE('',#45647,1.02140828085145);
#7897=CYLINDRICAL_SURFACE('',#45648,0.500000000000058);
#7898=CYLINDRICAL_SURFACE('',#45650,0.948084450180161);
#7899=CYLINDRICAL_SURFACE('',#45651,0.500000000000172);
#7900=CYLINDRICAL_SURFACE('',#45653,1.02140828085157);
#7901=CYLINDRICAL_SURFACE('',#45654,0.499999999999935);
#7902=CYLINDRICAL_SURFACE('',#45656,0.948084450180161);
#7903=CYLINDRICAL_SURFACE('',#45657,0.500000000000058);
#7904=CYLINDRICAL_SURFACE('',#45659,1.02140828085134);
#7905=CYLINDRICAL_SURFACE('',#45660,0.499999999999935);
#7906=CYLINDRICAL_SURFACE('',#45662,0.948084450180275);
#7907=CYLINDRICAL_SURFACE('',#45663,0.500000000000058);
#7908=CYLINDRICAL_SURFACE('',#45665,1.02140828085134);
#7909=CYLINDRICAL_SURFACE('',#45666,0.500000000000058);
#7910=CYLINDRICAL_SURFACE('',#45668,0.948084450180152);
#7911=CYLINDRICAL_SURFACE('',#45669,0.499999999999944);
#7912=CYLINDRICAL_SURFACE('',#45671,1.02140828085157);
#7913=CYLINDRICAL_SURFACE('',#45672,0.500000000000067);
#7914=CYLINDRICAL_SURFACE('',#45674,0.948084450180047);
#7915=CYLINDRICAL_SURFACE('',#45675,0.499999999999935);
#7916=CYLINDRICAL_SURFACE('',#45677,1.02140828085145);
#7917=CYLINDRICAL_SURFACE('',#45678,0.499999999999935);
#7918=CYLINDRICAL_SURFACE('',#45680,0.94808445018017);
#7919=CYLINDRICAL_SURFACE('',#45681,0.500000000000058);
#7920=CYLINDRICAL_SURFACE('',#45683,1.02140828085121);
#7921=CYLINDRICAL_SURFACE('',#45684,0.499999999999944);
#7922=CYLINDRICAL_SURFACE('',#45686,0.948084450180161);
#7923=CYLINDRICAL_SURFACE('',#45687,0.499999999999944);
#7924=CYLINDRICAL_SURFACE('',#45689,1.02140828085145);
#7925=CYLINDRICAL_SURFACE('',#45690,0.499999999999939);
#7926=CYLINDRICAL_SURFACE('',#45692,0.948084450180161);
#7927=CYLINDRICAL_SURFACE('',#45693,0.500000000000167);
#7928=CYLINDRICAL_SURFACE('',#45695,1.02140828085134);
#7929=CYLINDRICAL_SURFACE('',#45696,0.499999999999944);
#7930=CYLINDRICAL_SURFACE('',#45698,0.948084450180275);
#7931=CYLINDRICAL_SURFACE('',#45699,0.500000000000054);
#7932=CYLINDRICAL_SURFACE('',#45701,1.02140828085134);
#7933=CYLINDRICAL_SURFACE('',#45702,0.499999999999939);
#7934=CYLINDRICAL_SURFACE('',#45704,0.948084450180161);
#7935=CYLINDRICAL_SURFACE('',#45705,0.500000000000054);
#7936=CYLINDRICAL_SURFACE('',#45707,1.02140828085145);
#7937=CYLINDRICAL_SURFACE('',#45708,0.500000000000054);
#7938=CYLINDRICAL_SURFACE('',#45710,0.948084450180157);
#7939=CYLINDRICAL_SURFACE('',#45711,0.500000000000049);
#7940=CYLINDRICAL_SURFACE('',#45713,1.02140828085145);
#7941=CYLINDRICAL_SURFACE('',#45714,0.500000000000054);
#7942=CYLINDRICAL_SURFACE('',#45716,0.948084450180157);
#7943=CYLINDRICAL_SURFACE('',#45717,0.500000000000054);
#7944=CYLINDRICAL_SURFACE('',#45719,1.02140828085134);
#7945=CYLINDRICAL_SURFACE('',#45720,0.500000000000049);
#7946=CYLINDRICAL_SURFACE('',#45722,0.948084450180157);
#7947=CYLINDRICAL_SURFACE('',#45723,0.500000000000049);
#7948=CYLINDRICAL_SURFACE('',#45725,1.02140828085145);
#7949=CYLINDRICAL_SURFACE('',#45726,0.500000000000058);
#7950=CYLINDRICAL_SURFACE('',#45728,0.948084450180161);
#7951=CYLINDRICAL_SURFACE('',#45729,0.499999999999944);
#7952=CYLINDRICAL_SURFACE('',#45731,1.02140828085133);
#7953=CYLINDRICAL_SURFACE('',#45732,0.499999999999935);
#7954=CYLINDRICAL_SURFACE('',#45734,0.948084450180047);
#7955=CYLINDRICAL_SURFACE('',#45735,0.499999999999944);
#7956=CYLINDRICAL_SURFACE('',#45737,1.54967110260237);
#7957=CYLINDRICAL_SURFACE('',#45739,0.499999999999939);
#7958=CYLINDRICAL_SURFACE('',#45742,1.25936103546568);
#7959=CYLINDRICAL_SURFACE('',#45744,0.500000000000049);
#7960=CYLINDRICAL_SURFACE('',#45747,1.02140828085145);
#7961=CYLINDRICAL_SURFACE('',#45748,0.499999999999939);
#7962=CYLINDRICAL_SURFACE('',#45750,0.948084450179933);
#7963=CYLINDRICAL_SURFACE('',#45751,0.499999999999939);
#7964=CYLINDRICAL_SURFACE('',#45753,1.54967110260249);
#7965=CYLINDRICAL_SURFACE('',#45755,0.499999999999944);
#7966=CYLINDRICAL_SURFACE('',#45758,1.25936103546569);
#7967=CYLINDRICAL_SURFACE('',#45760,0.500000000000058);
#7968=CYLINDRICAL_SURFACE('',#45763,1.02140828085145);
#7969=CYLINDRICAL_SURFACE('',#45764,0.500000000000058);
#7970=CYLINDRICAL_SURFACE('',#45766,0.948084450180166);
#7971=CYLINDRICAL_SURFACE('',#45767,0.500000000000054);
#7972=CYLINDRICAL_SURFACE('',#45769,1.25936103546568);
#7973=CYLINDRICAL_SURFACE('',#45771,0.500000000000054);
#7974=CYLINDRICAL_SURFACE('',#45774,1.02140828085145);
#7975=CYLINDRICAL_SURFACE('',#45775,0.500000000000058);
#7976=CYLINDRICAL_SURFACE('',#45777,0.948084450180275);
#7977=CYLINDRICAL_SURFACE('',#45778,0.500000000000058);
#7978=CYLINDRICAL_SURFACE('',#45780,1.25936103546568);
#7979=CYLINDRICAL_SURFACE('',#45782,0.499999999999939);
#7980=CYLINDRICAL_SURFACE('',#45785,1.02140828085145);
#7981=CYLINDRICAL_SURFACE('',#45786,0.500000000000058);
#7982=CYLINDRICAL_SURFACE('',#45788,0.948084450180161);
#7983=CYLINDRICAL_SURFACE('',#45789,0.499999999999939);
#7984=CYLINDRICAL_SURFACE('',#45791,1.02140828085133);
#7985=CYLINDRICAL_SURFACE('',#45792,0.499999999999944);
#7986=CYLINDRICAL_SURFACE('',#45794,0.948084450180166);
#7987=CYLINDRICAL_SURFACE('',#45795,0.499999999999944);
#7988=CYLINDRICAL_SURFACE('',#45797,1.02140828085146);
#7989=CYLINDRICAL_SURFACE('',#45798,0.500000000000058);
#7990=CYLINDRICAL_SURFACE('',#45800,0.948084450180161);
#7991=CYLINDRICAL_SURFACE('',#45801,0.500000000000054);
#7992=CYLINDRICAL_SURFACE('',#45803,1.02140828085144);
#7993=CYLINDRICAL_SURFACE('',#45804,0.499999999999944);
#7994=CYLINDRICAL_SURFACE('',#45806,0.948084450180157);
#7995=CYLINDRICAL_SURFACE('',#45807,0.500000000000063);
#7996=CYLINDRICAL_SURFACE('',#45809,1.02140828085156);
#7997=CYLINDRICAL_SURFACE('',#45810,0.499999999999939);
#7998=CYLINDRICAL_SURFACE('',#45812,0.948084450180161);
#7999=CYLINDRICAL_SURFACE('',#45813,0.500000000000054);
#8000=CYLINDRICAL_SURFACE('',#45815,1.02140828085134);
#8001=CYLINDRICAL_SURFACE('',#45816,0.500000000000054);
#8002=CYLINDRICAL_SURFACE('',#45818,0.948084450180157);
#8003=CYLINDRICAL_SURFACE('',#45819,0.499999999999939);
#8004=CYLINDRICAL_SURFACE('',#45821,0.948084450180161);
#8005=CYLINDRICAL_SURFACE('',#45822,0.500000000000054);
#8006=CYLINDRICAL_SURFACE('',#45824,1.02140828085134);
#8007=CYLINDRICAL_SURFACE('',#45825,0.499999999999944);
#8008=CYLINDRICAL_SURFACE('',#45827,1.0588834746273);
#8009=CYLINDRICAL_SURFACE('',#45830,0.500000000000054);
#8010=CYLINDRICAL_SURFACE('',#45833,1.29583333162394);
#8011=CYLINDRICAL_SURFACE('',#45836,0.500000000000054);
#8012=CYLINDRICAL_SURFACE('',#45839,1.60653900437062);
#8013=CYLINDRICAL_SURFACE('',#45842,0.500000000000054);
#8014=CYLINDRICAL_SURFACE('',#45845,1.82809807486272);
#8015=CYLINDRICAL_SURFACE('',#45848,0.499999999999944);
#8016=CYLINDRICAL_SURFACE('',#45851,1.85841829658605);
#8017=CYLINDRICAL_SURFACE('',#45854,0.500000000000054);
#8018=CYLINDRICAL_SURFACE('',#45857,1.81285717707166);
#8019=CYLINDRICAL_SURFACE('',#45860,0.500000000000054);
#8020=CYLINDRICAL_SURFACE('',#45863,1.91146602029503);
#8021=CYLINDRICAL_SURFACE('',#45866,0.500000000000054);
#8022=CYLINDRICAL_SURFACE('',#45869,1.54967110260249);
#8023=CYLINDRICAL_SURFACE('',#45872,0.499999999999944);
#8024=CYLINDRICAL_SURFACE('',#45875,1.25936103546568);
#8025=CYLINDRICAL_SURFACE('',#45878,0.500000000000054);
#8026=CYLINDRICAL_SURFACE('',#45881,1.0588834746273);
#8027=CYLINDRICAL_SURFACE('',#45884,0.500000000000054);
#8028=CYLINDRICAL_SURFACE('',#45887,1.29583333162394);
#8029=CYLINDRICAL_SURFACE('',#45890,0.499999999999944);
#8030=CYLINDRICAL_SURFACE('',#45893,1.60653900437062);
#8031=CYLINDRICAL_SURFACE('',#45896,0.500000000000054);
#8032=CYLINDRICAL_SURFACE('',#45899,1.82809807486272);
#8033=CYLINDRICAL_SURFACE('',#45902,0.499999999999944);
#8034=CYLINDRICAL_SURFACE('',#45905,1.85841829658605);
#8035=CYLINDRICAL_SURFACE('',#45908,0.499999999999944);
#8036=CYLINDRICAL_SURFACE('',#45911,1.81285717707166);
#8037=CYLINDRICAL_SURFACE('',#45914,0.499999999999944);
#8038=CYLINDRICAL_SURFACE('',#45917,1.91146602029502);
#8039=CYLINDRICAL_SURFACE('',#45920,0.500000000000054);
#8040=CYLINDRICAL_SURFACE('',#45923,1.54967110260249);
#8041=CYLINDRICAL_SURFACE('',#45926,0.499999999999944);
#8042=CYLINDRICAL_SURFACE('',#45929,1.25936103546569);
#8043=CYLINDRICAL_SURFACE('',#45932,0.500000000000054);
#8044=CYLINDRICAL_SURFACE('',#45935,1.0588834746273);
#8045=CYLINDRICAL_SURFACE('',#45938,0.499999999999935);
#8046=CYLINDRICAL_SURFACE('',#45941,1.29583333162394);
#8047=CYLINDRICAL_SURFACE('',#45944,0.500000000000054);
#8048=CYLINDRICAL_SURFACE('',#45947,1.60653900437051);
#8049=CYLINDRICAL_SURFACE('',#45950,0.499999999999935);
#8050=CYLINDRICAL_SURFACE('',#45953,1.82809807486262);
#8051=CYLINDRICAL_SURFACE('',#45956,0.500000000000049);
#8052=CYLINDRICAL_SURFACE('',#45959,1.85841829658605);
#8053=CYLINDRICAL_SURFACE('',#45962,0.500000000000054);
#8054=CYLINDRICAL_SURFACE('',#45965,1.91146602029503);
#8055=CYLINDRICAL_SURFACE('',#45968,0.500000000000049);
#8056=CYLINDRICAL_SURFACE('',#45971,1.54967110260249);
#8057=CYLINDRICAL_SURFACE('',#45974,0.500000000000058);
#8058=CYLINDRICAL_SURFACE('',#45977,1.25936103546568);
#8059=CYLINDRICAL_SURFACE('',#45980,0.500000000000049);
#8060=CYLINDRICAL_SURFACE('',#45983,1.05888347462729);
#8061=CYLINDRICAL_SURFACE('',#45986,0.500000000000049);
#8062=CYLINDRICAL_SURFACE('',#45989,1.29583333162383);
#8063=CYLINDRICAL_SURFACE('',#45992,0.499999999999826);
#8064=CYLINDRICAL_SURFACE('',#45995,1.60653900437051);
#8065=CYLINDRICAL_SURFACE('',#45998,0.500000000000054);
#8066=CYLINDRICAL_SURFACE('',#46001,1.82809807486273);
#8067=CYLINDRICAL_SURFACE('',#46004,0.500000000000049);
#8068=CYLINDRICAL_SURFACE('',#46007,1.85841829658605);
#8069=CYLINDRICAL_SURFACE('',#46010,0.500000000000049);
#8070=CYLINDRICAL_SURFACE('',#46013,1.81285717707167);
#8071=CYLINDRICAL_SURFACE('',#46016,0.499999999999944);
#8072=CYLINDRICAL_SURFACE('',#46019,1.91146602029503);
#8073=CYLINDRICAL_SURFACE('',#46022,0.500000000000058);
#8074=CYLINDRICAL_SURFACE('',#46025,1.5496711026026);
#8075=CYLINDRICAL_SURFACE('',#46028,0.500000000000058);
#8076=CYLINDRICAL_SURFACE('',#46031,1.25936103546569);
#8077=CYLINDRICAL_SURFACE('',#46034,0.500000000000049);
#8078=CYLINDRICAL_SURFACE('',#46037,1.05888347462741);
#8079=CYLINDRICAL_SURFACE('',#46040,0.500000000000054);
#8080=CYLINDRICAL_SURFACE('',#46043,1.29583333162417);
#8081=CYLINDRICAL_SURFACE('',#46046,0.500000000000177);
#8082=CYLINDRICAL_SURFACE('',#46049,1.60653900437062);
#8083=CYLINDRICAL_SURFACE('',#46052,0.500000000000063);
#8084=CYLINDRICAL_SURFACE('',#46055,1.82809807486272);
#8085=CYLINDRICAL_SURFACE('',#46058,0.500000000000054);
#8086=CYLINDRICAL_SURFACE('',#46061,1.85841829658605);
#8087=CYLINDRICAL_SURFACE('',#46064,0.499999999999935);
#8088=CYLINDRICAL_SURFACE('',#46067,1.81285717707167);
#8089=CYLINDRICAL_SURFACE('',#46070,0.499999999999944);
#8090=CYLINDRICAL_SURFACE('',#46073,1.91146602029502);
#8091=CYLINDRICAL_SURFACE('',#46076,0.499999999999935);
#8092=CYLINDRICAL_SURFACE('',#46079,1.54967110260249);
#8093=CYLINDRICAL_SURFACE('',#46082,0.499999999999935);
#8094=CYLINDRICAL_SURFACE('',#46085,1.25936103546568);
#8095=CYLINDRICAL_SURFACE('',#46088,0.500000000000058);
#8096=CYLINDRICAL_SURFACE('',#46091,1.05888347462741);
#8097=CYLINDRICAL_SURFACE('',#46094,0.500000000000054);
#8098=CYLINDRICAL_SURFACE('',#46097,1.29583333162394);
#8099=CYLINDRICAL_SURFACE('',#46100,0.499999999999939);
#8100=CYLINDRICAL_SURFACE('',#46103,1.60653900437051);
#8101=CYLINDRICAL_SURFACE('',#46106,0.499999999999939);
#8102=CYLINDRICAL_SURFACE('',#46109,1.82809807486272);
#8103=CYLINDRICAL_SURFACE('',#46112,0.499999999999935);
#8104=CYLINDRICAL_SURFACE('',#46115,1.85841829658605);
#8105=CYLINDRICAL_SURFACE('',#46118,0.500000000000049);
#8106=CYLINDRICAL_SURFACE('',#46121,1.81285717707144);
#8107=CYLINDRICAL_SURFACE('',#46124,0.499999999999821);
#8108=CYLINDRICAL_SURFACE('',#46127,1.9114660202949);
#8109=CYLINDRICAL_SURFACE('',#46130,0.499999999999935);
#8110=CYLINDRICAL_SURFACE('',#46133,1.54967110260237);
#8111=CYLINDRICAL_SURFACE('',#46136,0.500000000000049);
#8112=CYLINDRICAL_SURFACE('',#46139,1.25936103546556);
#8113=CYLINDRICAL_SURFACE('',#46142,0.499999999999821);
#8114=CYLINDRICAL_SURFACE('',#46145,1.0588834746273);
#8115=CYLINDRICAL_SURFACE('',#46148,0.500000000000058);
#8116=CYLINDRICAL_SURFACE('',#46151,1.29583333162394);
#8117=CYLINDRICAL_SURFACE('',#46154,0.500000000000058);
#8118=CYLINDRICAL_SURFACE('',#46157,1.60653900437062);
#8119=CYLINDRICAL_SURFACE('',#46160,0.499999999999944);
#8120=CYLINDRICAL_SURFACE('',#46163,1.82809807486284);
#8121=CYLINDRICAL_SURFACE('',#46166,0.500000000000172);
#8122=CYLINDRICAL_SURFACE('',#46169,1.85841829658605);
#8123=CYLINDRICAL_SURFACE('',#46172,0.500000000000058);
#8124=CYLINDRICAL_SURFACE('',#46175,1.81285717707155);
#8125=CYLINDRICAL_SURFACE('',#46178,0.500000000000058);
#8126=CYLINDRICAL_SURFACE('',#46181,1.91146602029503);
#8127=CYLINDRICAL_SURFACE('',#46184,0.499999999999944);
#8128=CYLINDRICAL_SURFACE('',#46187,1.5496711026025);
#8129=CYLINDRICAL_SURFACE('',#46190,0.499999999999944);
#8130=CYLINDRICAL_SURFACE('',#46193,1.2593610354658);
#8131=CYLINDRICAL_SURFACE('',#46196,0.500000000000172);
#8132=CYLINDRICAL_SURFACE('',#46199,1.0588834746273);
#8133=CYLINDRICAL_SURFACE('',#46202,0.499999999999939);
#8134=CYLINDRICAL_SURFACE('',#46205,1.29583333162394);
#8135=CYLINDRICAL_SURFACE('',#46208,0.499999999999944);
#8136=CYLINDRICAL_SURFACE('',#46211,1.60653900437051);
#8137=CYLINDRICAL_SURFACE('',#46214,0.499999999999944);
#8138=CYLINDRICAL_SURFACE('',#46217,1.82809807486261);
#8139=CYLINDRICAL_SURFACE('',#46220,0.499999999999939);
#8140=CYLINDRICAL_SURFACE('',#46223,1.85841829658593);
#8141=CYLINDRICAL_SURFACE('',#46226,0.499999999999939);
#8142=CYLINDRICAL_SURFACE('',#46229,1.91146602029514);
#8143=CYLINDRICAL_SURFACE('',#46232,0.500000000000058);
#8144=CYLINDRICAL_SURFACE('',#46235,1.54967110260249);
#8145=CYLINDRICAL_SURFACE('',#46238,0.499999999999935);
#8146=CYLINDRICAL_SURFACE('',#46241,1.25936103546568);
#8147=CYLINDRICAL_SURFACE('',#46244,0.499999999999944);
#8148=CYLINDRICAL_SURFACE('',#46247,1.05888347462741);
#8149=CYLINDRICAL_SURFACE('',#46250,0.500000000000058);
#8150=CYLINDRICAL_SURFACE('',#46253,1.29583333162394);
#8151=CYLINDRICAL_SURFACE('',#46256,0.499999999999939);
#8152=CYLINDRICAL_SURFACE('',#46259,1.60653900437051);
#8153=CYLINDRICAL_SURFACE('',#46262,0.500000000000058);
#8154=CYLINDRICAL_SURFACE('',#46265,1.82809807486273);
#8155=CYLINDRICAL_SURFACE('',#46268,0.500000000000058);
#8156=CYLINDRICAL_SURFACE('',#46271,1.85841829658593);
#8157=CYLINDRICAL_SURFACE('',#46274,0.500000000000058);
#8158=CYLINDRICAL_SURFACE('',#46277,1.81285717707167);
#8159=CYLINDRICAL_SURFACE('',#46280,0.500000000000058);
#8160=CYLINDRICAL_SURFACE('',#46283,1.91146602029491);
#8161=CYLINDRICAL_SURFACE('',#46286,0.499999999999944);
#8162=CYLINDRICAL_SURFACE('',#46289,1.54967110260237);
#8163=CYLINDRICAL_SURFACE('',#46292,0.499999999999935);
#8164=CYLINDRICAL_SURFACE('',#46295,1.25936103546569);
#8165=CYLINDRICAL_SURFACE('',#46298,0.500000000000058);
#8166=CYLINDRICAL_SURFACE('',#46301,1.05888347462741);
#8167=CYLINDRICAL_SURFACE('',#46304,0.500000000000054);
#8168=CYLINDRICAL_SURFACE('',#46307,1.29583333162383);
#8169=CYLINDRICAL_SURFACE('',#46310,0.500000000000054);
#8170=CYLINDRICAL_SURFACE('',#46313,1.60653900437062);
#8171=CYLINDRICAL_SURFACE('',#46316,0.499999999999935);
#8172=CYLINDRICAL_SURFACE('',#46319,1.82809807486272);
#8173=CYLINDRICAL_SURFACE('',#46322,0.499999999999935);
#8174=CYLINDRICAL_SURFACE('',#46325,1.85841829658616);
#8175=CYLINDRICAL_SURFACE('',#46328,0.500000000000054);
#8176=CYLINDRICAL_SURFACE('',#46331,1.81285717707168);
#8177=CYLINDRICAL_SURFACE('',#46334,0.500000000000054);
#8178=CYLINDRICAL_SURFACE('',#46337,1.91146602029514);
#8179=CYLINDRICAL_SURFACE('',#46340,0.500000000000054);
#8180=CYLINDRICAL_SURFACE('',#46343,1.5496711026025);
#8181=CYLINDRICAL_SURFACE('',#46346,0.500000000000049);
#8182=CYLINDRICAL_SURFACE('',#46349,1.25936103546568);
#8183=CYLINDRICAL_SURFACE('',#46352,0.500000000000049);
#8184=CYLINDRICAL_SURFACE('',#46355,1.05888347462729);
#8185=CYLINDRICAL_SURFACE('',#46358,0.500000000000058);
#8186=CYLINDRICAL_SURFACE('',#46361,1.29583333162394);
#8187=CYLINDRICAL_SURFACE('',#46364,0.499999999999939);
#8188=CYLINDRICAL_SURFACE('',#46367,1.60653900437051);
#8189=CYLINDRICAL_SURFACE('',#46370,0.499999999999939);
#8190=CYLINDRICAL_SURFACE('',#46373,1.82809807486273);
#8191=CYLINDRICAL_SURFACE('',#46376,0.499999999999939);
#8192=CYLINDRICAL_SURFACE('',#46379,1.85841829658616);
#8193=CYLINDRICAL_SURFACE('',#46382,0.500000000000054);
#8194=CYLINDRICAL_SURFACE('',#46385,1.81285717707166);
#8195=CYLINDRICAL_SURFACE('',#46388,0.499999999999821);
#8196=CYLINDRICAL_SURFACE('',#46391,1.91146602029503);
#8197=CYLINDRICAL_SURFACE('',#46394,0.499999999999821);
#8198=CYLINDRICAL_SURFACE('',#46397,1.54967110260249);
#8199=CYLINDRICAL_SURFACE('',#46400,0.500000000000054);
#8200=CYLINDRICAL_SURFACE('',#46403,1.25936103546579);
#8201=CYLINDRICAL_SURFACE('',#46406,0.500000000000058);
#8202=CYLINDRICAL_SURFACE('',#46409,1.0588834746273);
#8203=CYLINDRICAL_SURFACE('',#46412,0.500000000000058);
#8204=CYLINDRICAL_SURFACE('',#46415,1.29583333162395);
#8205=CYLINDRICAL_SURFACE('',#46418,0.499999999999935);
#8206=CYLINDRICAL_SURFACE('',#46421,1.60653900437051);
#8207=CYLINDRICAL_SURFACE('',#46424,0.500000000000054);
#8208=CYLINDRICAL_SURFACE('',#46427,1.82809807486273);
#8209=CYLINDRICAL_SURFACE('',#46430,0.500000000000063);
#8210=CYLINDRICAL_SURFACE('',#46433,1.85841829658605);
#8211=CYLINDRICAL_SURFACE('',#46436,0.499999999999821);
#8212=CYLINDRICAL_SURFACE('',#46439,1.81285717707144);
#8213=CYLINDRICAL_SURFACE('',#46442,0.499999999999821);
#8214=CYLINDRICAL_SURFACE('',#46445,1.91146602029503);
#8215=CYLINDRICAL_SURFACE('',#46448,0.500000000000054);
#8216=CYLINDRICAL_SURFACE('',#46451,1.54967110260249);
#8217=CYLINDRICAL_SURFACE('',#46454,0.499999999999944);
#8218=CYLINDRICAL_SURFACE('',#46457,1.25936103546568);
#8219=CYLINDRICAL_SURFACE('',#46460,0.499999999999944);
#8220=CYLINDRICAL_SURFACE('',#46463,1.0588834746273);
#8221=CYLINDRICAL_SURFACE('',#46466,0.500000000000054);
#8222=CYLINDRICAL_SURFACE('',#46469,1.29583333162382);
#8223=CYLINDRICAL_SURFACE('',#46472,0.499999999999826);
#8224=CYLINDRICAL_SURFACE('',#46475,1.60653900437062);
#8225=CYLINDRICAL_SURFACE('',#46478,0.500000000000058);
#8226=CYLINDRICAL_SURFACE('',#46481,1.82809807486272);
#8227=CYLINDRICAL_SURFACE('',#46484,0.499999999999944);
#8228=CYLINDRICAL_SURFACE('',#46487,1.85841829658605);
#8229=CYLINDRICAL_SURFACE('',#46490,0.499999999999939);
#8230=CYLINDRICAL_SURFACE('',#46493,1.9114660202949);
#8231=CYLINDRICAL_SURFACE('',#46496,0.499999999999821);
#8232=CYLINDRICAL_SURFACE('',#46499,1.54967110260249);
#8233=CYLINDRICAL_SURFACE('',#46502,0.500000000000054);
#8234=CYLINDRICAL_SURFACE('',#46505,1.25936103546569);
#8235=CYLINDRICAL_SURFACE('',#46508,0.499999999999939);
#8236=CYLINDRICAL_SURFACE('',#46511,1.05888347462729);
#8237=CYLINDRICAL_SURFACE('',#46514,0.500000000000054);
#8238=CYLINDRICAL_SURFACE('',#46517,1.29583333162371);
#8239=CYLINDRICAL_SURFACE('',#46520,0.499999999999935);
#8240=CYLINDRICAL_SURFACE('',#46523,1.60653900437051);
#8241=CYLINDRICAL_SURFACE('',#46526,0.499999999999944);
#8242=CYLINDRICAL_SURFACE('',#46529,1.82809807486262);
#8243=CYLINDRICAL_SURFACE('',#46532,0.500000000000058);
#8244=CYLINDRICAL_SURFACE('',#46535,1.85841829658605);
#8245=CYLINDRICAL_SURFACE('',#46538,0.499999999999944);
#8246=CYLINDRICAL_SURFACE('',#46541,1.81285717707166);
#8247=CYLINDRICAL_SURFACE('',#46544,0.499999999999944);
#8248=CYLINDRICAL_SURFACE('',#46547,1.91146602029514);
#8249=CYLINDRICAL_SURFACE('',#46550,0.500000000000054);
#8250=CYLINDRICAL_SURFACE('',#46553,1.54967110260238);
#8251=CYLINDRICAL_SURFACE('',#46556,0.499999999999935);
#8252=CYLINDRICAL_SURFACE('',#46559,1.25936103546568);
#8253=CYLINDRICAL_SURFACE('',#46562,0.499999999999939);
#8254=CYLINDRICAL_SURFACE('',#46565,1.0588834746273);
#8255=CYLINDRICAL_SURFACE('',#46568,0.499999999999944);
#8256=CYLINDRICAL_SURFACE('',#46571,1.29583333162395);
#8257=CYLINDRICAL_SURFACE('',#46574,0.500000000000054);
#8258=CYLINDRICAL_SURFACE('',#46577,1.60653900437063);
#8259=CYLINDRICAL_SURFACE('',#46580,0.500000000000054);
#8260=CYLINDRICAL_SURFACE('',#46583,1.82809807486273);
#8261=CYLINDRICAL_SURFACE('',#46586,0.500000000000058);
#8262=CYLINDRICAL_SURFACE('',#46589,1.85841829658594);
#8263=CYLINDRICAL_SURFACE('',#46592,0.499999999999939);
#8264=CYLINDRICAL_SURFACE('',#46595,1.81285717707156);
#8265=CYLINDRICAL_SURFACE('',#46598,0.500000000000058);
#8266=CYLINDRICAL_SURFACE('',#46601,1.91146602029491);
#8267=CYLINDRICAL_SURFACE('',#46604,0.500000000000054);
#8268=CYLINDRICAL_SURFACE('',#46607,1.54967110260249);
#8269=CYLINDRICAL_SURFACE('',#46610,0.499999999999944);
#8270=CYLINDRICAL_SURFACE('',#46613,1.25936103546568);
#8271=CYLINDRICAL_SURFACE('',#46616,0.500000000000058);
#8272=CYLINDRICAL_SURFACE('',#46619,1.0588834746273);
#8273=CYLINDRICAL_SURFACE('',#46622,0.500000000000054);
#8274=CYLINDRICAL_SURFACE('',#46625,1.29583333162394);
#8275=CYLINDRICAL_SURFACE('',#46628,0.500000000000054);
#8276=CYLINDRICAL_SURFACE('',#46631,1.60653900437062);
#8277=CYLINDRICAL_SURFACE('',#46634,0.500000000000054);
#8278=CYLINDRICAL_SURFACE('',#46637,1.82809807486272);
#8279=CYLINDRICAL_SURFACE('',#46640,0.499999999999944);
#8280=CYLINDRICAL_SURFACE('',#46643,1.85841829658605);
#8281=CYLINDRICAL_SURFACE('',#46646,0.500000000000054);
#8282=CYLINDRICAL_SURFACE('',#46649,1.81285717707167);
#8283=CYLINDRICAL_SURFACE('',#46652,0.500000000000054);
#8284=CYLINDRICAL_SURFACE('',#46655,1.91146602029503);
#8285=CYLINDRICAL_SURFACE('',#46658,0.500000000000049);
#8286=CYLINDRICAL_SURFACE('',#46661,1.54967110260249);
#8287=CYLINDRICAL_SURFACE('',#46664,0.499999999999944);
#8288=CYLINDRICAL_SURFACE('',#46667,1.25936103546569);
#8289=CYLINDRICAL_SURFACE('',#46670,0.500000000000054);
#8290=CYLINDRICAL_SURFACE('',#46673,1.0588834746274);
#8291=CYLINDRICAL_SURFACE('',#46676,0.499999999999944);
#8292=CYLINDRICAL_SURFACE('',#46679,1.29583333162394);
#8293=CYLINDRICAL_SURFACE('',#46682,0.500000000000054);
#8294=CYLINDRICAL_SURFACE('',#46685,1.60653900437062);
#8295=CYLINDRICAL_SURFACE('',#46688,0.500000000000054);
#8296=CYLINDRICAL_SURFACE('',#46691,1.82809807486272);
#8297=CYLINDRICAL_SURFACE('',#46694,0.500000000000054);
#8298=CYLINDRICAL_SURFACE('',#46697,1.85841829658605);
#8299=CYLINDRICAL_SURFACE('',#46700,0.500000000000049);
#8300=CYLINDRICAL_SURFACE('',#46703,1.81285717707167);
#8301=CYLINDRICAL_SURFACE('',#46706,0.500000000000054);
#8302=CYLINDRICAL_SURFACE('',#46709,1.91146602029502);
#8303=CYLINDRICAL_SURFACE('',#46712,0.500000000000054);
#8304=CYLINDRICAL_SURFACE('',#46715,1.54967110260249);
#8305=CYLINDRICAL_SURFACE('',#46718,0.500000000000054);
#8306=CYLINDRICAL_SURFACE('',#46721,1.25936103546568);
#8307=CYLINDRICAL_SURFACE('',#46724,0.499999999999944);
#8308=CYLINDRICAL_SURFACE('',#46727,1.05888347462741);
#8309=CYLINDRICAL_SURFACE('',#46730,0.500000000000054);
#8310=CYLINDRICAL_SURFACE('',#46733,1.29583333162394);
#8311=CYLINDRICAL_SURFACE('',#46736,0.500000000000054);
#8312=CYLINDRICAL_SURFACE('',#46739,1.60653900437062);
#8313=CYLINDRICAL_SURFACE('',#46742,0.500000000000054);
#8314=CYLINDRICAL_SURFACE('',#46745,1.82809807486262);
#8315=CYLINDRICAL_SURFACE('',#46748,0.499999999999939);
#8316=CYLINDRICAL_SURFACE('',#46751,1.85841829658605);
#8317=CYLINDRICAL_SURFACE('',#46754,0.500000000000054);
#8318=CYLINDRICAL_SURFACE('',#46757,1.91146602029503);
#8319=CYLINDRICAL_SURFACE('',#46760,0.500000000000054);
#8320=CYLINDRICAL_SURFACE('',#46763,1.54967110260249);
#8321=CYLINDRICAL_SURFACE('',#46766,0.500000000000054);
#8322=CYLINDRICAL_SURFACE('',#46769,1.25936103546568);
#8323=CYLINDRICAL_SURFACE('',#46772,0.500000000000054);
#8324=CYLINDRICAL_SURFACE('',#46775,1.05888347462729);
#8325=CYLINDRICAL_SURFACE('',#46778,0.499999999999935);
#8326=CYLINDRICAL_SURFACE('',#46781,1.29583333162395);
#8327=CYLINDRICAL_SURFACE('',#46784,0.500000000000063);
#8328=CYLINDRICAL_SURFACE('',#46787,1.60653900437062);
#8329=CYLINDRICAL_SURFACE('',#46790,0.500000000000054);
#8330=CYLINDRICAL_SURFACE('',#46793,1.82809807486273);
#8331=CYLINDRICAL_SURFACE('',#46796,0.500000000000058);
#8332=CYLINDRICAL_SURFACE('',#46799,1.85841829658605);
#8333=CYLINDRICAL_SURFACE('',#46802,0.499999999999939);
#8334=CYLINDRICAL_SURFACE('',#46805,1.81285717707167);
#8335=CYLINDRICAL_SURFACE('',#46808,0.499999999999939);
#8336=CYLINDRICAL_SURFACE('',#46811,1.91146602029491);
#8337=CYLINDRICAL_SURFACE('',#46814,0.499999999999826);
#8338=CYLINDRICAL_SURFACE('',#46817,1.54967110260249);
#8339=CYLINDRICAL_SURFACE('',#46820,0.500000000000054);
#8340=CYLINDRICAL_SURFACE('',#46823,1.2593610354658);
#8341=CYLINDRICAL_SURFACE('',#46827,0.500000000000058);
#8342=CYLINDRICAL_SURFACE('',#46830,1.0588834746273);
#8343=CYLINDRICAL_SURFACE('',#46833,0.499999999999935);
#8344=CYLINDRICAL_SURFACE('',#46836,1.29583333162395);
#8345=CYLINDRICAL_SURFACE('',#46839,0.500000000000054);
#8346=CYLINDRICAL_SURFACE('',#46842,1.60653900437074);
#8347=CYLINDRICAL_SURFACE('',#46845,0.500000000000058);
#8348=CYLINDRICAL_SURFACE('',#46848,1.82809807486272);
#8349=CYLINDRICAL_SURFACE('',#46851,0.500000000000054);
#8350=CYLINDRICAL_SURFACE('',#46854,1.85841829658616);
#8351=CYLINDRICAL_SURFACE('',#46857,0.500000000000167);
#8352=CYLINDRICAL_SURFACE('',#46860,1.81285717707155);
#8353=CYLINDRICAL_SURFACE('',#46863,0.499999999999935);
#8354=CYLINDRICAL_SURFACE('',#46866,1.91146602029503);
#8355=CYLINDRICAL_SURFACE('',#46869,0.500000000000054);
#8356=CYLINDRICAL_SURFACE('',#46872,1.54967110260249);
#8357=CYLINDRICAL_SURFACE('',#46876,0.499999999999939);
#8358=CYLINDRICAL_SURFACE('',#46879,1.25936103546556);
#8359=CYLINDRICAL_SURFACE('',#46883,0.499999999999821);
#8360=CYLINDRICAL_SURFACE('',#46886,1.05888347462729);
#8361=CYLINDRICAL_SURFACE('',#46889,0.500000000000058);
#8362=CYLINDRICAL_SURFACE('',#46892,1.29583333162382);
#8363=CYLINDRICAL_SURFACE('',#46895,0.500000000000054);
#8364=CYLINDRICAL_SURFACE('',#46898,1.60653900437074);
#8365=CYLINDRICAL_SURFACE('',#46901,0.500000000000063);
#8366=CYLINDRICAL_SURFACE('',#46904,1.82809807486272);
#8367=CYLINDRICAL_SURFACE('',#46907,0.500000000000054);
#8368=CYLINDRICAL_SURFACE('',#46910,1.85841829658605);
#8369=CYLINDRICAL_SURFACE('',#46913,0.500000000000049);
#8370=CYLINDRICAL_SURFACE('',#46916,1.81285717707166);
#8371=CYLINDRICAL_SURFACE('',#46919,0.500000000000049);
#8372=CYLINDRICAL_SURFACE('',#46922,1.91146602029503);
#8373=CYLINDRICAL_SURFACE('',#46926,0.500000000000054);
#8374=CYLINDRICAL_SURFACE('',#46929,1.0588834746273);
#8375=CYLINDRICAL_SURFACE('',#46932,0.500000000000058);
#8376=CYLINDRICAL_SURFACE('',#46935,1.29583333162395);
#8377=CYLINDRICAL_SURFACE('',#46938,0.500000000000058);
#8378=CYLINDRICAL_SURFACE('',#46941,1.60653900437063);
#8379=CYLINDRICAL_SURFACE('',#46944,0.500000000000058);
#8380=CYLINDRICAL_SURFACE('',#46947,1.82809807486273);
#8381=CYLINDRICAL_SURFACE('',#46950,0.499999999999939);
#8382=CYLINDRICAL_SURFACE('',#46953,1.85841829658605);
#8383=CYLINDRICAL_SURFACE('',#46956,0.499999999999935);
#8384=CYLINDRICAL_SURFACE('',#46959,1.81285717707167);
#8385=CYLINDRICAL_SURFACE('',#46962,0.499999999999944);
#8386=CYLINDRICAL_SURFACE('',#46965,1.91146602029503);
#8387=CYLINDRICAL_SURFACE('',#46968,0.500000000000167);
#8388=CYLINDRICAL_SURFACE('',#46971,1.0588834746273);
#8389=CYLINDRICAL_SURFACE('',#46974,0.499999999999944);
#8390=CYLINDRICAL_SURFACE('',#46977,1.29583333162394);
#8391=CYLINDRICAL_SURFACE('',#46980,0.500000000000054);
#8392=CYLINDRICAL_SURFACE('',#46983,1.60653900437062);
#8393=CYLINDRICAL_SURFACE('',#46986,0.499999999999944);
#8394=CYLINDRICAL_SURFACE('',#46989,1.82809807486273);
#8395=CYLINDRICAL_SURFACE('',#46992,0.499999999999944);
#8396=CYLINDRICAL_SURFACE('',#46995,1.85841829658605);
#8397=CYLINDRICAL_SURFACE('',#46998,0.499999999999944);
#8398=CYLINDRICAL_SURFACE('',#47001,1.91146602029503);
#8399=CYLINDRICAL_SURFACE('',#47004,0.500000000000058);
#8400=CYLINDRICAL_SURFACE('',#47007,1.54967110260249);
#8401=CYLINDRICAL_SURFACE('',#47011,0.499999999999939);
#8402=CYLINDRICAL_SURFACE('',#47014,1.05888347462741);
#8403=CYLINDRICAL_SURFACE('',#47017,0.499999999999939);
#8404=CYLINDRICAL_SURFACE('',#47020,1.29583333162394);
#8405=CYLINDRICAL_SURFACE('',#47023,0.499999999999939);
#8406=CYLINDRICAL_SURFACE('',#47026,1.60653900437063);
#8407=CYLINDRICAL_SURFACE('',#47029,0.500000000000058);
#8408=CYLINDRICAL_SURFACE('',#47032,1.82809807486273);
#8409=CYLINDRICAL_SURFACE('',#47035,0.500000000000058);
#8410=CYLINDRICAL_SURFACE('',#47038,1.85841829658593);
#8411=CYLINDRICAL_SURFACE('',#47041,0.499999999999939);
#8412=CYLINDRICAL_SURFACE('',#47044,1.81285717707155);
#8413=CYLINDRICAL_SURFACE('',#47047,0.499999999999939);
#8414=CYLINDRICAL_SURFACE('',#47050,1.91146602029503);
#8415=CYLINDRICAL_SURFACE('',#47053,0.499999999999939);
#8416=CYLINDRICAL_SURFACE('',#47056,1.54967110260237);
#8417=CYLINDRICAL_SURFACE('',#47059,0.499999999999939);
#8418=CYLINDRICAL_SURFACE('',#47062,1.05888347462729);
#8419=CYLINDRICAL_SURFACE('',#47065,0.500000000000054);
#8420=CYLINDRICAL_SURFACE('',#47068,1.29583333162383);
#8421=CYLINDRICAL_SURFACE('',#47071,0.500000000000054);
#8422=CYLINDRICAL_SURFACE('',#47074,1.60653900437051);
#8423=CYLINDRICAL_SURFACE('',#47077,0.499999999999935);
#8424=CYLINDRICAL_SURFACE('',#47080,1.82809807486262);
#8425=CYLINDRICAL_SURFACE('',#47083,0.500000000000063);
#8426=CYLINDRICAL_SURFACE('',#47086,1.85841829658605);
#8427=CYLINDRICAL_SURFACE('',#47089,0.500000000000054);
#8428=CYLINDRICAL_SURFACE('',#47092,1.81285717707166);
#8429=CYLINDRICAL_SURFACE('',#47095,0.499999999999935);
#8430=CYLINDRICAL_SURFACE('',#47098,1.9114660202949);
#8431=CYLINDRICAL_SURFACE('',#47101,0.499999999999935);
#8432=CYLINDRICAL_SURFACE('',#47104,1.54967110260238);
#8433=CYLINDRICAL_SURFACE('',#47107,0.499999999999935);
#8434=CYLINDRICAL_SURFACE('',#47110,1.25936103546556);
#8435=CYLINDRICAL_SURFACE('',#47114,0.499999999999935);
#8436=CYLINDRICAL_SURFACE('',#47117,1.05888347462741);
#8437=CYLINDRICAL_SURFACE('',#47120,0.500000000000058);
#8438=CYLINDRICAL_SURFACE('',#47123,1.29583333162406);
#8439=CYLINDRICAL_SURFACE('',#47126,0.499999999999939);
#8440=CYLINDRICAL_SURFACE('',#47129,1.60653900437063);
#8441=CYLINDRICAL_SURFACE('',#47132,0.500000000000058);
#8442=CYLINDRICAL_SURFACE('',#47135,1.82809807486262);
#8443=CYLINDRICAL_SURFACE('',#47138,0.499999999999939);
#8444=CYLINDRICAL_SURFACE('',#47141,1.85841829658593);
#8445=CYLINDRICAL_SURFACE('',#47144,0.499999999999939);
#8446=CYLINDRICAL_SURFACE('',#47147,1.81285717707179);
#8447=CYLINDRICAL_SURFACE('',#47150,0.499999999999939);
#8448=CYLINDRICAL_SURFACE('',#47153,1.91146602029502);
#8449=CYLINDRICAL_SURFACE('',#47156,0.499999999999939);
#8450=CYLINDRICAL_SURFACE('',#47159,1.54967110260249);
#8451=CYLINDRICAL_SURFACE('',#47162,0.500000000000058);
#8452=CYLINDRICAL_SURFACE('',#47165,1.25936103546569);
#8453=CYLINDRICAL_SURFACE('',#47169,0.499999999999935);
#8454=CYLINDRICAL_SURFACE('',#47172,1.0588834746273);
#8455=CYLINDRICAL_SURFACE('',#47175,0.500000000000054);
#8456=CYLINDRICAL_SURFACE('',#47178,1.29583333162406);
#8457=CYLINDRICAL_SURFACE('',#47181,0.500000000000177);
#8458=CYLINDRICAL_SURFACE('',#47184,1.60653900437051);
#8459=CYLINDRICAL_SURFACE('',#47187,0.499999999999939);
#8460=CYLINDRICAL_SURFACE('',#47190,1.82809807486261);
#8461=CYLINDRICAL_SURFACE('',#47193,0.499999999999944);
#8462=CYLINDRICAL_SURFACE('',#47196,1.85841829658594);
#8463=CYLINDRICAL_SURFACE('',#47199,0.499999999999939);
#8464=CYLINDRICAL_SURFACE('',#47202,1.81285717707156);
#8465=CYLINDRICAL_SURFACE('',#47205,0.499999999999944);
#8466=CYLINDRICAL_SURFACE('',#47208,1.91146602029503);
#8467=CYLINDRICAL_SURFACE('',#47211,0.500000000000054);
#8468=CYLINDRICAL_SURFACE('',#47214,1.5496711026026);
#8469=CYLINDRICAL_SURFACE('',#47217,0.500000000000058);
#8470=CYLINDRICAL_SURFACE('',#47220,1.2593610354658);
#8471=CYLINDRICAL_SURFACE('',#47223,0.500000000000063);
#8472=CYLINDRICAL_SURFACE('',#47226,1.05888347462741);
#8473=CYLINDRICAL_SURFACE('',#47229,0.499999999999939);
#8474=CYLINDRICAL_SURFACE('',#47232,1.29583333162395);
#8475=CYLINDRICAL_SURFACE('',#47235,0.500000000000054);
#8476=CYLINDRICAL_SURFACE('',#47238,1.60653900437063);
#8477=CYLINDRICAL_SURFACE('',#47241,0.500000000000167);
#8478=CYLINDRICAL_SURFACE('',#47244,1.82809807486262);
#8479=CYLINDRICAL_SURFACE('',#47247,0.499999999999944);
#8480=CYLINDRICAL_SURFACE('',#47250,1.85841829658605);
#8481=CYLINDRICAL_SURFACE('',#47253,0.499999999999944);
#8482=CYLINDRICAL_SURFACE('',#47256,1.91146602029502);
#8483=CYLINDRICAL_SURFACE('',#47259,0.499999999999944);
#8484=CYLINDRICAL_SURFACE('',#47262,1.5496711026026);
#8485=CYLINDRICAL_SURFACE('',#47265,0.500000000000054);
#8486=CYLINDRICAL_SURFACE('',#47268,1.25936103546567);
#8487=CYLINDRICAL_SURFACE('',#47271,0.499999999999939);
#8488=CYLINDRICAL_SURFACE('',#47274,1.05888347462741);
#8489=CYLINDRICAL_SURFACE('',#47277,0.500000000000054);
#8490=CYLINDRICAL_SURFACE('',#47280,1.29583333162394);
#8491=CYLINDRICAL_SURFACE('',#47283,0.499999999999939);
#8492=CYLINDRICAL_SURFACE('',#47286,1.6065390043705);
#8493=CYLINDRICAL_SURFACE('',#47289,0.499999999999939);
#8494=CYLINDRICAL_SURFACE('',#47292,1.82809807486262);
#8495=CYLINDRICAL_SURFACE('',#47295,0.500000000000054);
#8496=CYLINDRICAL_SURFACE('',#47298,1.85841829658593);
#8497=CYLINDRICAL_SURFACE('',#47301,0.499999999999939);
#8498=CYLINDRICAL_SURFACE('',#47304,1.81285717707167);
#8499=CYLINDRICAL_SURFACE('',#47307,0.500000000000058);
#8500=CYLINDRICAL_SURFACE('',#47310,1.91146602029503);
#8501=CYLINDRICAL_SURFACE('',#47313,0.500000000000054);
#8502=CYLINDRICAL_SURFACE('',#47316,1.54967110260249);
#8503=CYLINDRICAL_SURFACE('',#47319,0.500000000000058);
#8504=CYLINDRICAL_SURFACE('',#47322,1.25936103546568);
#8505=CYLINDRICAL_SURFACE('',#47325,0.499999999999939);
#8506=CYLINDRICAL_SURFACE('',#47328,1.0588834746273);
#8507=CYLINDRICAL_SURFACE('',#47331,0.500000000000054);
#8508=CYLINDRICAL_SURFACE('',#47334,1.29583333162383);
#8509=CYLINDRICAL_SURFACE('',#47337,0.499999999999935);
#8510=CYLINDRICAL_SURFACE('',#47340,1.60653900437062);
#8511=CYLINDRICAL_SURFACE('',#47343,0.500000000000058);
#8512=CYLINDRICAL_SURFACE('',#47346,1.82809807486272);
#8513=CYLINDRICAL_SURFACE('',#47349,0.500000000000058);
#8514=CYLINDRICAL_SURFACE('',#47352,1.85841829658594);
#8515=CYLINDRICAL_SURFACE('',#47355,0.499999999999826);
#8516=CYLINDRICAL_SURFACE('',#47358,1.81285717707156);
#8517=CYLINDRICAL_SURFACE('',#47361,0.499999999999944);
#8518=CYLINDRICAL_SURFACE('',#47364,1.91146602029502);
#8519=CYLINDRICAL_SURFACE('',#47367,0.499999999999935);
#8520=CYLINDRICAL_SURFACE('',#47370,1.54967110260249);
#8521=CYLINDRICAL_SURFACE('',#47373,0.500000000000054);
#8522=CYLINDRICAL_SURFACE('',#47376,1.25936103546568);
#8523=CYLINDRICAL_SURFACE('',#47379,0.500000000000054);
#8524=CYLINDRICAL_SURFACE('',#47433,0.5);
#8525=CYLINDRICAL_SURFACE('',#47439,8.99091713639503);
#8526=CYLINDRICAL_SURFACE('',#47445,0.500000000000054);
#8527=CYLINDRICAL_SURFACE('',#47447,1.02140828085145);
#8528=CYLINDRICAL_SURFACE('',#47451,8.3031389659941);
#8529=CYLINDRICAL_SURFACE('',#47456,8.3031389659941);
#8530=CYLINDRICAL_SURFACE('',#47459,8.3031389659941);
#8531=CYLINDRICAL_SURFACE('',#47476,0.999999999999995);
#8532=CYLINDRICAL_SURFACE('',#47478,0.999999999999995);
#8533=CYLINDRICAL_SURFACE('',#47483,0.999999999999995);
#8534=CYLINDRICAL_SURFACE('',#47485,0.999999999999995);
#8535=CYLINDRICAL_SURFACE('',#47491,0.500000017388205);
#8536=CYLINDRICAL_SURFACE('',#47494,0.500000017611928);
#8537=CYLINDRICAL_SURFACE('',#47496,8.3031389659941);
#8538=CYLINDRICAL_SURFACE('',#47510,0.5);
#8539=CYLINDRICAL_SURFACE('',#47514,65.);
#8540=CYLINDRICAL_SURFACE('',#47537,8.3031389659941);
#9474=FACE_OUTER_BOUND('',#12875,.T.);
#9475=FACE_OUTER_BOUND('',#12876,.T.);
#9476=FACE_OUTER_BOUND('',#12877,.T.);
#9477=FACE_OUTER_BOUND('',#12878,.T.);
#9478=FACE_OUTER_BOUND('',#12879,.T.);
#9479=FACE_OUTER_BOUND('',#12880,.T.);
#9480=FACE_OUTER_BOUND('',#12881,.T.);
#9481=FACE_OUTER_BOUND('',#12882,.T.);
#9482=FACE_OUTER_BOUND('',#12883,.T.);
#9483=FACE_OUTER_BOUND('',#12884,.T.);
#9484=FACE_OUTER_BOUND('',#12885,.T.);
#9485=FACE_OUTER_BOUND('',#12886,.T.);
#9486=FACE_OUTER_BOUND('',#12887,.T.);
#9487=FACE_OUTER_BOUND('',#12888,.T.);
#9488=FACE_OUTER_BOUND('',#12889,.T.);
#9489=FACE_OUTER_BOUND('',#12890,.T.);
#9490=FACE_OUTER_BOUND('',#12891,.T.);
#9491=FACE_OUTER_BOUND('',#12892,.T.);
#9492=FACE_OUTER_BOUND('',#12893,.T.);
#9493=FACE_OUTER_BOUND('',#12894,.T.);
#9494=FACE_OUTER_BOUND('',#12895,.T.);
#9495=FACE_OUTER_BOUND('',#12896,.T.);
#9496=FACE_OUTER_BOUND('',#12897,.T.);
#9497=FACE_OUTER_BOUND('',#12898,.T.);
#9498=FACE_OUTER_BOUND('',#12899,.T.);
#9499=FACE_OUTER_BOUND('',#12900,.T.);
#9500=FACE_OUTER_BOUND('',#12901,.T.);
#9501=FACE_OUTER_BOUND('',#12902,.T.);
#9502=FACE_OUTER_BOUND('',#12903,.T.);
#9503=FACE_OUTER_BOUND('',#12904,.T.);
#9504=FACE_OUTER_BOUND('',#12905,.T.);
#9505=FACE_OUTER_BOUND('',#12906,.T.);
#9506=FACE_OUTER_BOUND('',#12907,.T.);
#9507=FACE_OUTER_BOUND('',#12908,.T.);
#9508=FACE_OUTER_BOUND('',#12909,.T.);
#9509=FACE_OUTER_BOUND('',#12910,.T.);
#9510=FACE_OUTER_BOUND('',#12911,.T.);
#9511=FACE_OUTER_BOUND('',#12912,.T.);
#9512=FACE_OUTER_BOUND('',#12913,.T.);
#9513=FACE_OUTER_BOUND('',#12914,.T.);
#9514=FACE_OUTER_BOUND('',#12915,.T.);
#9515=FACE_OUTER_BOUND('',#12916,.T.);
#9516=FACE_OUTER_BOUND('',#12917,.T.);
#9517=FACE_OUTER_BOUND('',#12918,.T.);
#9518=FACE_OUTER_BOUND('',#12919,.T.);
#9519=FACE_OUTER_BOUND('',#12920,.T.);
#9520=FACE_OUTER_BOUND('',#12921,.T.);
#9521=FACE_OUTER_BOUND('',#12922,.T.);
#9522=FACE_OUTER_BOUND('',#12923,.T.);
#9523=FACE_OUTER_BOUND('',#12924,.T.);
#9524=FACE_OUTER_BOUND('',#12925,.T.);
#9525=FACE_OUTER_BOUND('',#12926,.T.);
#9526=FACE_OUTER_BOUND('',#12927,.T.);
#9527=FACE_OUTER_BOUND('',#12928,.T.);
#9528=FACE_OUTER_BOUND('',#12929,.T.);
#9529=FACE_OUTER_BOUND('',#12930,.T.);
#9530=FACE_OUTER_BOUND('',#12931,.T.);
#9531=FACE_OUTER_BOUND('',#12932,.T.);
#9532=FACE_OUTER_BOUND('',#12933,.T.);
#9533=FACE_OUTER_BOUND('',#12934,.T.);
#9534=FACE_OUTER_BOUND('',#12935,.T.);
#9535=FACE_OUTER_BOUND('',#12936,.T.);
#9536=FACE_OUTER_BOUND('',#12937,.T.);
#9537=FACE_OUTER_BOUND('',#12938,.T.);
#9538=FACE_OUTER_BOUND('',#12939,.T.);
#9539=FACE_OUTER_BOUND('',#12940,.T.);
#9540=FACE_OUTER_BOUND('',#12941,.T.);
#9541=FACE_OUTER_BOUND('',#12942,.T.);
#9542=FACE_OUTER_BOUND('',#12943,.T.);
#9543=FACE_OUTER_BOUND('',#12944,.T.);
#9544=FACE_OUTER_BOUND('',#12945,.T.);
#9545=FACE_OUTER_BOUND('',#12946,.T.);
#9546=FACE_OUTER_BOUND('',#12947,.T.);
#9547=FACE_OUTER_BOUND('',#12948,.T.);
#9548=FACE_OUTER_BOUND('',#12949,.T.);
#9549=FACE_OUTER_BOUND('',#12950,.T.);
#9550=FACE_OUTER_BOUND('',#12951,.T.);
#9551=FACE_OUTER_BOUND('',#12952,.T.);
#9552=FACE_OUTER_BOUND('',#12953,.T.);
#9553=FACE_OUTER_BOUND('',#12954,.T.);
#9554=FACE_OUTER_BOUND('',#12955,.T.);
#9555=FACE_OUTER_BOUND('',#12956,.T.);
#9556=FACE_OUTER_BOUND('',#12957,.T.);
#9557=FACE_OUTER_BOUND('',#12958,.T.);
#9558=FACE_OUTER_BOUND('',#12959,.T.);
#9559=FACE_OUTER_BOUND('',#12960,.T.);
#9560=FACE_OUTER_BOUND('',#12961,.T.);
#9561=FACE_OUTER_BOUND('',#12962,.T.);
#9562=FACE_OUTER_BOUND('',#12963,.T.);
#9563=FACE_OUTER_BOUND('',#12964,.T.);
#9564=FACE_OUTER_BOUND('',#12965,.T.);
#9565=FACE_OUTER_BOUND('',#12966,.T.);
#9566=FACE_OUTER_BOUND('',#12967,.T.);
#9567=FACE_OUTER_BOUND('',#12968,.T.);
#9568=FACE_OUTER_BOUND('',#12969,.T.);
#9569=FACE_OUTER_BOUND('',#12970,.T.);
#9570=FACE_OUTER_BOUND('',#12971,.T.);
#9571=FACE_OUTER_BOUND('',#12972,.T.);
#9572=FACE_OUTER_BOUND('',#12973,.T.);
#9573=FACE_OUTER_BOUND('',#12974,.T.);
#9574=FACE_OUTER_BOUND('',#12975,.T.);
#9575=FACE_OUTER_BOUND('',#12976,.T.);
#9576=FACE_OUTER_BOUND('',#12977,.T.);
#9577=FACE_OUTER_BOUND('',#12978,.T.);
#9578=FACE_OUTER_BOUND('',#12979,.T.);
#9579=FACE_OUTER_BOUND('',#12980,.T.);
#9580=FACE_OUTER_BOUND('',#12981,.T.);
#9581=FACE_OUTER_BOUND('',#12982,.T.);
#9582=FACE_OUTER_BOUND('',#12983,.T.);
#9583=FACE_OUTER_BOUND('',#12984,.T.);
#9584=FACE_OUTER_BOUND('',#12985,.T.);
#9585=FACE_OUTER_BOUND('',#12986,.T.);
#9586=FACE_OUTER_BOUND('',#12987,.T.);
#9587=FACE_OUTER_BOUND('',#12988,.T.);
#9588=FACE_OUTER_BOUND('',#12989,.T.);
#9589=FACE_OUTER_BOUND('',#12990,.T.);
#9590=FACE_OUTER_BOUND('',#12991,.T.);
#9591=FACE_OUTER_BOUND('',#12992,.T.);
#9592=FACE_OUTER_BOUND('',#12993,.T.);
#9593=FACE_OUTER_BOUND('',#12994,.T.);
#9594=FACE_OUTER_BOUND('',#12995,.T.);
#9595=FACE_OUTER_BOUND('',#12996,.T.);
#9596=FACE_OUTER_BOUND('',#12997,.T.);
#9597=FACE_OUTER_BOUND('',#12998,.T.);
#9598=FACE_OUTER_BOUND('',#12999,.T.);
#9599=FACE_OUTER_BOUND('',#13000,.T.);
#9600=FACE_OUTER_BOUND('',#13001,.T.);
#9601=FACE_OUTER_BOUND('',#13002,.T.);
#9602=FACE_OUTER_BOUND('',#13003,.T.);
#9603=FACE_OUTER_BOUND('',#13004,.T.);
#9604=FACE_OUTER_BOUND('',#13005,.T.);
#9605=FACE_OUTER_BOUND('',#13006,.T.);
#9606=FACE_OUTER_BOUND('',#13007,.T.);
#9607=FACE_OUTER_BOUND('',#13008,.T.);
#9608=FACE_OUTER_BOUND('',#13009,.T.);
#9609=FACE_OUTER_BOUND('',#13010,.T.);
#9610=FACE_OUTER_BOUND('',#13011,.T.);
#9611=FACE_OUTER_BOUND('',#13012,.T.);
#9612=FACE_OUTER_BOUND('',#13013,.T.);
#9613=FACE_OUTER_BOUND('',#13014,.T.);
#9614=FACE_OUTER_BOUND('',#13015,.T.);
#9615=FACE_OUTER_BOUND('',#13016,.T.);
#9616=FACE_OUTER_BOUND('',#13017,.T.);
#9617=FACE_OUTER_BOUND('',#13018,.T.);
#9618=FACE_OUTER_BOUND('',#13019,.T.);
#9619=FACE_OUTER_BOUND('',#13020,.T.);
#9620=FACE_OUTER_BOUND('',#13021,.T.);
#9621=FACE_OUTER_BOUND('',#13022,.T.);
#9622=FACE_OUTER_BOUND('',#13023,.T.);
#9623=FACE_OUTER_BOUND('',#13024,.T.);
#9624=FACE_OUTER_BOUND('',#13025,.T.);
#9625=FACE_OUTER_BOUND('',#13026,.T.);
#9626=FACE_OUTER_BOUND('',#13027,.T.);
#9627=FACE_OUTER_BOUND('',#13028,.T.);
#9628=FACE_OUTER_BOUND('',#13029,.T.);
#9629=FACE_OUTER_BOUND('',#13030,.T.);
#9630=FACE_OUTER_BOUND('',#13031,.T.);
#9631=FACE_OUTER_BOUND('',#13032,.T.);
#9632=FACE_OUTER_BOUND('',#13033,.T.);
#9633=FACE_OUTER_BOUND('',#13034,.T.);
#9634=FACE_OUTER_BOUND('',#13035,.T.);
#9635=FACE_OUTER_BOUND('',#13036,.T.);
#9636=FACE_OUTER_BOUND('',#13037,.T.);
#9637=FACE_OUTER_BOUND('',#13038,.T.);
#9638=FACE_OUTER_BOUND('',#13039,.T.);
#9639=FACE_OUTER_BOUND('',#13040,.T.);
#9640=FACE_OUTER_BOUND('',#13041,.T.);
#9641=FACE_OUTER_BOUND('',#13042,.T.);
#9642=FACE_OUTER_BOUND('',#13043,.T.);
#9643=FACE_OUTER_BOUND('',#13044,.T.);
#9644=FACE_OUTER_BOUND('',#13045,.T.);
#9645=FACE_OUTER_BOUND('',#13046,.T.);
#9646=FACE_OUTER_BOUND('',#13047,.T.);
#9647=FACE_OUTER_BOUND('',#13048,.T.);
#9648=FACE_OUTER_BOUND('',#13049,.T.);
#9649=FACE_OUTER_BOUND('',#13050,.T.);
#9650=FACE_OUTER_BOUND('',#13051,.T.);
#9651=FACE_OUTER_BOUND('',#13052,.T.);
#9652=FACE_OUTER_BOUND('',#13053,.T.);
#9653=FACE_OUTER_BOUND('',#13054,.T.);
#9654=FACE_OUTER_BOUND('',#13055,.T.);
#9655=FACE_OUTER_BOUND('',#13056,.T.);
#9656=FACE_OUTER_BOUND('',#13057,.T.);
#9657=FACE_OUTER_BOUND('',#13058,.T.);
#9658=FACE_OUTER_BOUND('',#13059,.T.);
#9659=FACE_OUTER_BOUND('',#13060,.T.);
#9660=FACE_OUTER_BOUND('',#13061,.T.);
#9661=FACE_OUTER_BOUND('',#13062,.T.);
#9662=FACE_OUTER_BOUND('',#13063,.T.);
#9663=FACE_OUTER_BOUND('',#13064,.T.);
#9664=FACE_OUTER_BOUND('',#13065,.T.);
#9665=FACE_OUTER_BOUND('',#13066,.T.);
#9666=FACE_OUTER_BOUND('',#13067,.T.);
#9667=FACE_OUTER_BOUND('',#13068,.T.);
#9668=FACE_OUTER_BOUND('',#13069,.T.);
#9669=FACE_OUTER_BOUND('',#13070,.T.);
#9670=FACE_OUTER_BOUND('',#13071,.T.);
#9671=FACE_OUTER_BOUND('',#13072,.T.);
#9672=FACE_OUTER_BOUND('',#13073,.T.);
#9673=FACE_OUTER_BOUND('',#13074,.T.);
#9674=FACE_OUTER_BOUND('',#13075,.T.);
#9675=FACE_OUTER_BOUND('',#13076,.T.);
#9676=FACE_OUTER_BOUND('',#13077,.T.);
#9677=FACE_OUTER_BOUND('',#13078,.T.);
#9678=FACE_OUTER_BOUND('',#13079,.T.);
#9679=FACE_OUTER_BOUND('',#13080,.T.);
#9680=FACE_OUTER_BOUND('',#13081,.T.);
#9681=FACE_OUTER_BOUND('',#13082,.T.);
#9682=FACE_OUTER_BOUND('',#13083,.T.);
#9683=FACE_OUTER_BOUND('',#13084,.T.);
#9684=FACE_OUTER_BOUND('',#13085,.T.);
#9685=FACE_OUTER_BOUND('',#13086,.T.);
#9686=FACE_OUTER_BOUND('',#13087,.T.);
#9687=FACE_OUTER_BOUND('',#13088,.T.);
#9688=FACE_OUTER_BOUND('',#13089,.T.);
#9689=FACE_OUTER_BOUND('',#13090,.T.);
#9690=FACE_OUTER_BOUND('',#13091,.T.);
#9691=FACE_OUTER_BOUND('',#13092,.T.);
#9692=FACE_OUTER_BOUND('',#13093,.T.);
#9693=FACE_OUTER_BOUND('',#13094,.T.);
#9694=FACE_OUTER_BOUND('',#13095,.T.);
#9695=FACE_OUTER_BOUND('',#13096,.T.);
#9696=FACE_OUTER_BOUND('',#13097,.T.);
#9697=FACE_OUTER_BOUND('',#13098,.T.);
#9698=FACE_OUTER_BOUND('',#13099,.T.);
#9699=FACE_OUTER_BOUND('',#13100,.T.);
#9700=FACE_OUTER_BOUND('',#13101,.T.);
#9701=FACE_OUTER_BOUND('',#13102,.T.);
#9702=FACE_OUTER_BOUND('',#13103,.T.);
#9703=FACE_OUTER_BOUND('',#13104,.T.);
#9704=FACE_OUTER_BOUND('',#13105,.T.);
#9705=FACE_OUTER_BOUND('',#13106,.T.);
#9706=FACE_OUTER_BOUND('',#13107,.T.);
#9707=FACE_OUTER_BOUND('',#13108,.T.);
#9708=FACE_OUTER_BOUND('',#13109,.T.);
#9709=FACE_OUTER_BOUND('',#13110,.T.);
#9710=FACE_OUTER_BOUND('',#13111,.T.);
#9711=FACE_OUTER_BOUND('',#13112,.T.);
#9712=FACE_OUTER_BOUND('',#13113,.T.);
#9713=FACE_OUTER_BOUND('',#13114,.T.);
#9714=FACE_OUTER_BOUND('',#13115,.T.);
#9715=FACE_OUTER_BOUND('',#13116,.T.);
#9716=FACE_OUTER_BOUND('',#13117,.T.);
#9717=FACE_OUTER_BOUND('',#13118,.T.);
#9718=FACE_OUTER_BOUND('',#13119,.T.);
#9719=FACE_OUTER_BOUND('',#13120,.T.);
#9720=FACE_OUTER_BOUND('',#13121,.T.);
#9721=FACE_OUTER_BOUND('',#13122,.T.);
#9722=FACE_OUTER_BOUND('',#13123,.T.);
#9723=FACE_OUTER_BOUND('',#13124,.T.);
#9724=FACE_OUTER_BOUND('',#13125,.T.);
#9725=FACE_OUTER_BOUND('',#13126,.T.);
#9726=FACE_OUTER_BOUND('',#13127,.T.);
#9727=FACE_OUTER_BOUND('',#13128,.T.);
#9728=FACE_OUTER_BOUND('',#13129,.T.);
#9729=FACE_OUTER_BOUND('',#13130,.T.);
#9730=FACE_OUTER_BOUND('',#13131,.T.);
#9731=FACE_OUTER_BOUND('',#13132,.T.);
#9732=FACE_OUTER_BOUND('',#13133,.T.);
#9733=FACE_OUTER_BOUND('',#13134,.T.);
#9734=FACE_OUTER_BOUND('',#13135,.T.);
#9735=FACE_OUTER_BOUND('',#13136,.T.);
#9736=FACE_OUTER_BOUND('',#13137,.T.);
#9737=FACE_OUTER_BOUND('',#13138,.T.);
#9738=FACE_OUTER_BOUND('',#13139,.T.);
#9739=FACE_OUTER_BOUND('',#13140,.T.);
#9740=FACE_OUTER_BOUND('',#13141,.T.);
#9741=FACE_OUTER_BOUND('',#13142,.T.);
#9742=FACE_OUTER_BOUND('',#13143,.T.);
#9743=FACE_OUTER_BOUND('',#13144,.T.);
#9744=FACE_OUTER_BOUND('',#13145,.T.);
#9745=FACE_OUTER_BOUND('',#13146,.T.);
#9746=FACE_OUTER_BOUND('',#13147,.T.);
#9747=FACE_OUTER_BOUND('',#13148,.T.);
#9748=FACE_OUTER_BOUND('',#13149,.T.);
#9749=FACE_OUTER_BOUND('',#13150,.T.);
#9750=FACE_OUTER_BOUND('',#13151,.T.);
#9751=FACE_OUTER_BOUND('',#13152,.T.);
#9752=FACE_OUTER_BOUND('',#13153,.T.);
#9753=FACE_OUTER_BOUND('',#13154,.T.);
#9754=FACE_OUTER_BOUND('',#13155,.T.);
#9755=FACE_OUTER_BOUND('',#13156,.T.);
#9756=FACE_OUTER_BOUND('',#13157,.T.);
#9757=FACE_OUTER_BOUND('',#13158,.T.);
#9758=FACE_OUTER_BOUND('',#13159,.T.);
#9759=FACE_OUTER_BOUND('',#13160,.T.);
#9760=FACE_OUTER_BOUND('',#13161,.T.);
#9761=FACE_OUTER_BOUND('',#13162,.T.);
#9762=FACE_OUTER_BOUND('',#13163,.T.);
#9763=FACE_OUTER_BOUND('',#13164,.T.);
#9764=FACE_OUTER_BOUND('',#13165,.T.);
#9765=FACE_OUTER_BOUND('',#13166,.T.);
#9766=FACE_OUTER_BOUND('',#13167,.T.);
#9767=FACE_OUTER_BOUND('',#13168,.T.);
#9768=FACE_OUTER_BOUND('',#13169,.T.);
#9769=FACE_OUTER_BOUND('',#13170,.T.);
#9770=FACE_OUTER_BOUND('',#13171,.T.);
#9771=FACE_OUTER_BOUND('',#13172,.T.);
#9772=FACE_OUTER_BOUND('',#13173,.T.);
#9773=FACE_OUTER_BOUND('',#13174,.T.);
#9774=FACE_OUTER_BOUND('',#13175,.T.);
#9775=FACE_OUTER_BOUND('',#13176,.T.);
#9776=FACE_OUTER_BOUND('',#13177,.T.);
#9777=FACE_OUTER_BOUND('',#13178,.T.);
#9778=FACE_OUTER_BOUND('',#13179,.T.);
#9779=FACE_OUTER_BOUND('',#13180,.T.);
#9780=FACE_OUTER_BOUND('',#13181,.T.);
#9781=FACE_OUTER_BOUND('',#13182,.T.);
#9782=FACE_OUTER_BOUND('',#13183,.T.);
#9783=FACE_OUTER_BOUND('',#13184,.T.);
#9784=FACE_OUTER_BOUND('',#13185,.T.);
#9785=FACE_OUTER_BOUND('',#13186,.T.);
#9786=FACE_OUTER_BOUND('',#13187,.T.);
#9787=FACE_OUTER_BOUND('',#13188,.T.);
#9788=FACE_OUTER_BOUND('',#13189,.T.);
#9789=FACE_OUTER_BOUND('',#13190,.T.);
#9790=FACE_OUTER_BOUND('',#13191,.T.);
#9791=FACE_OUTER_BOUND('',#13192,.T.);
#9792=FACE_OUTER_BOUND('',#13193,.T.);
#9793=FACE_OUTER_BOUND('',#13194,.T.);
#9794=FACE_OUTER_BOUND('',#13195,.T.);
#9795=FACE_OUTER_BOUND('',#13196,.T.);
#9796=FACE_OUTER_BOUND('',#13197,.T.);
#9797=FACE_OUTER_BOUND('',#13198,.T.);
#9798=FACE_OUTER_BOUND('',#13199,.T.);
#9799=FACE_OUTER_BOUND('',#13200,.T.);
#9800=FACE_OUTER_BOUND('',#13201,.T.);
#9801=FACE_OUTER_BOUND('',#13202,.T.);
#9802=FACE_OUTER_BOUND('',#13203,.T.);
#9803=FACE_OUTER_BOUND('',#13204,.T.);
#9804=FACE_OUTER_BOUND('',#13205,.T.);
#9805=FACE_OUTER_BOUND('',#13206,.T.);
#9806=FACE_OUTER_BOUND('',#13207,.T.);
#9807=FACE_OUTER_BOUND('',#13208,.T.);
#9808=FACE_OUTER_BOUND('',#13209,.T.);
#9809=FACE_OUTER_BOUND('',#13210,.T.);
#9810=FACE_OUTER_BOUND('',#13211,.T.);
#9811=FACE_OUTER_BOUND('',#13212,.T.);
#9812=FACE_OUTER_BOUND('',#13213,.T.);
#9813=FACE_OUTER_BOUND('',#13214,.T.);
#9814=FACE_OUTER_BOUND('',#13215,.T.);
#9815=FACE_OUTER_BOUND('',#13216,.T.);
#9816=FACE_OUTER_BOUND('',#13217,.T.);
#9817=FACE_OUTER_BOUND('',#13218,.T.);
#9818=FACE_OUTER_BOUND('',#13219,.T.);
#9819=FACE_OUTER_BOUND('',#13220,.T.);
#9820=FACE_OUTER_BOUND('',#13221,.T.);
#9821=FACE_OUTER_BOUND('',#13222,.T.);
#9822=FACE_OUTER_BOUND('',#13223,.T.);
#9823=FACE_OUTER_BOUND('',#13224,.T.);
#9824=FACE_OUTER_BOUND('',#13225,.T.);
#9825=FACE_OUTER_BOUND('',#13226,.T.);
#9826=FACE_OUTER_BOUND('',#13227,.T.);
#9827=FACE_OUTER_BOUND('',#13228,.T.);
#9828=FACE_OUTER_BOUND('',#13229,.T.);
#9829=FACE_OUTER_BOUND('',#13230,.T.);
#9830=FACE_OUTER_BOUND('',#13231,.T.);
#9831=FACE_OUTER_BOUND('',#13232,.T.);
#9832=FACE_OUTER_BOUND('',#13233,.T.);
#9833=FACE_OUTER_BOUND('',#13234,.T.);
#9834=FACE_OUTER_BOUND('',#13235,.T.);
#9835=FACE_OUTER_BOUND('',#13236,.T.);
#9836=FACE_OUTER_BOUND('',#13237,.T.);
#9837=FACE_OUTER_BOUND('',#13238,.T.);
#9838=FACE_OUTER_BOUND('',#13239,.T.);
#9839=FACE_OUTER_BOUND('',#13240,.T.);
#9840=FACE_OUTER_BOUND('',#13241,.T.);
#9841=FACE_OUTER_BOUND('',#13242,.T.);
#9842=FACE_OUTER_BOUND('',#13243,.T.);
#9843=FACE_OUTER_BOUND('',#13244,.T.);
#9844=FACE_OUTER_BOUND('',#13245,.T.);
#9845=FACE_OUTER_BOUND('',#13246,.T.);
#9846=FACE_OUTER_BOUND('',#13247,.T.);
#9847=FACE_OUTER_BOUND('',#13248,.T.);
#9848=FACE_OUTER_BOUND('',#13249,.T.);
#9849=FACE_OUTER_BOUND('',#13250,.T.);
#9850=FACE_OUTER_BOUND('',#13251,.T.);
#9851=FACE_OUTER_BOUND('',#13252,.T.);
#9852=FACE_OUTER_BOUND('',#13253,.T.);
#9853=FACE_OUTER_BOUND('',#13254,.T.);
#9854=FACE_OUTER_BOUND('',#13255,.T.);
#9855=FACE_OUTER_BOUND('',#13256,.T.);
#9856=FACE_OUTER_BOUND('',#13257,.T.);
#9857=FACE_OUTER_BOUND('',#13258,.T.);
#9858=FACE_OUTER_BOUND('',#13259,.T.);
#9859=FACE_OUTER_BOUND('',#13260,.T.);
#9860=FACE_OUTER_BOUND('',#13261,.T.);
#9861=FACE_OUTER_BOUND('',#13262,.T.);
#9862=FACE_OUTER_BOUND('',#13263,.T.);
#9863=FACE_OUTER_BOUND('',#13264,.T.);
#9864=FACE_OUTER_BOUND('',#13265,.T.);
#9865=FACE_OUTER_BOUND('',#13266,.T.);
#9866=FACE_OUTER_BOUND('',#13267,.T.);
#9867=FACE_OUTER_BOUND('',#13268,.T.);
#9868=FACE_OUTER_BOUND('',#13269,.T.);
#9869=FACE_OUTER_BOUND('',#13270,.T.);
#9870=FACE_OUTER_BOUND('',#13271,.T.);
#9871=FACE_OUTER_BOUND('',#13272,.T.);
#9872=FACE_OUTER_BOUND('',#13273,.T.);
#9873=FACE_OUTER_BOUND('',#13274,.T.);
#9874=FACE_OUTER_BOUND('',#13275,.T.);
#9875=FACE_OUTER_BOUND('',#13276,.T.);
#9876=FACE_OUTER_BOUND('',#13277,.T.);
#9877=FACE_OUTER_BOUND('',#13278,.T.);
#9878=FACE_OUTER_BOUND('',#13279,.T.);
#9879=FACE_OUTER_BOUND('',#13280,.T.);
#9880=FACE_OUTER_BOUND('',#13281,.T.);
#9881=FACE_OUTER_BOUND('',#13282,.T.);
#9882=FACE_OUTER_BOUND('',#13283,.T.);
#9883=FACE_OUTER_BOUND('',#13284,.T.);
#9884=FACE_OUTER_BOUND('',#13285,.T.);
#9885=FACE_OUTER_BOUND('',#13286,.T.);
#9886=FACE_OUTER_BOUND('',#13287,.T.);
#9887=FACE_OUTER_BOUND('',#13288,.T.);
#9888=FACE_OUTER_BOUND('',#13289,.T.);
#9889=FACE_OUTER_BOUND('',#13290,.T.);
#9890=FACE_OUTER_BOUND('',#13291,.T.);
#9891=FACE_OUTER_BOUND('',#13292,.T.);
#9892=FACE_OUTER_BOUND('',#13293,.T.);
#9893=FACE_OUTER_BOUND('',#13294,.T.);
#9894=FACE_OUTER_BOUND('',#13295,.T.);
#9895=FACE_OUTER_BOUND('',#13296,.T.);
#9896=FACE_OUTER_BOUND('',#13297,.T.);
#9897=FACE_OUTER_BOUND('',#13298,.T.);
#9898=FACE_OUTER_BOUND('',#13299,.T.);
#9899=FACE_OUTER_BOUND('',#13300,.T.);
#9900=FACE_OUTER_BOUND('',#13301,.T.);
#9901=FACE_OUTER_BOUND('',#13302,.T.);
#9902=FACE_OUTER_BOUND('',#13303,.T.);
#9903=FACE_OUTER_BOUND('',#13304,.T.);
#9904=FACE_OUTER_BOUND('',#13305,.T.);
#9905=FACE_OUTER_BOUND('',#13306,.T.);
#9906=FACE_OUTER_BOUND('',#13307,.T.);
#9907=FACE_OUTER_BOUND('',#13308,.T.);
#9908=FACE_OUTER_BOUND('',#13309,.T.);
#9909=FACE_OUTER_BOUND('',#13310,.T.);
#9910=FACE_OUTER_BOUND('',#13311,.T.);
#9911=FACE_OUTER_BOUND('',#13312,.T.);
#9912=FACE_OUTER_BOUND('',#13313,.T.);
#9913=FACE_OUTER_BOUND('',#13314,.T.);
#9914=FACE_OUTER_BOUND('',#13315,.T.);
#9915=FACE_OUTER_BOUND('',#13316,.T.);
#9916=FACE_OUTER_BOUND('',#13317,.T.);
#9917=FACE_OUTER_BOUND('',#13318,.T.);
#9918=FACE_OUTER_BOUND('',#13319,.T.);
#9919=FACE_OUTER_BOUND('',#13320,.T.);
#9920=FACE_OUTER_BOUND('',#13321,.T.);
#9921=FACE_OUTER_BOUND('',#13322,.T.);
#9922=FACE_OUTER_BOUND('',#13323,.T.);
#9923=FACE_OUTER_BOUND('',#13324,.T.);
#9924=FACE_OUTER_BOUND('',#13325,.T.);
#9925=FACE_OUTER_BOUND('',#13326,.T.);
#9926=FACE_OUTER_BOUND('',#13327,.T.);
#9927=FACE_OUTER_BOUND('',#13328,.T.);
#9928=FACE_OUTER_BOUND('',#13329,.T.);
#9929=FACE_OUTER_BOUND('',#13330,.T.);
#9930=FACE_OUTER_BOUND('',#13331,.T.);
#9931=FACE_OUTER_BOUND('',#13332,.T.);
#9932=FACE_OUTER_BOUND('',#13333,.T.);
#9933=FACE_OUTER_BOUND('',#13334,.T.);
#9934=FACE_OUTER_BOUND('',#13335,.T.);
#9935=FACE_OUTER_BOUND('',#13336,.T.);
#9936=FACE_OUTER_BOUND('',#13337,.T.);
#9937=FACE_OUTER_BOUND('',#13338,.T.);
#9938=FACE_OUTER_BOUND('',#13339,.T.);
#9939=FACE_OUTER_BOUND('',#13340,.T.);
#9940=FACE_OUTER_BOUND('',#13341,.T.);
#9941=FACE_OUTER_BOUND('',#13342,.T.);
#9942=FACE_OUTER_BOUND('',#13343,.T.);
#9943=FACE_OUTER_BOUND('',#13344,.T.);
#9944=FACE_OUTER_BOUND('',#13345,.T.);
#9945=FACE_OUTER_BOUND('',#13346,.T.);
#9946=FACE_OUTER_BOUND('',#13347,.T.);
#9947=FACE_OUTER_BOUND('',#13348,.T.);
#9948=FACE_OUTER_BOUND('',#13349,.T.);
#9949=FACE_OUTER_BOUND('',#13350,.T.);
#9950=FACE_OUTER_BOUND('',#13351,.T.);
#9951=FACE_OUTER_BOUND('',#13352,.T.);
#9952=FACE_OUTER_BOUND('',#13353,.T.);
#9953=FACE_OUTER_BOUND('',#13354,.T.);
#9954=FACE_OUTER_BOUND('',#13355,.T.);
#9955=FACE_OUTER_BOUND('',#13356,.T.);
#9956=FACE_OUTER_BOUND('',#13357,.T.);
#9957=FACE_OUTER_BOUND('',#13358,.T.);
#9958=FACE_OUTER_BOUND('',#13359,.T.);
#9959=FACE_OUTER_BOUND('',#13360,.T.);
#9960=FACE_OUTER_BOUND('',#13361,.T.);
#9961=FACE_OUTER_BOUND('',#13362,.T.);
#9962=FACE_OUTER_BOUND('',#13363,.T.);
#9963=FACE_OUTER_BOUND('',#13364,.T.);
#9964=FACE_OUTER_BOUND('',#13365,.T.);
#9965=FACE_OUTER_BOUND('',#13366,.T.);
#9966=FACE_OUTER_BOUND('',#13367,.T.);
#9967=FACE_OUTER_BOUND('',#13368,.T.);
#9968=FACE_OUTER_BOUND('',#13369,.T.);
#9969=FACE_OUTER_BOUND('',#13370,.T.);
#9970=FACE_OUTER_BOUND('',#13371,.T.);
#9971=FACE_OUTER_BOUND('',#13372,.T.);
#9972=FACE_OUTER_BOUND('',#13373,.T.);
#9973=FACE_OUTER_BOUND('',#13374,.T.);
#9974=FACE_OUTER_BOUND('',#13375,.T.);
#9975=FACE_OUTER_BOUND('',#13376,.T.);
#9976=FACE_OUTER_BOUND('',#13377,.T.);
#9977=FACE_OUTER_BOUND('',#13378,.T.);
#9978=FACE_OUTER_BOUND('',#13379,.T.);
#9979=FACE_OUTER_BOUND('',#13380,.T.);
#9980=FACE_OUTER_BOUND('',#13381,.T.);
#9981=FACE_OUTER_BOUND('',#13382,.T.);
#9982=FACE_OUTER_BOUND('',#13383,.T.);
#9983=FACE_OUTER_BOUND('',#13384,.T.);
#9984=FACE_OUTER_BOUND('',#13385,.T.);
#9985=FACE_OUTER_BOUND('',#13386,.T.);
#9986=FACE_OUTER_BOUND('',#13387,.T.);
#9987=FACE_OUTER_BOUND('',#13388,.T.);
#9988=FACE_OUTER_BOUND('',#13389,.T.);
#9989=FACE_OUTER_BOUND('',#13390,.T.);
#9990=FACE_OUTER_BOUND('',#13391,.T.);
#9991=FACE_OUTER_BOUND('',#13392,.T.);
#9992=FACE_OUTER_BOUND('',#13393,.T.);
#9993=FACE_OUTER_BOUND('',#13394,.T.);
#9994=FACE_OUTER_BOUND('',#13395,.T.);
#9995=FACE_OUTER_BOUND('',#13396,.T.);
#9996=FACE_OUTER_BOUND('',#13397,.T.);
#9997=FACE_OUTER_BOUND('',#13398,.T.);
#9998=FACE_OUTER_BOUND('',#13399,.T.);
#9999=FACE_OUTER_BOUND('',#13400,.T.);
#10000=FACE_OUTER_BOUND('',#13401,.T.);
#10001=FACE_OUTER_BOUND('',#13402,.T.);
#10002=FACE_OUTER_BOUND('',#13403,.T.);
#10003=FACE_OUTER_BOUND('',#13404,.T.);
#10004=FACE_OUTER_BOUND('',#13405,.T.);
#10005=FACE_OUTER_BOUND('',#13406,.T.);
#10006=FACE_OUTER_BOUND('',#13407,.T.);
#10007=FACE_OUTER_BOUND('',#13408,.T.);
#10008=FACE_OUTER_BOUND('',#13409,.T.);
#10009=FACE_OUTER_BOUND('',#13410,.T.);
#10010=FACE_OUTER_BOUND('',#13411,.T.);
#10011=FACE_OUTER_BOUND('',#13412,.T.);
#10012=FACE_OUTER_BOUND('',#13413,.T.);
#10013=FACE_OUTER_BOUND('',#13414,.T.);
#10014=FACE_OUTER_BOUND('',#13415,.T.);
#10015=FACE_OUTER_BOUND('',#13416,.T.);
#10016=FACE_OUTER_BOUND('',#13417,.T.);
#10017=FACE_OUTER_BOUND('',#13418,.T.);
#10018=FACE_OUTER_BOUND('',#13419,.T.);
#10019=FACE_OUTER_BOUND('',#13420,.T.);
#10020=FACE_OUTER_BOUND('',#13421,.T.);
#10021=FACE_OUTER_BOUND('',#13422,.T.);
#10022=FACE_OUTER_BOUND('',#13423,.T.);
#10023=FACE_OUTER_BOUND('',#13424,.T.);
#10024=FACE_OUTER_BOUND('',#13425,.T.);
#10025=FACE_OUTER_BOUND('',#13426,.T.);
#10026=FACE_OUTER_BOUND('',#13427,.T.);
#10027=FACE_OUTER_BOUND('',#13428,.T.);
#10028=FACE_OUTER_BOUND('',#13429,.T.);
#10029=FACE_OUTER_BOUND('',#13430,.T.);
#10030=FACE_OUTER_BOUND('',#13431,.T.);
#10031=FACE_OUTER_BOUND('',#13432,.T.);
#10032=FACE_OUTER_BOUND('',#13433,.T.);
#10033=FACE_OUTER_BOUND('',#13434,.T.);
#10034=FACE_OUTER_BOUND('',#13435,.T.);
#10035=FACE_OUTER_BOUND('',#13436,.T.);
#10036=FACE_OUTER_BOUND('',#13437,.T.);
#10037=FACE_OUTER_BOUND('',#13438,.T.);
#10038=FACE_OUTER_BOUND('',#13439,.T.);
#10039=FACE_OUTER_BOUND('',#13440,.T.);
#10040=FACE_OUTER_BOUND('',#13441,.T.);
#10041=FACE_OUTER_BOUND('',#13442,.T.);
#10042=FACE_OUTER_BOUND('',#13443,.T.);
#10043=FACE_OUTER_BOUND('',#13444,.T.);
#10044=FACE_OUTER_BOUND('',#13445,.T.);
#10045=FACE_OUTER_BOUND('',#13446,.T.);
#10046=FACE_OUTER_BOUND('',#13447,.T.);
#10047=FACE_OUTER_BOUND('',#13448,.T.);
#10048=FACE_OUTER_BOUND('',#13449,.T.);
#10049=FACE_OUTER_BOUND('',#13450,.T.);
#10050=FACE_OUTER_BOUND('',#13451,.T.);
#10051=FACE_OUTER_BOUND('',#13452,.T.);
#10052=FACE_OUTER_BOUND('',#13453,.T.);
#10053=FACE_OUTER_BOUND('',#13454,.T.);
#10054=FACE_OUTER_BOUND('',#13455,.T.);
#10055=FACE_OUTER_BOUND('',#13456,.T.);
#10056=FACE_OUTER_BOUND('',#13457,.T.);
#10057=FACE_OUTER_BOUND('',#13458,.T.);
#10058=FACE_OUTER_BOUND('',#13459,.T.);
#10059=FACE_OUTER_BOUND('',#13460,.T.);
#10060=FACE_OUTER_BOUND('',#13461,.T.);
#10061=FACE_OUTER_BOUND('',#13462,.T.);
#10062=FACE_OUTER_BOUND('',#13463,.T.);
#10063=FACE_OUTER_BOUND('',#13464,.T.);
#10064=FACE_OUTER_BOUND('',#13465,.T.);
#10065=FACE_OUTER_BOUND('',#13466,.T.);
#10066=FACE_OUTER_BOUND('',#13467,.T.);
#10067=FACE_OUTER_BOUND('',#13468,.T.);
#10068=FACE_OUTER_BOUND('',#13469,.T.);
#10069=FACE_OUTER_BOUND('',#13470,.T.);
#10070=FACE_OUTER_BOUND('',#13471,.T.);
#10071=FACE_OUTER_BOUND('',#13472,.T.);
#10072=FACE_OUTER_BOUND('',#13473,.T.);
#10073=FACE_OUTER_BOUND('',#13474,.T.);
#10074=FACE_OUTER_BOUND('',#13475,.T.);
#10075=FACE_OUTER_BOUND('',#13476,.T.);
#10076=FACE_OUTER_BOUND('',#13477,.T.);
#10077=FACE_OUTER_BOUND('',#13478,.T.);
#10078=FACE_OUTER_BOUND('',#13479,.T.);
#10079=FACE_OUTER_BOUND('',#13480,.T.);
#10080=FACE_OUTER_BOUND('',#13481,.T.);
#10081=FACE_OUTER_BOUND('',#13482,.T.);
#10082=FACE_OUTER_BOUND('',#13483,.T.);
#10083=FACE_OUTER_BOUND('',#13484,.T.);
#10084=FACE_OUTER_BOUND('',#13485,.T.);
#10085=FACE_OUTER_BOUND('',#13486,.T.);
#10086=FACE_OUTER_BOUND('',#13487,.T.);
#10087=FACE_OUTER_BOUND('',#13488,.T.);
#10088=FACE_OUTER_BOUND('',#13489,.T.);
#10089=FACE_OUTER_BOUND('',#13490,.T.);
#10090=FACE_OUTER_BOUND('',#13491,.T.);
#10091=FACE_OUTER_BOUND('',#13492,.T.);
#10092=FACE_OUTER_BOUND('',#13493,.T.);
#10093=FACE_OUTER_BOUND('',#13494,.T.);
#10094=FACE_OUTER_BOUND('',#13495,.T.);
#10095=FACE_OUTER_BOUND('',#13496,.T.);
#10096=FACE_OUTER_BOUND('',#13497,.T.);
#10097=FACE_OUTER_BOUND('',#13498,.T.);
#10098=FACE_OUTER_BOUND('',#13499,.T.);
#10099=FACE_OUTER_BOUND('',#13500,.T.);
#10100=FACE_OUTER_BOUND('',#13501,.T.);
#10101=FACE_OUTER_BOUND('',#13502,.T.);
#10102=FACE_OUTER_BOUND('',#13503,.T.);
#10103=FACE_OUTER_BOUND('',#13504,.T.);
#10104=FACE_OUTER_BOUND('',#13505,.T.);
#10105=FACE_OUTER_BOUND('',#13506,.T.);
#10106=FACE_OUTER_BOUND('',#13507,.T.);
#10107=FACE_OUTER_BOUND('',#13508,.T.);
#10108=FACE_OUTER_BOUND('',#13509,.T.);
#10109=FACE_OUTER_BOUND('',#13510,.T.);
#10110=FACE_OUTER_BOUND('',#13511,.T.);
#10111=FACE_OUTER_BOUND('',#13512,.T.);
#10112=FACE_OUTER_BOUND('',#13513,.T.);
#10113=FACE_OUTER_BOUND('',#13514,.T.);
#10114=FACE_OUTER_BOUND('',#13515,.T.);
#10115=FACE_OUTER_BOUND('',#13516,.T.);
#10116=FACE_OUTER_BOUND('',#13517,.T.);
#10117=FACE_OUTER_BOUND('',#13518,.T.);
#10118=FACE_OUTER_BOUND('',#13519,.T.);
#10119=FACE_OUTER_BOUND('',#13520,.T.);
#10120=FACE_OUTER_BOUND('',#13521,.T.);
#10121=FACE_OUTER_BOUND('',#13522,.T.);
#10122=FACE_OUTER_BOUND('',#13523,.T.);
#10123=FACE_OUTER_BOUND('',#13524,.T.);
#10124=FACE_OUTER_BOUND('',#13525,.T.);
#10125=FACE_OUTER_BOUND('',#13526,.T.);
#10126=FACE_OUTER_BOUND('',#13527,.T.);
#10127=FACE_OUTER_BOUND('',#13528,.T.);
#10128=FACE_OUTER_BOUND('',#13529,.T.);
#10129=FACE_OUTER_BOUND('',#13530,.T.);
#10130=FACE_OUTER_BOUND('',#13531,.T.);
#10131=FACE_OUTER_BOUND('',#13532,.T.);
#10132=FACE_OUTER_BOUND('',#13533,.T.);
#10133=FACE_OUTER_BOUND('',#13534,.T.);
#10134=FACE_OUTER_BOUND('',#13535,.T.);
#10135=FACE_OUTER_BOUND('',#13536,.T.);
#10136=FACE_OUTER_BOUND('',#13537,.T.);
#10137=FACE_OUTER_BOUND('',#13538,.T.);
#10138=FACE_OUTER_BOUND('',#13539,.T.);
#10139=FACE_OUTER_BOUND('',#13540,.T.);
#10140=FACE_OUTER_BOUND('',#13541,.T.);
#10141=FACE_OUTER_BOUND('',#13542,.T.);
#10142=FACE_OUTER_BOUND('',#13543,.T.);
#10143=FACE_OUTER_BOUND('',#13592,.T.);
#10144=FACE_OUTER_BOUND('',#13593,.T.);
#10145=FACE_OUTER_BOUND('',#13594,.T.);
#10146=FACE_OUTER_BOUND('',#13595,.T.);
#10147=FACE_OUTER_BOUND('',#13596,.T.);
#10148=FACE_OUTER_BOUND('',#13597,.T.);
#10149=FACE_OUTER_BOUND('',#13598,.T.);
#10150=FACE_OUTER_BOUND('',#13599,.T.);
#10151=FACE_OUTER_BOUND('',#13600,.T.);
#10152=FACE_OUTER_BOUND('',#13601,.T.);
#10153=FACE_OUTER_BOUND('',#13602,.T.);
#10154=FACE_OUTER_BOUND('',#13603,.T.);
#10155=FACE_OUTER_BOUND('',#13604,.T.);
#10156=FACE_OUTER_BOUND('',#13606,.T.);
#10157=FACE_OUTER_BOUND('',#13607,.T.);
#10158=FACE_OUTER_BOUND('',#13608,.T.);
#10159=FACE_OUTER_BOUND('',#13609,.T.);
#10160=FACE_OUTER_BOUND('',#13610,.T.);
#10161=FACE_OUTER_BOUND('',#13611,.T.);
#10162=FACE_OUTER_BOUND('',#13612,.T.);
#10163=FACE_OUTER_BOUND('',#13613,.T.);
#10164=FACE_OUTER_BOUND('',#13614,.T.);
#10165=FACE_OUTER_BOUND('',#13615,.T.);
#10166=FACE_OUTER_BOUND('',#13616,.T.);
#10167=FACE_OUTER_BOUND('',#13617,.T.);
#10168=FACE_OUTER_BOUND('',#13618,.T.);
#10169=FACE_OUTER_BOUND('',#13619,.T.);
#10170=FACE_OUTER_BOUND('',#13620,.T.);
#10171=FACE_OUTER_BOUND('',#13621,.T.);
#10172=FACE_OUTER_BOUND('',#13622,.T.);
#10173=FACE_OUTER_BOUND('',#13623,.T.);
#10174=FACE_OUTER_BOUND('',#13624,.T.);
#10175=FACE_OUTER_BOUND('',#13625,.T.);
#10176=FACE_OUTER_BOUND('',#13626,.T.);
#10177=FACE_OUTER_BOUND('',#13627,.T.);
#10178=FACE_OUTER_BOUND('',#13628,.T.);
#10179=FACE_OUTER_BOUND('',#13629,.T.);
#10180=FACE_OUTER_BOUND('',#13630,.T.);
#10181=FACE_OUTER_BOUND('',#13631,.T.);
#10182=FACE_OUTER_BOUND('',#13632,.T.);
#10183=FACE_OUTER_BOUND('',#13633,.T.);
#10184=FACE_OUTER_BOUND('',#13634,.T.);
#10185=FACE_OUTER_BOUND('',#13635,.T.);
#10186=FACE_OUTER_BOUND('',#13636,.T.);
#10187=FACE_OUTER_BOUND('',#13637,.T.);
#10188=FACE_OUTER_BOUND('',#13638,.T.);
#10189=FACE_OUTER_BOUND('',#13639,.T.);
#10190=FACE_OUTER_BOUND('',#13640,.T.);
#10191=FACE_OUTER_BOUND('',#13641,.T.);
#10192=FACE_OUTER_BOUND('',#13642,.T.);
#10193=FACE_OUTER_BOUND('',#13643,.T.);
#10194=FACE_OUTER_BOUND('',#13644,.T.);
#10195=FACE_OUTER_BOUND('',#13645,.T.);
#10196=FACE_OUTER_BOUND('',#13646,.T.);
#10197=FACE_OUTER_BOUND('',#13647,.T.);
#10198=FACE_OUTER_BOUND('',#13648,.T.);
#10199=FACE_OUTER_BOUND('',#13649,.T.);
#10200=FACE_OUTER_BOUND('',#13650,.T.);
#10201=FACE_OUTER_BOUND('',#13651,.T.);
#10202=FACE_OUTER_BOUND('',#13652,.T.);
#10203=FACE_OUTER_BOUND('',#13653,.T.);
#10204=FACE_OUTER_BOUND('',#13654,.T.);
#10205=FACE_OUTER_BOUND('',#13655,.T.);
#10206=FACE_OUTER_BOUND('',#13656,.T.);
#10207=FACE_OUTER_BOUND('',#13657,.T.);
#10208=FACE_OUTER_BOUND('',#13658,.T.);
#10209=FACE_OUTER_BOUND('',#13659,.T.);
#10210=FACE_OUTER_BOUND('',#13660,.T.);
#10211=FACE_OUTER_BOUND('',#13661,.T.);
#10212=FACE_OUTER_BOUND('',#13662,.T.);
#10213=FACE_OUTER_BOUND('',#13663,.T.);
#10214=FACE_OUTER_BOUND('',#13664,.T.);
#10215=FACE_OUTER_BOUND('',#13665,.T.);
#10216=FACE_OUTER_BOUND('',#13666,.T.);
#10217=FACE_OUTER_BOUND('',#13667,.T.);
#10218=FACE_OUTER_BOUND('',#13668,.T.);
#10219=FACE_OUTER_BOUND('',#13669,.T.);
#10220=FACE_OUTER_BOUND('',#13688,.T.);
#10221=FACE_OUTER_BOUND('',#13925,.T.);
#10222=FACE_OUTER_BOUND('',#13926,.T.);
#10223=FACE_OUTER_BOUND('',#13927,.T.);
#10224=FACE_OUTER_BOUND('',#13928,.T.);
#10225=FACE_OUTER_BOUND('',#13929,.T.);
#10226=FACE_OUTER_BOUND('',#13930,.T.);
#10227=FACE_OUTER_BOUND('',#13931,.T.);
#10228=FACE_OUTER_BOUND('',#13932,.T.);
#10229=FACE_OUTER_BOUND('',#13934,.T.);
#10230=FACE_OUTER_BOUND('',#13935,.T.);
#10231=FACE_OUTER_BOUND('',#13937,.T.);
#10232=FACE_OUTER_BOUND('',#13938,.T.);
#10233=FACE_OUTER_BOUND('',#13940,.T.);
#10234=FACE_OUTER_BOUND('',#13941,.T.);
#10235=FACE_OUTER_BOUND('',#13943,.T.);
#10236=FACE_OUTER_BOUND('',#13944,.T.);
#10237=FACE_OUTER_BOUND('',#13946,.T.);
#10238=FACE_OUTER_BOUND('',#13947,.T.);
#10239=FACE_OUTER_BOUND('',#13949,.T.);
#10240=FACE_OUTER_BOUND('',#13950,.T.);
#10241=FACE_OUTER_BOUND('',#13952,.T.);
#10242=FACE_OUTER_BOUND('',#13953,.T.);
#10243=FACE_OUTER_BOUND('',#13955,.T.);
#10244=FACE_OUTER_BOUND('',#13956,.T.);
#10245=FACE_OUTER_BOUND('',#13958,.T.);
#10246=FACE_OUTER_BOUND('',#13959,.T.);
#10247=FACE_OUTER_BOUND('',#13961,.T.);
#10248=FACE_OUTER_BOUND('',#13962,.T.);
#10249=FACE_OUTER_BOUND('',#13964,.T.);
#10250=FACE_OUTER_BOUND('',#13965,.T.);
#10251=FACE_OUTER_BOUND('',#13967,.T.);
#10252=FACE_OUTER_BOUND('',#13968,.T.);
#10253=FACE_OUTER_BOUND('',#13970,.T.);
#10254=FACE_OUTER_BOUND('',#13971,.T.);
#10255=FACE_OUTER_BOUND('',#13973,.T.);
#10256=FACE_OUTER_BOUND('',#13974,.T.);
#10257=FACE_OUTER_BOUND('',#13976,.T.);
#10258=FACE_OUTER_BOUND('',#13977,.T.);
#10259=FACE_OUTER_BOUND('',#13979,.T.);
#10260=FACE_OUTER_BOUND('',#13980,.T.);
#10261=FACE_OUTER_BOUND('',#13982,.T.);
#10262=FACE_OUTER_BOUND('',#13983,.T.);
#10263=FACE_OUTER_BOUND('',#13985,.T.);
#10264=FACE_OUTER_BOUND('',#13986,.T.);
#10265=FACE_OUTER_BOUND('',#13988,.T.);
#10266=FACE_OUTER_BOUND('',#13989,.T.);
#10267=FACE_OUTER_BOUND('',#13991,.T.);
#10268=FACE_OUTER_BOUND('',#13992,.T.);
#10269=FACE_OUTER_BOUND('',#13994,.T.);
#10270=FACE_OUTER_BOUND('',#13995,.T.);
#10271=FACE_OUTER_BOUND('',#13997,.T.);
#10272=FACE_OUTER_BOUND('',#13998,.T.);
#10273=FACE_OUTER_BOUND('',#14000,.T.);
#10274=FACE_OUTER_BOUND('',#14001,.T.);
#10275=FACE_OUTER_BOUND('',#14003,.T.);
#10276=FACE_OUTER_BOUND('',#14004,.T.);
#10277=FACE_OUTER_BOUND('',#14006,.T.);
#10278=FACE_OUTER_BOUND('',#14007,.T.);
#10279=FACE_OUTER_BOUND('',#14009,.T.);
#10280=FACE_OUTER_BOUND('',#14010,.T.);
#10281=FACE_OUTER_BOUND('',#14012,.T.);
#10282=FACE_OUTER_BOUND('',#14013,.T.);
#10283=FACE_OUTER_BOUND('',#14015,.T.);
#10284=FACE_OUTER_BOUND('',#14016,.T.);
#10285=FACE_OUTER_BOUND('',#14018,.T.);
#10286=FACE_OUTER_BOUND('',#14019,.T.);
#10287=FACE_OUTER_BOUND('',#14021,.T.);
#10288=FACE_OUTER_BOUND('',#14022,.T.);
#10289=FACE_OUTER_BOUND('',#14024,.T.);
#10290=FACE_OUTER_BOUND('',#14025,.T.);
#10291=FACE_OUTER_BOUND('',#14027,.T.);
#10292=FACE_OUTER_BOUND('',#14028,.T.);
#10293=FACE_OUTER_BOUND('',#14030,.T.);
#10294=FACE_OUTER_BOUND('',#14031,.T.);
#10295=FACE_OUTER_BOUND('',#14033,.T.);
#10296=FACE_OUTER_BOUND('',#14034,.T.);
#10297=FACE_OUTER_BOUND('',#14036,.T.);
#10298=FACE_OUTER_BOUND('',#14037,.T.);
#10299=FACE_OUTER_BOUND('',#14039,.T.);
#10300=FACE_OUTER_BOUND('',#14040,.T.);
#10301=FACE_OUTER_BOUND('',#14042,.T.);
#10302=FACE_OUTER_BOUND('',#14043,.T.);
#10303=FACE_OUTER_BOUND('',#14045,.T.);
#10304=FACE_OUTER_BOUND('',#14046,.T.);
#10305=FACE_OUTER_BOUND('',#14048,.T.);
#10306=FACE_OUTER_BOUND('',#14049,.T.);
#10307=FACE_OUTER_BOUND('',#14051,.T.);
#10308=FACE_OUTER_BOUND('',#14052,.T.);
#10309=FACE_OUTER_BOUND('',#14054,.T.);
#10310=FACE_OUTER_BOUND('',#14055,.T.);
#10311=FACE_OUTER_BOUND('',#14057,.T.);
#10312=FACE_OUTER_BOUND('',#14058,.T.);
#10313=FACE_OUTER_BOUND('',#14060,.T.);
#10314=FACE_OUTER_BOUND('',#14061,.T.);
#10315=FACE_OUTER_BOUND('',#14063,.T.);
#10316=FACE_OUTER_BOUND('',#14064,.T.);
#10317=FACE_OUTER_BOUND('',#14066,.T.);
#10318=FACE_OUTER_BOUND('',#14067,.T.);
#10319=FACE_OUTER_BOUND('',#14069,.T.);
#10320=FACE_OUTER_BOUND('',#14070,.T.);
#10321=FACE_OUTER_BOUND('',#14072,.T.);
#10322=FACE_OUTER_BOUND('',#14073,.T.);
#10323=FACE_OUTER_BOUND('',#14075,.T.);
#10324=FACE_OUTER_BOUND('',#14076,.T.);
#10325=FACE_OUTER_BOUND('',#14078,.T.);
#10326=FACE_OUTER_BOUND('',#14079,.T.);
#10327=FACE_OUTER_BOUND('',#14081,.T.);
#10328=FACE_OUTER_BOUND('',#14082,.T.);
#10329=FACE_OUTER_BOUND('',#14084,.T.);
#10330=FACE_OUTER_BOUND('',#14085,.T.);
#10331=FACE_OUTER_BOUND('',#14087,.T.);
#10332=FACE_OUTER_BOUND('',#14088,.T.);
#10333=FACE_OUTER_BOUND('',#14090,.T.);
#10334=FACE_OUTER_BOUND('',#14091,.T.);
#10335=FACE_OUTER_BOUND('',#14093,.T.);
#10336=FACE_OUTER_BOUND('',#14094,.T.);
#10337=FACE_OUTER_BOUND('',#14096,.T.);
#10338=FACE_OUTER_BOUND('',#14097,.T.);
#10339=FACE_OUTER_BOUND('',#14099,.T.);
#10340=FACE_OUTER_BOUND('',#14100,.T.);
#10341=FACE_OUTER_BOUND('',#14102,.T.);
#10342=FACE_OUTER_BOUND('',#14103,.T.);
#10343=FACE_OUTER_BOUND('',#14105,.T.);
#10344=FACE_OUTER_BOUND('',#14106,.T.);
#10345=FACE_OUTER_BOUND('',#14108,.T.);
#10346=FACE_OUTER_BOUND('',#14109,.T.);
#10347=FACE_OUTER_BOUND('',#14111,.T.);
#10348=FACE_OUTER_BOUND('',#14112,.T.);
#10349=FACE_OUTER_BOUND('',#14114,.T.);
#10350=FACE_OUTER_BOUND('',#14115,.T.);
#10351=FACE_OUTER_BOUND('',#14117,.T.);
#10352=FACE_OUTER_BOUND('',#14118,.T.);
#10353=FACE_OUTER_BOUND('',#14120,.T.);
#10354=FACE_OUTER_BOUND('',#14121,.T.);
#10355=FACE_OUTER_BOUND('',#14123,.T.);
#10356=FACE_OUTER_BOUND('',#14124,.T.);
#10357=FACE_OUTER_BOUND('',#14126,.T.);
#10358=FACE_OUTER_BOUND('',#14127,.T.);
#10359=FACE_OUTER_BOUND('',#14129,.T.);
#10360=FACE_OUTER_BOUND('',#14130,.T.);
#10361=FACE_OUTER_BOUND('',#14132,.T.);
#10362=FACE_OUTER_BOUND('',#14133,.T.);
#10363=FACE_OUTER_BOUND('',#14135,.T.);
#10364=FACE_OUTER_BOUND('',#14136,.T.);
#10365=FACE_OUTER_BOUND('',#14138,.T.);
#10366=FACE_OUTER_BOUND('',#14139,.T.);
#10367=FACE_OUTER_BOUND('',#14141,.T.);
#10368=FACE_OUTER_BOUND('',#14142,.T.);
#10369=FACE_OUTER_BOUND('',#14144,.T.);
#10370=FACE_OUTER_BOUND('',#14145,.T.);
#10371=FACE_OUTER_BOUND('',#14147,.T.);
#10372=FACE_OUTER_BOUND('',#14148,.T.);
#10373=FACE_OUTER_BOUND('',#14150,.T.);
#10374=FACE_OUTER_BOUND('',#14151,.T.);
#10375=FACE_OUTER_BOUND('',#14153,.T.);
#10376=FACE_OUTER_BOUND('',#14154,.T.);
#10377=FACE_OUTER_BOUND('',#14156,.T.);
#10378=FACE_OUTER_BOUND('',#14157,.T.);
#10379=FACE_OUTER_BOUND('',#14159,.T.);
#10380=FACE_OUTER_BOUND('',#14160,.T.);
#10381=FACE_OUTER_BOUND('',#14162,.T.);
#10382=FACE_OUTER_BOUND('',#14163,.T.);
#10383=FACE_OUTER_BOUND('',#14165,.T.);
#10384=FACE_OUTER_BOUND('',#14166,.T.);
#10385=FACE_OUTER_BOUND('',#14168,.T.);
#10386=FACE_OUTER_BOUND('',#14169,.T.);
#10387=FACE_OUTER_BOUND('',#14171,.T.);
#10388=FACE_OUTER_BOUND('',#14172,.T.);
#10389=FACE_OUTER_BOUND('',#14174,.T.);
#10390=FACE_OUTER_BOUND('',#14175,.T.);
#10391=FACE_OUTER_BOUND('',#14177,.T.);
#10392=FACE_OUTER_BOUND('',#14178,.T.);
#10393=FACE_OUTER_BOUND('',#14180,.T.);
#10394=FACE_OUTER_BOUND('',#14181,.T.);
#10395=FACE_OUTER_BOUND('',#14183,.T.);
#10396=FACE_OUTER_BOUND('',#14184,.T.);
#10397=FACE_OUTER_BOUND('',#14186,.T.);
#10398=FACE_OUTER_BOUND('',#14187,.T.);
#10399=FACE_OUTER_BOUND('',#14189,.T.);
#10400=FACE_OUTER_BOUND('',#14190,.T.);
#10401=FACE_OUTER_BOUND('',#14192,.T.);
#10402=FACE_OUTER_BOUND('',#14193,.T.);
#10403=FACE_OUTER_BOUND('',#14195,.T.);
#10404=FACE_OUTER_BOUND('',#14196,.T.);
#10405=FACE_OUTER_BOUND('',#14198,.T.);
#10406=FACE_OUTER_BOUND('',#14199,.T.);
#10407=FACE_OUTER_BOUND('',#14201,.T.);
#10408=FACE_OUTER_BOUND('',#14202,.T.);
#10409=FACE_OUTER_BOUND('',#14204,.T.);
#10410=FACE_OUTER_BOUND('',#14205,.T.);
#10411=FACE_OUTER_BOUND('',#14207,.T.);
#10412=FACE_OUTER_BOUND('',#14208,.T.);
#10413=FACE_OUTER_BOUND('',#14210,.T.);
#10414=FACE_OUTER_BOUND('',#14211,.T.);
#10415=FACE_OUTER_BOUND('',#14213,.T.);
#10416=FACE_OUTER_BOUND('',#14214,.T.);
#10417=FACE_OUTER_BOUND('',#14216,.T.);
#10418=FACE_OUTER_BOUND('',#14217,.T.);
#10419=FACE_OUTER_BOUND('',#14219,.T.);
#10420=FACE_OUTER_BOUND('',#14220,.T.);
#10421=FACE_OUTER_BOUND('',#14222,.T.);
#10422=FACE_OUTER_BOUND('',#14223,.T.);
#10423=FACE_OUTER_BOUND('',#14225,.T.);
#10424=FACE_OUTER_BOUND('',#14226,.T.);
#10425=FACE_OUTER_BOUND('',#14228,.T.);
#10426=FACE_OUTER_BOUND('',#14229,.T.);
#10427=FACE_OUTER_BOUND('',#14231,.T.);
#10428=FACE_OUTER_BOUND('',#14232,.T.);
#10429=FACE_OUTER_BOUND('',#14234,.T.);
#10430=FACE_OUTER_BOUND('',#14235,.T.);
#10431=FACE_OUTER_BOUND('',#14237,.T.);
#10432=FACE_OUTER_BOUND('',#14238,.T.);
#10433=FACE_OUTER_BOUND('',#14240,.T.);
#10434=FACE_OUTER_BOUND('',#14241,.T.);
#10435=FACE_OUTER_BOUND('',#14243,.T.);
#10436=FACE_OUTER_BOUND('',#14244,.T.);
#10437=FACE_OUTER_BOUND('',#14246,.T.);
#10438=FACE_OUTER_BOUND('',#14247,.T.);
#10439=FACE_OUTER_BOUND('',#14249,.T.);
#10440=FACE_OUTER_BOUND('',#14250,.T.);
#10441=FACE_OUTER_BOUND('',#14252,.T.);
#10442=FACE_OUTER_BOUND('',#14253,.T.);
#10443=FACE_OUTER_BOUND('',#14255,.T.);
#10444=FACE_OUTER_BOUND('',#14256,.T.);
#10445=FACE_OUTER_BOUND('',#14258,.T.);
#10446=FACE_OUTER_BOUND('',#14259,.T.);
#10447=FACE_OUTER_BOUND('',#14261,.T.);
#10448=FACE_OUTER_BOUND('',#14262,.T.);
#10449=FACE_OUTER_BOUND('',#14264,.T.);
#10450=FACE_OUTER_BOUND('',#14265,.T.);
#10451=FACE_OUTER_BOUND('',#14267,.T.);
#10452=FACE_OUTER_BOUND('',#14268,.T.);
#10453=FACE_OUTER_BOUND('',#14270,.T.);
#10454=FACE_OUTER_BOUND('',#14271,.T.);
#10455=FACE_OUTER_BOUND('',#14273,.T.);
#10456=FACE_OUTER_BOUND('',#14274,.T.);
#10457=FACE_OUTER_BOUND('',#14276,.T.);
#10458=FACE_OUTER_BOUND('',#14277,.T.);
#10459=FACE_OUTER_BOUND('',#14279,.T.);
#10460=FACE_OUTER_BOUND('',#14280,.T.);
#10461=FACE_OUTER_BOUND('',#14282,.T.);
#10462=FACE_OUTER_BOUND('',#14283,.T.);
#10463=FACE_OUTER_BOUND('',#14285,.T.);
#10464=FACE_OUTER_BOUND('',#14286,.T.);
#10465=FACE_OUTER_BOUND('',#14288,.T.);
#10466=FACE_OUTER_BOUND('',#14289,.T.);
#10467=FACE_OUTER_BOUND('',#14291,.T.);
#10468=FACE_OUTER_BOUND('',#14292,.T.);
#10469=FACE_OUTER_BOUND('',#14294,.T.);
#10470=FACE_OUTER_BOUND('',#14295,.T.);
#10471=FACE_OUTER_BOUND('',#14297,.T.);
#10472=FACE_OUTER_BOUND('',#14298,.T.);
#10473=FACE_OUTER_BOUND('',#14300,.T.);
#10474=FACE_OUTER_BOUND('',#14301,.T.);
#10475=FACE_OUTER_BOUND('',#14303,.T.);
#10476=FACE_OUTER_BOUND('',#14304,.T.);
#10477=FACE_OUTER_BOUND('',#14306,.T.);
#10478=FACE_OUTER_BOUND('',#14307,.T.);
#10479=FACE_OUTER_BOUND('',#14309,.T.);
#10480=FACE_OUTER_BOUND('',#14310,.T.);
#10481=FACE_OUTER_BOUND('',#14312,.T.);
#10482=FACE_OUTER_BOUND('',#14313,.T.);
#10483=FACE_OUTER_BOUND('',#14315,.T.);
#10484=FACE_OUTER_BOUND('',#14316,.T.);
#10485=FACE_OUTER_BOUND('',#14318,.T.);
#10486=FACE_OUTER_BOUND('',#14319,.T.);
#10487=FACE_OUTER_BOUND('',#14321,.T.);
#10488=FACE_OUTER_BOUND('',#14322,.T.);
#10489=FACE_OUTER_BOUND('',#14324,.T.);
#10490=FACE_OUTER_BOUND('',#14325,.T.);
#10491=FACE_OUTER_BOUND('',#14327,.T.);
#10492=FACE_OUTER_BOUND('',#14328,.T.);
#10493=FACE_OUTER_BOUND('',#14330,.T.);
#10494=FACE_OUTER_BOUND('',#14331,.T.);
#10495=FACE_OUTER_BOUND('',#14333,.T.);
#10496=FACE_OUTER_BOUND('',#14334,.T.);
#10497=FACE_OUTER_BOUND('',#14336,.T.);
#10498=FACE_OUTER_BOUND('',#14337,.T.);
#10499=FACE_OUTER_BOUND('',#14339,.T.);
#10500=FACE_OUTER_BOUND('',#14340,.T.);
#10501=FACE_OUTER_BOUND('',#14342,.T.);
#10502=FACE_OUTER_BOUND('',#14343,.T.);
#10503=FACE_OUTER_BOUND('',#14345,.T.);
#10504=FACE_OUTER_BOUND('',#14346,.T.);
#10505=FACE_OUTER_BOUND('',#14348,.T.);
#10506=FACE_OUTER_BOUND('',#14349,.T.);
#10507=FACE_OUTER_BOUND('',#14351,.T.);
#10508=FACE_OUTER_BOUND('',#14352,.T.);
#10509=FACE_OUTER_BOUND('',#14354,.T.);
#10510=FACE_OUTER_BOUND('',#14355,.T.);
#10511=FACE_OUTER_BOUND('',#14357,.T.);
#10512=FACE_OUTER_BOUND('',#14358,.T.);
#10513=FACE_OUTER_BOUND('',#14360,.T.);
#10514=FACE_OUTER_BOUND('',#14361,.T.);
#10515=FACE_OUTER_BOUND('',#14363,.T.);
#10516=FACE_OUTER_BOUND('',#14364,.T.);
#10517=FACE_OUTER_BOUND('',#14366,.T.);
#10518=FACE_OUTER_BOUND('',#14367,.T.);
#10519=FACE_OUTER_BOUND('',#14369,.T.);
#10520=FACE_OUTER_BOUND('',#14370,.T.);
#10521=FACE_OUTER_BOUND('',#14372,.T.);
#10522=FACE_OUTER_BOUND('',#14373,.T.);
#10523=FACE_OUTER_BOUND('',#14375,.T.);
#10524=FACE_OUTER_BOUND('',#14376,.T.);
#10525=FACE_OUTER_BOUND('',#14378,.T.);
#10526=FACE_OUTER_BOUND('',#14379,.T.);
#10527=FACE_OUTER_BOUND('',#14381,.T.);
#10528=FACE_OUTER_BOUND('',#14382,.T.);
#10529=FACE_OUTER_BOUND('',#14384,.T.);
#10530=FACE_OUTER_BOUND('',#14385,.T.);
#10531=FACE_OUTER_BOUND('',#14387,.T.);
#10532=FACE_OUTER_BOUND('',#14388,.T.);
#10533=FACE_OUTER_BOUND('',#14390,.T.);
#10534=FACE_OUTER_BOUND('',#14391,.T.);
#10535=FACE_OUTER_BOUND('',#14393,.T.);
#10536=FACE_OUTER_BOUND('',#14394,.T.);
#10537=FACE_OUTER_BOUND('',#14396,.T.);
#10538=FACE_OUTER_BOUND('',#14397,.T.);
#10539=FACE_OUTER_BOUND('',#14399,.T.);
#10540=FACE_OUTER_BOUND('',#14400,.T.);
#10541=FACE_OUTER_BOUND('',#14402,.T.);
#10542=FACE_OUTER_BOUND('',#14403,.T.);
#10543=FACE_OUTER_BOUND('',#14405,.T.);
#10544=FACE_OUTER_BOUND('',#14406,.T.);
#10545=FACE_OUTER_BOUND('',#14408,.T.);
#10546=FACE_OUTER_BOUND('',#14409,.T.);
#10547=FACE_OUTER_BOUND('',#14411,.T.);
#10548=FACE_OUTER_BOUND('',#14412,.T.);
#10549=FACE_OUTER_BOUND('',#14414,.T.);
#10550=FACE_OUTER_BOUND('',#14415,.T.);
#10551=FACE_OUTER_BOUND('',#14417,.T.);
#10552=FACE_OUTER_BOUND('',#14418,.T.);
#10553=FACE_OUTER_BOUND('',#14420,.T.);
#10554=FACE_OUTER_BOUND('',#14421,.T.);
#10555=FACE_OUTER_BOUND('',#14423,.T.);
#10556=FACE_OUTER_BOUND('',#14424,.T.);
#10557=FACE_OUTER_BOUND('',#14426,.T.);
#10558=FACE_OUTER_BOUND('',#14427,.T.);
#10559=FACE_OUTER_BOUND('',#14429,.T.);
#10560=FACE_OUTER_BOUND('',#14430,.T.);
#10561=FACE_OUTER_BOUND('',#14432,.T.);
#10562=FACE_OUTER_BOUND('',#14433,.T.);
#10563=FACE_OUTER_BOUND('',#14435,.T.);
#10564=FACE_OUTER_BOUND('',#14436,.T.);
#10565=FACE_OUTER_BOUND('',#14438,.T.);
#10566=FACE_OUTER_BOUND('',#14439,.T.);
#10567=FACE_OUTER_BOUND('',#14441,.T.);
#10568=FACE_OUTER_BOUND('',#14442,.T.);
#10569=FACE_OUTER_BOUND('',#14444,.T.);
#10570=FACE_OUTER_BOUND('',#14445,.T.);
#10571=FACE_OUTER_BOUND('',#14447,.T.);
#10572=FACE_OUTER_BOUND('',#14448,.T.);
#10573=FACE_OUTER_BOUND('',#14450,.T.);
#10574=FACE_OUTER_BOUND('',#14451,.T.);
#10575=FACE_OUTER_BOUND('',#14453,.T.);
#10576=FACE_OUTER_BOUND('',#14454,.T.);
#10577=FACE_OUTER_BOUND('',#14456,.T.);
#10578=FACE_OUTER_BOUND('',#14457,.T.);
#10579=FACE_OUTER_BOUND('',#14459,.T.);
#10580=FACE_OUTER_BOUND('',#14460,.T.);
#10581=FACE_OUTER_BOUND('',#14462,.T.);
#10582=FACE_OUTER_BOUND('',#14463,.T.);
#10583=FACE_OUTER_BOUND('',#14465,.T.);
#10584=FACE_OUTER_BOUND('',#14466,.T.);
#10585=FACE_OUTER_BOUND('',#14468,.T.);
#10586=FACE_OUTER_BOUND('',#14469,.T.);
#10587=FACE_OUTER_BOUND('',#14471,.T.);
#10588=FACE_OUTER_BOUND('',#14472,.T.);
#10589=FACE_OUTER_BOUND('',#14474,.T.);
#10590=FACE_OUTER_BOUND('',#14475,.T.);
#10591=FACE_OUTER_BOUND('',#14477,.T.);
#10592=FACE_OUTER_BOUND('',#14478,.T.);
#10593=FACE_OUTER_BOUND('',#14480,.T.);
#10594=FACE_OUTER_BOUND('',#14481,.T.);
#10595=FACE_OUTER_BOUND('',#14483,.T.);
#10596=FACE_OUTER_BOUND('',#14484,.T.);
#10597=FACE_OUTER_BOUND('',#14486,.T.);
#10598=FACE_OUTER_BOUND('',#14487,.T.);
#10599=FACE_OUTER_BOUND('',#14489,.T.);
#10600=FACE_OUTER_BOUND('',#14490,.T.);
#10601=FACE_OUTER_BOUND('',#14492,.T.);
#10602=FACE_OUTER_BOUND('',#14493,.T.);
#10603=FACE_OUTER_BOUND('',#14495,.T.);
#10604=FACE_OUTER_BOUND('',#14496,.T.);
#10605=FACE_OUTER_BOUND('',#14498,.T.);
#10606=FACE_OUTER_BOUND('',#14499,.T.);
#10607=FACE_OUTER_BOUND('',#14501,.T.);
#10608=FACE_OUTER_BOUND('',#14502,.T.);
#10609=FACE_OUTER_BOUND('',#14504,.T.);
#10610=FACE_OUTER_BOUND('',#14505,.T.);
#10611=FACE_OUTER_BOUND('',#14507,.T.);
#10612=FACE_OUTER_BOUND('',#14508,.T.);
#10613=FACE_OUTER_BOUND('',#14510,.T.);
#10614=FACE_OUTER_BOUND('',#14511,.T.);
#10615=FACE_OUTER_BOUND('',#14513,.T.);
#10616=FACE_OUTER_BOUND('',#14514,.T.);
#10617=FACE_OUTER_BOUND('',#14516,.T.);
#10618=FACE_OUTER_BOUND('',#14517,.T.);
#10619=FACE_OUTER_BOUND('',#14519,.T.);
#10620=FACE_OUTER_BOUND('',#14520,.T.);
#10621=FACE_OUTER_BOUND('',#14522,.T.);
#10622=FACE_OUTER_BOUND('',#14523,.T.);
#10623=FACE_OUTER_BOUND('',#14525,.T.);
#10624=FACE_OUTER_BOUND('',#14526,.T.);
#10625=FACE_OUTER_BOUND('',#14528,.T.);
#10626=FACE_OUTER_BOUND('',#14529,.T.);
#10627=FACE_OUTER_BOUND('',#14531,.T.);
#10628=FACE_OUTER_BOUND('',#14532,.T.);
#10629=FACE_OUTER_BOUND('',#14534,.T.);
#10630=FACE_OUTER_BOUND('',#14535,.T.);
#10631=FACE_OUTER_BOUND('',#14537,.T.);
#10632=FACE_OUTER_BOUND('',#14538,.T.);
#10633=FACE_OUTER_BOUND('',#14540,.T.);
#10634=FACE_OUTER_BOUND('',#14541,.T.);
#10635=FACE_OUTER_BOUND('',#14543,.T.);
#10636=FACE_OUTER_BOUND('',#14544,.T.);
#10637=FACE_OUTER_BOUND('',#14546,.T.);
#10638=FACE_OUTER_BOUND('',#14547,.T.);
#10639=FACE_OUTER_BOUND('',#14549,.T.);
#10640=FACE_OUTER_BOUND('',#14550,.T.);
#10641=FACE_OUTER_BOUND('',#14552,.T.);
#10642=FACE_OUTER_BOUND('',#14553,.T.);
#10643=FACE_OUTER_BOUND('',#14555,.T.);
#10644=FACE_OUTER_BOUND('',#14556,.T.);
#10645=FACE_OUTER_BOUND('',#14558,.T.);
#10646=FACE_OUTER_BOUND('',#14559,.T.);
#10647=FACE_OUTER_BOUND('',#14561,.T.);
#10648=FACE_OUTER_BOUND('',#14562,.T.);
#10649=FACE_OUTER_BOUND('',#14564,.T.);
#10650=FACE_OUTER_BOUND('',#14565,.T.);
#10651=FACE_OUTER_BOUND('',#14567,.T.);
#10652=FACE_OUTER_BOUND('',#14568,.T.);
#10653=FACE_OUTER_BOUND('',#14570,.T.);
#10654=FACE_OUTER_BOUND('',#14571,.T.);
#10655=FACE_OUTER_BOUND('',#14573,.T.);
#10656=FACE_OUTER_BOUND('',#14574,.T.);
#10657=FACE_OUTER_BOUND('',#14576,.T.);
#10658=FACE_OUTER_BOUND('',#14577,.T.);
#10659=FACE_OUTER_BOUND('',#14579,.T.);
#10660=FACE_OUTER_BOUND('',#14580,.T.);
#10661=FACE_OUTER_BOUND('',#14582,.T.);
#10662=FACE_OUTER_BOUND('',#14583,.T.);
#10663=FACE_OUTER_BOUND('',#14585,.T.);
#10664=FACE_OUTER_BOUND('',#14586,.T.);
#10665=FACE_OUTER_BOUND('',#14588,.T.);
#10666=FACE_OUTER_BOUND('',#14589,.T.);
#10667=FACE_OUTER_BOUND('',#14591,.T.);
#10668=FACE_OUTER_BOUND('',#14592,.T.);
#10669=FACE_OUTER_BOUND('',#14594,.T.);
#10670=FACE_OUTER_BOUND('',#14595,.T.);
#10671=FACE_OUTER_BOUND('',#14597,.T.);
#10672=FACE_OUTER_BOUND('',#14598,.T.);
#10673=FACE_OUTER_BOUND('',#14600,.T.);
#10674=FACE_OUTER_BOUND('',#14601,.T.);
#10675=FACE_OUTER_BOUND('',#14603,.T.);
#10676=FACE_OUTER_BOUND('',#14604,.T.);
#10677=FACE_OUTER_BOUND('',#14606,.T.);
#10678=FACE_OUTER_BOUND('',#14607,.T.);
#10679=FACE_OUTER_BOUND('',#14609,.T.);
#10680=FACE_OUTER_BOUND('',#14610,.T.);
#10681=FACE_OUTER_BOUND('',#14612,.T.);
#10682=FACE_OUTER_BOUND('',#14613,.T.);
#10683=FACE_OUTER_BOUND('',#14615,.T.);
#10684=FACE_OUTER_BOUND('',#14616,.T.);
#10685=FACE_OUTER_BOUND('',#14618,.T.);
#10686=FACE_OUTER_BOUND('',#14619,.T.);
#10687=FACE_OUTER_BOUND('',#14621,.T.);
#10688=FACE_OUTER_BOUND('',#14622,.T.);
#10689=FACE_OUTER_BOUND('',#14624,.T.);
#10690=FACE_OUTER_BOUND('',#14625,.T.);
#10691=FACE_OUTER_BOUND('',#14627,.T.);
#10692=FACE_OUTER_BOUND('',#14628,.T.);
#10693=FACE_OUTER_BOUND('',#14630,.T.);
#10694=FACE_OUTER_BOUND('',#14631,.T.);
#10695=FACE_OUTER_BOUND('',#14633,.T.);
#10696=FACE_OUTER_BOUND('',#14634,.T.);
#10697=FACE_OUTER_BOUND('',#14636,.T.);
#10698=FACE_OUTER_BOUND('',#14637,.T.);
#10699=FACE_OUTER_BOUND('',#14639,.T.);
#10700=FACE_OUTER_BOUND('',#14640,.T.);
#10701=FACE_OUTER_BOUND('',#14642,.T.);
#10702=FACE_OUTER_BOUND('',#14643,.T.);
#10703=FACE_OUTER_BOUND('',#14645,.T.);
#10704=FACE_OUTER_BOUND('',#14646,.T.);
#10705=FACE_OUTER_BOUND('',#14648,.T.);
#10706=FACE_OUTER_BOUND('',#14649,.T.);
#10707=FACE_OUTER_BOUND('',#14651,.T.);
#10708=FACE_OUTER_BOUND('',#14652,.T.);
#10709=FACE_OUTER_BOUND('',#14654,.T.);
#10710=FACE_OUTER_BOUND('',#14655,.T.);
#10711=FACE_OUTER_BOUND('',#14657,.T.);
#10712=FACE_OUTER_BOUND('',#14658,.T.);
#10713=FACE_OUTER_BOUND('',#14660,.T.);
#10714=FACE_OUTER_BOUND('',#14661,.T.);
#10715=FACE_OUTER_BOUND('',#14663,.T.);
#10716=FACE_OUTER_BOUND('',#14664,.T.);
#10717=FACE_OUTER_BOUND('',#14666,.T.);
#10718=FACE_OUTER_BOUND('',#14667,.T.);
#10719=FACE_OUTER_BOUND('',#14669,.T.);
#10720=FACE_OUTER_BOUND('',#14670,.T.);
#10721=FACE_OUTER_BOUND('',#14672,.T.);
#10722=FACE_OUTER_BOUND('',#14673,.T.);
#10723=FACE_OUTER_BOUND('',#14675,.T.);
#10724=FACE_OUTER_BOUND('',#14676,.T.);
#10725=FACE_OUTER_BOUND('',#14678,.T.);
#10726=FACE_OUTER_BOUND('',#14679,.T.);
#10727=FACE_OUTER_BOUND('',#14681,.T.);
#10728=FACE_OUTER_BOUND('',#14682,.T.);
#10729=FACE_OUTER_BOUND('',#14684,.T.);
#10730=FACE_OUTER_BOUND('',#14685,.T.);
#10731=FACE_OUTER_BOUND('',#14687,.T.);
#10732=FACE_OUTER_BOUND('',#14688,.T.);
#10733=FACE_OUTER_BOUND('',#14690,.T.);
#10734=FACE_OUTER_BOUND('',#14691,.T.);
#10735=FACE_OUTER_BOUND('',#14693,.T.);
#10736=FACE_OUTER_BOUND('',#14694,.T.);
#10737=FACE_OUTER_BOUND('',#14696,.T.);
#10738=FACE_OUTER_BOUND('',#14697,.T.);
#10739=FACE_OUTER_BOUND('',#14699,.T.);
#10740=FACE_OUTER_BOUND('',#14700,.T.);
#10741=FACE_OUTER_BOUND('',#14702,.T.);
#10742=FACE_OUTER_BOUND('',#14703,.T.);
#10743=FACE_OUTER_BOUND('',#14705,.T.);
#10744=FACE_OUTER_BOUND('',#14706,.T.);
#10745=FACE_OUTER_BOUND('',#14708,.T.);
#10746=FACE_OUTER_BOUND('',#14709,.T.);
#10747=FACE_OUTER_BOUND('',#14711,.T.);
#10748=FACE_OUTER_BOUND('',#14712,.T.);
#10749=FACE_OUTER_BOUND('',#14714,.T.);
#10750=FACE_OUTER_BOUND('',#14715,.T.);
#10751=FACE_OUTER_BOUND('',#14717,.T.);
#10752=FACE_OUTER_BOUND('',#14718,.T.);
#10753=FACE_OUTER_BOUND('',#14720,.T.);
#10754=FACE_OUTER_BOUND('',#14721,.T.);
#10755=FACE_OUTER_BOUND('',#14723,.T.);
#10756=FACE_OUTER_BOUND('',#14724,.T.);
#10757=FACE_OUTER_BOUND('',#14726,.T.);
#10758=FACE_OUTER_BOUND('',#14727,.T.);
#10759=FACE_OUTER_BOUND('',#14729,.T.);
#10760=FACE_OUTER_BOUND('',#14730,.T.);
#10761=FACE_OUTER_BOUND('',#14732,.T.);
#10762=FACE_OUTER_BOUND('',#14733,.T.);
#10763=FACE_OUTER_BOUND('',#14735,.T.);
#10764=FACE_OUTER_BOUND('',#14736,.T.);
#10765=FACE_OUTER_BOUND('',#14738,.T.);
#10766=FACE_OUTER_BOUND('',#14739,.T.);
#10767=FACE_OUTER_BOUND('',#14741,.T.);
#10768=FACE_OUTER_BOUND('',#14742,.T.);
#10769=FACE_OUTER_BOUND('',#14744,.T.);
#10770=FACE_OUTER_BOUND('',#14745,.T.);
#10771=FACE_OUTER_BOUND('',#14747,.T.);
#10772=FACE_OUTER_BOUND('',#14748,.T.);
#10773=FACE_OUTER_BOUND('',#14750,.T.);
#10774=FACE_OUTER_BOUND('',#14751,.T.);
#10775=FACE_OUTER_BOUND('',#14753,.T.);
#10776=FACE_OUTER_BOUND('',#14754,.T.);
#10777=FACE_OUTER_BOUND('',#14756,.T.);
#10778=FACE_OUTER_BOUND('',#14757,.T.);
#10779=FACE_OUTER_BOUND('',#14759,.T.);
#10780=FACE_OUTER_BOUND('',#14760,.T.);
#10781=FACE_OUTER_BOUND('',#14762,.T.);
#10782=FACE_OUTER_BOUND('',#14763,.T.);
#10783=FACE_OUTER_BOUND('',#14765,.T.);
#10784=FACE_OUTER_BOUND('',#14766,.T.);
#10785=FACE_OUTER_BOUND('',#14768,.T.);
#10786=FACE_OUTER_BOUND('',#14769,.T.);
#10787=FACE_OUTER_BOUND('',#14771,.T.);
#10788=FACE_OUTER_BOUND('',#14772,.T.);
#10789=FACE_OUTER_BOUND('',#14774,.T.);
#10790=FACE_OUTER_BOUND('',#14775,.T.);
#10791=FACE_OUTER_BOUND('',#14777,.T.);
#10792=FACE_OUTER_BOUND('',#14778,.T.);
#10793=FACE_OUTER_BOUND('',#14780,.T.);
#10794=FACE_OUTER_BOUND('',#14781,.T.);
#10795=FACE_OUTER_BOUND('',#14783,.T.);
#10796=FACE_OUTER_BOUND('',#14784,.T.);
#10797=FACE_OUTER_BOUND('',#14786,.T.);
#10798=FACE_OUTER_BOUND('',#14787,.T.);
#10799=FACE_OUTER_BOUND('',#14789,.T.);
#10800=FACE_OUTER_BOUND('',#14790,.T.);
#10801=FACE_OUTER_BOUND('',#14792,.T.);
#10802=FACE_OUTER_BOUND('',#14793,.T.);
#10803=FACE_OUTER_BOUND('',#14795,.T.);
#10804=FACE_OUTER_BOUND('',#14796,.T.);
#10805=FACE_OUTER_BOUND('',#14798,.T.);
#10806=FACE_OUTER_BOUND('',#14799,.T.);
#10807=FACE_OUTER_BOUND('',#14801,.T.);
#10808=FACE_OUTER_BOUND('',#14802,.T.);
#10809=FACE_OUTER_BOUND('',#14804,.T.);
#10810=FACE_OUTER_BOUND('',#14805,.T.);
#10811=FACE_OUTER_BOUND('',#14807,.T.);
#10812=FACE_OUTER_BOUND('',#14808,.T.);
#10813=FACE_OUTER_BOUND('',#14810,.T.);
#10814=FACE_OUTER_BOUND('',#14811,.T.);
#10815=FACE_OUTER_BOUND('',#14813,.T.);
#10816=FACE_OUTER_BOUND('',#14814,.T.);
#10817=FACE_OUTER_BOUND('',#14816,.T.);
#10818=FACE_OUTER_BOUND('',#14817,.T.);
#10819=FACE_OUTER_BOUND('',#14819,.T.);
#10820=FACE_OUTER_BOUND('',#14820,.T.);
#10821=FACE_OUTER_BOUND('',#14822,.T.);
#10822=FACE_OUTER_BOUND('',#14823,.T.);
#10823=FACE_OUTER_BOUND('',#14825,.T.);
#10824=FACE_OUTER_BOUND('',#14826,.T.);
#10825=FACE_OUTER_BOUND('',#14828,.T.);
#10826=FACE_OUTER_BOUND('',#14829,.T.);
#10827=FACE_OUTER_BOUND('',#14831,.T.);
#10828=FACE_OUTER_BOUND('',#14832,.T.);
#10829=FACE_OUTER_BOUND('',#14834,.T.);
#10830=FACE_OUTER_BOUND('',#14835,.T.);
#10831=FACE_OUTER_BOUND('',#14837,.T.);
#10832=FACE_OUTER_BOUND('',#14838,.T.);
#10833=FACE_OUTER_BOUND('',#14840,.T.);
#10834=FACE_OUTER_BOUND('',#14841,.T.);
#10835=FACE_OUTER_BOUND('',#14843,.T.);
#10836=FACE_OUTER_BOUND('',#14844,.T.);
#10837=FACE_OUTER_BOUND('',#14846,.T.);
#10838=FACE_OUTER_BOUND('',#14847,.T.);
#10839=FACE_OUTER_BOUND('',#14849,.T.);
#10840=FACE_OUTER_BOUND('',#14850,.T.);
#10841=FACE_OUTER_BOUND('',#14852,.T.);
#10842=FACE_OUTER_BOUND('',#14853,.T.);
#10843=FACE_OUTER_BOUND('',#14855,.T.);
#10844=FACE_OUTER_BOUND('',#14856,.T.);
#10845=FACE_OUTER_BOUND('',#14858,.T.);
#10846=FACE_OUTER_BOUND('',#14859,.T.);
#10847=FACE_OUTER_BOUND('',#14861,.T.);
#10848=FACE_OUTER_BOUND('',#14862,.T.);
#10849=FACE_OUTER_BOUND('',#14864,.T.);
#10850=FACE_OUTER_BOUND('',#14865,.T.);
#10851=FACE_OUTER_BOUND('',#14867,.T.);
#10852=FACE_OUTER_BOUND('',#14868,.T.);
#10853=FACE_OUTER_BOUND('',#14870,.T.);
#10854=FACE_OUTER_BOUND('',#14871,.T.);
#10855=FACE_OUTER_BOUND('',#14873,.T.);
#10856=FACE_OUTER_BOUND('',#14874,.T.);
#10857=FACE_OUTER_BOUND('',#14876,.T.);
#10858=FACE_OUTER_BOUND('',#14877,.T.);
#10859=FACE_OUTER_BOUND('',#14879,.T.);
#10860=FACE_OUTER_BOUND('',#14880,.T.);
#10861=FACE_OUTER_BOUND('',#14882,.T.);
#10862=FACE_OUTER_BOUND('',#14883,.T.);
#10863=FACE_OUTER_BOUND('',#14885,.T.);
#10864=FACE_OUTER_BOUND('',#14886,.T.);
#10865=FACE_OUTER_BOUND('',#14888,.T.);
#10866=FACE_OUTER_BOUND('',#14889,.T.);
#10867=FACE_OUTER_BOUND('',#14891,.T.);
#10868=FACE_OUTER_BOUND('',#14892,.T.);
#10869=FACE_OUTER_BOUND('',#14894,.T.);
#10870=FACE_OUTER_BOUND('',#14895,.T.);
#10871=FACE_OUTER_BOUND('',#14897,.T.);
#10872=FACE_OUTER_BOUND('',#14898,.T.);
#10873=FACE_OUTER_BOUND('',#14900,.T.);
#10874=FACE_OUTER_BOUND('',#14902,.T.);
#10875=FACE_OUTER_BOUND('',#14903,.T.);
#10876=FACE_OUTER_BOUND('',#14905,.T.);
#10877=FACE_OUTER_BOUND('',#14906,.T.);
#10878=FACE_OUTER_BOUND('',#14908,.T.);
#10879=FACE_OUTER_BOUND('',#14909,.T.);
#10880=FACE_OUTER_BOUND('',#14911,.T.);
#10881=FACE_OUTER_BOUND('',#14912,.T.);
#10882=FACE_OUTER_BOUND('',#14914,.T.);
#10883=FACE_OUTER_BOUND('',#14915,.T.);
#10884=FACE_OUTER_BOUND('',#14917,.T.);
#12875=EDGE_LOOP('',(#30342,#30343,#30344,#30345));
#12876=EDGE_LOOP('',(#30346,#30347,#30348,#30349));
#12877=EDGE_LOOP('',(#30350,#30351,#30352,#30353));
#12878=EDGE_LOOP('',(#30354,#30355,#30356));
#12879=EDGE_LOOP('',(#30357,#30358,#30359));
#12880=EDGE_LOOP('',(#30360,#30361,#30362,#30363));
#12881=EDGE_LOOP('',(#30364,#30365,#30366));
#12882=EDGE_LOOP('',(#30367,#30368,#30369));
#12883=EDGE_LOOP('',(#30370,#30371,#30372,#30373));
#12884=EDGE_LOOP('',(#30374,#30375,#30376,#30377));
#12885=EDGE_LOOP('',(#30378,#30379,#30380,#30381));
#12886=EDGE_LOOP('',(#30382,#30383,#30384,#30385));
#12887=EDGE_LOOP('',(#30386,#30387,#30388,#30389));
#12888=EDGE_LOOP('',(#30390,#30391,#30392,#30393));
#12889=EDGE_LOOP('',(#30394,#30395,#30396,#30397));
#12890=EDGE_LOOP('',(#30398,#30399,#30400,#30401));
#12891=EDGE_LOOP('',(#30402,#30403,#30404,#30405));
#12892=EDGE_LOOP('',(#30406,#30407,#30408,#30409));
#12893=EDGE_LOOP('',(#30410,#30411,#30412,#30413));
#12894=EDGE_LOOP('',(#30414,#30415,#30416,#30417));
#12895=EDGE_LOOP('',(#30418,#30419,#30420,#30421));
#12896=EDGE_LOOP('',(#30422,#30423,#30424,#30425));
#12897=EDGE_LOOP('',(#30426,#30427,#30428,#30429,#30430));
#12898=EDGE_LOOP('',(#30431,#30432,#30433,#30434));
#12899=EDGE_LOOP('',(#30435,#30436,#30437,#30438,#30439));
#12900=EDGE_LOOP('',(#30440,#30441,#30442,#30443));
#12901=EDGE_LOOP('',(#30444,#30445,#30446,#30447,#30448));
#12902=EDGE_LOOP('',(#30449,#30450,#30451,#30452));
#12903=EDGE_LOOP('',(#30453,#30454,#30455,#30456,#30457));
#12904=EDGE_LOOP('',(#30458,#30459,#30460,#30461));
#12905=EDGE_LOOP('',(#30462,#30463,#30464,#30465,#30466));
#12906=EDGE_LOOP('',(#30467,#30468,#30469,#30470));
#12907=EDGE_LOOP('',(#30471,#30472,#30473,#30474,#30475));
#12908=EDGE_LOOP('',(#30476,#30477,#30478,#30479));
#12909=EDGE_LOOP('',(#30480,#30481,#30482,#30483,#30484));
#12910=EDGE_LOOP('',(#30485,#30486,#30487,#30488));
#12911=EDGE_LOOP('',(#30489,#30490,#30491,#30492,#30493));
#12912=EDGE_LOOP('',(#30494,#30495,#30496,#30497));
#12913=EDGE_LOOP('',(#30498,#30499,#30500,#30501,#30502));
#12914=EDGE_LOOP('',(#30503,#30504,#30505,#30506));
#12915=EDGE_LOOP('',(#30507,#30508,#30509,#30510,#30511));
#12916=EDGE_LOOP('',(#30512,#30513,#30514,#30515));
#12917=EDGE_LOOP('',(#30516,#30517,#30518,#30519,#30520));
#12918=EDGE_LOOP('',(#30521,#30522,#30523,#30524));
#12919=EDGE_LOOP('',(#30525,#30526,#30527,#30528,#30529));
#12920=EDGE_LOOP('',(#30530,#30531,#30532,#30533));
#12921=EDGE_LOOP('',(#30534,#30535,#30536,#30537,#30538));
#12922=EDGE_LOOP('',(#30539,#30540,#30541,#30542));
#12923=EDGE_LOOP('',(#30543,#30544,#30545,#30546,#30547));
#12924=EDGE_LOOP('',(#30548,#30549,#30550,#30551));
#12925=EDGE_LOOP('',(#30552,#30553,#30554,#30555,#30556));
#12926=EDGE_LOOP('',(#30557,#30558,#30559,#30560));
#12927=EDGE_LOOP('',(#30561,#30562,#30563,#30564,#30565));
#12928=EDGE_LOOP('',(#30566,#30567,#30568,#30569));
#12929=EDGE_LOOP('',(#30570,#30571,#30572,#30573,#30574));
#12930=EDGE_LOOP('',(#30575,#30576,#30577,#30578));
#12931=EDGE_LOOP('',(#30579,#30580,#30581,#30582,#30583));
#12932=EDGE_LOOP('',(#30584,#30585,#30586,#30587));
#12933=EDGE_LOOP('',(#30588,#30589,#30590,#30591,#30592));
#12934=EDGE_LOOP('',(#30593,#30594,#30595,#30596));
#12935=EDGE_LOOP('',(#30597,#30598,#30599,#30600,#30601));
#12936=EDGE_LOOP('',(#30602,#30603,#30604,#30605));
#12937=EDGE_LOOP('',(#30606,#30607,#30608,#30609,#30610));
#12938=EDGE_LOOP('',(#30611,#30612,#30613,#30614));
#12939=EDGE_LOOP('',(#30615,#30616,#30617,#30618,#30619));
#12940=EDGE_LOOP('',(#30620,#30621,#30622,#30623));
#12941=EDGE_LOOP('',(#30624,#30625,#30626,#30627,#30628));
#12942=EDGE_LOOP('',(#30629,#30630,#30631,#30632));
#12943=EDGE_LOOP('',(#30633,#30634,#30635,#30636,#30637));
#12944=EDGE_LOOP('',(#30638,#30639,#30640,#30641));
#12945=EDGE_LOOP('',(#30642,#30643,#30644,#30645,#30646));
#12946=EDGE_LOOP('',(#30647,#30648,#30649,#30650));
#12947=EDGE_LOOP('',(#30651,#30652,#30653,#30654,#30655));
#12948=EDGE_LOOP('',(#30656,#30657,#30658,#30659));
#12949=EDGE_LOOP('',(#30660,#30661,#30662,#30663,#30664));
#12950=EDGE_LOOP('',(#30665,#30666,#30667,#30668));
#12951=EDGE_LOOP('',(#30669,#30670,#30671,#30672,#30673));
#12952=EDGE_LOOP('',(#30674,#30675,#30676,#30677));
#12953=EDGE_LOOP('',(#30678,#30679,#30680,#30681,#30682));
#12954=EDGE_LOOP('',(#30683,#30684,#30685,#30686));
#12955=EDGE_LOOP('',(#30687,#30688,#30689,#30690,#30691));
#12956=EDGE_LOOP('',(#30692,#30693,#30694,#30695));
#12957=EDGE_LOOP('',(#30696,#30697,#30698,#30699,#30700));
#12958=EDGE_LOOP('',(#30701,#30702,#30703,#30704));
#12959=EDGE_LOOP('',(#30705,#30706,#30707,#30708,#30709));
#12960=EDGE_LOOP('',(#30710,#30711,#30712,#30713));
#12961=EDGE_LOOP('',(#30714,#30715,#30716,#30717,#30718));
#12962=EDGE_LOOP('',(#30719,#30720,#30721,#30722));
#12963=EDGE_LOOP('',(#30723,#30724,#30725,#30726,#30727));
#12964=EDGE_LOOP('',(#30728,#30729,#30730,#30731));
#12965=EDGE_LOOP('',(#30732,#30733,#30734,#30735,#30736));
#12966=EDGE_LOOP('',(#30737,#30738,#30739,#30740));
#12967=EDGE_LOOP('',(#30741,#30742,#30743,#30744,#30745));
#12968=EDGE_LOOP('',(#30746,#30747,#30748,#30749));
#12969=EDGE_LOOP('',(#30750,#30751,#30752,#30753,#30754));
#12970=EDGE_LOOP('',(#30755,#30756,#30757,#30758));
#12971=EDGE_LOOP('',(#30759,#30760,#30761,#30762,#30763));
#12972=EDGE_LOOP('',(#30764,#30765,#30766,#30767));
#12973=EDGE_LOOP('',(#30768,#30769,#30770,#30771,#30772));
#12974=EDGE_LOOP('',(#30773,#30774,#30775,#30776));
#12975=EDGE_LOOP('',(#30777,#30778,#30779,#30780));
#12976=EDGE_LOOP('',(#30781,#30782,#30783,#30784));
#12977=EDGE_LOOP('',(#30785,#30786,#30787,#30788));
#12978=EDGE_LOOP('',(#30789,#30790,#30791,#30792));
#12979=EDGE_LOOP('',(#30793,#30794,#30795,#30796,#30797));
#12980=EDGE_LOOP('',(#30798,#30799,#30800,#30801));
#12981=EDGE_LOOP('',(#30802,#30803,#30804,#30805,#30806));
#12982=EDGE_LOOP('',(#30807,#30808,#30809,#30810));
#12983=EDGE_LOOP('',(#30811,#30812,#30813,#30814));
#12984=EDGE_LOOP('',(#30815,#30816,#30817,#30818));
#12985=EDGE_LOOP('',(#30819,#30820,#30821,#30822));
#12986=EDGE_LOOP('',(#30823,#30824,#30825,#30826));
#12987=EDGE_LOOP('',(#30827,#30828,#30829,#30830,#30831));
#12988=EDGE_LOOP('',(#30832,#30833,#30834,#30835));
#12989=EDGE_LOOP('',(#30836,#30837,#30838,#30839,#30840));
#12990=EDGE_LOOP('',(#30841,#30842,#30843,#30844));
#12991=EDGE_LOOP('',(#30845,#30846,#30847,#30848));
#12992=EDGE_LOOP('',(#30849,#30850,#30851,#30852));
#12993=EDGE_LOOP('',(#30853,#30854,#30855,#30856,#30857));
#12994=EDGE_LOOP('',(#30858,#30859,#30860,#30861));
#12995=EDGE_LOOP('',(#30862,#30863,#30864,#30865,#30866));
#12996=EDGE_LOOP('',(#30867,#30868,#30869,#30870));
#12997=EDGE_LOOP('',(#30871,#30872,#30873,#30874));
#12998=EDGE_LOOP('',(#30875,#30876,#30877,#30878));
#12999=EDGE_LOOP('',(#30879,#30880,#30881,#30882,#30883));
#13000=EDGE_LOOP('',(#30884,#30885,#30886,#30887));
#13001=EDGE_LOOP('',(#30888,#30889,#30890,#30891,#30892));
#13002=EDGE_LOOP('',(#30893,#30894,#30895,#30896));
#13003=EDGE_LOOP('',(#30897,#30898,#30899,#30900,#30901));
#13004=EDGE_LOOP('',(#30902,#30903,#30904,#30905));
#13005=EDGE_LOOP('',(#30906,#30907,#30908,#30909,#30910));
#13006=EDGE_LOOP('',(#30911,#30912,#30913,#30914));
#13007=EDGE_LOOP('',(#30915,#30916,#30917,#30918,#30919));
#13008=EDGE_LOOP('',(#30920,#30921,#30922,#30923));
#13009=EDGE_LOOP('',(#30924,#30925,#30926,#30927,#30928));
#13010=EDGE_LOOP('',(#30929,#30930,#30931,#30932));
#13011=EDGE_LOOP('',(#30933,#30934,#30935,#30936,#30937));
#13012=EDGE_LOOP('',(#30938,#30939,#30940,#30941));
#13013=EDGE_LOOP('',(#30942,#30943,#30944,#30945,#30946));
#13014=EDGE_LOOP('',(#30947,#30948,#30949,#30950));
#13015=EDGE_LOOP('',(#30951,#30952,#30953,#30954,#30955));
#13016=EDGE_LOOP('',(#30956,#30957,#30958,#30959));
#13017=EDGE_LOOP('',(#30960,#30961,#30962,#30963,#30964));
#13018=EDGE_LOOP('',(#30965,#30966,#30967,#30968));
#13019=EDGE_LOOP('',(#30969,#30970,#30971,#30972,#30973));
#13020=EDGE_LOOP('',(#30974,#30975,#30976,#30977));
#13021=EDGE_LOOP('',(#30978,#30979,#30980,#30981,#30982));
#13022=EDGE_LOOP('',(#30983,#30984,#30985,#30986));
#13023=EDGE_LOOP('',(#30987,#30988,#30989,#30990,#30991));
#13024=EDGE_LOOP('',(#30992,#30993,#30994,#30995));
#13025=EDGE_LOOP('',(#30996,#30997,#30998,#30999,#31000));
#13026=EDGE_LOOP('',(#31001,#31002,#31003,#31004));
#13027=EDGE_LOOP('',(#31005,#31006,#31007,#31008));
#13028=EDGE_LOOP('',(#31009,#31010,#31011,#31012));
#13029=EDGE_LOOP('',(#31013,#31014,#31015,#31016));
#13030=EDGE_LOOP('',(#31017,#31018,#31019,#31020));
#13031=EDGE_LOOP('',(#31021,#31022,#31023,#31024));
#13032=EDGE_LOOP('',(#31025,#31026,#31027,#31028));
#13033=EDGE_LOOP('',(#31029,#31030,#31031,#31032));
#13034=EDGE_LOOP('',(#31033,#31034,#31035,#31036));
#13035=EDGE_LOOP('',(#31037,#31038,#31039,#31040));
#13036=EDGE_LOOP('',(#31041,#31042,#31043,#31044));
#13037=EDGE_LOOP('',(#31045,#31046,#31047,#31048));
#13038=EDGE_LOOP('',(#31049,#31050,#31051,#31052));
#13039=EDGE_LOOP('',(#31053,#31054,#31055,#31056));
#13040=EDGE_LOOP('',(#31057,#31058,#31059,#31060));
#13041=EDGE_LOOP('',(#31061,#31062,#31063,#31064));
#13042=EDGE_LOOP('',(#31065,#31066,#31067,#31068));
#13043=EDGE_LOOP('',(#31069,#31070,#31071,#31072,#31073,#31074));
#13044=EDGE_LOOP('',(#31075,#31076,#31077,#31078));
#13045=EDGE_LOOP('',(#31079,#31080,#31081,#31082));
#13046=EDGE_LOOP('',(#31083,#31084,#31085,#31086));
#13047=EDGE_LOOP('',(#31087,#31088,#31089,#31090));
#13048=EDGE_LOOP('',(#31091,#31092,#31093,#31094));
#13049=EDGE_LOOP('',(#31095,#31096,#31097,#31098));
#13050=EDGE_LOOP('',(#31099,#31100,#31101,#31102));
#13051=EDGE_LOOP('',(#31103,#31104,#31105,#31106));
#13052=EDGE_LOOP('',(#31107,#31108,#31109,#31110));
#13053=EDGE_LOOP('',(#31111,#31112,#31113,#31114));
#13054=EDGE_LOOP('',(#31115,#31116,#31117,#31118));
#13055=EDGE_LOOP('',(#31119,#31120,#31121,#31122));
#13056=EDGE_LOOP('',(#31123,#31124,#31125,#31126));
#13057=EDGE_LOOP('',(#31127,#31128,#31129,#31130));
#13058=EDGE_LOOP('',(#31131,#31132,#31133,#31134));
#13059=EDGE_LOOP('',(#31135,#31136,#31137,#31138));
#13060=EDGE_LOOP('',(#31139,#31140,#31141,#31142));
#13061=EDGE_LOOP('',(#31143,#31144,#31145,#31146,#31147,#31148));
#13062=EDGE_LOOP('',(#31149,#31150,#31151,#31152));
#13063=EDGE_LOOP('',(#31153,#31154,#31155,#31156));
#13064=EDGE_LOOP('',(#31157,#31158,#31159,#31160));
#13065=EDGE_LOOP('',(#31161,#31162,#31163,#31164));
#13066=EDGE_LOOP('',(#31165,#31166,#31167,#31168));
#13067=EDGE_LOOP('',(#31169,#31170,#31171,#31172));
#13068=EDGE_LOOP('',(#31173,#31174,#31175,#31176));
#13069=EDGE_LOOP('',(#31177,#31178,#31179,#31180));
#13070=EDGE_LOOP('',(#31181,#31182,#31183,#31184));
#13071=EDGE_LOOP('',(#31185,#31186,#31187,#31188));
#13072=EDGE_LOOP('',(#31189,#31190,#31191,#31192));
#13073=EDGE_LOOP('',(#31193,#31194,#31195,#31196));
#13074=EDGE_LOOP('',(#31197,#31198,#31199,#31200));
#13075=EDGE_LOOP('',(#31201,#31202,#31203,#31204));
#13076=EDGE_LOOP('',(#31205,#31206,#31207,#31208));
#13077=EDGE_LOOP('',(#31209,#31210,#31211,#31212,#31213,#31214));
#13078=EDGE_LOOP('',(#31215,#31216,#31217,#31218));
#13079=EDGE_LOOP('',(#31219,#31220,#31221,#31222));
#13080=EDGE_LOOP('',(#31223,#31224,#31225,#31226));
#13081=EDGE_LOOP('',(#31227,#31228,#31229,#31230));
#13082=EDGE_LOOP('',(#31231,#31232,#31233,#31234));
#13083=EDGE_LOOP('',(#31235,#31236,#31237,#31238));
#13084=EDGE_LOOP('',(#31239,#31240,#31241,#31242));
#13085=EDGE_LOOP('',(#31243,#31244,#31245,#31246));
#13086=EDGE_LOOP('',(#31247,#31248,#31249,#31250));
#13087=EDGE_LOOP('',(#31251,#31252,#31253,#31254));
#13088=EDGE_LOOP('',(#31255,#31256,#31257,#31258));
#13089=EDGE_LOOP('',(#31259,#31260,#31261,#31262));
#13090=EDGE_LOOP('',(#31263,#31264,#31265,#31266));
#13091=EDGE_LOOP('',(#31267,#31268,#31269,#31270));
#13092=EDGE_LOOP('',(#31271,#31272,#31273,#31274));
#13093=EDGE_LOOP('',(#31275,#31276,#31277,#31278));
#13094=EDGE_LOOP('',(#31279,#31280,#31281,#31282));
#13095=EDGE_LOOP('',(#31283,#31284,#31285,#31286,#31287,#31288));
#13096=EDGE_LOOP('',(#31289,#31290,#31291,#31292));
#13097=EDGE_LOOP('',(#31293,#31294,#31295,#31296));
#13098=EDGE_LOOP('',(#31297,#31298,#31299,#31300));
#13099=EDGE_LOOP('',(#31301,#31302,#31303,#31304));
#13100=EDGE_LOOP('',(#31305,#31306,#31307,#31308));
#13101=EDGE_LOOP('',(#31309,#31310,#31311,#31312));
#13102=EDGE_LOOP('',(#31313,#31314,#31315,#31316));
#13103=EDGE_LOOP('',(#31317,#31318,#31319,#31320));
#13104=EDGE_LOOP('',(#31321,#31322,#31323,#31324));
#13105=EDGE_LOOP('',(#31325,#31326,#31327,#31328));
#13106=EDGE_LOOP('',(#31329,#31330,#31331,#31332));
#13107=EDGE_LOOP('',(#31333,#31334,#31335,#31336));
#13108=EDGE_LOOP('',(#31337,#31338,#31339,#31340));
#13109=EDGE_LOOP('',(#31341,#31342,#31343,#31344));
#13110=EDGE_LOOP('',(#31345,#31346,#31347,#31348));
#13111=EDGE_LOOP('',(#31349,#31350,#31351,#31352));
#13112=EDGE_LOOP('',(#31353,#31354,#31355,#31356));
#13113=EDGE_LOOP('',(#31357,#31358,#31359,#31360,#31361,#31362));
#13114=EDGE_LOOP('',(#31363,#31364,#31365,#31366));
#13115=EDGE_LOOP('',(#31367,#31368,#31369,#31370));
#13116=EDGE_LOOP('',(#31371,#31372,#31373,#31374));
#13117=EDGE_LOOP('',(#31375,#31376,#31377,#31378));
#13118=EDGE_LOOP('',(#31379,#31380,#31381,#31382));
#13119=EDGE_LOOP('',(#31383,#31384,#31385,#31386));
#13120=EDGE_LOOP('',(#31387,#31388,#31389,#31390));
#13121=EDGE_LOOP('',(#31391,#31392,#31393,#31394));
#13122=EDGE_LOOP('',(#31395,#31396,#31397,#31398));
#13123=EDGE_LOOP('',(#31399,#31400,#31401,#31402));
#13124=EDGE_LOOP('',(#31403,#31404,#31405,#31406));
#13125=EDGE_LOOP('',(#31407,#31408,#31409,#31410));
#13126=EDGE_LOOP('',(#31411,#31412,#31413,#31414));
#13127=EDGE_LOOP('',(#31415,#31416,#31417,#31418));
#13128=EDGE_LOOP('',(#31419,#31420,#31421,#31422));
#13129=EDGE_LOOP('',(#31423,#31424,#31425,#31426));
#13130=EDGE_LOOP('',(#31427,#31428,#31429,#31430));
#13131=EDGE_LOOP('',(#31431,#31432,#31433,#31434,#31435,#31436));
#13132=EDGE_LOOP('',(#31437,#31438,#31439,#31440));
#13133=EDGE_LOOP('',(#31441,#31442,#31443,#31444));
#13134=EDGE_LOOP('',(#31445,#31446,#31447,#31448));
#13135=EDGE_LOOP('',(#31449,#31450,#31451,#31452));
#13136=EDGE_LOOP('',(#31453,#31454,#31455,#31456));
#13137=EDGE_LOOP('',(#31457,#31458,#31459,#31460));
#13138=EDGE_LOOP('',(#31461,#31462,#31463,#31464));
#13139=EDGE_LOOP('',(#31465,#31466,#31467,#31468));
#13140=EDGE_LOOP('',(#31469,#31470,#31471,#31472));
#13141=EDGE_LOOP('',(#31473,#31474,#31475,#31476));
#13142=EDGE_LOOP('',(#31477,#31478,#31479,#31480));
#13143=EDGE_LOOP('',(#31481,#31482,#31483,#31484));
#13144=EDGE_LOOP('',(#31485,#31486,#31487,#31488));
#13145=EDGE_LOOP('',(#31489,#31490,#31491,#31492));
#13146=EDGE_LOOP('',(#31493,#31494,#31495,#31496));
#13147=EDGE_LOOP('',(#31497,#31498,#31499,#31500));
#13148=EDGE_LOOP('',(#31501,#31502,#31503,#31504));
#13149=EDGE_LOOP('',(#31505,#31506,#31507,#31508,#31509,#31510));
#13150=EDGE_LOOP('',(#31511,#31512,#31513,#31514));
#13151=EDGE_LOOP('',(#31515,#31516,#31517,#31518));
#13152=EDGE_LOOP('',(#31519,#31520,#31521,#31522));
#13153=EDGE_LOOP('',(#31523,#31524,#31525,#31526));
#13154=EDGE_LOOP('',(#31527,#31528,#31529,#31530));
#13155=EDGE_LOOP('',(#31531,#31532,#31533,#31534));
#13156=EDGE_LOOP('',(#31535,#31536,#31537,#31538));
#13157=EDGE_LOOP('',(#31539,#31540,#31541,#31542));
#13158=EDGE_LOOP('',(#31543,#31544,#31545,#31546));
#13159=EDGE_LOOP('',(#31547,#31548,#31549,#31550));
#13160=EDGE_LOOP('',(#31551,#31552,#31553,#31554));
#13161=EDGE_LOOP('',(#31555,#31556,#31557,#31558));
#13162=EDGE_LOOP('',(#31559,#31560,#31561,#31562));
#13163=EDGE_LOOP('',(#31563,#31564,#31565,#31566));
#13164=EDGE_LOOP('',(#31567,#31568,#31569,#31570));
#13165=EDGE_LOOP('',(#31571,#31572,#31573,#31574,#31575,#31576));
#13166=EDGE_LOOP('',(#31577,#31578,#31579,#31580));
#13167=EDGE_LOOP('',(#31581,#31582,#31583,#31584));
#13168=EDGE_LOOP('',(#31585,#31586,#31587,#31588));
#13169=EDGE_LOOP('',(#31589,#31590,#31591,#31592));
#13170=EDGE_LOOP('',(#31593,#31594,#31595,#31596));
#13171=EDGE_LOOP('',(#31597,#31598,#31599,#31600));
#13172=EDGE_LOOP('',(#31601,#31602,#31603,#31604));
#13173=EDGE_LOOP('',(#31605,#31606,#31607,#31608));
#13174=EDGE_LOOP('',(#31609,#31610,#31611,#31612));
#13175=EDGE_LOOP('',(#31613,#31614,#31615,#31616));
#13176=EDGE_LOOP('',(#31617,#31618,#31619,#31620));
#13177=EDGE_LOOP('',(#31621,#31622,#31623,#31624));
#13178=EDGE_LOOP('',(#31625,#31626,#31627,#31628));
#13179=EDGE_LOOP('',(#31629,#31630,#31631,#31632));
#13180=EDGE_LOOP('',(#31633,#31634,#31635,#31636));
#13181=EDGE_LOOP('',(#31637,#31638,#31639,#31640));
#13182=EDGE_LOOP('',(#31641,#31642,#31643,#31644));
#13183=EDGE_LOOP('',(#31645,#31646,#31647,#31648,#31649,#31650));
#13184=EDGE_LOOP('',(#31651,#31652,#31653,#31654));
#13185=EDGE_LOOP('',(#31655,#31656,#31657,#31658));
#13186=EDGE_LOOP('',(#31659,#31660,#31661,#31662));
#13187=EDGE_LOOP('',(#31663,#31664,#31665,#31666));
#13188=EDGE_LOOP('',(#31667,#31668,#31669,#31670));
#13189=EDGE_LOOP('',(#31671,#31672,#31673,#31674));
#13190=EDGE_LOOP('',(#31675,#31676,#31677,#31678));
#13191=EDGE_LOOP('',(#31679,#31680,#31681,#31682));
#13192=EDGE_LOOP('',(#31683,#31684,#31685,#31686));
#13193=EDGE_LOOP('',(#31687,#31688,#31689,#31690));
#13194=EDGE_LOOP('',(#31691,#31692,#31693,#31694));
#13195=EDGE_LOOP('',(#31695,#31696,#31697,#31698));
#13196=EDGE_LOOP('',(#31699,#31700,#31701,#31702));
#13197=EDGE_LOOP('',(#31703,#31704,#31705,#31706));
#13198=EDGE_LOOP('',(#31707,#31708,#31709,#31710));
#13199=EDGE_LOOP('',(#31711,#31712,#31713,#31714));
#13200=EDGE_LOOP('',(#31715,#31716,#31717,#31718));
#13201=EDGE_LOOP('',(#31719,#31720,#31721,#31722,#31723,#31724));
#13202=EDGE_LOOP('',(#31725,#31726,#31727,#31728));
#13203=EDGE_LOOP('',(#31729,#31730,#31731,#31732));
#13204=EDGE_LOOP('',(#31733,#31734,#31735,#31736));
#13205=EDGE_LOOP('',(#31737,#31738,#31739,#31740));
#13206=EDGE_LOOP('',(#31741,#31742,#31743,#31744));
#13207=EDGE_LOOP('',(#31745,#31746,#31747,#31748));
#13208=EDGE_LOOP('',(#31749,#31750,#31751,#31752));
#13209=EDGE_LOOP('',(#31753,#31754,#31755,#31756));
#13210=EDGE_LOOP('',(#31757,#31758,#31759,#31760));
#13211=EDGE_LOOP('',(#31761,#31762,#31763,#31764));
#13212=EDGE_LOOP('',(#31765,#31766,#31767,#31768));
#13213=EDGE_LOOP('',(#31769,#31770,#31771,#31772));
#13214=EDGE_LOOP('',(#31773,#31774,#31775,#31776));
#13215=EDGE_LOOP('',(#31777,#31778,#31779,#31780));
#13216=EDGE_LOOP('',(#31781,#31782,#31783,#31784));
#13217=EDGE_LOOP('',(#31785,#31786,#31787,#31788));
#13218=EDGE_LOOP('',(#31789,#31790,#31791,#31792));
#13219=EDGE_LOOP('',(#31793,#31794,#31795,#31796,#31797,#31798));
#13220=EDGE_LOOP('',(#31799,#31800,#31801,#31802));
#13221=EDGE_LOOP('',(#31803,#31804,#31805,#31806));
#13222=EDGE_LOOP('',(#31807,#31808,#31809,#31810));
#13223=EDGE_LOOP('',(#31811,#31812,#31813,#31814));
#13224=EDGE_LOOP('',(#31815,#31816,#31817,#31818));
#13225=EDGE_LOOP('',(#31819,#31820,#31821,#31822));
#13226=EDGE_LOOP('',(#31823,#31824,#31825,#31826));
#13227=EDGE_LOOP('',(#31827,#31828,#31829,#31830));
#13228=EDGE_LOOP('',(#31831,#31832,#31833,#31834));
#13229=EDGE_LOOP('',(#31835,#31836,#31837,#31838));
#13230=EDGE_LOOP('',(#31839,#31840,#31841,#31842));
#13231=EDGE_LOOP('',(#31843,#31844,#31845,#31846));
#13232=EDGE_LOOP('',(#31847,#31848,#31849,#31850));
#13233=EDGE_LOOP('',(#31851,#31852,#31853,#31854));
#13234=EDGE_LOOP('',(#31855,#31856,#31857,#31858));
#13235=EDGE_LOOP('',(#31859,#31860,#31861,#31862));
#13236=EDGE_LOOP('',(#31863,#31864,#31865,#31866));
#13237=EDGE_LOOP('',(#31867,#31868,#31869,#31870,#31871,#31872));
#13238=EDGE_LOOP('',(#31873,#31874,#31875,#31876));
#13239=EDGE_LOOP('',(#31877,#31878,#31879,#31880));
#13240=EDGE_LOOP('',(#31881,#31882,#31883,#31884));
#13241=EDGE_LOOP('',(#31885,#31886,#31887,#31888));
#13242=EDGE_LOOP('',(#31889,#31890,#31891,#31892));
#13243=EDGE_LOOP('',(#31893,#31894,#31895,#31896));
#13244=EDGE_LOOP('',(#31897,#31898,#31899,#31900));
#13245=EDGE_LOOP('',(#31901,#31902,#31903,#31904));
#13246=EDGE_LOOP('',(#31905,#31906,#31907,#31908));
#13247=EDGE_LOOP('',(#31909,#31910,#31911,#31912));
#13248=EDGE_LOOP('',(#31913,#31914,#31915,#31916));
#13249=EDGE_LOOP('',(#31917,#31918,#31919,#31920));
#13250=EDGE_LOOP('',(#31921,#31922,#31923,#31924));
#13251=EDGE_LOOP('',(#31925,#31926,#31927,#31928));
#13252=EDGE_LOOP('',(#31929,#31930,#31931,#31932));
#13253=EDGE_LOOP('',(#31933,#31934,#31935,#31936,#31937,#31938));
#13254=EDGE_LOOP('',(#31939,#31940,#31941,#31942));
#13255=EDGE_LOOP('',(#31943,#31944,#31945,#31946));
#13256=EDGE_LOOP('',(#31947,#31948,#31949,#31950));
#13257=EDGE_LOOP('',(#31951,#31952,#31953,#31954));
#13258=EDGE_LOOP('',(#31955,#31956,#31957,#31958));
#13259=EDGE_LOOP('',(#31959,#31960,#31961,#31962));
#13260=EDGE_LOOP('',(#31963,#31964,#31965,#31966));
#13261=EDGE_LOOP('',(#31967,#31968,#31969,#31970));
#13262=EDGE_LOOP('',(#31971,#31972,#31973,#31974));
#13263=EDGE_LOOP('',(#31975,#31976,#31977,#31978));
#13264=EDGE_LOOP('',(#31979,#31980,#31981,#31982));
#13265=EDGE_LOOP('',(#31983,#31984,#31985,#31986));
#13266=EDGE_LOOP('',(#31987,#31988,#31989,#31990));
#13267=EDGE_LOOP('',(#31991,#31992,#31993,#31994));
#13268=EDGE_LOOP('',(#31995,#31996,#31997,#31998));
#13269=EDGE_LOOP('',(#31999,#32000,#32001,#32002));
#13270=EDGE_LOOP('',(#32003,#32004,#32005,#32006));
#13271=EDGE_LOOP('',(#32007,#32008,#32009,#32010,#32011,#32012));
#13272=EDGE_LOOP('',(#32013,#32014,#32015,#32016));
#13273=EDGE_LOOP('',(#32017,#32018,#32019,#32020));
#13274=EDGE_LOOP('',(#32021,#32022,#32023,#32024));
#13275=EDGE_LOOP('',(#32025,#32026,#32027,#32028));
#13276=EDGE_LOOP('',(#32029,#32030,#32031,#32032));
#13277=EDGE_LOOP('',(#32033,#32034,#32035,#32036));
#13278=EDGE_LOOP('',(#32037,#32038,#32039,#32040));
#13279=EDGE_LOOP('',(#32041,#32042,#32043,#32044));
#13280=EDGE_LOOP('',(#32045,#32046,#32047,#32048));
#13281=EDGE_LOOP('',(#32049,#32050,#32051,#32052));
#13282=EDGE_LOOP('',(#32053,#32054,#32055,#32056));
#13283=EDGE_LOOP('',(#32057,#32058,#32059,#32060));
#13284=EDGE_LOOP('',(#32061,#32062,#32063,#32064));
#13285=EDGE_LOOP('',(#32065,#32066,#32067,#32068));
#13286=EDGE_LOOP('',(#32069,#32070,#32071,#32072));
#13287=EDGE_LOOP('',(#32073,#32074,#32075,#32076));
#13288=EDGE_LOOP('',(#32077,#32078,#32079,#32080));
#13289=EDGE_LOOP('',(#32081,#32082,#32083,#32084,#32085,#32086));
#13290=EDGE_LOOP('',(#32087,#32088,#32089,#32090));
#13291=EDGE_LOOP('',(#32091,#32092,#32093,#32094));
#13292=EDGE_LOOP('',(#32095,#32096,#32097,#32098));
#13293=EDGE_LOOP('',(#32099,#32100,#32101,#32102));
#13294=EDGE_LOOP('',(#32103,#32104,#32105,#32106));
#13295=EDGE_LOOP('',(#32107,#32108,#32109,#32110));
#13296=EDGE_LOOP('',(#32111,#32112,#32113,#32114));
#13297=EDGE_LOOP('',(#32115,#32116,#32117,#32118));
#13298=EDGE_LOOP('',(#32119,#32120,#32121,#32122));
#13299=EDGE_LOOP('',(#32123,#32124,#32125,#32126));
#13300=EDGE_LOOP('',(#32127,#32128,#32129,#32130));
#13301=EDGE_LOOP('',(#32131,#32132,#32133,#32134));
#13302=EDGE_LOOP('',(#32135,#32136,#32137,#32138));
#13303=EDGE_LOOP('',(#32139,#32140,#32141,#32142));
#13304=EDGE_LOOP('',(#32143,#32144,#32145,#32146));
#13305=EDGE_LOOP('',(#32147,#32148,#32149,#32150));
#13306=EDGE_LOOP('',(#32151,#32152,#32153,#32154));
#13307=EDGE_LOOP('',(#32155,#32156,#32157,#32158,#32159,#32160));
#13308=EDGE_LOOP('',(#32161,#32162,#32163,#32164));
#13309=EDGE_LOOP('',(#32165,#32166,#32167,#32168));
#13310=EDGE_LOOP('',(#32169,#32170,#32171,#32172));
#13311=EDGE_LOOP('',(#32173,#32174,#32175,#32176));
#13312=EDGE_LOOP('',(#32177,#32178,#32179,#32180));
#13313=EDGE_LOOP('',(#32181,#32182,#32183,#32184));
#13314=EDGE_LOOP('',(#32185,#32186,#32187,#32188));
#13315=EDGE_LOOP('',(#32189,#32190,#32191,#32192));
#13316=EDGE_LOOP('',(#32193,#32194,#32195,#32196));
#13317=EDGE_LOOP('',(#32197,#32198,#32199,#32200));
#13318=EDGE_LOOP('',(#32201,#32202,#32203,#32204));
#13319=EDGE_LOOP('',(#32205,#32206,#32207,#32208));
#13320=EDGE_LOOP('',(#32209,#32210,#32211,#32212));
#13321=EDGE_LOOP('',(#32213,#32214,#32215,#32216));
#13322=EDGE_LOOP('',(#32217,#32218,#32219,#32220));
#13323=EDGE_LOOP('',(#32221,#32222,#32223,#32224));
#13324=EDGE_LOOP('',(#32225,#32226,#32227,#32228));
#13325=EDGE_LOOP('',(#32229,#32230,#32231,#32232,#32233,#32234));
#13326=EDGE_LOOP('',(#32235,#32236,#32237,#32238));
#13327=EDGE_LOOP('',(#32239,#32240,#32241,#32242));
#13328=EDGE_LOOP('',(#32243,#32244,#32245,#32246));
#13329=EDGE_LOOP('',(#32247,#32248,#32249,#32250));
#13330=EDGE_LOOP('',(#32251,#32252,#32253,#32254));
#13331=EDGE_LOOP('',(#32255,#32256,#32257,#32258));
#13332=EDGE_LOOP('',(#32259,#32260,#32261,#32262));
#13333=EDGE_LOOP('',(#32263,#32264,#32265,#32266));
#13334=EDGE_LOOP('',(#32267,#32268,#32269,#32270));
#13335=EDGE_LOOP('',(#32271,#32272,#32273,#32274));
#13336=EDGE_LOOP('',(#32275,#32276,#32277,#32278));
#13337=EDGE_LOOP('',(#32279,#32280,#32281,#32282));
#13338=EDGE_LOOP('',(#32283,#32284,#32285,#32286));
#13339=EDGE_LOOP('',(#32287,#32288,#32289,#32290));
#13340=EDGE_LOOP('',(#32291,#32292,#32293,#32294));
#13341=EDGE_LOOP('',(#32295,#32296,#32297,#32298,#32299,#32300));
#13342=EDGE_LOOP('',(#32301,#32302,#32303,#32304));
#13343=EDGE_LOOP('',(#32305,#32306,#32307,#32308));
#13344=EDGE_LOOP('',(#32309,#32310,#32311,#32312));
#13345=EDGE_LOOP('',(#32313,#32314,#32315,#32316));
#13346=EDGE_LOOP('',(#32317,#32318,#32319,#32320));
#13347=EDGE_LOOP('',(#32321,#32322,#32323,#32324));
#13348=EDGE_LOOP('',(#32325,#32326,#32327,#32328));
#13349=EDGE_LOOP('',(#32329,#32330,#32331,#32332));
#13350=EDGE_LOOP('',(#32333,#32334,#32335,#32336));
#13351=EDGE_LOOP('',(#32337,#32338,#32339,#32340));
#13352=EDGE_LOOP('',(#32341,#32342,#32343,#32344));
#13353=EDGE_LOOP('',(#32345,#32346,#32347,#32348));
#13354=EDGE_LOOP('',(#32349,#32350,#32351,#32352));
#13355=EDGE_LOOP('',(#32353,#32354,#32355,#32356));
#13356=EDGE_LOOP('',(#32357,#32358,#32359,#32360));
#13357=EDGE_LOOP('',(#32361,#32362,#32363,#32364));
#13358=EDGE_LOOP('',(#32365,#32366,#32367,#32368));
#13359=EDGE_LOOP('',(#32369,#32370,#32371,#32372,#32373,#32374));
#13360=EDGE_LOOP('',(#32375,#32376,#32377,#32378));
#13361=EDGE_LOOP('',(#32379,#32380,#32381,#32382));
#13362=EDGE_LOOP('',(#32383,#32384,#32385,#32386));
#13363=EDGE_LOOP('',(#32387,#32388,#32389,#32390));
#13364=EDGE_LOOP('',(#32391,#32392,#32393,#32394));
#13365=EDGE_LOOP('',(#32395,#32396,#32397,#32398));
#13366=EDGE_LOOP('',(#32399,#32400,#32401,#32402));
#13367=EDGE_LOOP('',(#32403,#32404,#32405,#32406));
#13368=EDGE_LOOP('',(#32407,#32408,#32409,#32410));
#13369=EDGE_LOOP('',(#32411,#32412,#32413,#32414));
#13370=EDGE_LOOP('',(#32415,#32416,#32417,#32418));
#13371=EDGE_LOOP('',(#32419,#32420,#32421,#32422));
#13372=EDGE_LOOP('',(#32423,#32424,#32425,#32426));
#13373=EDGE_LOOP('',(#32427,#32428,#32429,#32430));
#13374=EDGE_LOOP('',(#32431,#32432,#32433,#32434));
#13375=EDGE_LOOP('',(#32435,#32436,#32437,#32438,#32439,#32440));
#13376=EDGE_LOOP('',(#32441,#32442,#32443,#32444));
#13377=EDGE_LOOP('',(#32445,#32446,#32447,#32448,#32449,#32450));
#13378=EDGE_LOOP('',(#32451,#32452,#32453,#32454));
#13379=EDGE_LOOP('',(#32455,#32456,#32457,#32458));
#13380=EDGE_LOOP('',(#32459,#32460,#32461,#32462));
#13381=EDGE_LOOP('',(#32463,#32464,#32465,#32466));
#13382=EDGE_LOOP('',(#32467,#32468,#32469,#32470));
#13383=EDGE_LOOP('',(#32471,#32472,#32473,#32474));
#13384=EDGE_LOOP('',(#32475,#32476,#32477,#32478));
#13385=EDGE_LOOP('',(#32479,#32480,#32481,#32482));
#13386=EDGE_LOOP('',(#32483,#32484,#32485,#32486));
#13387=EDGE_LOOP('',(#32487,#32488,#32489,#32490));
#13388=EDGE_LOOP('',(#32491,#32492,#32493,#32494));
#13389=EDGE_LOOP('',(#32495,#32496,#32497,#32498));
#13390=EDGE_LOOP('',(#32499,#32500,#32501,#32502));
#13391=EDGE_LOOP('',(#32503,#32504,#32505,#32506,#32507,#32508));
#13392=EDGE_LOOP('',(#32509,#32510,#32511,#32512));
#13393=EDGE_LOOP('',(#32513,#32514,#32515,#32516));
#13394=EDGE_LOOP('',(#32517,#32518,#32519,#32520));
#13395=EDGE_LOOP('',(#32521,#32522,#32523,#32524));
#13396=EDGE_LOOP('',(#32525,#32526,#32527,#32528));
#13397=EDGE_LOOP('',(#32529,#32530,#32531,#32532));
#13398=EDGE_LOOP('',(#32533,#32534,#32535,#32536));
#13399=EDGE_LOOP('',(#32537,#32538,#32539,#32540));
#13400=EDGE_LOOP('',(#32541,#32542,#32543,#32544));
#13401=EDGE_LOOP('',(#32545,#32546,#32547,#32548));
#13402=EDGE_LOOP('',(#32549,#32550,#32551,#32552));
#13403=EDGE_LOOP('',(#32553,#32554,#32555,#32556));
#13404=EDGE_LOOP('',(#32557,#32558,#32559,#32560));
#13405=EDGE_LOOP('',(#32561,#32562,#32563,#32564));
#13406=EDGE_LOOP('',(#32565,#32566,#32567,#32568));
#13407=EDGE_LOOP('',(#32569,#32570,#32571,#32572));
#13408=EDGE_LOOP('',(#32573,#32574,#32575,#32576));
#13409=EDGE_LOOP('',(#32577,#32578,#32579,#32580));
#13410=EDGE_LOOP('',(#32581,#32582,#32583,#32584));
#13411=EDGE_LOOP('',(#32585,#32586,#32587,#32588));
#13412=EDGE_LOOP('',(#32589,#32590,#32591,#32592));
#13413=EDGE_LOOP('',(#32593,#32594,#32595,#32596));
#13414=EDGE_LOOP('',(#32597,#32598,#32599,#32600));
#13415=EDGE_LOOP('',(#32601,#32602,#32603,#32604));
#13416=EDGE_LOOP('',(#32605,#32606,#32607,#32608));
#13417=EDGE_LOOP('',(#32609,#32610,#32611,#32612));
#13418=EDGE_LOOP('',(#32613,#32614,#32615,#32616));
#13419=EDGE_LOOP('',(#32617,#32618,#32619,#32620,#32621,#32622));
#13420=EDGE_LOOP('',(#32623,#32624,#32625,#32626));
#13421=EDGE_LOOP('',(#32627,#32628,#32629,#32630));
#13422=EDGE_LOOP('',(#32631,#32632,#32633,#32634));
#13423=EDGE_LOOP('',(#32635,#32636,#32637,#32638));
#13424=EDGE_LOOP('',(#32639,#32640,#32641,#32642));
#13425=EDGE_LOOP('',(#32643,#32644,#32645,#32646));
#13426=EDGE_LOOP('',(#32647,#32648,#32649,#32650));
#13427=EDGE_LOOP('',(#32651,#32652,#32653,#32654));
#13428=EDGE_LOOP('',(#32655,#32656,#32657,#32658));
#13429=EDGE_LOOP('',(#32659,#32660,#32661,#32662));
#13430=EDGE_LOOP('',(#32663,#32664,#32665,#32666));
#13431=EDGE_LOOP('',(#32667,#32668,#32669,#32670));
#13432=EDGE_LOOP('',(#32671,#32672,#32673,#32674));
#13433=EDGE_LOOP('',(#32675,#32676,#32677,#32678));
#13434=EDGE_LOOP('',(#32679,#32680,#32681,#32682));
#13435=EDGE_LOOP('',(#32683,#32684,#32685,#32686));
#13436=EDGE_LOOP('',(#32687,#32688,#32689,#32690));
#13437=EDGE_LOOP('',(#32691,#32692,#32693,#32694));
#13438=EDGE_LOOP('',(#32695,#32696,#32697,#32698));
#13439=EDGE_LOOP('',(#32699,#32700,#32701,#32702));
#13440=EDGE_LOOP('',(#32703,#32704,#32705,#32706));
#13441=EDGE_LOOP('',(#32707,#32708,#32709,#32710));
#13442=EDGE_LOOP('',(#32711,#32712,#32713,#32714));
#13443=EDGE_LOOP('',(#32715,#32716,#32717,#32718));
#13444=EDGE_LOOP('',(#32719,#32720,#32721,#32722));
#13445=EDGE_LOOP('',(#32723,#32724,#32725,#32726));
#13446=EDGE_LOOP('',(#32727,#32728,#32729,#32730));
#13447=EDGE_LOOP('',(#32731,#32732,#32733,#32734));
#13448=EDGE_LOOP('',(#32735,#32736,#32737,#32738));
#13449=EDGE_LOOP('',(#32739,#32740,#32741,#32742));
#13450=EDGE_LOOP('',(#32743,#32744,#32745,#32746));
#13451=EDGE_LOOP('',(#32747,#32748,#32749,#32750));
#13452=EDGE_LOOP('',(#32751,#32752,#32753,#32754));
#13453=EDGE_LOOP('',(#32755,#32756,#32757,#32758,#32759,#32760,#32761));
#13454=EDGE_LOOP('',(#32762,#32763,#32764,#32765));
#13455=EDGE_LOOP('',(#32766,#32767,#32768,#32769));
#13456=EDGE_LOOP('',(#32770,#32771,#32772,#32773));
#13457=EDGE_LOOP('',(#32774,#32775,#32776,#32777));
#13458=EDGE_LOOP('',(#32778,#32779,#32780,#32781));
#13459=EDGE_LOOP('',(#32782,#32783,#32784,#32785));
#13460=EDGE_LOOP('',(#32786,#32787,#32788,#32789));
#13461=EDGE_LOOP('',(#32790,#32791,#32792,#32793));
#13462=EDGE_LOOP('',(#32794,#32795,#32796,#32797));
#13463=EDGE_LOOP('',(#32798,#32799,#32800,#32801));
#13464=EDGE_LOOP('',(#32802,#32803,#32804,#32805));
#13465=EDGE_LOOP('',(#32806,#32807,#32808,#32809));
#13466=EDGE_LOOP('',(#32810,#32811,#32812,#32813));
#13467=EDGE_LOOP('',(#32814,#32815,#32816,#32817));
#13468=EDGE_LOOP('',(#32818,#32819,#32820,#32821));
#13469=EDGE_LOOP('',(#32822,#32823,#32824,#32825));
#13470=EDGE_LOOP('',(#32826,#32827,#32828,#32829));
#13471=EDGE_LOOP('',(#32830,#32831,#32832,#32833,#32834,#32835));
#13472=EDGE_LOOP('',(#32836,#32837,#32838,#32839));
#13473=EDGE_LOOP('',(#32840,#32841,#32842,#32843));
#13474=EDGE_LOOP('',(#32844,#32845,#32846,#32847));
#13475=EDGE_LOOP('',(#32848,#32849,#32850,#32851));
#13476=EDGE_LOOP('',(#32852,#32853,#32854,#32855));
#13477=EDGE_LOOP('',(#32856,#32857,#32858,#32859));
#13478=EDGE_LOOP('',(#32860,#32861,#32862,#32863));
#13479=EDGE_LOOP('',(#32864,#32865,#32866,#32867));
#13480=EDGE_LOOP('',(#32868,#32869,#32870,#32871));
#13481=EDGE_LOOP('',(#32872,#32873,#32874,#32875));
#13482=EDGE_LOOP('',(#32876,#32877,#32878,#32879));
#13483=EDGE_LOOP('',(#32880,#32881,#32882,#32883));
#13484=EDGE_LOOP('',(#32884,#32885,#32886,#32887));
#13485=EDGE_LOOP('',(#32888,#32889,#32890,#32891));
#13486=EDGE_LOOP('',(#32892,#32893,#32894,#32895));
#13487=EDGE_LOOP('',(#32896,#32897,#32898,#32899));
#13488=EDGE_LOOP('',(#32900,#32901,#32902,#32903));
#13489=EDGE_LOOP('',(#32904,#32905,#32906,#32907,#32908,#32909));
#13490=EDGE_LOOP('',(#32910,#32911,#32912,#32913));
#13491=EDGE_LOOP('',(#32914,#32915,#32916,#32917));
#13492=EDGE_LOOP('',(#32918,#32919,#32920,#32921));
#13493=EDGE_LOOP('',(#32922,#32923,#32924,#32925));
#13494=EDGE_LOOP('',(#32926,#32927,#32928,#32929));
#13495=EDGE_LOOP('',(#32930,#32931,#32932,#32933));
#13496=EDGE_LOOP('',(#32934,#32935,#32936,#32937));
#13497=EDGE_LOOP('',(#32938,#32939,#32940,#32941));
#13498=EDGE_LOOP('',(#32942,#32943,#32944,#32945));
#13499=EDGE_LOOP('',(#32946,#32947,#32948,#32949));
#13500=EDGE_LOOP('',(#32950,#32951,#32952,#32953));
#13501=EDGE_LOOP('',(#32954,#32955,#32956,#32957));
#13502=EDGE_LOOP('',(#32958,#32959,#32960,#32961));
#13503=EDGE_LOOP('',(#32962,#32963,#32964,#32965));
#13504=EDGE_LOOP('',(#32966,#32967,#32968,#32969));
#13505=EDGE_LOOP('',(#32970,#32971,#32972,#32973,#32974,#32975));
#13506=EDGE_LOOP('',(#32976,#32977,#32978,#32979));
#13507=EDGE_LOOP('',(#32980,#32981,#32982,#32983));
#13508=EDGE_LOOP('',(#32984,#32985,#32986,#32987));
#13509=EDGE_LOOP('',(#32988,#32989,#32990,#32991));
#13510=EDGE_LOOP('',(#32992,#32993,#32994,#32995));
#13511=EDGE_LOOP('',(#32996,#32997,#32998,#32999));
#13512=EDGE_LOOP('',(#33000,#33001,#33002,#33003));
#13513=EDGE_LOOP('',(#33004,#33005,#33006,#33007));
#13514=EDGE_LOOP('',(#33008,#33009,#33010,#33011));
#13515=EDGE_LOOP('',(#33012,#33013,#33014,#33015));
#13516=EDGE_LOOP('',(#33016,#33017,#33018,#33019));
#13517=EDGE_LOOP('',(#33020,#33021,#33022,#33023));
#13518=EDGE_LOOP('',(#33024,#33025,#33026,#33027));
#13519=EDGE_LOOP('',(#33028,#33029,#33030,#33031));
#13520=EDGE_LOOP('',(#33032,#33033,#33034,#33035));
#13521=EDGE_LOOP('',(#33036,#33037,#33038,#33039));
#13522=EDGE_LOOP('',(#33040,#33041,#33042,#33043));
#13523=EDGE_LOOP('',(#33044,#33045,#33046,#33047,#33048,#33049));
#13524=EDGE_LOOP('',(#33050,#33051,#33052,#33053));
#13525=EDGE_LOOP('',(#33054,#33055,#33056,#33057));
#13526=EDGE_LOOP('',(#33058,#33059,#33060,#33061));
#13527=EDGE_LOOP('',(#33062,#33063,#33064,#33065));
#13528=EDGE_LOOP('',(#33066,#33067,#33068,#33069));
#13529=EDGE_LOOP('',(#33070,#33071,#33072,#33073));
#13530=EDGE_LOOP('',(#33074,#33075,#33076,#33077));
#13531=EDGE_LOOP('',(#33078,#33079,#33080,#33081));
#13532=EDGE_LOOP('',(#33082,#33083,#33084,#33085));
#13533=EDGE_LOOP('',(#33086,#33087,#33088,#33089));
#13534=EDGE_LOOP('',(#33090,#33091,#33092,#33093));
#13535=EDGE_LOOP('',(#33094,#33095,#33096,#33097));
#13536=EDGE_LOOP('',(#33098,#33099,#33100,#33101));
#13537=EDGE_LOOP('',(#33102,#33103,#33104,#33105));
#13538=EDGE_LOOP('',(#33106,#33107,#33108,#33109));
#13539=EDGE_LOOP('',(#33110,#33111,#33112,#33113));
#13540=EDGE_LOOP('',(#33114,#33115,#33116,#33117));
#13541=EDGE_LOOP('',(#33118,#33119,#33120,#33121,#33122,#33123));
#13542=EDGE_LOOP('',(#33124,#33125,#33126,#33127));
#13543=EDGE_LOOP('',(#33128,#33129,#33130,#33131,#33132,#33133,#33134,#33135,
#33136,#33137,#33138,#33139,#33140,#33141,#33142,#33143,#33144,#33145,#33146,
#33147,#33148,#33149,#33150,#33151,#33152,#33153,#33154,#33155,#33156,#33157,
#33158,#33159,#33160,#33161,#33162,#33163,#33164,#33165,#33166,#33167,#33168,
#33169,#33170,#33171,#33172,#33173,#33174,#33175,#33176,#33177,#33178,#33179,
#33180,#33181,#33182,#33183,#33184,#33185,#33186,#33187,#33188,#33189,#33190,
#33191,#33192,#33193,#33194,#33195,#33196,#33197,#33198,#33199,#33200,#33201,
#33202));
#13544=EDGE_LOOP('',(#33203));
#13545=EDGE_LOOP('',(#33204));
#13546=EDGE_LOOP('',(#33205));
#13547=EDGE_LOOP('',(#33206));
#13548=EDGE_LOOP('',(#33207));
#13549=EDGE_LOOP('',(#33208));
#13550=EDGE_LOOP('',(#33209));
#13551=EDGE_LOOP('',(#33210));
#13552=EDGE_LOOP('',(#33211));
#13553=EDGE_LOOP('',(#33212,#33213));
#13554=EDGE_LOOP('',(#33214));
#13555=EDGE_LOOP('',(#33215));
#13556=EDGE_LOOP('',(#33216));
#13557=EDGE_LOOP('',(#33217));
#13558=EDGE_LOOP('',(#33218));
#13559=EDGE_LOOP('',(#33219));
#13560=EDGE_LOOP('',(#33220));
#13561=EDGE_LOOP('',(#33221));
#13562=EDGE_LOOP('',(#33222));
#13563=EDGE_LOOP('',(#33223));
#13564=EDGE_LOOP('',(#33224));
#13565=EDGE_LOOP('',(#33225));
#13566=EDGE_LOOP('',(#33226));
#13567=EDGE_LOOP('',(#33227));
#13568=EDGE_LOOP('',(#33228));
#13569=EDGE_LOOP('',(#33229));
#13570=EDGE_LOOP('',(#33230));
#13571=EDGE_LOOP('',(#33231));
#13572=EDGE_LOOP('',(#33232));
#13573=EDGE_LOOP('',(#33233));
#13574=EDGE_LOOP('',(#33234));
#13575=EDGE_LOOP('',(#33235));
#13576=EDGE_LOOP('',(#33236));
#13577=EDGE_LOOP('',(#33237));
#13578=EDGE_LOOP('',(#33238));
#13579=EDGE_LOOP('',(#33239));
#13580=EDGE_LOOP('',(#33240));
#13581=EDGE_LOOP('',(#33241));
#13582=EDGE_LOOP('',(#33242));
#13583=EDGE_LOOP('',(#33243));
#13584=EDGE_LOOP('',(#33244));
#13585=EDGE_LOOP('',(#33245));
#13586=EDGE_LOOP('',(#33246));
#13587=EDGE_LOOP('',(#33247));
#13588=EDGE_LOOP('',(#33248));
#13589=EDGE_LOOP('',(#33249));
#13590=EDGE_LOOP('',(#33250));
#13591=EDGE_LOOP('',(#33251));
#13592=EDGE_LOOP('',(#33252,#33253,#33254,#33255,#33256,#33257,#33258,#33259,
#33260));
#13593=EDGE_LOOP('',(#33261,#33262,#33263,#33264,#33265));
#13594=EDGE_LOOP('',(#33266,#33267,#33268,#33269));
#13595=EDGE_LOOP('',(#33270,#33271,#33272,#33273,#33274,#33275));
#13596=EDGE_LOOP('',(#33276,#33277,#33278,#33279));
#13597=EDGE_LOOP('',(#33280,#33281,#33282,#33283));
#13598=EDGE_LOOP('',(#33284,#33285,#33286,#33287,#33288));
#13599=EDGE_LOOP('',(#33289,#33290,#33291,#33292,#33293));
#13600=EDGE_LOOP('',(#33294,#33295,#33296,#33297,#33298,#33299));
#13601=EDGE_LOOP('',(#33300,#33301,#33302,#33303,#33304));
#13602=EDGE_LOOP('',(#33305,#33306,#33307,#33308));
#13603=EDGE_LOOP('',(#33309,#33310,#33311,#33312,#33313,#33314));
#13604=EDGE_LOOP('',(#33315,#33316));
#13605=EDGE_LOOP('',(#33317));
#13606=EDGE_LOOP('',(#33318));
#13607=EDGE_LOOP('',(#33319));
#13608=EDGE_LOOP('',(#33320,#33321,#33322,#33323,#33324,#33325));
#13609=EDGE_LOOP('',(#33326,#33327,#33328));
#13610=EDGE_LOOP('',(#33329,#33330,#33331,#33332));
#13611=EDGE_LOOP('',(#33333,#33334,#33335,#33336,#33337,#33338));
#13612=EDGE_LOOP('',(#33339,#33340,#33341));
#13613=EDGE_LOOP('',(#33342,#33343,#33344,#33345,#33346,#33347));
#13614=EDGE_LOOP('',(#33348,#33349,#33350,#33351));
#13615=EDGE_LOOP('',(#33352,#33353,#33354,#33355));
#13616=EDGE_LOOP('',(#33356,#33357,#33358,#33359));
#13617=EDGE_LOOP('',(#33360,#33361,#33362,#33363,#33364,#33365,#33366,#33367));
#13618=EDGE_LOOP('',(#33368,#33369,#33370,#33371));
#13619=EDGE_LOOP('',(#33372,#33373,#33374,#33375));
#13620=EDGE_LOOP('',(#33376,#33377,#33378,#33379));
#13621=EDGE_LOOP('',(#33380,#33381,#33382,#33383));
#13622=EDGE_LOOP('',(#33384,#33385,#33386,#33387));
#13623=EDGE_LOOP('',(#33388,#33389,#33390,#33391));
#13624=EDGE_LOOP('',(#33392,#33393,#33394,#33395));
#13625=EDGE_LOOP('',(#33396,#33397,#33398,#33399));
#13626=EDGE_LOOP('',(#33400,#33401,#33402,#33403));
#13627=EDGE_LOOP('',(#33404,#33405,#33406,#33407,#33408));
#13628=EDGE_LOOP('',(#33409,#33410,#33411,#33412));
#13629=EDGE_LOOP('',(#33413,#33414,#33415,#33416));
#13630=EDGE_LOOP('',(#33417,#33418,#33419,#33420,#33421));
#13631=EDGE_LOOP('',(#33422,#33423,#33424,#33425));
#13632=EDGE_LOOP('',(#33426,#33427));
#13633=EDGE_LOOP('',(#33428,#33429,#33430,#33431,#33432));
#13634=EDGE_LOOP('',(#33433,#33434,#33435,#33436,#33437,#33438));
#13635=EDGE_LOOP('',(#33439,#33440,#33441,#33442));
#13636=EDGE_LOOP('',(#33443,#33444,#33445,#33446,#33447));
#13637=EDGE_LOOP('',(#33448,#33449,#33450,#33451));
#13638=EDGE_LOOP('',(#33452,#33453,#33454,#33455));
#13639=EDGE_LOOP('',(#33456,#33457,#33458,#33459));
#13640=EDGE_LOOP('',(#33460,#33461,#33462,#33463));
#13641=EDGE_LOOP('',(#33464,#33465,#33466,#33467,#33468));
#13642=EDGE_LOOP('',(#33469,#33470,#33471,#33472));
#13643=EDGE_LOOP('',(#33473,#33474,#33475,#33476));
#13644=EDGE_LOOP('',(#33477,#33478,#33479,#33480));
#13645=EDGE_LOOP('',(#33481,#33482,#33483,#33484));
#13646=EDGE_LOOP('',(#33485,#33486,#33487,#33488,#33489,#33490));
#13647=EDGE_LOOP('',(#33491,#33492,#33493,#33494,#33495));
#13648=EDGE_LOOP('',(#33496,#33497,#33498,#33499,#33500));
#13649=EDGE_LOOP('',(#33501,#33502,#33503,#33504,#33505));
#13650=EDGE_LOOP('',(#33506,#33507,#33508,#33509,#33510));
#13651=EDGE_LOOP('',(#33511,#33512));
#13652=EDGE_LOOP('',(#33513,#33514,#33515,#33516,#33517,#33518));
#13653=EDGE_LOOP('',(#33519,#33520,#33521,#33522));
#13654=EDGE_LOOP('',(#33523,#33524,#33525,#33526));
#13655=EDGE_LOOP('',(#33527,#33528,#33529,#33530));
#13656=EDGE_LOOP('',(#33531,#33532,#33533,#33534));
#13657=EDGE_LOOP('',(#33535,#33536,#33537,#33538));
#13658=EDGE_LOOP('',(#33539,#33540,#33541,#33542));
#13659=EDGE_LOOP('',(#33543,#33544,#33545,#33546));
#13660=EDGE_LOOP('',(#33547,#33548,#33549,#33550,#33551,#33552,#33553,#33554));
#13661=EDGE_LOOP('',(#33555,#33556,#33557,#33558));
#13662=EDGE_LOOP('',(#33559,#33560,#33561,#33562));
#13663=EDGE_LOOP('',(#33563,#33564,#33565,#33566));
#13664=EDGE_LOOP('',(#33567,#33568,#33569,#33570));
#13665=EDGE_LOOP('',(#33571,#33572,#33573,#33574));
#13666=EDGE_LOOP('',(#33575,#33576,#33577,#33578,#33579,#33580,#33581,#33582));
#13667=EDGE_LOOP('',(#33583,#33584,#33585,#33586,#33587,#33588,#33589,#33590));
#13668=EDGE_LOOP('',(#33591,#33592,#33593,#33594,#33595,#33596,#33597,#33598));
#13669=EDGE_LOOP('',(#33599,#33600,#33601,#33602,#33603,#33604,#33605,#33606,
#33607,#33608,#33609,#33610,#33611));
#13670=EDGE_LOOP('',(#33612));
#13671=EDGE_LOOP('',(#33613));
#13672=EDGE_LOOP('',(#33614));
#13673=EDGE_LOOP('',(#33615));
#13674=EDGE_LOOP('',(#33616));
#13675=EDGE_LOOP('',(#33617));
#13676=EDGE_LOOP('',(#33618));
#13677=EDGE_LOOP('',(#33619));
#13678=EDGE_LOOP('',(#33620));
#13679=EDGE_LOOP('',(#33621));
#13680=EDGE_LOOP('',(#33622));
#13681=EDGE_LOOP('',(#33623));
#13682=EDGE_LOOP('',(#33624));
#13683=EDGE_LOOP('',(#33625));
#13684=EDGE_LOOP('',(#33626));
#13685=EDGE_LOOP('',(#33627));
#13686=EDGE_LOOP('',(#33628));
#13687=EDGE_LOOP('',(#33629));
#13688=EDGE_LOOP('',(#33630,#33631,#33632,#33633,#33634,#33635,#33636,#33637,
#33638,#33639,#33640,#33641,#33642,#33643,#33644,#33645,#33646,#33647,#33648,
#33649,#33650,#33651,#33652,#33653,#33654,#33655,#33656,#33657,#33658,#33659,
#33660,#33661,#33662,#33663,#33664,#33665,#33666,#33667,#33668,#33669,#33670,
#33671,#33672,#33673,#33674,#33675,#33676,#33677,#33678,#33679,#33680,#33681,
#33682,#33683,#33684,#33685,#33686,#33687,#33688,#33689,#33690,#33691,#33692,
#33693,#33694,#33695));
#13689=EDGE_LOOP('',(#33696));
#13690=EDGE_LOOP('',(#33697));
#13691=EDGE_LOOP('',(#33698));
#13692=EDGE_LOOP('',(#33699));
#13693=EDGE_LOOP('',(#33700));
#13694=EDGE_LOOP('',(#33701));
#13695=EDGE_LOOP('',(#33702));
#13696=EDGE_LOOP('',(#33703));
#13697=EDGE_LOOP('',(#33704));
#13698=EDGE_LOOP('',(#33705));
#13699=EDGE_LOOP('',(#33706));
#13700=EDGE_LOOP('',(#33707));
#13701=EDGE_LOOP('',(#33708));
#13702=EDGE_LOOP('',(#33709));
#13703=EDGE_LOOP('',(#33710));
#13704=EDGE_LOOP('',(#33711));
#13705=EDGE_LOOP('',(#33712));
#13706=EDGE_LOOP('',(#33713));
#13707=EDGE_LOOP('',(#33714));
#13708=EDGE_LOOP('',(#33715));
#13709=EDGE_LOOP('',(#33716));
#13710=EDGE_LOOP('',(#33717));
#13711=EDGE_LOOP('',(#33718));
#13712=EDGE_LOOP('',(#33719));
#13713=EDGE_LOOP('',(#33720));
#13714=EDGE_LOOP('',(#33721));
#13715=EDGE_LOOP('',(#33722));
#13716=EDGE_LOOP('',(#33723));
#13717=EDGE_LOOP('',(#33724));
#13718=EDGE_LOOP('',(#33725));
#13719=EDGE_LOOP('',(#33726));
#13720=EDGE_LOOP('',(#33727));
#13721=EDGE_LOOP('',(#33728));
#13722=EDGE_LOOP('',(#33729));
#13723=EDGE_LOOP('',(#33730));
#13724=EDGE_LOOP('',(#33731));
#13725=EDGE_LOOP('',(#33732));
#13726=EDGE_LOOP('',(#33733));
#13727=EDGE_LOOP('',(#33734));
#13728=EDGE_LOOP('',(#33735));
#13729=EDGE_LOOP('',(#33736));
#13730=EDGE_LOOP('',(#33737));
#13731=EDGE_LOOP('',(#33738));
#13732=EDGE_LOOP('',(#33739));
#13733=EDGE_LOOP('',(#33740));
#13734=EDGE_LOOP('',(#33741));
#13735=EDGE_LOOP('',(#33742));
#13736=EDGE_LOOP('',(#33743));
#13737=EDGE_LOOP('',(#33744));
#13738=EDGE_LOOP('',(#33745));
#13739=EDGE_LOOP('',(#33746));
#13740=EDGE_LOOP('',(#33747));
#13741=EDGE_LOOP('',(#33748));
#13742=EDGE_LOOP('',(#33749));
#13743=EDGE_LOOP('',(#33750));
#13744=EDGE_LOOP('',(#33751));
#13745=EDGE_LOOP('',(#33752));
#13746=EDGE_LOOP('',(#33753));
#13747=EDGE_LOOP('',(#33754));
#13748=EDGE_LOOP('',(#33755));
#13749=EDGE_LOOP('',(#33756));
#13750=EDGE_LOOP('',(#33757));
#13751=EDGE_LOOP('',(#33758));
#13752=EDGE_LOOP('',(#33759));
#13753=EDGE_LOOP('',(#33760));
#13754=EDGE_LOOP('',(#33761));
#13755=EDGE_LOOP('',(#33762));
#13756=EDGE_LOOP('',(#33763));
#13757=EDGE_LOOP('',(#33764));
#13758=EDGE_LOOP('',(#33765));
#13759=EDGE_LOOP('',(#33766));
#13760=EDGE_LOOP('',(#33767));
#13761=EDGE_LOOP('',(#33768));
#13762=EDGE_LOOP('',(#33769));
#13763=EDGE_LOOP('',(#33770));
#13764=EDGE_LOOP('',(#33771));
#13765=EDGE_LOOP('',(#33772));
#13766=EDGE_LOOP('',(#33773));
#13767=EDGE_LOOP('',(#33774));
#13768=EDGE_LOOP('',(#33775));
#13769=EDGE_LOOP('',(#33776));
#13770=EDGE_LOOP('',(#33777));
#13771=EDGE_LOOP('',(#33778));
#13772=EDGE_LOOP('',(#33779));
#13773=EDGE_LOOP('',(#33780));
#13774=EDGE_LOOP('',(#33781));
#13775=EDGE_LOOP('',(#33782));
#13776=EDGE_LOOP('',(#33783));
#13777=EDGE_LOOP('',(#33784));
#13778=EDGE_LOOP('',(#33785));
#13779=EDGE_LOOP('',(#33786));
#13780=EDGE_LOOP('',(#33787));
#13781=EDGE_LOOP('',(#33788));
#13782=EDGE_LOOP('',(#33789));
#13783=EDGE_LOOP('',(#33790));
#13784=EDGE_LOOP('',(#33791));
#13785=EDGE_LOOP('',(#33792));
#13786=EDGE_LOOP('',(#33793));
#13787=EDGE_LOOP('',(#33794));
#13788=EDGE_LOOP('',(#33795));
#13789=EDGE_LOOP('',(#33796));
#13790=EDGE_LOOP('',(#33797));
#13791=EDGE_LOOP('',(#33798));
#13792=EDGE_LOOP('',(#33799));
#13793=EDGE_LOOP('',(#33800));
#13794=EDGE_LOOP('',(#33801));
#13795=EDGE_LOOP('',(#33802));
#13796=EDGE_LOOP('',(#33803));
#13797=EDGE_LOOP('',(#33804));
#13798=EDGE_LOOP('',(#33805));
#13799=EDGE_LOOP('',(#33806));
#13800=EDGE_LOOP('',(#33807));
#13801=EDGE_LOOP('',(#33808));
#13802=EDGE_LOOP('',(#33809));
#13803=EDGE_LOOP('',(#33810));
#13804=EDGE_LOOP('',(#33811));
#13805=EDGE_LOOP('',(#33812));
#13806=EDGE_LOOP('',(#33813));
#13807=EDGE_LOOP('',(#33814));
#13808=EDGE_LOOP('',(#33815));
#13809=EDGE_LOOP('',(#33816));
#13810=EDGE_LOOP('',(#33817));
#13811=EDGE_LOOP('',(#33818));
#13812=EDGE_LOOP('',(#33819));
#13813=EDGE_LOOP('',(#33820));
#13814=EDGE_LOOP('',(#33821));
#13815=EDGE_LOOP('',(#33822));
#13816=EDGE_LOOP('',(#33823));
#13817=EDGE_LOOP('',(#33824));
#13818=EDGE_LOOP('',(#33825));
#13819=EDGE_LOOP('',(#33826));
#13820=EDGE_LOOP('',(#33827));
#13821=EDGE_LOOP('',(#33828));
#13822=EDGE_LOOP('',(#33829));
#13823=EDGE_LOOP('',(#33830));
#13824=EDGE_LOOP('',(#33831));
#13825=EDGE_LOOP('',(#33832));
#13826=EDGE_LOOP('',(#33833));
#13827=EDGE_LOOP('',(#33834));
#13828=EDGE_LOOP('',(#33835));
#13829=EDGE_LOOP('',(#33836));
#13830=EDGE_LOOP('',(#33837));
#13831=EDGE_LOOP('',(#33838));
#13832=EDGE_LOOP('',(#33839));
#13833=EDGE_LOOP('',(#33840));
#13834=EDGE_LOOP('',(#33841));
#13835=EDGE_LOOP('',(#33842));
#13836=EDGE_LOOP('',(#33843));
#13837=EDGE_LOOP('',(#33844));
#13838=EDGE_LOOP('',(#33845));
#13839=EDGE_LOOP('',(#33846));
#13840=EDGE_LOOP('',(#33847));
#13841=EDGE_LOOP('',(#33848));
#13842=EDGE_LOOP('',(#33849));
#13843=EDGE_LOOP('',(#33850));
#13844=EDGE_LOOP('',(#33851));
#13845=EDGE_LOOP('',(#33852));
#13846=EDGE_LOOP('',(#33853));
#13847=EDGE_LOOP('',(#33854));
#13848=EDGE_LOOP('',(#33855));
#13849=EDGE_LOOP('',(#33856));
#13850=EDGE_LOOP('',(#33857));
#13851=EDGE_LOOP('',(#33858));
#13852=EDGE_LOOP('',(#33859));
#13853=EDGE_LOOP('',(#33860));
#13854=EDGE_LOOP('',(#33861));
#13855=EDGE_LOOP('',(#33862));
#13856=EDGE_LOOP('',(#33863));
#13857=EDGE_LOOP('',(#33864));
#13858=EDGE_LOOP('',(#33865));
#13859=EDGE_LOOP('',(#33866));
#13860=EDGE_LOOP('',(#33867));
#13861=EDGE_LOOP('',(#33868));
#13862=EDGE_LOOP('',(#33869));
#13863=EDGE_LOOP('',(#33870));
#13864=EDGE_LOOP('',(#33871));
#13865=EDGE_LOOP('',(#33872));
#13866=EDGE_LOOP('',(#33873));
#13867=EDGE_LOOP('',(#33874));
#13868=EDGE_LOOP('',(#33875));
#13869=EDGE_LOOP('',(#33876));
#13870=EDGE_LOOP('',(#33877));
#13871=EDGE_LOOP('',(#33878));
#13872=EDGE_LOOP('',(#33879));
#13873=EDGE_LOOP('',(#33880));
#13874=EDGE_LOOP('',(#33881));
#13875=EDGE_LOOP('',(#33882));
#13876=EDGE_LOOP('',(#33883));
#13877=EDGE_LOOP('',(#33884));
#13878=EDGE_LOOP('',(#33885));
#13879=EDGE_LOOP('',(#33886));
#13880=EDGE_LOOP('',(#33887));
#13881=EDGE_LOOP('',(#33888));
#13882=EDGE_LOOP('',(#33889));
#13883=EDGE_LOOP('',(#33890));
#13884=EDGE_LOOP('',(#33891));
#13885=EDGE_LOOP('',(#33892));
#13886=EDGE_LOOP('',(#33893));
#13887=EDGE_LOOP('',(#33894));
#13888=EDGE_LOOP('',(#33895));
#13889=EDGE_LOOP('',(#33896));
#13890=EDGE_LOOP('',(#33897));
#13891=EDGE_LOOP('',(#33898));
#13892=EDGE_LOOP('',(#33899));
#13893=EDGE_LOOP('',(#33900));
#13894=EDGE_LOOP('',(#33901));
#13895=EDGE_LOOP('',(#33902));
#13896=EDGE_LOOP('',(#33903));
#13897=EDGE_LOOP('',(#33904));
#13898=EDGE_LOOP('',(#33905));
#13899=EDGE_LOOP('',(#33906));
#13900=EDGE_LOOP('',(#33907));
#13901=EDGE_LOOP('',(#33908));
#13902=EDGE_LOOP('',(#33909));
#13903=EDGE_LOOP('',(#33910));
#13904=EDGE_LOOP('',(#33911));
#13905=EDGE_LOOP('',(#33912));
#13906=EDGE_LOOP('',(#33913));
#13907=EDGE_LOOP('',(#33914));
#13908=EDGE_LOOP('',(#33915));
#13909=EDGE_LOOP('',(#33916));
#13910=EDGE_LOOP('',(#33917));
#13911=EDGE_LOOP('',(#33918));
#13912=EDGE_LOOP('',(#33919));
#13913=EDGE_LOOP('',(#33920));
#13914=EDGE_LOOP('',(#33921));
#13915=EDGE_LOOP('',(#33922));
#13916=EDGE_LOOP('',(#33923));
#13917=EDGE_LOOP('',(#33924));
#13918=EDGE_LOOP('',(#33925));
#13919=EDGE_LOOP('',(#33926));
#13920=EDGE_LOOP('',(#33927));
#13921=EDGE_LOOP('',(#33928));
#13922=EDGE_LOOP('',(#33929));
#13923=EDGE_LOOP('',(#33930));
#13924=EDGE_LOOP('',(#33931));
#13925=EDGE_LOOP('',(#33932,#33933,#33934,#33935));
#13926=EDGE_LOOP('',(#33936,#33937,#33938,#33939));
#13927=EDGE_LOOP('',(#33940,#33941,#33942,#33943,#33944,#33945,#33946,#33947,
#33948,#33949,#33950,#33951));
#13928=EDGE_LOOP('',(#33952,#33953,#33954));
#13929=EDGE_LOOP('',(#33955,#33956,#33957));
#13930=EDGE_LOOP('',(#33958,#33959,#33960,#33961));
#13931=EDGE_LOOP('',(#33962));
#13932=EDGE_LOOP('',(#33963));
#13933=EDGE_LOOP('',(#33964));
#13934=EDGE_LOOP('',(#33965));
#13935=EDGE_LOOP('',(#33966));
#13936=EDGE_LOOP('',(#33967));
#13937=EDGE_LOOP('',(#33968));
#13938=EDGE_LOOP('',(#33969));
#13939=EDGE_LOOP('',(#33970));
#13940=EDGE_LOOP('',(#33971));
#13941=EDGE_LOOP('',(#33972));
#13942=EDGE_LOOP('',(#33973));
#13943=EDGE_LOOP('',(#33974));
#13944=EDGE_LOOP('',(#33975));
#13945=EDGE_LOOP('',(#33976));
#13946=EDGE_LOOP('',(#33977));
#13947=EDGE_LOOP('',(#33978));
#13948=EDGE_LOOP('',(#33979));
#13949=EDGE_LOOP('',(#33980));
#13950=EDGE_LOOP('',(#33981));
#13951=EDGE_LOOP('',(#33982));
#13952=EDGE_LOOP('',(#33983));
#13953=EDGE_LOOP('',(#33984));
#13954=EDGE_LOOP('',(#33985));
#13955=EDGE_LOOP('',(#33986));
#13956=EDGE_LOOP('',(#33987));
#13957=EDGE_LOOP('',(#33988));
#13958=EDGE_LOOP('',(#33989));
#13959=EDGE_LOOP('',(#33990));
#13960=EDGE_LOOP('',(#33991));
#13961=EDGE_LOOP('',(#33992));
#13962=EDGE_LOOP('',(#33993));
#13963=EDGE_LOOP('',(#33994));
#13964=EDGE_LOOP('',(#33995));
#13965=EDGE_LOOP('',(#33996));
#13966=EDGE_LOOP('',(#33997));
#13967=EDGE_LOOP('',(#33998));
#13968=EDGE_LOOP('',(#33999));
#13969=EDGE_LOOP('',(#34000));
#13970=EDGE_LOOP('',(#34001));
#13971=EDGE_LOOP('',(#34002));
#13972=EDGE_LOOP('',(#34003));
#13973=EDGE_LOOP('',(#34004));
#13974=EDGE_LOOP('',(#34005));
#13975=EDGE_LOOP('',(#34006));
#13976=EDGE_LOOP('',(#34007));
#13977=EDGE_LOOP('',(#34008));
#13978=EDGE_LOOP('',(#34009));
#13979=EDGE_LOOP('',(#34010));
#13980=EDGE_LOOP('',(#34011));
#13981=EDGE_LOOP('',(#34012));
#13982=EDGE_LOOP('',(#34013));
#13983=EDGE_LOOP('',(#34014));
#13984=EDGE_LOOP('',(#34015));
#13985=EDGE_LOOP('',(#34016));
#13986=EDGE_LOOP('',(#34017));
#13987=EDGE_LOOP('',(#34018));
#13988=EDGE_LOOP('',(#34019));
#13989=EDGE_LOOP('',(#34020));
#13990=EDGE_LOOP('',(#34021));
#13991=EDGE_LOOP('',(#34022));
#13992=EDGE_LOOP('',(#34023));
#13993=EDGE_LOOP('',(#34024));
#13994=EDGE_LOOP('',(#34025));
#13995=EDGE_LOOP('',(#34026));
#13996=EDGE_LOOP('',(#34027));
#13997=EDGE_LOOP('',(#34028));
#13998=EDGE_LOOP('',(#34029));
#13999=EDGE_LOOP('',(#34030));
#14000=EDGE_LOOP('',(#34031));
#14001=EDGE_LOOP('',(#34032));
#14002=EDGE_LOOP('',(#34033));
#14003=EDGE_LOOP('',(#34034));
#14004=EDGE_LOOP('',(#34035));
#14005=EDGE_LOOP('',(#34036));
#14006=EDGE_LOOP('',(#34037));
#14007=EDGE_LOOP('',(#34038));
#14008=EDGE_LOOP('',(#34039));
#14009=EDGE_LOOP('',(#34040));
#14010=EDGE_LOOP('',(#34041));
#14011=EDGE_LOOP('',(#34042));
#14012=EDGE_LOOP('',(#34043));
#14013=EDGE_LOOP('',(#34044));
#14014=EDGE_LOOP('',(#34045));
#14015=EDGE_LOOP('',(#34046));
#14016=EDGE_LOOP('',(#34047));
#14017=EDGE_LOOP('',(#34048));
#14018=EDGE_LOOP('',(#34049));
#14019=EDGE_LOOP('',(#34050));
#14020=EDGE_LOOP('',(#34051));
#14021=EDGE_LOOP('',(#34052));
#14022=EDGE_LOOP('',(#34053));
#14023=EDGE_LOOP('',(#34054));
#14024=EDGE_LOOP('',(#34055));
#14025=EDGE_LOOP('',(#34056));
#14026=EDGE_LOOP('',(#34057));
#14027=EDGE_LOOP('',(#34058));
#14028=EDGE_LOOP('',(#34059));
#14029=EDGE_LOOP('',(#34060));
#14030=EDGE_LOOP('',(#34061));
#14031=EDGE_LOOP('',(#34062));
#14032=EDGE_LOOP('',(#34063));
#14033=EDGE_LOOP('',(#34064));
#14034=EDGE_LOOP('',(#34065));
#14035=EDGE_LOOP('',(#34066));
#14036=EDGE_LOOP('',(#34067));
#14037=EDGE_LOOP('',(#34068));
#14038=EDGE_LOOP('',(#34069));
#14039=EDGE_LOOP('',(#34070));
#14040=EDGE_LOOP('',(#34071));
#14041=EDGE_LOOP('',(#34072));
#14042=EDGE_LOOP('',(#34073));
#14043=EDGE_LOOP('',(#34074));
#14044=EDGE_LOOP('',(#34075));
#14045=EDGE_LOOP('',(#34076));
#14046=EDGE_LOOP('',(#34077));
#14047=EDGE_LOOP('',(#34078));
#14048=EDGE_LOOP('',(#34079));
#14049=EDGE_LOOP('',(#34080));
#14050=EDGE_LOOP('',(#34081));
#14051=EDGE_LOOP('',(#34082));
#14052=EDGE_LOOP('',(#34083));
#14053=EDGE_LOOP('',(#34084));
#14054=EDGE_LOOP('',(#34085));
#14055=EDGE_LOOP('',(#34086));
#14056=EDGE_LOOP('',(#34087));
#14057=EDGE_LOOP('',(#34088));
#14058=EDGE_LOOP('',(#34089));
#14059=EDGE_LOOP('',(#34090));
#14060=EDGE_LOOP('',(#34091));
#14061=EDGE_LOOP('',(#34092));
#14062=EDGE_LOOP('',(#34093));
#14063=EDGE_LOOP('',(#34094));
#14064=EDGE_LOOP('',(#34095));
#14065=EDGE_LOOP('',(#34096));
#14066=EDGE_LOOP('',(#34097));
#14067=EDGE_LOOP('',(#34098));
#14068=EDGE_LOOP('',(#34099));
#14069=EDGE_LOOP('',(#34100));
#14070=EDGE_LOOP('',(#34101));
#14071=EDGE_LOOP('',(#34102));
#14072=EDGE_LOOP('',(#34103));
#14073=EDGE_LOOP('',(#34104));
#14074=EDGE_LOOP('',(#34105));
#14075=EDGE_LOOP('',(#34106));
#14076=EDGE_LOOP('',(#34107));
#14077=EDGE_LOOP('',(#34108));
#14078=EDGE_LOOP('',(#34109));
#14079=EDGE_LOOP('',(#34110));
#14080=EDGE_LOOP('',(#34111));
#14081=EDGE_LOOP('',(#34112));
#14082=EDGE_LOOP('',(#34113));
#14083=EDGE_LOOP('',(#34114));
#14084=EDGE_LOOP('',(#34115));
#14085=EDGE_LOOP('',(#34116));
#14086=EDGE_LOOP('',(#34117));
#14087=EDGE_LOOP('',(#34118));
#14088=EDGE_LOOP('',(#34119));
#14089=EDGE_LOOP('',(#34120));
#14090=EDGE_LOOP('',(#34121));
#14091=EDGE_LOOP('',(#34122));
#14092=EDGE_LOOP('',(#34123));
#14093=EDGE_LOOP('',(#34124));
#14094=EDGE_LOOP('',(#34125));
#14095=EDGE_LOOP('',(#34126));
#14096=EDGE_LOOP('',(#34127));
#14097=EDGE_LOOP('',(#34128));
#14098=EDGE_LOOP('',(#34129));
#14099=EDGE_LOOP('',(#34130));
#14100=EDGE_LOOP('',(#34131));
#14101=EDGE_LOOP('',(#34132));
#14102=EDGE_LOOP('',(#34133));
#14103=EDGE_LOOP('',(#34134));
#14104=EDGE_LOOP('',(#34135));
#14105=EDGE_LOOP('',(#34136));
#14106=EDGE_LOOP('',(#34137));
#14107=EDGE_LOOP('',(#34138));
#14108=EDGE_LOOP('',(#34139));
#14109=EDGE_LOOP('',(#34140));
#14110=EDGE_LOOP('',(#34141));
#14111=EDGE_LOOP('',(#34142));
#14112=EDGE_LOOP('',(#34143));
#14113=EDGE_LOOP('',(#34144));
#14114=EDGE_LOOP('',(#34145));
#14115=EDGE_LOOP('',(#34146));
#14116=EDGE_LOOP('',(#34147));
#14117=EDGE_LOOP('',(#34148));
#14118=EDGE_LOOP('',(#34149));
#14119=EDGE_LOOP('',(#34150));
#14120=EDGE_LOOP('',(#34151));
#14121=EDGE_LOOP('',(#34152));
#14122=EDGE_LOOP('',(#34153));
#14123=EDGE_LOOP('',(#34154));
#14124=EDGE_LOOP('',(#34155));
#14125=EDGE_LOOP('',(#34156));
#14126=EDGE_LOOP('',(#34157));
#14127=EDGE_LOOP('',(#34158));
#14128=EDGE_LOOP('',(#34159));
#14129=EDGE_LOOP('',(#34160));
#14130=EDGE_LOOP('',(#34161));
#14131=EDGE_LOOP('',(#34162));
#14132=EDGE_LOOP('',(#34163));
#14133=EDGE_LOOP('',(#34164));
#14134=EDGE_LOOP('',(#34165));
#14135=EDGE_LOOP('',(#34166));
#14136=EDGE_LOOP('',(#34167));
#14137=EDGE_LOOP('',(#34168));
#14138=EDGE_LOOP('',(#34169));
#14139=EDGE_LOOP('',(#34170));
#14140=EDGE_LOOP('',(#34171));
#14141=EDGE_LOOP('',(#34172));
#14142=EDGE_LOOP('',(#34173));
#14143=EDGE_LOOP('',(#34174));
#14144=EDGE_LOOP('',(#34175));
#14145=EDGE_LOOP('',(#34176));
#14146=EDGE_LOOP('',(#34177));
#14147=EDGE_LOOP('',(#34178));
#14148=EDGE_LOOP('',(#34179));
#14149=EDGE_LOOP('',(#34180));
#14150=EDGE_LOOP('',(#34181));
#14151=EDGE_LOOP('',(#34182));
#14152=EDGE_LOOP('',(#34183));
#14153=EDGE_LOOP('',(#34184));
#14154=EDGE_LOOP('',(#34185));
#14155=EDGE_LOOP('',(#34186));
#14156=EDGE_LOOP('',(#34187));
#14157=EDGE_LOOP('',(#34188));
#14158=EDGE_LOOP('',(#34189));
#14159=EDGE_LOOP('',(#34190));
#14160=EDGE_LOOP('',(#34191));
#14161=EDGE_LOOP('',(#34192));
#14162=EDGE_LOOP('',(#34193));
#14163=EDGE_LOOP('',(#34194));
#14164=EDGE_LOOP('',(#34195));
#14165=EDGE_LOOP('',(#34196));
#14166=EDGE_LOOP('',(#34197));
#14167=EDGE_LOOP('',(#34198));
#14168=EDGE_LOOP('',(#34199));
#14169=EDGE_LOOP('',(#34200));
#14170=EDGE_LOOP('',(#34201));
#14171=EDGE_LOOP('',(#34202));
#14172=EDGE_LOOP('',(#34203));
#14173=EDGE_LOOP('',(#34204));
#14174=EDGE_LOOP('',(#34205));
#14175=EDGE_LOOP('',(#34206));
#14176=EDGE_LOOP('',(#34207));
#14177=EDGE_LOOP('',(#34208));
#14178=EDGE_LOOP('',(#34209));
#14179=EDGE_LOOP('',(#34210));
#14180=EDGE_LOOP('',(#34211));
#14181=EDGE_LOOP('',(#34212));
#14182=EDGE_LOOP('',(#34213));
#14183=EDGE_LOOP('',(#34214));
#14184=EDGE_LOOP('',(#34215));
#14185=EDGE_LOOP('',(#34216));
#14186=EDGE_LOOP('',(#34217));
#14187=EDGE_LOOP('',(#34218));
#14188=EDGE_LOOP('',(#34219));
#14189=EDGE_LOOP('',(#34220));
#14190=EDGE_LOOP('',(#34221));
#14191=EDGE_LOOP('',(#34222));
#14192=EDGE_LOOP('',(#34223));
#14193=EDGE_LOOP('',(#34224));
#14194=EDGE_LOOP('',(#34225));
#14195=EDGE_LOOP('',(#34226));
#14196=EDGE_LOOP('',(#34227));
#14197=EDGE_LOOP('',(#34228));
#14198=EDGE_LOOP('',(#34229));
#14199=EDGE_LOOP('',(#34230));
#14200=EDGE_LOOP('',(#34231));
#14201=EDGE_LOOP('',(#34232));
#14202=EDGE_LOOP('',(#34233));
#14203=EDGE_LOOP('',(#34234));
#14204=EDGE_LOOP('',(#34235));
#14205=EDGE_LOOP('',(#34236));
#14206=EDGE_LOOP('',(#34237));
#14207=EDGE_LOOP('',(#34238));
#14208=EDGE_LOOP('',(#34239));
#14209=EDGE_LOOP('',(#34240));
#14210=EDGE_LOOP('',(#34241));
#14211=EDGE_LOOP('',(#34242));
#14212=EDGE_LOOP('',(#34243));
#14213=EDGE_LOOP('',(#34244));
#14214=EDGE_LOOP('',(#34245));
#14215=EDGE_LOOP('',(#34246));
#14216=EDGE_LOOP('',(#34247));
#14217=EDGE_LOOP('',(#34248));
#14218=EDGE_LOOP('',(#34249));
#14219=EDGE_LOOP('',(#34250));
#14220=EDGE_LOOP('',(#34251));
#14221=EDGE_LOOP('',(#34252));
#14222=EDGE_LOOP('',(#34253));
#14223=EDGE_LOOP('',(#34254));
#14224=EDGE_LOOP('',(#34255));
#14225=EDGE_LOOP('',(#34256));
#14226=EDGE_LOOP('',(#34257));
#14227=EDGE_LOOP('',(#34258));
#14228=EDGE_LOOP('',(#34259));
#14229=EDGE_LOOP('',(#34260));
#14230=EDGE_LOOP('',(#34261));
#14231=EDGE_LOOP('',(#34262));
#14232=EDGE_LOOP('',(#34263));
#14233=EDGE_LOOP('',(#34264));
#14234=EDGE_LOOP('',(#34265));
#14235=EDGE_LOOP('',(#34266));
#14236=EDGE_LOOP('',(#34267));
#14237=EDGE_LOOP('',(#34268));
#14238=EDGE_LOOP('',(#34269));
#14239=EDGE_LOOP('',(#34270));
#14240=EDGE_LOOP('',(#34271));
#14241=EDGE_LOOP('',(#34272));
#14242=EDGE_LOOP('',(#34273));
#14243=EDGE_LOOP('',(#34274));
#14244=EDGE_LOOP('',(#34275));
#14245=EDGE_LOOP('',(#34276));
#14246=EDGE_LOOP('',(#34277));
#14247=EDGE_LOOP('',(#34278));
#14248=EDGE_LOOP('',(#34279));
#14249=EDGE_LOOP('',(#34280));
#14250=EDGE_LOOP('',(#34281));
#14251=EDGE_LOOP('',(#34282));
#14252=EDGE_LOOP('',(#34283));
#14253=EDGE_LOOP('',(#34284));
#14254=EDGE_LOOP('',(#34285));
#14255=EDGE_LOOP('',(#34286));
#14256=EDGE_LOOP('',(#34287));
#14257=EDGE_LOOP('',(#34288));
#14258=EDGE_LOOP('',(#34289));
#14259=EDGE_LOOP('',(#34290));
#14260=EDGE_LOOP('',(#34291));
#14261=EDGE_LOOP('',(#34292));
#14262=EDGE_LOOP('',(#34293));
#14263=EDGE_LOOP('',(#34294));
#14264=EDGE_LOOP('',(#34295));
#14265=EDGE_LOOP('',(#34296));
#14266=EDGE_LOOP('',(#34297));
#14267=EDGE_LOOP('',(#34298));
#14268=EDGE_LOOP('',(#34299));
#14269=EDGE_LOOP('',(#34300));
#14270=EDGE_LOOP('',(#34301));
#14271=EDGE_LOOP('',(#34302));
#14272=EDGE_LOOP('',(#34303));
#14273=EDGE_LOOP('',(#34304));
#14274=EDGE_LOOP('',(#34305));
#14275=EDGE_LOOP('',(#34306));
#14276=EDGE_LOOP('',(#34307));
#14277=EDGE_LOOP('',(#34308));
#14278=EDGE_LOOP('',(#34309));
#14279=EDGE_LOOP('',(#34310));
#14280=EDGE_LOOP('',(#34311));
#14281=EDGE_LOOP('',(#34312));
#14282=EDGE_LOOP('',(#34313));
#14283=EDGE_LOOP('',(#34314));
#14284=EDGE_LOOP('',(#34315));
#14285=EDGE_LOOP('',(#34316));
#14286=EDGE_LOOP('',(#34317));
#14287=EDGE_LOOP('',(#34318));
#14288=EDGE_LOOP('',(#34319));
#14289=EDGE_LOOP('',(#34320));
#14290=EDGE_LOOP('',(#34321));
#14291=EDGE_LOOP('',(#34322));
#14292=EDGE_LOOP('',(#34323));
#14293=EDGE_LOOP('',(#34324));
#14294=EDGE_LOOP('',(#34325));
#14295=EDGE_LOOP('',(#34326));
#14296=EDGE_LOOP('',(#34327));
#14297=EDGE_LOOP('',(#34328));
#14298=EDGE_LOOP('',(#34329));
#14299=EDGE_LOOP('',(#34330));
#14300=EDGE_LOOP('',(#34331));
#14301=EDGE_LOOP('',(#34332));
#14302=EDGE_LOOP('',(#34333));
#14303=EDGE_LOOP('',(#34334));
#14304=EDGE_LOOP('',(#34335));
#14305=EDGE_LOOP('',(#34336));
#14306=EDGE_LOOP('',(#34337));
#14307=EDGE_LOOP('',(#34338));
#14308=EDGE_LOOP('',(#34339));
#14309=EDGE_LOOP('',(#34340));
#14310=EDGE_LOOP('',(#34341));
#14311=EDGE_LOOP('',(#34342));
#14312=EDGE_LOOP('',(#34343));
#14313=EDGE_LOOP('',(#34344));
#14314=EDGE_LOOP('',(#34345));
#14315=EDGE_LOOP('',(#34346));
#14316=EDGE_LOOP('',(#34347));
#14317=EDGE_LOOP('',(#34348));
#14318=EDGE_LOOP('',(#34349));
#14319=EDGE_LOOP('',(#34350));
#14320=EDGE_LOOP('',(#34351));
#14321=EDGE_LOOP('',(#34352));
#14322=EDGE_LOOP('',(#34353));
#14323=EDGE_LOOP('',(#34354));
#14324=EDGE_LOOP('',(#34355));
#14325=EDGE_LOOP('',(#34356));
#14326=EDGE_LOOP('',(#34357));
#14327=EDGE_LOOP('',(#34358));
#14328=EDGE_LOOP('',(#34359));
#14329=EDGE_LOOP('',(#34360));
#14330=EDGE_LOOP('',(#34361));
#14331=EDGE_LOOP('',(#34362));
#14332=EDGE_LOOP('',(#34363));
#14333=EDGE_LOOP('',(#34364));
#14334=EDGE_LOOP('',(#34365));
#14335=EDGE_LOOP('',(#34366));
#14336=EDGE_LOOP('',(#34367));
#14337=EDGE_LOOP('',(#34368));
#14338=EDGE_LOOP('',(#34369));
#14339=EDGE_LOOP('',(#34370));
#14340=EDGE_LOOP('',(#34371));
#14341=EDGE_LOOP('',(#34372));
#14342=EDGE_LOOP('',(#34373));
#14343=EDGE_LOOP('',(#34374));
#14344=EDGE_LOOP('',(#34375));
#14345=EDGE_LOOP('',(#34376));
#14346=EDGE_LOOP('',(#34377));
#14347=EDGE_LOOP('',(#34378));
#14348=EDGE_LOOP('',(#34379));
#14349=EDGE_LOOP('',(#34380));
#14350=EDGE_LOOP('',(#34381));
#14351=EDGE_LOOP('',(#34382));
#14352=EDGE_LOOP('',(#34383));
#14353=EDGE_LOOP('',(#34384));
#14354=EDGE_LOOP('',(#34385));
#14355=EDGE_LOOP('',(#34386));
#14356=EDGE_LOOP('',(#34387));
#14357=EDGE_LOOP('',(#34388));
#14358=EDGE_LOOP('',(#34389));
#14359=EDGE_LOOP('',(#34390));
#14360=EDGE_LOOP('',(#34391));
#14361=EDGE_LOOP('',(#34392));
#14362=EDGE_LOOP('',(#34393));
#14363=EDGE_LOOP('',(#34394));
#14364=EDGE_LOOP('',(#34395));
#14365=EDGE_LOOP('',(#34396));
#14366=EDGE_LOOP('',(#34397));
#14367=EDGE_LOOP('',(#34398));
#14368=EDGE_LOOP('',(#34399));
#14369=EDGE_LOOP('',(#34400));
#14370=EDGE_LOOP('',(#34401));
#14371=EDGE_LOOP('',(#34402));
#14372=EDGE_LOOP('',(#34403));
#14373=EDGE_LOOP('',(#34404));
#14374=EDGE_LOOP('',(#34405));
#14375=EDGE_LOOP('',(#34406));
#14376=EDGE_LOOP('',(#34407));
#14377=EDGE_LOOP('',(#34408));
#14378=EDGE_LOOP('',(#34409));
#14379=EDGE_LOOP('',(#34410));
#14380=EDGE_LOOP('',(#34411));
#14381=EDGE_LOOP('',(#34412));
#14382=EDGE_LOOP('',(#34413));
#14383=EDGE_LOOP('',(#34414));
#14384=EDGE_LOOP('',(#34415));
#14385=EDGE_LOOP('',(#34416));
#14386=EDGE_LOOP('',(#34417));
#14387=EDGE_LOOP('',(#34418));
#14388=EDGE_LOOP('',(#34419));
#14389=EDGE_LOOP('',(#34420));
#14390=EDGE_LOOP('',(#34421));
#14391=EDGE_LOOP('',(#34422));
#14392=EDGE_LOOP('',(#34423));
#14393=EDGE_LOOP('',(#34424));
#14394=EDGE_LOOP('',(#34425));
#14395=EDGE_LOOP('',(#34426));
#14396=EDGE_LOOP('',(#34427));
#14397=EDGE_LOOP('',(#34428));
#14398=EDGE_LOOP('',(#34429));
#14399=EDGE_LOOP('',(#34430));
#14400=EDGE_LOOP('',(#34431));
#14401=EDGE_LOOP('',(#34432));
#14402=EDGE_LOOP('',(#34433));
#14403=EDGE_LOOP('',(#34434));
#14404=EDGE_LOOP('',(#34435));
#14405=EDGE_LOOP('',(#34436));
#14406=EDGE_LOOP('',(#34437));
#14407=EDGE_LOOP('',(#34438));
#14408=EDGE_LOOP('',(#34439));
#14409=EDGE_LOOP('',(#34440));
#14410=EDGE_LOOP('',(#34441));
#14411=EDGE_LOOP('',(#34442));
#14412=EDGE_LOOP('',(#34443));
#14413=EDGE_LOOP('',(#34444));
#14414=EDGE_LOOP('',(#34445));
#14415=EDGE_LOOP('',(#34446));
#14416=EDGE_LOOP('',(#34447));
#14417=EDGE_LOOP('',(#34448));
#14418=EDGE_LOOP('',(#34449));
#14419=EDGE_LOOP('',(#34450));
#14420=EDGE_LOOP('',(#34451));
#14421=EDGE_LOOP('',(#34452));
#14422=EDGE_LOOP('',(#34453));
#14423=EDGE_LOOP('',(#34454));
#14424=EDGE_LOOP('',(#34455));
#14425=EDGE_LOOP('',(#34456));
#14426=EDGE_LOOP('',(#34457));
#14427=EDGE_LOOP('',(#34458));
#14428=EDGE_LOOP('',(#34459));
#14429=EDGE_LOOP('',(#34460));
#14430=EDGE_LOOP('',(#34461));
#14431=EDGE_LOOP('',(#34462));
#14432=EDGE_LOOP('',(#34463));
#14433=EDGE_LOOP('',(#34464));
#14434=EDGE_LOOP('',(#34465));
#14435=EDGE_LOOP('',(#34466));
#14436=EDGE_LOOP('',(#34467));
#14437=EDGE_LOOP('',(#34468));
#14438=EDGE_LOOP('',(#34469));
#14439=EDGE_LOOP('',(#34470));
#14440=EDGE_LOOP('',(#34471));
#14441=EDGE_LOOP('',(#34472));
#14442=EDGE_LOOP('',(#34473));
#14443=EDGE_LOOP('',(#34474));
#14444=EDGE_LOOP('',(#34475));
#14445=EDGE_LOOP('',(#34476));
#14446=EDGE_LOOP('',(#34477));
#14447=EDGE_LOOP('',(#34478));
#14448=EDGE_LOOP('',(#34479));
#14449=EDGE_LOOP('',(#34480));
#14450=EDGE_LOOP('',(#34481));
#14451=EDGE_LOOP('',(#34482));
#14452=EDGE_LOOP('',(#34483));
#14453=EDGE_LOOP('',(#34484));
#14454=EDGE_LOOP('',(#34485));
#14455=EDGE_LOOP('',(#34486));
#14456=EDGE_LOOP('',(#34487));
#14457=EDGE_LOOP('',(#34488));
#14458=EDGE_LOOP('',(#34489));
#14459=EDGE_LOOP('',(#34490));
#14460=EDGE_LOOP('',(#34491));
#14461=EDGE_LOOP('',(#34492));
#14462=EDGE_LOOP('',(#34493));
#14463=EDGE_LOOP('',(#34494));
#14464=EDGE_LOOP('',(#34495));
#14465=EDGE_LOOP('',(#34496));
#14466=EDGE_LOOP('',(#34497));
#14467=EDGE_LOOP('',(#34498));
#14468=EDGE_LOOP('',(#34499));
#14469=EDGE_LOOP('',(#34500));
#14470=EDGE_LOOP('',(#34501));
#14471=EDGE_LOOP('',(#34502));
#14472=EDGE_LOOP('',(#34503));
#14473=EDGE_LOOP('',(#34504));
#14474=EDGE_LOOP('',(#34505));
#14475=EDGE_LOOP('',(#34506));
#14476=EDGE_LOOP('',(#34507));
#14477=EDGE_LOOP('',(#34508));
#14478=EDGE_LOOP('',(#34509));
#14479=EDGE_LOOP('',(#34510));
#14480=EDGE_LOOP('',(#34511));
#14481=EDGE_LOOP('',(#34512));
#14482=EDGE_LOOP('',(#34513));
#14483=EDGE_LOOP('',(#34514));
#14484=EDGE_LOOP('',(#34515));
#14485=EDGE_LOOP('',(#34516));
#14486=EDGE_LOOP('',(#34517));
#14487=EDGE_LOOP('',(#34518));
#14488=EDGE_LOOP('',(#34519));
#14489=EDGE_LOOP('',(#34520));
#14490=EDGE_LOOP('',(#34521));
#14491=EDGE_LOOP('',(#34522));
#14492=EDGE_LOOP('',(#34523));
#14493=EDGE_LOOP('',(#34524));
#14494=EDGE_LOOP('',(#34525));
#14495=EDGE_LOOP('',(#34526));
#14496=EDGE_LOOP('',(#34527));
#14497=EDGE_LOOP('',(#34528));
#14498=EDGE_LOOP('',(#34529));
#14499=EDGE_LOOP('',(#34530));
#14500=EDGE_LOOP('',(#34531));
#14501=EDGE_LOOP('',(#34532));
#14502=EDGE_LOOP('',(#34533));
#14503=EDGE_LOOP('',(#34534));
#14504=EDGE_LOOP('',(#34535));
#14505=EDGE_LOOP('',(#34536));
#14506=EDGE_LOOP('',(#34537));
#14507=EDGE_LOOP('',(#34538));
#14508=EDGE_LOOP('',(#34539));
#14509=EDGE_LOOP('',(#34540));
#14510=EDGE_LOOP('',(#34541));
#14511=EDGE_LOOP('',(#34542));
#14512=EDGE_LOOP('',(#34543));
#14513=EDGE_LOOP('',(#34544));
#14514=EDGE_LOOP('',(#34545));
#14515=EDGE_LOOP('',(#34546));
#14516=EDGE_LOOP('',(#34547));
#14517=EDGE_LOOP('',(#34548));
#14518=EDGE_LOOP('',(#34549));
#14519=EDGE_LOOP('',(#34550));
#14520=EDGE_LOOP('',(#34551));
#14521=EDGE_LOOP('',(#34552));
#14522=EDGE_LOOP('',(#34553));
#14523=EDGE_LOOP('',(#34554));
#14524=EDGE_LOOP('',(#34555));
#14525=EDGE_LOOP('',(#34556));
#14526=EDGE_LOOP('',(#34557));
#14527=EDGE_LOOP('',(#34558));
#14528=EDGE_LOOP('',(#34559));
#14529=EDGE_LOOP('',(#34560));
#14530=EDGE_LOOP('',(#34561));
#14531=EDGE_LOOP('',(#34562));
#14532=EDGE_LOOP('',(#34563));
#14533=EDGE_LOOP('',(#34564));
#14534=EDGE_LOOP('',(#34565));
#14535=EDGE_LOOP('',(#34566));
#14536=EDGE_LOOP('',(#34567));
#14537=EDGE_LOOP('',(#34568));
#14538=EDGE_LOOP('',(#34569));
#14539=EDGE_LOOP('',(#34570));
#14540=EDGE_LOOP('',(#34571));
#14541=EDGE_LOOP('',(#34572));
#14542=EDGE_LOOP('',(#34573));
#14543=EDGE_LOOP('',(#34574));
#14544=EDGE_LOOP('',(#34575));
#14545=EDGE_LOOP('',(#34576));
#14546=EDGE_LOOP('',(#34577));
#14547=EDGE_LOOP('',(#34578));
#14548=EDGE_LOOP('',(#34579));
#14549=EDGE_LOOP('',(#34580));
#14550=EDGE_LOOP('',(#34581));
#14551=EDGE_LOOP('',(#34582));
#14552=EDGE_LOOP('',(#34583));
#14553=EDGE_LOOP('',(#34584));
#14554=EDGE_LOOP('',(#34585));
#14555=EDGE_LOOP('',(#34586));
#14556=EDGE_LOOP('',(#34587));
#14557=EDGE_LOOP('',(#34588));
#14558=EDGE_LOOP('',(#34589));
#14559=EDGE_LOOP('',(#34590));
#14560=EDGE_LOOP('',(#34591));
#14561=EDGE_LOOP('',(#34592));
#14562=EDGE_LOOP('',(#34593));
#14563=EDGE_LOOP('',(#34594));
#14564=EDGE_LOOP('',(#34595));
#14565=EDGE_LOOP('',(#34596));
#14566=EDGE_LOOP('',(#34597));
#14567=EDGE_LOOP('',(#34598));
#14568=EDGE_LOOP('',(#34599));
#14569=EDGE_LOOP('',(#34600));
#14570=EDGE_LOOP('',(#34601));
#14571=EDGE_LOOP('',(#34602));
#14572=EDGE_LOOP('',(#34603));
#14573=EDGE_LOOP('',(#34604));
#14574=EDGE_LOOP('',(#34605));
#14575=EDGE_LOOP('',(#34606));
#14576=EDGE_LOOP('',(#34607));
#14577=EDGE_LOOP('',(#34608));
#14578=EDGE_LOOP('',(#34609));
#14579=EDGE_LOOP('',(#34610));
#14580=EDGE_LOOP('',(#34611));
#14581=EDGE_LOOP('',(#34612));
#14582=EDGE_LOOP('',(#34613));
#14583=EDGE_LOOP('',(#34614));
#14584=EDGE_LOOP('',(#34615));
#14585=EDGE_LOOP('',(#34616));
#14586=EDGE_LOOP('',(#34617));
#14587=EDGE_LOOP('',(#34618));
#14588=EDGE_LOOP('',(#34619));
#14589=EDGE_LOOP('',(#34620));
#14590=EDGE_LOOP('',(#34621));
#14591=EDGE_LOOP('',(#34622));
#14592=EDGE_LOOP('',(#34623));
#14593=EDGE_LOOP('',(#34624));
#14594=EDGE_LOOP('',(#34625));
#14595=EDGE_LOOP('',(#34626));
#14596=EDGE_LOOP('',(#34627));
#14597=EDGE_LOOP('',(#34628));
#14598=EDGE_LOOP('',(#34629));
#14599=EDGE_LOOP('',(#34630));
#14600=EDGE_LOOP('',(#34631));
#14601=EDGE_LOOP('',(#34632));
#14602=EDGE_LOOP('',(#34633));
#14603=EDGE_LOOP('',(#34634));
#14604=EDGE_LOOP('',(#34635));
#14605=EDGE_LOOP('',(#34636));
#14606=EDGE_LOOP('',(#34637));
#14607=EDGE_LOOP('',(#34638));
#14608=EDGE_LOOP('',(#34639));
#14609=EDGE_LOOP('',(#34640));
#14610=EDGE_LOOP('',(#34641));
#14611=EDGE_LOOP('',(#34642));
#14612=EDGE_LOOP('',(#34643));
#14613=EDGE_LOOP('',(#34644));
#14614=EDGE_LOOP('',(#34645));
#14615=EDGE_LOOP('',(#34646));
#14616=EDGE_LOOP('',(#34647));
#14617=EDGE_LOOP('',(#34648));
#14618=EDGE_LOOP('',(#34649));
#14619=EDGE_LOOP('',(#34650));
#14620=EDGE_LOOP('',(#34651));
#14621=EDGE_LOOP('',(#34652));
#14622=EDGE_LOOP('',(#34653));
#14623=EDGE_LOOP('',(#34654));
#14624=EDGE_LOOP('',(#34655));
#14625=EDGE_LOOP('',(#34656));
#14626=EDGE_LOOP('',(#34657));
#14627=EDGE_LOOP('',(#34658));
#14628=EDGE_LOOP('',(#34659));
#14629=EDGE_LOOP('',(#34660));
#14630=EDGE_LOOP('',(#34661));
#14631=EDGE_LOOP('',(#34662));
#14632=EDGE_LOOP('',(#34663));
#14633=EDGE_LOOP('',(#34664));
#14634=EDGE_LOOP('',(#34665));
#14635=EDGE_LOOP('',(#34666));
#14636=EDGE_LOOP('',(#34667));
#14637=EDGE_LOOP('',(#34668));
#14638=EDGE_LOOP('',(#34669));
#14639=EDGE_LOOP('',(#34670));
#14640=EDGE_LOOP('',(#34671));
#14641=EDGE_LOOP('',(#34672));
#14642=EDGE_LOOP('',(#34673));
#14643=EDGE_LOOP('',(#34674));
#14644=EDGE_LOOP('',(#34675));
#14645=EDGE_LOOP('',(#34676));
#14646=EDGE_LOOP('',(#34677));
#14647=EDGE_LOOP('',(#34678));
#14648=EDGE_LOOP('',(#34679));
#14649=EDGE_LOOP('',(#34680));
#14650=EDGE_LOOP('',(#34681));
#14651=EDGE_LOOP('',(#34682));
#14652=EDGE_LOOP('',(#34683));
#14653=EDGE_LOOP('',(#34684));
#14654=EDGE_LOOP('',(#34685));
#14655=EDGE_LOOP('',(#34686));
#14656=EDGE_LOOP('',(#34687));
#14657=EDGE_LOOP('',(#34688));
#14658=EDGE_LOOP('',(#34689));
#14659=EDGE_LOOP('',(#34690));
#14660=EDGE_LOOP('',(#34691));
#14661=EDGE_LOOP('',(#34692));
#14662=EDGE_LOOP('',(#34693));
#14663=EDGE_LOOP('',(#34694));
#14664=EDGE_LOOP('',(#34695));
#14665=EDGE_LOOP('',(#34696));
#14666=EDGE_LOOP('',(#34697));
#14667=EDGE_LOOP('',(#34698));
#14668=EDGE_LOOP('',(#34699));
#14669=EDGE_LOOP('',(#34700));
#14670=EDGE_LOOP('',(#34701));
#14671=EDGE_LOOP('',(#34702));
#14672=EDGE_LOOP('',(#34703));
#14673=EDGE_LOOP('',(#34704));
#14674=EDGE_LOOP('',(#34705));
#14675=EDGE_LOOP('',(#34706));
#14676=EDGE_LOOP('',(#34707));
#14677=EDGE_LOOP('',(#34708));
#14678=EDGE_LOOP('',(#34709));
#14679=EDGE_LOOP('',(#34710));
#14680=EDGE_LOOP('',(#34711));
#14681=EDGE_LOOP('',(#34712));
#14682=EDGE_LOOP('',(#34713));
#14683=EDGE_LOOP('',(#34714));
#14684=EDGE_LOOP('',(#34715));
#14685=EDGE_LOOP('',(#34716));
#14686=EDGE_LOOP('',(#34717));
#14687=EDGE_LOOP('',(#34718));
#14688=EDGE_LOOP('',(#34719));
#14689=EDGE_LOOP('',(#34720));
#14690=EDGE_LOOP('',(#34721));
#14691=EDGE_LOOP('',(#34722));
#14692=EDGE_LOOP('',(#34723));
#14693=EDGE_LOOP('',(#34724));
#14694=EDGE_LOOP('',(#34725));
#14695=EDGE_LOOP('',(#34726));
#14696=EDGE_LOOP('',(#34727));
#14697=EDGE_LOOP('',(#34728));
#14698=EDGE_LOOP('',(#34729));
#14699=EDGE_LOOP('',(#34730));
#14700=EDGE_LOOP('',(#34731));
#14701=EDGE_LOOP('',(#34732));
#14702=EDGE_LOOP('',(#34733));
#14703=EDGE_LOOP('',(#34734));
#14704=EDGE_LOOP('',(#34735));
#14705=EDGE_LOOP('',(#34736));
#14706=EDGE_LOOP('',(#34737,#34738));
#14707=EDGE_LOOP('',(#34739));
#14708=EDGE_LOOP('',(#34740));
#14709=EDGE_LOOP('',(#34741,#34742));
#14710=EDGE_LOOP('',(#34743));
#14711=EDGE_LOOP('',(#34744));
#14712=EDGE_LOOP('',(#34745,#34746));
#14713=EDGE_LOOP('',(#34747));
#14714=EDGE_LOOP('',(#34748));
#14715=EDGE_LOOP('',(#34749,#34750));
#14716=EDGE_LOOP('',(#34751));
#14717=EDGE_LOOP('',(#34752));
#14718=EDGE_LOOP('',(#34753,#34754));
#14719=EDGE_LOOP('',(#34755));
#14720=EDGE_LOOP('',(#34756));
#14721=EDGE_LOOP('',(#34757,#34758));
#14722=EDGE_LOOP('',(#34759));
#14723=EDGE_LOOP('',(#34760));
#14724=EDGE_LOOP('',(#34761,#34762));
#14725=EDGE_LOOP('',(#34763));
#14726=EDGE_LOOP('',(#34764));
#14727=EDGE_LOOP('',(#34765,#34766));
#14728=EDGE_LOOP('',(#34767));
#14729=EDGE_LOOP('',(#34768));
#14730=EDGE_LOOP('',(#34769,#34770));
#14731=EDGE_LOOP('',(#34771));
#14732=EDGE_LOOP('',(#34772));
#14733=EDGE_LOOP('',(#34773,#34774));
#14734=EDGE_LOOP('',(#34775));
#14735=EDGE_LOOP('',(#34776));
#14736=EDGE_LOOP('',(#34777,#34778));
#14737=EDGE_LOOP('',(#34779));
#14738=EDGE_LOOP('',(#34780));
#14739=EDGE_LOOP('',(#34781,#34782));
#14740=EDGE_LOOP('',(#34783));
#14741=EDGE_LOOP('',(#34784));
#14742=EDGE_LOOP('',(#34785,#34786));
#14743=EDGE_LOOP('',(#34787));
#14744=EDGE_LOOP('',(#34788));
#14745=EDGE_LOOP('',(#34789,#34790));
#14746=EDGE_LOOP('',(#34791));
#14747=EDGE_LOOP('',(#34792));
#14748=EDGE_LOOP('',(#34793));
#14749=EDGE_LOOP('',(#34794));
#14750=EDGE_LOOP('',(#34795));
#14751=EDGE_LOOP('',(#34796,#34797));
#14752=EDGE_LOOP('',(#34798));
#14753=EDGE_LOOP('',(#34799));
#14754=EDGE_LOOP('',(#34800,#34801));
#14755=EDGE_LOOP('',(#34802));
#14756=EDGE_LOOP('',(#34803));
#14757=EDGE_LOOP('',(#34804));
#14758=EDGE_LOOP('',(#34805));
#14759=EDGE_LOOP('',(#34806));
#14760=EDGE_LOOP('',(#34807,#34808));
#14761=EDGE_LOOP('',(#34809));
#14762=EDGE_LOOP('',(#34810));
#14763=EDGE_LOOP('',(#34811,#34812));
#14764=EDGE_LOOP('',(#34813));
#14765=EDGE_LOOP('',(#34814));
#14766=EDGE_LOOP('',(#34815));
#14767=EDGE_LOOP('',(#34816));
#14768=EDGE_LOOP('',(#34817));
#14769=EDGE_LOOP('',(#34818));
#14770=EDGE_LOOP('',(#34819));
#14771=EDGE_LOOP('',(#34820));
#14772=EDGE_LOOP('',(#34821,#34822));
#14773=EDGE_LOOP('',(#34823));
#14774=EDGE_LOOP('',(#34824));
#14775=EDGE_LOOP('',(#34825,#34826));
#14776=EDGE_LOOP('',(#34827));
#14777=EDGE_LOOP('',(#34828));
#14778=EDGE_LOOP('',(#34829));
#14779=EDGE_LOOP('',(#34830));
#14780=EDGE_LOOP('',(#34831));
#14781=EDGE_LOOP('',(#34832));
#14782=EDGE_LOOP('',(#34833));
#14783=EDGE_LOOP('',(#34834));
#14784=EDGE_LOOP('',(#34835,#34836));
#14785=EDGE_LOOP('',(#34837));
#14786=EDGE_LOOP('',(#34838));
#14787=EDGE_LOOP('',(#34839,#34840));
#14788=EDGE_LOOP('',(#34841));
#14789=EDGE_LOOP('',(#34842));
#14790=EDGE_LOOP('',(#34843,#34844));
#14791=EDGE_LOOP('',(#34845));
#14792=EDGE_LOOP('',(#34846));
#14793=EDGE_LOOP('',(#34847,#34848));
#14794=EDGE_LOOP('',(#34849));
#14795=EDGE_LOOP('',(#34850));
#14796=EDGE_LOOP('',(#34851,#34852));
#14797=EDGE_LOOP('',(#34853));
#14798=EDGE_LOOP('',(#34854));
#14799=EDGE_LOOP('',(#34855,#34856));
#14800=EDGE_LOOP('',(#34857));
#14801=EDGE_LOOP('',(#34858));
#14802=EDGE_LOOP('',(#34859,#34860));
#14803=EDGE_LOOP('',(#34861));
#14804=EDGE_LOOP('',(#34862));
#14805=EDGE_LOOP('',(#34863,#34864));
#14806=EDGE_LOOP('',(#34865));
#14807=EDGE_LOOP('',(#34866));
#14808=EDGE_LOOP('',(#34867,#34868));
#14809=EDGE_LOOP('',(#34869));
#14810=EDGE_LOOP('',(#34870));
#14811=EDGE_LOOP('',(#34871,#34872));
#14812=EDGE_LOOP('',(#34873));
#14813=EDGE_LOOP('',(#34874));
#14814=EDGE_LOOP('',(#34875,#34876));
#14815=EDGE_LOOP('',(#34877));
#14816=EDGE_LOOP('',(#34878));
#14817=EDGE_LOOP('',(#34879,#34880));
#14818=EDGE_LOOP('',(#34881));
#14819=EDGE_LOOP('',(#34882));
#14820=EDGE_LOOP('',(#34883,#34884));
#14821=EDGE_LOOP('',(#34885));
#14822=EDGE_LOOP('',(#34886));
#14823=EDGE_LOOP('',(#34887,#34888));
#14824=EDGE_LOOP('',(#34889));
#14825=EDGE_LOOP('',(#34890));
#14826=EDGE_LOOP('',(#34891,#34892));
#14827=EDGE_LOOP('',(#34893));
#14828=EDGE_LOOP('',(#34894));
#14829=EDGE_LOOP('',(#34895,#34896));
#14830=EDGE_LOOP('',(#34897));
#14831=EDGE_LOOP('',(#34898));
#14832=EDGE_LOOP('',(#34899,#34900));
#14833=EDGE_LOOP('',(#34901));
#14834=EDGE_LOOP('',(#34902));
#14835=EDGE_LOOP('',(#34903,#34904));
#14836=EDGE_LOOP('',(#34905));
#14837=EDGE_LOOP('',(#34906));
#14838=EDGE_LOOP('',(#34907,#34908));
#14839=EDGE_LOOP('',(#34909));
#14840=EDGE_LOOP('',(#34910));
#14841=EDGE_LOOP('',(#34911,#34912));
#14842=EDGE_LOOP('',(#34913));
#14843=EDGE_LOOP('',(#34914));
#14844=EDGE_LOOP('',(#34915,#34916));
#14845=EDGE_LOOP('',(#34917));
#14846=EDGE_LOOP('',(#34918));
#14847=EDGE_LOOP('',(#34919,#34920));
#14848=EDGE_LOOP('',(#34921));
#14849=EDGE_LOOP('',(#34922));
#14850=EDGE_LOOP('',(#34923,#34924));
#14851=EDGE_LOOP('',(#34925));
#14852=EDGE_LOOP('',(#34926));
#14853=EDGE_LOOP('',(#34927,#34928));
#14854=EDGE_LOOP('',(#34929));
#14855=EDGE_LOOP('',(#34930));
#14856=EDGE_LOOP('',(#34931,#34932));
#14857=EDGE_LOOP('',(#34933));
#14858=EDGE_LOOP('',(#34934));
#14859=EDGE_LOOP('',(#34935,#34936));
#14860=EDGE_LOOP('',(#34937));
#14861=EDGE_LOOP('',(#34938));
#14862=EDGE_LOOP('',(#34939,#34940));
#14863=EDGE_LOOP('',(#34941));
#14864=EDGE_LOOP('',(#34942));
#14865=EDGE_LOOP('',(#34943,#34944));
#14866=EDGE_LOOP('',(#34945));
#14867=EDGE_LOOP('',(#34946));
#14868=EDGE_LOOP('',(#34947,#34948));
#14869=EDGE_LOOP('',(#34949));
#14870=EDGE_LOOP('',(#34950));
#14871=EDGE_LOOP('',(#34951,#34952));
#14872=EDGE_LOOP('',(#34953));
#14873=EDGE_LOOP('',(#34954));
#14874=EDGE_LOOP('',(#34955,#34956));
#14875=EDGE_LOOP('',(#34957));
#14876=EDGE_LOOP('',(#34958));
#14877=EDGE_LOOP('',(#34959,#34960));
#14878=EDGE_LOOP('',(#34961));
#14879=EDGE_LOOP('',(#34962));
#14880=EDGE_LOOP('',(#34963,#34964));
#14881=EDGE_LOOP('',(#34965));
#14882=EDGE_LOOP('',(#34966));
#14883=EDGE_LOOP('',(#34967,#34968));
#14884=EDGE_LOOP('',(#34969));
#14885=EDGE_LOOP('',(#34970));
#14886=EDGE_LOOP('',(#34971,#34972));
#14887=EDGE_LOOP('',(#34973));
#14888=EDGE_LOOP('',(#34974));
#14889=EDGE_LOOP('',(#34975,#34976));
#14890=EDGE_LOOP('',(#34977));
#14891=EDGE_LOOP('',(#34978));
#14892=EDGE_LOOP('',(#34979,#34980));
#14893=EDGE_LOOP('',(#34981));
#14894=EDGE_LOOP('',(#34982));
#14895=EDGE_LOOP('',(#34983,#34984));
#14896=EDGE_LOOP('',(#34985));
#14897=EDGE_LOOP('',(#34986));
#14898=EDGE_LOOP('',(#34987,#34988));
#14899=EDGE_LOOP('',(#34989));
#14900=EDGE_LOOP('',(#34990));
#14901=EDGE_LOOP('',(#34991));
#14902=EDGE_LOOP('',(#34992));
#14903=EDGE_LOOP('',(#34993));
#14904=EDGE_LOOP('',(#34994));
#14905=EDGE_LOOP('',(#34995));
#14906=EDGE_LOOP('',(#34996));
#14907=EDGE_LOOP('',(#34997));
#14908=EDGE_LOOP('',(#34998));
#14909=EDGE_LOOP('',(#34999));
#14910=EDGE_LOOP('',(#35000));
#14911=EDGE_LOOP('',(#35001));
#14912=EDGE_LOOP('',(#35002));
#14913=EDGE_LOOP('',(#35003));
#14914=EDGE_LOOP('',(#35004));
#14915=EDGE_LOOP('',(#35005));
#14916=EDGE_LOOP('',(#35006));
#14917=EDGE_LOOP('',(#35007));
#17713=CIRCLE('',#45572,8.3031389659941);
#17714=CIRCLE('',#45582,8.3031389659941);
#17715=CIRCLE('',#45585,0.500000000000054);
#17716=CIRCLE('',#45586,0.500000000000054);
#17717=CIRCLE('',#45588,1.81285717707167);
#17718=CIRCLE('',#45589,1.81285717707168);
#17719=CIRCLE('',#45591,0.500000000000054);
#17720=CIRCLE('',#45592,0.500000000000054);
#17721=CIRCLE('',#45594,1.81285717707167);
#17722=CIRCLE('',#45595,1.81285717707167);
#17723=CIRCLE('',#45597,0.500000000000054);
#17724=CIRCLE('',#45598,0.500000000000054);
#17725=CIRCLE('',#45600,1.81285717707166);
#17726=CIRCLE('',#45601,1.81285717707166);
#17727=CIRCLE('',#45603,0.499999999999939);
#17728=CIRCLE('',#45604,0.499999999999935);
#17729=CIRCLE('',#45606,1.81285717707155);
#17730=CIRCLE('',#45607,1.81285717707156);
#17731=CIRCLE('',#45609,0.499999999999935);
#17732=CIRCLE('',#45610,0.499999999999935);
#17733=CIRCLE('',#45612,1.81285717707155);
#17734=CIRCLE('',#45613,1.81285717707155);
#17735=CIRCLE('',#45615,0.499999999999944);
#17736=CIRCLE('',#45616,0.499999999999944);
#17737=CIRCLE('',#45618,1.81285717707167);
#17738=CIRCLE('',#45619,1.81285717707167);
#17739=CIRCLE('',#45622,0.500000000000053);
#17740=CIRCLE('',#45625,0.500000000000049);
#17741=CIRCLE('',#45628,0.500000000000049);
#17742=CIRCLE('',#45631,0.500000000000049);
#17743=CIRCLE('',#45634,0.500000000000049);
#17744=CIRCLE('',#45637,0.499999999999944);
#17745=CIRCLE('',#45640,0.499999999999944);
#17746=CIRCLE('',#45643,0.500000000000058);
#17747=CIRCLE('',#45646,0.500000000000058);
#17748=CIRCLE('',#45649,0.500000000000058);
#17749=CIRCLE('',#45652,0.500000000000172);
#17750=CIRCLE('',#45655,0.499999999999935);
#17751=CIRCLE('',#45658,0.500000000000058);
#17752=CIRCLE('',#45661,0.499999999999935);
#17753=CIRCLE('',#45664,0.500000000000058);
#17754=CIRCLE('',#45667,0.500000000000058);
#17755=CIRCLE('',#45670,0.499999999999944);
#17756=CIRCLE('',#45673,0.500000000000067);
#17757=CIRCLE('',#45676,0.499999999999935);
#17758=CIRCLE('',#45679,0.499999999999935);
#17759=CIRCLE('',#45682,0.500000000000058);
#17760=CIRCLE('',#45685,0.499999999999944);
#17761=CIRCLE('',#45688,0.499999999999944);
#17762=CIRCLE('',#45691,0.499999999999944);
#17763=CIRCLE('',#45694,0.500000000000172);
#17764=CIRCLE('',#45697,0.499999999999944);
#17765=CIRCLE('',#45700,0.500000000000049);
#17766=CIRCLE('',#45703,0.499999999999939);
#17767=CIRCLE('',#45706,0.500000000000053);
#17768=CIRCLE('',#45709,0.500000000000053);
#17769=CIRCLE('',#45712,0.500000000000049);
#17770=CIRCLE('',#45715,0.500000000000053);
#17771=CIRCLE('',#45718,0.500000000000053);
#17772=CIRCLE('',#45721,0.500000000000049);
#17773=CIRCLE('',#45724,0.500000000000049);
#17774=CIRCLE('',#45727,0.500000000000063);
#17775=CIRCLE('',#45730,0.499999999999944);
#17776=CIRCLE('',#45733,0.499999999999935);
#17777=CIRCLE('',#45736,0.499999999999944);
#17778=CIRCLE('',#45738,1.54967110260237);
#17779=CIRCLE('',#45740,0.499999999999939);
#17780=CIRCLE('',#45741,0.499999999999939);
#17781=CIRCLE('',#45743,1.25936103546568);
#17782=CIRCLE('',#45745,0.500000000000049);
#17783=CIRCLE('',#45746,0.500000000000049);
#17784=CIRCLE('',#45749,0.499999999999939);
#17785=CIRCLE('',#45752,0.499999999999939);
#17786=CIRCLE('',#45754,1.54967110260249);
#17787=CIRCLE('',#45756,0.499999999999944);
#17788=CIRCLE('',#45757,0.499999999999944);
#17789=CIRCLE('',#45759,1.25936103546569);
#17790=CIRCLE('',#45761,0.500000000000058);
#17791=CIRCLE('',#45762,0.500000000000058);
#17792=CIRCLE('',#45765,0.500000000000058);
#17793=CIRCLE('',#45768,0.500000000000053);
#17794=CIRCLE('',#45770,1.25936103546568);
#17795=CIRCLE('',#45772,0.500000000000053);
#17796=CIRCLE('',#45773,0.500000000000049);
#17797=CIRCLE('',#45776,0.500000000000058);
#17798=CIRCLE('',#45779,0.500000000000058);
#17799=CIRCLE('',#45781,1.25936103546568);
#17800=CIRCLE('',#45783,0.499999999999939);
#17801=CIRCLE('',#45784,0.499999999999939);
#17802=CIRCLE('',#45787,0.500000000000058);
#17803=CIRCLE('',#45790,0.499999999999939);
#17804=CIRCLE('',#45793,0.499999999999944);
#17805=CIRCLE('',#45796,0.499999999999944);
#17806=CIRCLE('',#45799,0.500000000000058);
#17807=CIRCLE('',#45802,0.500000000000053);
#17808=CIRCLE('',#45805,0.499999999999944);
#17809=CIRCLE('',#45808,0.500000000000063);
#17810=CIRCLE('',#45811,0.499999999999939);
#17811=CIRCLE('',#45814,0.500000000000053);
#17812=CIRCLE('',#45817,0.500000000000053);
#17813=CIRCLE('',#45820,0.499999999999939);
#17814=CIRCLE('',#45823,0.500000000000053);
#17815=CIRCLE('',#45826,0.499999999999944);
#17816=CIRCLE('',#45828,1.05888347462729);
#17817=CIRCLE('',#45829,1.05888347462729);
#17818=CIRCLE('',#45831,0.500000000000049);
#17819=CIRCLE('',#45832,0.500000000000049);
#17820=CIRCLE('',#45834,1.29583333162394);
#17821=CIRCLE('',#45835,1.29583333162394);
#17822=CIRCLE('',#45837,0.500000000000049);
#17823=CIRCLE('',#45838,0.500000000000049);
#17824=CIRCLE('',#45840,1.60653900437062);
#17825=CIRCLE('',#45841,1.60653900437062);
#17826=CIRCLE('',#45843,0.500000000000049);
#17827=CIRCLE('',#45844,0.500000000000049);
#17828=CIRCLE('',#45846,1.82809807486272);
#17829=CIRCLE('',#45847,1.82809807486272);
#17830=CIRCLE('',#45849,0.499999999999944);
#17831=CIRCLE('',#45850,0.499999999999944);
#17832=CIRCLE('',#45852,1.85841829658605);
#17833=CIRCLE('',#45853,1.85841829658605);
#17834=CIRCLE('',#45855,0.500000000000049);
#17835=CIRCLE('',#45856,0.500000000000049);
#17836=CIRCLE('',#45858,1.81285717707166);
#17837=CIRCLE('',#45859,1.81285717707167);
#17838=CIRCLE('',#45861,0.500000000000049);
#17839=CIRCLE('',#45862,0.500000000000049);
#17840=CIRCLE('',#45864,1.91146602029503);
#17841=CIRCLE('',#45865,1.91146602029503);
#17842=CIRCLE('',#45867,0.500000000000049);
#17843=CIRCLE('',#45868,0.500000000000049);
#17844=CIRCLE('',#45870,1.54967110260248);
#17845=CIRCLE('',#45871,1.54967110260249);
#17846=CIRCLE('',#45873,0.499999999999944);
#17847=CIRCLE('',#45874,0.499999999999944);
#17848=CIRCLE('',#45876,1.25936103546569);
#17849=CIRCLE('',#45877,1.25936103546556);
#17850=CIRCLE('',#45879,0.500000000000049);
#17851=CIRCLE('',#45880,0.500000000000049);
#17852=CIRCLE('',#45882,1.0588834746273);
#17853=CIRCLE('',#45883,1.0588834746273);
#17854=CIRCLE('',#45885,0.500000000000049);
#17855=CIRCLE('',#45886,0.500000000000049);
#17856=CIRCLE('',#45888,1.29583333162394);
#17857=CIRCLE('',#45889,1.29583333162394);
#17858=CIRCLE('',#45891,0.499999999999944);
#17859=CIRCLE('',#45892,0.499999999999944);
#17860=CIRCLE('',#45894,1.60653900437062);
#17861=CIRCLE('',#45895,1.60653900437062);
#17862=CIRCLE('',#45897,0.500000000000058);
#17863=CIRCLE('',#45898,0.500000000000058);
#17864=CIRCLE('',#45900,1.82809807486272);
#17865=CIRCLE('',#45901,1.82809807486272);
#17866=CIRCLE('',#45903,0.499999999999944);
#17867=CIRCLE('',#45904,0.499999999999944);
#17868=CIRCLE('',#45906,1.85841829658605);
#17869=CIRCLE('',#45907,1.85841829658605);
#17870=CIRCLE('',#45909,0.499999999999944);
#17871=CIRCLE('',#45910,0.499999999999944);
#17872=CIRCLE('',#45912,1.81285717707166);
#17873=CIRCLE('',#45913,1.81285717707167);
#17874=CIRCLE('',#45915,0.499999999999944);
#17875=CIRCLE('',#45916,0.499999999999944);
#17876=CIRCLE('',#45918,1.91146602029502);
#17877=CIRCLE('',#45919,1.91146602029503);
#17878=CIRCLE('',#45921,0.500000000000049);
#17879=CIRCLE('',#45922,0.500000000000049);
#17880=CIRCLE('',#45924,1.54967110260249);
#17881=CIRCLE('',#45925,1.54967110260249);
#17882=CIRCLE('',#45927,0.499999999999944);
#17883=CIRCLE('',#45928,0.499999999999944);
#17884=CIRCLE('',#45930,1.25936103546569);
#17885=CIRCLE('',#45931,1.25936103546556);
#17886=CIRCLE('',#45933,0.500000000000049);
#17887=CIRCLE('',#45934,0.500000000000049);
#17888=CIRCLE('',#45936,1.05888347462729);
#17889=CIRCLE('',#45937,1.05888347462729);
#17890=CIRCLE('',#45939,0.499999999999935);
#17891=CIRCLE('',#45940,0.499999999999935);
#17892=CIRCLE('',#45942,1.29583333162394);
#17893=CIRCLE('',#45943,1.29583333162394);
#17894=CIRCLE('',#45945,0.500000000000058);
#17895=CIRCLE('',#45946,0.500000000000058);
#17896=CIRCLE('',#45948,1.60653900437051);
#17897=CIRCLE('',#45949,1.60653900437051);
#17898=CIRCLE('',#45951,0.499999999999935);
#17899=CIRCLE('',#45952,0.499999999999935);
#17900=CIRCLE('',#45954,1.82809807486262);
#17901=CIRCLE('',#45955,1.82809807486262);
#17902=CIRCLE('',#45957,0.500000000000049);
#17903=CIRCLE('',#45958,0.500000000000049);
#17904=CIRCLE('',#45960,1.85841829658605);
#17905=CIRCLE('',#45961,1.85841829658605);
#17906=CIRCLE('',#45963,0.500000000000049);
#17907=CIRCLE('',#45964,0.500000000000049);
#17908=CIRCLE('',#45966,1.91146602029503);
#17909=CIRCLE('',#45967,1.91146602029503);
#17910=CIRCLE('',#45969,0.500000000000049);
#17911=CIRCLE('',#45970,0.500000000000049);
#17912=CIRCLE('',#45972,1.54967110260249);
#17913=CIRCLE('',#45973,1.54967110260249);
#17914=CIRCLE('',#45975,0.500000000000058);
#17915=CIRCLE('',#45976,0.500000000000058);
#17916=CIRCLE('',#45978,1.25936103546568);
#17917=CIRCLE('',#45979,1.25936103546556);
#17918=CIRCLE('',#45981,0.500000000000049);
#17919=CIRCLE('',#45982,0.500000000000049);
#17920=CIRCLE('',#45984,1.05888347462729);
#17921=CIRCLE('',#45985,1.05888347462729);
#17922=CIRCLE('',#45987,0.500000000000049);
#17923=CIRCLE('',#45988,0.500000000000049);
#17924=CIRCLE('',#45990,1.29583333162382);
#17925=CIRCLE('',#45991,1.29583333162382);
#17926=CIRCLE('',#45993,0.499999999999821);
#17927=CIRCLE('',#45994,0.499999999999821);
#17928=CIRCLE('',#45996,1.6065390043705);
#17929=CIRCLE('',#45997,1.60653900437051);
#17930=CIRCLE('',#45999,0.500000000000058);
#17931=CIRCLE('',#46000,0.500000000000058);
#17932=CIRCLE('',#46002,1.82809807486273);
#17933=CIRCLE('',#46003,1.82809807486273);
#17934=CIRCLE('',#46005,0.500000000000049);
#17935=CIRCLE('',#46006,0.500000000000049);
#17936=CIRCLE('',#46008,1.85841829658605);
#17937=CIRCLE('',#46009,1.85841829658605);
#17938=CIRCLE('',#46011,0.500000000000049);
#17939=CIRCLE('',#46012,0.500000000000049);
#17940=CIRCLE('',#46014,1.81285717707167);
#17941=CIRCLE('',#46015,1.81285717707167);
#17942=CIRCLE('',#46017,0.499999999999944);
#17943=CIRCLE('',#46018,0.499999999999944);
#17944=CIRCLE('',#46020,1.91146602029503);
#17945=CIRCLE('',#46021,1.91146602029503);
#17946=CIRCLE('',#46023,0.500000000000058);
#17947=CIRCLE('',#46024,0.500000000000058);
#17948=CIRCLE('',#46026,1.5496711026026);
#17949=CIRCLE('',#46027,1.5496711026026);
#17950=CIRCLE('',#46029,0.500000000000058);
#17951=CIRCLE('',#46030,0.500000000000058);
#17952=CIRCLE('',#46032,1.25936103546569);
#17953=CIRCLE('',#46033,1.25936103546568);
#17954=CIRCLE('',#46035,0.500000000000049);
#17955=CIRCLE('',#46036,0.500000000000049);
#17956=CIRCLE('',#46038,1.05888347462741);
#17957=CIRCLE('',#46039,1.05888347462741);
#17958=CIRCLE('',#46041,0.500000000000049);
#17959=CIRCLE('',#46042,0.500000000000049);
#17960=CIRCLE('',#46044,1.29583333162417);
#17961=CIRCLE('',#46045,1.29583333162417);
#17962=CIRCLE('',#46047,0.500000000000172);
#17963=CIRCLE('',#46048,0.500000000000172);
#17964=CIRCLE('',#46050,1.60653900437062);
#17965=CIRCLE('',#46051,1.60653900437062);
#17966=CIRCLE('',#46053,0.500000000000058);
#17967=CIRCLE('',#46054,0.500000000000058);
#17968=CIRCLE('',#46056,1.82809807486272);
#17969=CIRCLE('',#46057,1.82809807486272);
#17970=CIRCLE('',#46059,0.500000000000049);
#17971=CIRCLE('',#46060,0.500000000000049);
#17972=CIRCLE('',#46062,1.85841829658604);
#17973=CIRCLE('',#46063,1.85841829658605);
#17974=CIRCLE('',#46065,0.499999999999935);
#17975=CIRCLE('',#46066,0.499999999999935);
#17976=CIRCLE('',#46068,1.81285717707167);
#17977=CIRCLE('',#46069,1.81285717707167);
#17978=CIRCLE('',#46071,0.499999999999944);
#17979=CIRCLE('',#46072,0.499999999999944);
#17980=CIRCLE('',#46074,1.91146602029502);
#17981=CIRCLE('',#46075,1.91146602029502);
#17982=CIRCLE('',#46077,0.499999999999935);
#17983=CIRCLE('',#46078,0.499999999999935);
#17984=CIRCLE('',#46080,1.54967110260249);
#17985=CIRCLE('',#46081,1.54967110260249);
#17986=CIRCLE('',#46083,0.499999999999935);
#17987=CIRCLE('',#46084,0.499999999999935);
#17988=CIRCLE('',#46086,1.25936103546568);
#17989=CIRCLE('',#46087,1.25936103546568);
#17990=CIRCLE('',#46089,0.500000000000058);
#17991=CIRCLE('',#46090,0.500000000000058);
#17992=CIRCLE('',#46092,1.05888347462741);
#17993=CIRCLE('',#46093,1.05888347462741);
#17994=CIRCLE('',#46095,0.500000000000049);
#17995=CIRCLE('',#46096,0.500000000000049);
#17996=CIRCLE('',#46098,1.29583333162394);
#17997=CIRCLE('',#46099,1.29583333162394);
#17998=CIRCLE('',#46101,0.499999999999935);
#17999=CIRCLE('',#46102,0.499999999999935);
#18000=CIRCLE('',#46104,1.60653900437051);
#18001=CIRCLE('',#46105,1.60653900437051);
#18002=CIRCLE('',#46107,0.499999999999935);
#18003=CIRCLE('',#46108,0.499999999999935);
#18004=CIRCLE('',#46110,1.82809807486272);
#18005=CIRCLE('',#46111,1.82809807486273);
#18006=CIRCLE('',#46113,0.499999999999935);
#18007=CIRCLE('',#46114,0.499999999999935);
#18008=CIRCLE('',#46116,1.85841829658605);
#18009=CIRCLE('',#46117,1.85841829658605);
#18010=CIRCLE('',#46119,0.500000000000049);
#18011=CIRCLE('',#46120,0.500000000000049);
#18012=CIRCLE('',#46122,1.81285717707144);
#18013=CIRCLE('',#46123,1.81285717707144);
#18014=CIRCLE('',#46125,0.499999999999821);
#18015=CIRCLE('',#46126,0.499999999999821);
#18016=CIRCLE('',#46128,1.9114660202949);
#18017=CIRCLE('',#46129,1.9114660202949);
#18018=CIRCLE('',#46131,0.499999999999935);
#18019=CIRCLE('',#46132,0.499999999999935);
#18020=CIRCLE('',#46134,1.54967110260237);
#18021=CIRCLE('',#46135,1.54967110260237);
#18022=CIRCLE('',#46137,0.500000000000049);
#18023=CIRCLE('',#46138,0.500000000000049);
#18024=CIRCLE('',#46140,1.25936103546556);
#18025=CIRCLE('',#46141,1.25936103546568);
#18026=CIRCLE('',#46143,0.499999999999821);
#18027=CIRCLE('',#46144,0.499999999999821);
#18028=CIRCLE('',#46146,1.05888347462729);
#18029=CIRCLE('',#46147,1.0588834746273);
#18030=CIRCLE('',#46149,0.500000000000058);
#18031=CIRCLE('',#46150,0.500000000000058);
#18032=CIRCLE('',#46152,1.29583333162394);
#18033=CIRCLE('',#46153,1.29583333162394);
#18034=CIRCLE('',#46155,0.500000000000058);
#18035=CIRCLE('',#46156,0.500000000000058);
#18036=CIRCLE('',#46158,1.60653900437062);
#18037=CIRCLE('',#46159,1.60653900437062);
#18038=CIRCLE('',#46161,0.499999999999944);
#18039=CIRCLE('',#46162,0.499999999999944);
#18040=CIRCLE('',#46164,1.82809807486284);
#18041=CIRCLE('',#46165,1.82809807486284);
#18042=CIRCLE('',#46167,0.500000000000172);
#18043=CIRCLE('',#46168,0.500000000000172);
#18044=CIRCLE('',#46170,1.85841829658606);
#18045=CIRCLE('',#46171,1.85841829658606);
#18046=CIRCLE('',#46173,0.500000000000058);
#18047=CIRCLE('',#46174,0.500000000000058);
#18048=CIRCLE('',#46176,1.81285717707155);
#18049=CIRCLE('',#46177,1.81285717707155);
#18050=CIRCLE('',#46179,0.500000000000058);
#18051=CIRCLE('',#46180,0.500000000000058);
#18052=CIRCLE('',#46182,1.91146602029503);
#18053=CIRCLE('',#46183,1.91146602029503);
#18054=CIRCLE('',#46185,0.499999999999944);
#18055=CIRCLE('',#46186,0.499999999999944);
#18056=CIRCLE('',#46188,1.54967110260249);
#18057=CIRCLE('',#46189,1.5496711026025);
#18058=CIRCLE('',#46191,0.499999999999944);
#18059=CIRCLE('',#46192,0.499999999999944);
#18060=CIRCLE('',#46194,1.2593610354658);
#18061=CIRCLE('',#46195,1.25936103546556);
#18062=CIRCLE('',#46197,0.500000000000172);
#18063=CIRCLE('',#46198,0.500000000000172);
#18064=CIRCLE('',#46200,1.05888347462729);
#18065=CIRCLE('',#46201,1.05888347462729);
#18066=CIRCLE('',#46203,0.499999999999939);
#18067=CIRCLE('',#46204,0.499999999999935);
#18068=CIRCLE('',#46206,1.29583333162394);
#18069=CIRCLE('',#46207,1.29583333162394);
#18070=CIRCLE('',#46209,0.499999999999944);
#18071=CIRCLE('',#46210,0.499999999999944);
#18072=CIRCLE('',#46212,1.60653900437051);
#18073=CIRCLE('',#46213,1.60653900437051);
#18074=CIRCLE('',#46215,0.499999999999944);
#18075=CIRCLE('',#46216,0.499999999999944);
#18076=CIRCLE('',#46218,1.82809807486262);
#18077=CIRCLE('',#46219,1.82809807486262);
#18078=CIRCLE('',#46221,0.499999999999935);
#18079=CIRCLE('',#46222,0.499999999999935);
#18080=CIRCLE('',#46224,1.85841829658593);
#18081=CIRCLE('',#46225,1.85841829658593);
#18082=CIRCLE('',#46227,0.499999999999935);
#18083=CIRCLE('',#46228,0.499999999999935);
#18084=CIRCLE('',#46230,1.91146602029514);
#18085=CIRCLE('',#46231,1.91146602029514);
#18086=CIRCLE('',#46233,0.500000000000058);
#18087=CIRCLE('',#46234,0.500000000000058);
#18088=CIRCLE('',#46236,1.54967110260249);
#18089=CIRCLE('',#46237,1.54967110260249);
#18090=CIRCLE('',#46239,0.499999999999935);
#18091=CIRCLE('',#46240,0.499999999999935);
#18092=CIRCLE('',#46242,1.25936103546568);
#18093=CIRCLE('',#46243,1.2593610354658);
#18094=CIRCLE('',#46245,0.499999999999944);
#18095=CIRCLE('',#46246,0.499999999999944);
#18096=CIRCLE('',#46248,1.05888347462742);
#18097=CIRCLE('',#46249,1.05888347462742);
#18098=CIRCLE('',#46251,0.500000000000058);
#18099=CIRCLE('',#46252,0.500000000000058);
#18100=CIRCLE('',#46254,1.29583333162394);
#18101=CIRCLE('',#46255,1.29583333162395);
#18102=CIRCLE('',#46257,0.499999999999939);
#18103=CIRCLE('',#46258,0.499999999999944);
#18104=CIRCLE('',#46260,1.60653900437051);
#18105=CIRCLE('',#46261,1.60653900437051);
#18106=CIRCLE('',#46263,0.500000000000058);
#18107=CIRCLE('',#46264,0.500000000000058);
#18108=CIRCLE('',#46266,1.82809807486273);
#18109=CIRCLE('',#46267,1.82809807486273);
#18110=CIRCLE('',#46269,0.500000000000058);
#18111=CIRCLE('',#46270,0.500000000000058);
#18112=CIRCLE('',#46272,1.85841829658593);
#18113=CIRCLE('',#46273,1.85841829658594);
#18114=CIRCLE('',#46275,0.500000000000058);
#18115=CIRCLE('',#46276,0.500000000000058);
#18116=CIRCLE('',#46278,1.81285717707167);
#18117=CIRCLE('',#46279,1.81285717707167);
#18118=CIRCLE('',#46281,0.500000000000058);
#18119=CIRCLE('',#46282,0.500000000000058);
#18120=CIRCLE('',#46284,1.91146602029491);
#18121=CIRCLE('',#46285,1.91146602029491);
#18122=CIRCLE('',#46287,0.499999999999944);
#18123=CIRCLE('',#46288,0.499999999999944);
#18124=CIRCLE('',#46290,1.54967110260237);
#18125=CIRCLE('',#46291,1.54967110260237);
#18126=CIRCLE('',#46293,0.499999999999935);
#18127=CIRCLE('',#46294,0.499999999999935);
#18128=CIRCLE('',#46296,1.25936103546568);
#18129=CIRCLE('',#46297,1.25936103546556);
#18130=CIRCLE('',#46299,0.500000000000058);
#18131=CIRCLE('',#46300,0.500000000000058);
#18132=CIRCLE('',#46302,1.05888347462741);
#18133=CIRCLE('',#46303,1.05888347462741);
#18134=CIRCLE('',#46305,0.500000000000053);
#18135=CIRCLE('',#46306,0.500000000000058);
#18136=CIRCLE('',#46308,1.29583333162383);
#18137=CIRCLE('',#46309,1.29583333162383);
#18138=CIRCLE('',#46311,0.500000000000053);
#18139=CIRCLE('',#46312,0.500000000000058);
#18140=CIRCLE('',#46314,1.60653900437062);
#18141=CIRCLE('',#46315,1.60653900437062);
#18142=CIRCLE('',#46317,0.499999999999935);
#18143=CIRCLE('',#46318,0.499999999999935);
#18144=CIRCLE('',#46320,1.82809807486272);
#18145=CIRCLE('',#46321,1.82809807486272);
#18146=CIRCLE('',#46323,0.499999999999935);
#18147=CIRCLE('',#46324,0.499999999999935);
#18148=CIRCLE('',#46326,1.85841829658616);
#18149=CIRCLE('',#46327,1.85841829658616);
#18150=CIRCLE('',#46329,0.500000000000058);
#18151=CIRCLE('',#46330,0.500000000000058);
#18152=CIRCLE('',#46332,1.81285717707168);
#18153=CIRCLE('',#46333,1.81285717707168);
#18154=CIRCLE('',#46335,0.500000000000058);
#18155=CIRCLE('',#46336,0.500000000000049);
#18156=CIRCLE('',#46338,1.91146602029513);
#18157=CIRCLE('',#46339,1.91146602029514);
#18158=CIRCLE('',#46341,0.500000000000058);
#18159=CIRCLE('',#46342,0.500000000000058);
#18160=CIRCLE('',#46344,1.54967110260249);
#18161=CIRCLE('',#46345,1.5496711026025);
#18162=CIRCLE('',#46347,0.500000000000049);
#18163=CIRCLE('',#46348,0.500000000000049);
#18164=CIRCLE('',#46350,1.25936103546568);
#18165=CIRCLE('',#46351,1.25936103546568);
#18166=CIRCLE('',#46353,0.500000000000049);
#18167=CIRCLE('',#46354,0.500000000000049);
#18168=CIRCLE('',#46356,1.05888347462729);
#18169=CIRCLE('',#46357,1.05888347462729);
#18170=CIRCLE('',#46359,0.500000000000058);
#18171=CIRCLE('',#46360,0.500000000000058);
#18172=CIRCLE('',#46362,1.29583333162394);
#18173=CIRCLE('',#46363,1.29583333162394);
#18174=CIRCLE('',#46365,0.499999999999939);
#18175=CIRCLE('',#46366,0.499999999999944);
#18176=CIRCLE('',#46368,1.6065390043705);
#18177=CIRCLE('',#46369,1.60653900437051);
#18178=CIRCLE('',#46371,0.499999999999939);
#18179=CIRCLE('',#46372,0.499999999999944);
#18180=CIRCLE('',#46374,1.82809807486273);
#18181=CIRCLE('',#46375,1.82809807486273);
#18182=CIRCLE('',#46377,0.499999999999939);
#18183=CIRCLE('',#46378,0.499999999999935);
#18184=CIRCLE('',#46380,1.85841829658616);
#18185=CIRCLE('',#46381,1.85841829658616);
#18186=CIRCLE('',#46383,0.500000000000058);
#18187=CIRCLE('',#46384,0.500000000000049);
#18188=CIRCLE('',#46386,1.81285717707166);
#18189=CIRCLE('',#46387,1.81285717707167);
#18190=CIRCLE('',#46389,0.499999999999821);
#18191=CIRCLE('',#46390,0.499999999999821);
#18192=CIRCLE('',#46392,1.91146602029503);
#18193=CIRCLE('',#46393,1.91146602029503);
#18194=CIRCLE('',#46395,0.499999999999821);
#18195=CIRCLE('',#46396,0.499999999999821);
#18196=CIRCLE('',#46398,1.54967110260248);
#18197=CIRCLE('',#46399,1.54967110260248);
#18198=CIRCLE('',#46401,0.500000000000058);
#18199=CIRCLE('',#46402,0.500000000000058);
#18200=CIRCLE('',#46404,1.25936103546579);
#18201=CIRCLE('',#46405,1.25936103546568);
#18202=CIRCLE('',#46407,0.500000000000058);
#18203=CIRCLE('',#46408,0.500000000000058);
#18204=CIRCLE('',#46410,1.0588834746273);
#18205=CIRCLE('',#46411,1.0588834746273);
#18206=CIRCLE('',#46413,0.500000000000058);
#18207=CIRCLE('',#46414,0.500000000000058);
#18208=CIRCLE('',#46416,1.29583333162395);
#18209=CIRCLE('',#46417,1.29583333162395);
#18210=CIRCLE('',#46419,0.499999999999935);
#18211=CIRCLE('',#46420,0.499999999999935);
#18212=CIRCLE('',#46422,1.60653900437051);
#18213=CIRCLE('',#46423,1.60653900437051);
#18214=CIRCLE('',#46425,0.500000000000053);
#18215=CIRCLE('',#46426,0.500000000000049);
#18216=CIRCLE('',#46428,1.82809807486273);
#18217=CIRCLE('',#46429,1.82809807486273);
#18218=CIRCLE('',#46431,0.500000000000063);
#18219=CIRCLE('',#46432,0.500000000000058);
#18220=CIRCLE('',#46434,1.85841829658604);
#18221=CIRCLE('',#46435,1.85841829658605);
#18222=CIRCLE('',#46437,0.499999999999821);
#18223=CIRCLE('',#46438,0.499999999999821);
#18224=CIRCLE('',#46440,1.81285717707144);
#18225=CIRCLE('',#46441,1.81285717707144);
#18226=CIRCLE('',#46443,0.499999999999821);
#18227=CIRCLE('',#46444,0.499999999999821);
#18228=CIRCLE('',#46446,1.91146602029503);
#18229=CIRCLE('',#46447,1.91146602029503);
#18230=CIRCLE('',#46449,0.500000000000058);
#18231=CIRCLE('',#46450,0.500000000000058);
#18232=CIRCLE('',#46452,1.54967110260248);
#18233=CIRCLE('',#46453,1.54967110260249);
#18234=CIRCLE('',#46455,0.499999999999944);
#18235=CIRCLE('',#46456,0.499999999999944);
#18236=CIRCLE('',#46458,1.25936103546569);
#18237=CIRCLE('',#46459,1.25936103546568);
#18238=CIRCLE('',#46461,0.499999999999944);
#18239=CIRCLE('',#46462,0.499999999999944);
#18240=CIRCLE('',#46464,1.0588834746273);
#18241=CIRCLE('',#46465,1.0588834746273);
#18242=CIRCLE('',#46467,0.500000000000053);
#18243=CIRCLE('',#46468,0.500000000000054);
#18244=CIRCLE('',#46470,1.29583333162382);
#18245=CIRCLE('',#46471,1.29583333162382);
#18246=CIRCLE('',#46473,0.499999999999826);
#18247=CIRCLE('',#46474,0.499999999999826);
#18248=CIRCLE('',#46476,1.60653900437062);
#18249=CIRCLE('',#46477,1.60653900437062);
#18250=CIRCLE('',#46479,0.500000000000058);
#18251=CIRCLE('',#46480,0.500000000000058);
#18252=CIRCLE('',#46482,1.82809807486273);
#18253=CIRCLE('',#46483,1.82809807486272);
#18254=CIRCLE('',#46485,0.499999999999944);
#18255=CIRCLE('',#46486,0.499999999999944);
#18256=CIRCLE('',#46488,1.85841829658604);
#18257=CIRCLE('',#46489,1.85841829658605);
#18258=CIRCLE('',#46491,0.499999999999939);
#18259=CIRCLE('',#46492,0.499999999999939);
#18260=CIRCLE('',#46494,1.9114660202949);
#18261=CIRCLE('',#46495,1.9114660202949);
#18262=CIRCLE('',#46497,0.499999999999821);
#18263=CIRCLE('',#46498,0.499999999999821);
#18264=CIRCLE('',#46500,1.54967110260249);
#18265=CIRCLE('',#46501,1.54967110260249);
#18266=CIRCLE('',#46503,0.500000000000053);
#18267=CIRCLE('',#46504,0.500000000000049);
#18268=CIRCLE('',#46506,1.25936103546569);
#18269=CIRCLE('',#46507,1.25936103546556);
#18270=CIRCLE('',#46509,0.499999999999935);
#18271=CIRCLE('',#46510,0.499999999999935);
#18272=CIRCLE('',#46512,1.05888347462729);
#18273=CIRCLE('',#46513,1.05888347462729);
#18274=CIRCLE('',#46515,0.500000000000053);
#18275=CIRCLE('',#46516,0.500000000000054);
#18276=CIRCLE('',#46518,1.29583333162382);
#18277=CIRCLE('',#46519,1.29583333162371);
#18278=CIRCLE('',#46521,0.499999999999935);
#18279=CIRCLE('',#46522,0.499999999999935);
#18280=CIRCLE('',#46524,1.60653900437051);
#18281=CIRCLE('',#46525,1.60653900437051);
#18282=CIRCLE('',#46527,0.499999999999944);
#18283=CIRCLE('',#46528,0.499999999999939);
#18284=CIRCLE('',#46530,1.82809807486262);
#18285=CIRCLE('',#46531,1.82809807486262);
#18286=CIRCLE('',#46533,0.500000000000058);
#18287=CIRCLE('',#46534,0.500000000000058);
#18288=CIRCLE('',#46536,1.85841829658605);
#18289=CIRCLE('',#46537,1.85841829658605);
#18290=CIRCLE('',#46539,0.499999999999944);
#18291=CIRCLE('',#46540,0.499999999999939);
#18292=CIRCLE('',#46542,1.81285717707166);
#18293=CIRCLE('',#46543,1.81285717707166);
#18294=CIRCLE('',#46545,0.499999999999944);
#18295=CIRCLE('',#46546,0.499999999999944);
#18296=CIRCLE('',#46548,1.91146602029514);
#18297=CIRCLE('',#46549,1.91146602029514);
#18298=CIRCLE('',#46551,0.500000000000053);
#18299=CIRCLE('',#46552,0.500000000000054);
#18300=CIRCLE('',#46554,1.54967110260238);
#18301=CIRCLE('',#46555,1.54967110260238);
#18302=CIRCLE('',#46557,0.499999999999935);
#18303=CIRCLE('',#46558,0.499999999999935);
#18304=CIRCLE('',#46560,1.25936103546569);
#18305=CIRCLE('',#46561,1.25936103546579);
#18306=CIRCLE('',#46563,0.499999999999939);
#18307=CIRCLE('',#46564,0.499999999999944);
#18308=CIRCLE('',#46566,1.0588834746273);
#18309=CIRCLE('',#46567,1.0588834746273);
#18310=CIRCLE('',#46569,0.499999999999944);
#18311=CIRCLE('',#46570,0.499999999999944);
#18312=CIRCLE('',#46572,1.29583333162395);
#18313=CIRCLE('',#46573,1.29583333162395);
#18314=CIRCLE('',#46575,0.500000000000053);
#18315=CIRCLE('',#46576,0.500000000000054);
#18316=CIRCLE('',#46578,1.60653900437062);
#18317=CIRCLE('',#46579,1.60653900437063);
#18318=CIRCLE('',#46581,0.500000000000053);
#18319=CIRCLE('',#46582,0.500000000000054);
#18320=CIRCLE('',#46584,1.82809807486273);
#18321=CIRCLE('',#46585,1.82809807486273);
#18322=CIRCLE('',#46587,0.500000000000058);
#18323=CIRCLE('',#46588,0.500000000000058);
#18324=CIRCLE('',#46590,1.85841829658593);
#18325=CIRCLE('',#46591,1.85841829658594);
#18326=CIRCLE('',#46593,0.499999999999939);
#18327=CIRCLE('',#46594,0.499999999999939);
#18328=CIRCLE('',#46596,1.81285717707155);
#18329=CIRCLE('',#46597,1.81285717707156);
#18330=CIRCLE('',#46599,0.500000000000058);
#18331=CIRCLE('',#46600,0.500000000000058);
#18332=CIRCLE('',#46602,1.91146602029491);
#18333=CIRCLE('',#46603,1.91146602029491);
#18334=CIRCLE('',#46605,0.500000000000053);
#18335=CIRCLE('',#46606,0.500000000000054);
#18336=CIRCLE('',#46608,1.54967110260249);
#18337=CIRCLE('',#46609,1.54967110260249);
#18338=CIRCLE('',#46611,0.499999999999944);
#18339=CIRCLE('',#46612,0.499999999999944);
#18340=CIRCLE('',#46614,1.25936103546568);
#18341=CIRCLE('',#46615,1.25936103546569);
#18342=CIRCLE('',#46617,0.500000000000058);
#18343=CIRCLE('',#46618,0.500000000000058);
#18344=CIRCLE('',#46620,1.0588834746273);
#18345=CIRCLE('',#46621,1.0588834746273);
#18346=CIRCLE('',#46623,0.500000000000053);
#18347=CIRCLE('',#46624,0.500000000000054);
#18348=CIRCLE('',#46626,1.29583333162394);
#18349=CIRCLE('',#46627,1.29583333162394);
#18350=CIRCLE('',#46629,0.500000000000053);
#18351=CIRCLE('',#46630,0.500000000000054);
#18352=CIRCLE('',#46632,1.60653900437062);
#18353=CIRCLE('',#46633,1.60653900437062);
#18354=CIRCLE('',#46635,0.500000000000053);
#18355=CIRCLE('',#46636,0.500000000000054);
#18356=CIRCLE('',#46638,1.82809807486273);
#18357=CIRCLE('',#46639,1.82809807486272);
#18358=CIRCLE('',#46641,0.499999999999944);
#18359=CIRCLE('',#46642,0.499999999999944);
#18360=CIRCLE('',#46644,1.85841829658605);
#18361=CIRCLE('',#46645,1.85841829658605);
#18362=CIRCLE('',#46647,0.500000000000053);
#18363=CIRCLE('',#46648,0.500000000000054);
#18364=CIRCLE('',#46650,1.81285717707167);
#18365=CIRCLE('',#46651,1.81285717707167);
#18366=CIRCLE('',#46653,0.500000000000053);
#18367=CIRCLE('',#46654,0.500000000000054);
#18368=CIRCLE('',#46656,1.91146602029503);
#18369=CIRCLE('',#46657,1.91146602029503);
#18370=CIRCLE('',#46659,0.500000000000049);
#18371=CIRCLE('',#46660,0.500000000000049);
#18372=CIRCLE('',#46662,1.54967110260249);
#18373=CIRCLE('',#46663,1.54967110260249);
#18374=CIRCLE('',#46665,0.499999999999944);
#18375=CIRCLE('',#46666,0.499999999999944);
#18376=CIRCLE('',#46668,1.25936103546568);
#18377=CIRCLE('',#46669,1.25936103546568);
#18378=CIRCLE('',#46671,0.500000000000053);
#18379=CIRCLE('',#46672,0.500000000000054);
#18380=CIRCLE('',#46674,1.0588834746274);
#18381=CIRCLE('',#46675,1.0588834746274);
#18382=CIRCLE('',#46677,0.499999999999944);
#18383=CIRCLE('',#46678,0.499999999999944);
#18384=CIRCLE('',#46680,1.29583333162394);
#18385=CIRCLE('',#46681,1.29583333162394);
#18386=CIRCLE('',#46683,0.500000000000053);
#18387=CIRCLE('',#46684,0.500000000000054);
#18388=CIRCLE('',#46686,1.60653900437062);
#18389=CIRCLE('',#46687,1.60653900437062);
#18390=CIRCLE('',#46689,0.500000000000053);
#18391=CIRCLE('',#46690,0.500000000000054);
#18392=CIRCLE('',#46692,1.82809807486272);
#18393=CIRCLE('',#46693,1.82809807486272);
#18394=CIRCLE('',#46695,0.500000000000053);
#18395=CIRCLE('',#46696,0.500000000000054);
#18396=CIRCLE('',#46698,1.85841829658605);
#18397=CIRCLE('',#46699,1.85841829658605);
#18398=CIRCLE('',#46701,0.500000000000049);
#18399=CIRCLE('',#46702,0.500000000000049);
#18400=CIRCLE('',#46704,1.81285717707167);
#18401=CIRCLE('',#46705,1.81285717707167);
#18402=CIRCLE('',#46707,0.500000000000053);
#18403=CIRCLE('',#46708,0.500000000000054);
#18404=CIRCLE('',#46710,1.91146602029502);
#18405=CIRCLE('',#46711,1.91146602029502);
#18406=CIRCLE('',#46713,0.500000000000053);
#18407=CIRCLE('',#46714,0.500000000000049);
#18408=CIRCLE('',#46716,1.54967110260249);
#18409=CIRCLE('',#46717,1.54967110260249);
#18410=CIRCLE('',#46719,0.500000000000053);
#18411=CIRCLE('',#46720,0.500000000000049);
#18412=CIRCLE('',#46722,1.25936103546568);
#18413=CIRCLE('',#46723,1.25936103546557);
#18414=CIRCLE('',#46725,0.499999999999944);
#18415=CIRCLE('',#46726,0.499999999999944);
#18416=CIRCLE('',#46728,1.0588834746274);
#18417=CIRCLE('',#46729,1.05888347462741);
#18418=CIRCLE('',#46731,0.500000000000053);
#18419=CIRCLE('',#46732,0.500000000000054);
#18420=CIRCLE('',#46734,1.29583333162394);
#18421=CIRCLE('',#46735,1.29583333162394);
#18422=CIRCLE('',#46737,0.500000000000053);
#18423=CIRCLE('',#46738,0.500000000000054);
#18424=CIRCLE('',#46740,1.60653900437062);
#18425=CIRCLE('',#46741,1.60653900437062);
#18426=CIRCLE('',#46743,0.500000000000053);
#18427=CIRCLE('',#46744,0.500000000000054);
#18428=CIRCLE('',#46746,1.82809807486262);
#18429=CIRCLE('',#46747,1.82809807486262);
#18430=CIRCLE('',#46749,0.499999999999939);
#18431=CIRCLE('',#46750,0.499999999999939);
#18432=CIRCLE('',#46752,1.85841829658605);
#18433=CIRCLE('',#46753,1.85841829658605);
#18434=CIRCLE('',#46755,0.500000000000053);
#18435=CIRCLE('',#46756,0.500000000000054);
#18436=CIRCLE('',#46758,1.91146602029503);
#18437=CIRCLE('',#46759,1.91146602029503);
#18438=CIRCLE('',#46761,0.500000000000053);
#18439=CIRCLE('',#46762,0.500000000000054);
#18440=CIRCLE('',#46764,1.54967110260249);
#18441=CIRCLE('',#46765,1.54967110260249);
#18442=CIRCLE('',#46767,0.500000000000053);
#18443=CIRCLE('',#46768,0.500000000000054);
#18444=CIRCLE('',#46770,1.25936103546568);
#18445=CIRCLE('',#46771,1.25936103546568);
#18446=CIRCLE('',#46773,0.500000000000053);
#18447=CIRCLE('',#46774,0.500000000000054);
#18448=CIRCLE('',#46776,1.05888347462729);
#18449=CIRCLE('',#46777,1.05888347462729);
#18450=CIRCLE('',#46779,0.499999999999935);
#18451=CIRCLE('',#46780,0.499999999999935);
#18452=CIRCLE('',#46782,1.29583333162395);
#18453=CIRCLE('',#46783,1.29583333162395);
#18454=CIRCLE('',#46785,0.500000000000063);
#18455=CIRCLE('',#46786,0.500000000000063);
#18456=CIRCLE('',#46788,1.60653900437062);
#18457=CIRCLE('',#46789,1.60653900437062);
#18458=CIRCLE('',#46791,0.500000000000053);
#18459=CIRCLE('',#46792,0.500000000000054);
#18460=CIRCLE('',#46794,1.82809807486273);
#18461=CIRCLE('',#46795,1.82809807486273);
#18462=CIRCLE('',#46797,0.500000000000058);
#18463=CIRCLE('',#46798,0.500000000000058);
#18464=CIRCLE('',#46800,1.85841829658605);
#18465=CIRCLE('',#46801,1.85841829658605);
#18466=CIRCLE('',#46803,0.499999999999939);
#18467=CIRCLE('',#46804,0.499999999999939);
#18468=CIRCLE('',#46806,1.81285717707167);
#18469=CIRCLE('',#46807,1.81285717707167);
#18470=CIRCLE('',#46809,0.499999999999939);
#18471=CIRCLE('',#46810,0.499999999999939);
#18472=CIRCLE('',#46812,1.91146602029491);
#18473=CIRCLE('',#46813,1.91146602029491);
#18474=CIRCLE('',#46815,0.499999999999826);
#18475=CIRCLE('',#46816,0.499999999999826);
#18476=CIRCLE('',#46818,1.5496711026025);
#18477=CIRCLE('',#46819,1.54967110260249);
#18478=CIRCLE('',#46821,0.500000000000053);
#18479=CIRCLE('',#46822,0.500000000000054);
#18480=CIRCLE('',#46824,1.25936103546579);
#18481=CIRCLE('',#46825,1.25936103546568);
#18482=CIRCLE('',#46826,1.25936103546568);
#18483=CIRCLE('',#46828,0.500000000000063);
#18484=CIRCLE('',#46829,0.500000000000058);
#18485=CIRCLE('',#46831,1.0588834746273);
#18486=CIRCLE('',#46832,1.0588834746273);
#18487=CIRCLE('',#46834,0.499999999999935);
#18488=CIRCLE('',#46835,0.499999999999935);
#18489=CIRCLE('',#46837,1.29583333162395);
#18490=CIRCLE('',#46838,1.29583333162395);
#18491=CIRCLE('',#46840,0.500000000000053);
#18492=CIRCLE('',#46841,0.500000000000054);
#18493=CIRCLE('',#46843,1.60653900437074);
#18494=CIRCLE('',#46844,1.60653900437074);
#18495=CIRCLE('',#46846,0.500000000000058);
#18496=CIRCLE('',#46847,0.500000000000058);
#18497=CIRCLE('',#46849,1.82809807486273);
#18498=CIRCLE('',#46850,1.82809807486272);
#18499=CIRCLE('',#46852,0.500000000000053);
#18500=CIRCLE('',#46853,0.500000000000054);
#18501=CIRCLE('',#46855,1.85841829658616);
#18502=CIRCLE('',#46856,1.85841829658616);
#18503=CIRCLE('',#46858,0.500000000000167);
#18504=CIRCLE('',#46859,0.500000000000167);
#18505=CIRCLE('',#46861,1.81285717707155);
#18506=CIRCLE('',#46862,1.81285717707155);
#18507=CIRCLE('',#46864,0.499999999999935);
#18508=CIRCLE('',#46865,0.499999999999935);
#18509=CIRCLE('',#46867,1.91146602029503);
#18510=CIRCLE('',#46868,1.91146602029503);
#18511=CIRCLE('',#46870,0.500000000000053);
#18512=CIRCLE('',#46871,0.500000000000054);
#18513=CIRCLE('',#46873,1.54967110260249);
#18514=CIRCLE('',#46874,1.54967110260249);
#18515=CIRCLE('',#46875,1.54967110260249);
#18516=CIRCLE('',#46877,0.499999999999939);
#18517=CIRCLE('',#46878,0.499999999999939);
#18518=CIRCLE('',#46880,1.25936103546556);
#18519=CIRCLE('',#46881,1.25936103546568);
#18520=CIRCLE('',#46882,1.25936103546568);
#18521=CIRCLE('',#46884,0.499999999999821);
#18522=CIRCLE('',#46885,0.499999999999821);
#18523=CIRCLE('',#46887,1.05888347462729);
#18524=CIRCLE('',#46888,1.05888347462729);
#18525=CIRCLE('',#46890,0.500000000000058);
#18526=CIRCLE('',#46891,0.500000000000058);
#18527=CIRCLE('',#46893,1.29583333162382);
#18528=CIRCLE('',#46894,1.29583333162382);
#18529=CIRCLE('',#46896,0.500000000000053);
#18530=CIRCLE('',#46897,0.500000000000054);
#18531=CIRCLE('',#46899,1.60653900437074);
#18532=CIRCLE('',#46900,1.60653900437074);
#18533=CIRCLE('',#46902,0.500000000000063);
#18534=CIRCLE('',#46903,0.500000000000063);
#18535=CIRCLE('',#46905,1.82809807486273);
#18536=CIRCLE('',#46906,1.82809807486272);
#18537=CIRCLE('',#46908,0.500000000000053);
#18538=CIRCLE('',#46909,0.500000000000054);
#18539=CIRCLE('',#46911,1.85841829658605);
#18540=CIRCLE('',#46912,1.85841829658605);
#18541=CIRCLE('',#46914,0.500000000000049);
#18542=CIRCLE('',#46915,0.500000000000049);
#18543=CIRCLE('',#46917,1.81285717707166);
#18544=CIRCLE('',#46918,1.81285717707166);
#18545=CIRCLE('',#46920,0.500000000000049);
#18546=CIRCLE('',#46921,0.500000000000049);
#18547=CIRCLE('',#46923,1.91146602029503);
#18548=CIRCLE('',#46924,1.91146602029503);
#18549=CIRCLE('',#46925,1.91146602029503);
#18550=CIRCLE('',#46927,0.500000000000053);
#18551=CIRCLE('',#46928,0.500000000000054);
#18552=CIRCLE('',#46930,1.0588834746274);
#18553=CIRCLE('',#46931,1.0588834746274);
#18554=CIRCLE('',#46933,0.500000000000058);
#18555=CIRCLE('',#46934,0.500000000000058);
#18556=CIRCLE('',#46936,1.29583333162394);
#18557=CIRCLE('',#46937,1.29583333162395);
#18558=CIRCLE('',#46939,0.500000000000058);
#18559=CIRCLE('',#46940,0.500000000000058);
#18560=CIRCLE('',#46942,1.60653900437063);
#18561=CIRCLE('',#46943,1.60653900437063);
#18562=CIRCLE('',#46945,0.500000000000058);
#18563=CIRCLE('',#46946,0.500000000000058);
#18564=CIRCLE('',#46948,1.82809807486273);
#18565=CIRCLE('',#46949,1.82809807486273);
#18566=CIRCLE('',#46951,0.499999999999939);
#18567=CIRCLE('',#46952,0.499999999999939);
#18568=CIRCLE('',#46954,1.85841829658605);
#18569=CIRCLE('',#46955,1.85841829658605);
#18570=CIRCLE('',#46957,0.499999999999935);
#18571=CIRCLE('',#46958,0.499999999999935);
#18572=CIRCLE('',#46960,1.81285717707167);
#18573=CIRCLE('',#46961,1.81285717707167);
#18574=CIRCLE('',#46963,0.499999999999944);
#18575=CIRCLE('',#46964,0.499999999999944);
#18576=CIRCLE('',#46966,1.91146602029514);
#18577=CIRCLE('',#46967,1.91146602029503);
#18578=CIRCLE('',#46969,0.500000000000167);
#18579=CIRCLE('',#46970,0.500000000000167);
#18580=CIRCLE('',#46972,1.05888347462729);
#18581=CIRCLE('',#46973,1.0588834746273);
#18582=CIRCLE('',#46975,0.499999999999944);
#18583=CIRCLE('',#46976,0.499999999999944);
#18584=CIRCLE('',#46978,1.29583333162394);
#18585=CIRCLE('',#46979,1.29583333162394);
#18586=CIRCLE('',#46981,0.500000000000053);
#18587=CIRCLE('',#46982,0.500000000000049);
#18588=CIRCLE('',#46984,1.60653900437062);
#18589=CIRCLE('',#46985,1.60653900437062);
#18590=CIRCLE('',#46987,0.499999999999944);
#18591=CIRCLE('',#46988,0.499999999999944);
#18592=CIRCLE('',#46990,1.82809807486273);
#18593=CIRCLE('',#46991,1.82809807486273);
#18594=CIRCLE('',#46993,0.499999999999944);
#18595=CIRCLE('',#46994,0.499999999999944);
#18596=CIRCLE('',#46996,1.85841829658605);
#18597=CIRCLE('',#46997,1.85841829658605);
#18598=CIRCLE('',#46999,0.499999999999944);
#18599=CIRCLE('',#47000,0.499999999999944);
#18600=CIRCLE('',#47002,1.91146602029502);
#18601=CIRCLE('',#47003,1.91146602029503);
#18602=CIRCLE('',#47005,0.500000000000058);
#18603=CIRCLE('',#47006,0.500000000000054);
#18604=CIRCLE('',#47008,1.54967110260249);
#18605=CIRCLE('',#47009,1.54967110260261);
#18606=CIRCLE('',#47010,1.54967110260261);
#18607=CIRCLE('',#47012,0.499999999999939);
#18608=CIRCLE('',#47013,0.499999999999939);
#18609=CIRCLE('',#47015,1.05888347462741);
#18610=CIRCLE('',#47016,1.05888347462741);
#18611=CIRCLE('',#47018,0.499999999999939);
#18612=CIRCLE('',#47019,0.499999999999939);
#18613=CIRCLE('',#47021,1.29583333162394);
#18614=CIRCLE('',#47022,1.29583333162394);
#18615=CIRCLE('',#47024,0.499999999999939);
#18616=CIRCLE('',#47025,0.499999999999939);
#18617=CIRCLE('',#47027,1.60653900437063);
#18618=CIRCLE('',#47028,1.60653900437063);
#18619=CIRCLE('',#47030,0.500000000000058);
#18620=CIRCLE('',#47031,0.500000000000058);
#18621=CIRCLE('',#47033,1.82809807486273);
#18622=CIRCLE('',#47034,1.82809807486273);
#18623=CIRCLE('',#47036,0.500000000000058);
#18624=CIRCLE('',#47037,0.500000000000058);
#18625=CIRCLE('',#47039,1.85841829658593);
#18626=CIRCLE('',#47040,1.85841829658593);
#18627=CIRCLE('',#47042,0.499999999999939);
#18628=CIRCLE('',#47043,0.499999999999939);
#18629=CIRCLE('',#47045,1.81285717707154);
#18630=CIRCLE('',#47046,1.81285717707155);
#18631=CIRCLE('',#47048,0.499999999999939);
#18632=CIRCLE('',#47049,0.499999999999939);
#18633=CIRCLE('',#47051,1.91146602029503);
#18634=CIRCLE('',#47052,1.91146602029503);
#18635=CIRCLE('',#47054,0.499999999999939);
#18636=CIRCLE('',#47055,0.499999999999939);
#18637=CIRCLE('',#47057,1.54967110260237);
#18638=CIRCLE('',#47058,1.54967110260237);
#18639=CIRCLE('',#47060,0.499999999999939);
#18640=CIRCLE('',#47061,0.499999999999939);
#18641=CIRCLE('',#47063,1.05888347462729);
#18642=CIRCLE('',#47064,1.05888347462729);
#18643=CIRCLE('',#47066,0.500000000000053);
#18644=CIRCLE('',#47067,0.500000000000054);
#18645=CIRCLE('',#47069,1.29583333162383);
#18646=CIRCLE('',#47070,1.29583333162383);
#18647=CIRCLE('',#47072,0.500000000000053);
#18648=CIRCLE('',#47073,0.500000000000054);
#18649=CIRCLE('',#47075,1.60653900437051);
#18650=CIRCLE('',#47076,1.60653900437051);
#18651=CIRCLE('',#47078,0.499999999999935);
#18652=CIRCLE('',#47079,0.499999999999935);
#18653=CIRCLE('',#47081,1.82809807486262);
#18654=CIRCLE('',#47082,1.82809807486262);
#18655=CIRCLE('',#47084,0.500000000000063);
#18656=CIRCLE('',#47085,0.500000000000063);
#18657=CIRCLE('',#47087,1.85841829658605);
#18658=CIRCLE('',#47088,1.85841829658605);
#18659=CIRCLE('',#47090,0.500000000000053);
#18660=CIRCLE('',#47091,0.500000000000054);
#18661=CIRCLE('',#47093,1.81285717707166);
#18662=CIRCLE('',#47094,1.81285717707166);
#18663=CIRCLE('',#47096,0.499999999999935);
#18664=CIRCLE('',#47097,0.499999999999935);
#18665=CIRCLE('',#47099,1.9114660202949);
#18666=CIRCLE('',#47100,1.9114660202949);
#18667=CIRCLE('',#47102,0.499999999999935);
#18668=CIRCLE('',#47103,0.499999999999935);
#18669=CIRCLE('',#47105,1.54967110260248);
#18670=CIRCLE('',#47106,1.54967110260249);
#18671=CIRCLE('',#47108,0.499999999999935);
#18672=CIRCLE('',#47109,0.499999999999935);
#18673=CIRCLE('',#47111,1.25936103546556);
#18674=CIRCLE('',#47112,1.25936103546569);
#18675=CIRCLE('',#47113,1.25936103546569);
#18676=CIRCLE('',#47115,0.499999999999935);
#18677=CIRCLE('',#47116,0.499999999999935);
#18678=CIRCLE('',#47118,1.05888347462741);
#18679=CIRCLE('',#47119,1.05888347462741);
#18680=CIRCLE('',#47121,0.500000000000058);
#18681=CIRCLE('',#47122,0.500000000000058);
#18682=CIRCLE('',#47124,1.29583333162406);
#18683=CIRCLE('',#47125,1.29583333162406);
#18684=CIRCLE('',#47127,0.499999999999939);
#18685=CIRCLE('',#47128,0.499999999999944);
#18686=CIRCLE('',#47130,1.60653900437063);
#18687=CIRCLE('',#47131,1.60653900437063);
#18688=CIRCLE('',#47133,0.500000000000058);
#18689=CIRCLE('',#47134,0.500000000000058);
#18690=CIRCLE('',#47136,1.82809807486262);
#18691=CIRCLE('',#47137,1.82809807486262);
#18692=CIRCLE('',#47139,0.499999999999939);
#18693=CIRCLE('',#47140,0.499999999999939);
#18694=CIRCLE('',#47142,1.85841829658593);
#18695=CIRCLE('',#47143,1.85841829658593);
#18696=CIRCLE('',#47145,0.499999999999939);
#18697=CIRCLE('',#47146,0.499999999999939);
#18698=CIRCLE('',#47148,1.81285717707178);
#18699=CIRCLE('',#47149,1.81285717707179);
#18700=CIRCLE('',#47151,0.499999999999939);
#18701=CIRCLE('',#47152,0.499999999999939);
#18702=CIRCLE('',#47154,1.91146602029502);
#18703=CIRCLE('',#47155,1.91146602029502);
#18704=CIRCLE('',#47157,0.499999999999939);
#18705=CIRCLE('',#47158,0.499999999999939);
#18706=CIRCLE('',#47160,1.54967110260249);
#18707=CIRCLE('',#47161,1.54967110260249);
#18708=CIRCLE('',#47163,0.500000000000058);
#18709=CIRCLE('',#47164,0.500000000000058);
#18710=CIRCLE('',#47166,1.25936103546568);
#18711=CIRCLE('',#47167,1.25936103546556);
#18712=CIRCLE('',#47168,1.25936103546556);
#18713=CIRCLE('',#47170,0.499999999999935);
#18714=CIRCLE('',#47171,0.499999999999935);
#18715=CIRCLE('',#47173,1.05888347462729);
#18716=CIRCLE('',#47174,1.0588834746273);
#18717=CIRCLE('',#47176,0.500000000000053);
#18718=CIRCLE('',#47177,0.500000000000058);
#18719=CIRCLE('',#47179,1.29583333162406);
#18720=CIRCLE('',#47180,1.29583333162406);
#18721=CIRCLE('',#47182,0.500000000000177);
#18722=CIRCLE('',#47183,0.500000000000181);
#18723=CIRCLE('',#47185,1.60653900437051);
#18724=CIRCLE('',#47186,1.60653900437051);
#18725=CIRCLE('',#47188,0.499999999999939);
#18726=CIRCLE('',#47189,0.499999999999944);
#18727=CIRCLE('',#47191,1.82809807486261);
#18728=CIRCLE('',#47192,1.82809807486261);
#18729=CIRCLE('',#47194,0.499999999999944);
#18730=CIRCLE('',#47195,0.499999999999944);
#18731=CIRCLE('',#47197,1.85841829658594);
#18732=CIRCLE('',#47198,1.85841829658594);
#18733=CIRCLE('',#47200,0.499999999999939);
#18734=CIRCLE('',#47201,0.499999999999939);
#18735=CIRCLE('',#47203,1.81285717707156);
#18736=CIRCLE('',#47204,1.81285717707156);
#18737=CIRCLE('',#47206,0.499999999999944);
#18738=CIRCLE('',#47207,0.499999999999939);
#18739=CIRCLE('',#47209,1.91146602029503);
#18740=CIRCLE('',#47210,1.91146602029503);
#18741=CIRCLE('',#47212,0.500000000000053);
#18742=CIRCLE('',#47213,0.500000000000054);
#18743=CIRCLE('',#47215,1.5496711026026);
#18744=CIRCLE('',#47216,1.5496711026026);
#18745=CIRCLE('',#47218,0.500000000000058);
#18746=CIRCLE('',#47219,0.500000000000058);
#18747=CIRCLE('',#47221,1.2593610354658);
#18748=CIRCLE('',#47222,1.25936103546556);
#18749=CIRCLE('',#47224,0.500000000000063);
#18750=CIRCLE('',#47225,0.500000000000063);
#18751=CIRCLE('',#47227,1.05888347462741);
#18752=CIRCLE('',#47228,1.05888347462741);
#18753=CIRCLE('',#47230,0.499999999999939);
#18754=CIRCLE('',#47231,0.499999999999944);
#18755=CIRCLE('',#47233,1.29583333162395);
#18756=CIRCLE('',#47234,1.29583333162395);
#18757=CIRCLE('',#47236,0.500000000000053);
#18758=CIRCLE('',#47237,0.500000000000049);
#18759=CIRCLE('',#47239,1.60653900437063);
#18760=CIRCLE('',#47240,1.60653900437063);
#18761=CIRCLE('',#47242,0.500000000000167);
#18762=CIRCLE('',#47243,0.500000000000172);
#18763=CIRCLE('',#47245,1.82809807486262);
#18764=CIRCLE('',#47246,1.82809807486262);
#18765=CIRCLE('',#47248,0.499999999999944);
#18766=CIRCLE('',#47249,0.499999999999944);
#18767=CIRCLE('',#47251,1.85841829658604);
#18768=CIRCLE('',#47252,1.85841829658605);
#18769=CIRCLE('',#47254,0.499999999999944);
#18770=CIRCLE('',#47255,0.499999999999944);
#18771=CIRCLE('',#47257,1.91146602029502);
#18772=CIRCLE('',#47258,1.91146602029502);
#18773=CIRCLE('',#47260,0.499999999999944);
#18774=CIRCLE('',#47261,0.499999999999944);
#18775=CIRCLE('',#47263,1.5496711026026);
#18776=CIRCLE('',#47264,1.5496711026026);
#18777=CIRCLE('',#47266,0.500000000000053);
#18778=CIRCLE('',#47267,0.500000000000049);
#18779=CIRCLE('',#47269,1.25936103546567);
#18780=CIRCLE('',#47270,1.25936103546556);
#18781=CIRCLE('',#47272,0.499999999999939);
#18782=CIRCLE('',#47273,0.499999999999939);
#18783=CIRCLE('',#47275,1.05888347462741);
#18784=CIRCLE('',#47276,1.05888347462741);
#18785=CIRCLE('',#47278,0.500000000000053);
#18786=CIRCLE('',#47279,0.500000000000049);
#18787=CIRCLE('',#47281,1.29583333162394);
#18788=CIRCLE('',#47282,1.29583333162394);
#18789=CIRCLE('',#47284,0.499999999999939);
#18790=CIRCLE('',#47285,0.499999999999944);
#18791=CIRCLE('',#47287,1.6065390043705);
#18792=CIRCLE('',#47288,1.6065390043705);
#18793=CIRCLE('',#47290,0.499999999999939);
#18794=CIRCLE('',#47291,0.499999999999935);
#18795=CIRCLE('',#47293,1.82809807486262);
#18796=CIRCLE('',#47294,1.82809807486262);
#18797=CIRCLE('',#47296,0.500000000000053);
#18798=CIRCLE('',#47297,0.500000000000058);
#18799=CIRCLE('',#47299,1.85841829658593);
#18800=CIRCLE('',#47300,1.85841829658593);
#18801=CIRCLE('',#47302,0.499999999999939);
#18802=CIRCLE('',#47303,0.499999999999944);
#18803=CIRCLE('',#47305,1.81285717707167);
#18804=CIRCLE('',#47306,1.81285717707168);
#18805=CIRCLE('',#47308,0.500000000000058);
#18806=CIRCLE('',#47309,0.500000000000058);
#18807=CIRCLE('',#47311,1.91146602029503);
#18808=CIRCLE('',#47312,1.91146602029503);
#18809=CIRCLE('',#47314,0.500000000000053);
#18810=CIRCLE('',#47315,0.500000000000049);
#18811=CIRCLE('',#47317,1.54967110260249);
#18812=CIRCLE('',#47318,1.54967110260249);
#18813=CIRCLE('',#47320,0.500000000000058);
#18814=CIRCLE('',#47321,0.500000000000058);
#18815=CIRCLE('',#47323,1.25936103546568);
#18816=CIRCLE('',#47324,1.25936103546557);
#18817=CIRCLE('',#47326,0.499999999999939);
#18818=CIRCLE('',#47327,0.499999999999939);
#18819=CIRCLE('',#47329,1.05888347462729);
#18820=CIRCLE('',#47330,1.05888347462729);
#18821=CIRCLE('',#47332,0.500000000000053);
#18822=CIRCLE('',#47333,0.500000000000049);
#18823=CIRCLE('',#47335,1.29583333162382);
#18824=CIRCLE('',#47336,1.29583333162382);
#18825=CIRCLE('',#47338,0.499999999999935);
#18826=CIRCLE('',#47339,0.499999999999935);
#18827=CIRCLE('',#47341,1.60653900437062);
#18828=CIRCLE('',#47342,1.60653900437062);
#18829=CIRCLE('',#47344,0.500000000000058);
#18830=CIRCLE('',#47345,0.500000000000058);
#18831=CIRCLE('',#47347,1.82809807486272);
#18832=CIRCLE('',#47348,1.82809807486272);
#18833=CIRCLE('',#47350,0.500000000000058);
#18834=CIRCLE('',#47351,0.500000000000058);
#18835=CIRCLE('',#47353,1.85841829658594);
#18836=CIRCLE('',#47354,1.85841829658594);
#18837=CIRCLE('',#47356,0.49999999999983);
#18838=CIRCLE('',#47357,0.49999999999983);
#18839=CIRCLE('',#47359,1.81285717707166);
#18840=CIRCLE('',#47360,1.81285717707156);
#18841=CIRCLE('',#47362,0.499999999999944);
#18842=CIRCLE('',#47363,0.499999999999944);
#18843=CIRCLE('',#47365,1.91146602029502);
#18844=CIRCLE('',#47366,1.91146602029502);
#18845=CIRCLE('',#47368,0.499999999999939);
#18846=CIRCLE('',#47369,0.499999999999935);
#18847=CIRCLE('',#47371,1.5496711026025);
#18848=CIRCLE('',#47372,1.5496711026025);
#18849=CIRCLE('',#47374,0.500000000000053);
#18850=CIRCLE('',#47375,0.500000000000058);
#18851=CIRCLE('',#47377,1.25936103546568);
#18852=CIRCLE('',#47378,1.25936103546568);
#18853=CIRCLE('',#47380,0.500000000000053);
#18854=CIRCLE('',#47381,0.500000000000058);
#18855=CIRCLE('',#47382,61.7766775875802);
#18856=CIRCLE('',#47383,69.9999992709118);
#18857=CIRCLE('',#47384,45.1634298617437);
#18858=CIRCLE('',#47385,45.1634298617437);
#18859=CIRCLE('',#47386,45.1634298617437);
#18860=CIRCLE('',#47387,45.1634298617437);
#18861=CIRCLE('',#47388,45.1634298617437);
#18862=CIRCLE('',#47389,45.1634298617437);
#18863=CIRCLE('',#47390,45.1634298617437);
#18864=CIRCLE('',#47391,45.1634298617437);
#18865=CIRCLE('',#47392,45.1634298617437);
#18866=CIRCLE('',#47393,45.1634298617437);
#18867=CIRCLE('',#47394,45.1634298617437);
#18868=CIRCLE('',#47395,45.1634298617437);
#18869=CIRCLE('',#47396,45.1634298617437);
#18870=CIRCLE('',#47397,45.1634298617437);
#18871=CIRCLE('',#47398,45.1634298617437);
#18872=CIRCLE('',#47399,45.1634298617437);
#18873=CIRCLE('',#47400,45.1634298617437);
#18874=CIRCLE('',#47401,45.1634298617437);
#18875=CIRCLE('',#47402,45.1634298617437);
#18876=CIRCLE('',#47403,45.1634298617437);
#18877=CIRCLE('',#47404,45.1634298617437);
#18878=CIRCLE('',#47405,45.1634298617437);
#18879=CIRCLE('',#47406,45.1634298617437);
#18880=CIRCLE('',#47407,45.1634298617437);
#18881=CIRCLE('',#47408,45.1634298617437);
#18882=CIRCLE('',#47409,69.9999999999885);
#18883=CIRCLE('',#47411,62.7000000000001);
#18884=CIRCLE('',#47412,0.299999997585228);
#18885=CIRCLE('',#47413,0.299999997585552);
#18886=CIRCLE('',#47415,9.13915332737463);
#18887=CIRCLE('',#47416,10.7297759926639);
#18888=CIRCLE('',#47417,9.13915332737463);
#18889=CIRCLE('',#47419,1.);
#18890=CIRCLE('',#47420,10.9885950377664);
#18891=CIRCLE('',#47422,0.2);
#18892=CIRCLE('',#47423,8.99091713639504);
#18893=CIRCLE('',#47424,8.99091713639504);
#18894=CIRCLE('',#47426,63.3529411764695);
#18895=CIRCLE('',#47427,65.);
#18896=CIRCLE('',#47429,22.9734468277121);
#18897=CIRCLE('',#47430,0.500000000000003);
#18898=CIRCLE('',#47431,22.4734498738832);
#18899=CIRCLE('',#47432,0.499999999999997);
#18900=CIRCLE('',#47434,0.5);
#18901=CIRCLE('',#47435,0.5);
#18902=CIRCLE('',#47436,0.5);
#18903=CIRCLE('',#47438,0.300000458890413);
#18904=CIRCLE('',#47440,8.99091713639514);
#18905=CIRCLE('',#47441,8.99091713639514);
#18906=CIRCLE('',#47443,0.2);
#18907=CIRCLE('',#47444,8.83409633647444);
#18908=CIRCLE('',#47446,0.500000000000053);
#18909=CIRCLE('',#47452,8.3031389659941);
#18910=CIRCLE('',#47454,0.999999999999995);
#18911=CIRCLE('',#47455,8.01024574718068);
#18912=CIRCLE('',#47458,8.3031389659941);
#18913=CIRCLE('',#47460,8.3031389659941);
#18914=CIRCLE('',#47463,5.888925403621);
#18915=CIRCLE('',#47464,5.888925403621);
#18916=CIRCLE('',#47467,6.59603218480755);
#18917=CIRCLE('',#47468,8.01024574718068);
#18918=CIRCLE('',#47470,6.59603218480755);
#18919=CIRCLE('',#47471,8.01024574718068);
#18920=CIRCLE('',#47474,0.999999999999995);
#18921=CIRCLE('',#47475,0.999999999999995);
#18922=CIRCLE('',#47477,0.999999999999995);
#18923=CIRCLE('',#47479,0.999999999999995);
#18924=CIRCLE('',#47482,0.999999999999995);
#18925=CIRCLE('',#47484,0.999999999999995);
#18926=CIRCLE('',#47486,0.999999999999995);
#18927=CIRCLE('',#47488,0.500000000000008);
#18928=CIRCLE('',#47489,0.500000000000007);
#18929=CIRCLE('',#47490,0.500000000000004);
#18930=CIRCLE('',#47492,0.499999999999999);
#18931=CIRCLE('',#47493,0.500000411450474);
#18932=CIRCLE('',#47495,0.499999999999999);
#18933=CIRCLE('',#47497,0.299999999999944);
#18934=CIRCLE('',#47498,0.299999999999994);
#18935=CIRCLE('',#47499,0.30000000000002);
#18936=CIRCLE('',#47500,0.300000000000048);
#18937=CIRCLE('',#47501,1.99999248610074);
#18938=CIRCLE('',#47502,0.500000000000003);
#18939=CIRCLE('',#47504,0.500000000000003);
#18940=CIRCLE('',#47505,22.4734498738832);
#18941=CIRCLE('',#47506,22.9734468277121);
#18942=CIRCLE('',#47507,0.5);
#18943=CIRCLE('',#47508,1.99999248601366);
#18944=CIRCLE('',#47509,1.9999924861154);
#18945=CIRCLE('',#47511,0.5);
#18946=CIRCLE('',#47512,1.99999248606425);
#18947=CIRCLE('',#47513,2.00000000000005);
#18948=CIRCLE('',#47515,65.);
#18949=CIRCLE('',#47516,1.9999999999645);
#18950=CIRCLE('',#47517,2.);
#18951=CIRCLE('',#47519,63.5880980163361);
#18952=CIRCLE('',#47521,2.00000590977433);
#18953=CIRCLE('',#47522,1.99999999999992);
#18954=CIRCLE('',#47524,1.99999999997966);
#18955=CIRCLE('',#47533,146.40821343272);
#18956=CIRCLE('',#47534,146.408212929521);
#20643=VERTEX_POINT('',#65511);
#20644=VERTEX_POINT('',#65512);
#20645=VERTEX_POINT('',#65514);
#20646=VERTEX_POINT('',#65516);
#20647=VERTEX_POINT('',#65520);
#20648=VERTEX_POINT('',#65522);
#20649=VERTEX_POINT('',#65531);
#20650=VERTEX_POINT('',#65532);
#20651=VERTEX_POINT('',#65534);
#20652=VERTEX_POINT('',#65536);
#20653=VERTEX_POINT('',#65540);
#20654=VERTEX_POINT('',#65544);
#20655=VERTEX_POINT('',#65551);
#20656=VERTEX_POINT('',#65553);
#20657=VERTEX_POINT('',#65557);
#20658=VERTEX_POINT('',#65559);
#20659=VERTEX_POINT('',#65563);
#20660=VERTEX_POINT('',#65565);
#20661=VERTEX_POINT('',#65569);
#20662=VERTEX_POINT('',#65571);
#20663=VERTEX_POINT('',#65575);
#20664=VERTEX_POINT('',#65577);
#20665=VERTEX_POINT('',#65581);
#20666=VERTEX_POINT('',#65583);
#20667=VERTEX_POINT('',#65587);
#20668=VERTEX_POINT('',#65589);
#20669=VERTEX_POINT('',#65593);
#20670=VERTEX_POINT('',#65595);
#20671=VERTEX_POINT('',#65599);
#20672=VERTEX_POINT('',#65601);
#20673=VERTEX_POINT('',#65605);
#20674=VERTEX_POINT('',#65607);
#20675=VERTEX_POINT('',#65611);
#20676=VERTEX_POINT('',#65613);
#20677=VERTEX_POINT('',#65617);
#20678=VERTEX_POINT('',#65619);
#20679=VERTEX_POINT('',#65623);
#20680=VERTEX_POINT('',#65624);
#20681=VERTEX_POINT('',#65646);
#20682=VERTEX_POINT('',#65705);
#20683=VERTEX_POINT('',#65707);
#20684=VERTEX_POINT('',#65744);
#20685=VERTEX_POINT('',#65745);
#20686=VERTEX_POINT('',#65766);
#20687=VERTEX_POINT('',#65826);
#20688=VERTEX_POINT('',#65828);
#20689=VERTEX_POINT('',#65865);
#20690=VERTEX_POINT('',#65866);
#20691=VERTEX_POINT('',#65890);
#20692=VERTEX_POINT('',#65947);
#20693=VERTEX_POINT('',#65949);
#20694=VERTEX_POINT('',#65986);
#20695=VERTEX_POINT('',#65987);
#20696=VERTEX_POINT('',#66008);
#20697=VERTEX_POINT('',#66068);
#20698=VERTEX_POINT('',#66070);
#20699=VERTEX_POINT('',#66107);
#20700=VERTEX_POINT('',#66108);
#20701=VERTEX_POINT('',#66132);
#20702=VERTEX_POINT('',#66189);
#20703=VERTEX_POINT('',#66191);
#20704=VERTEX_POINT('',#66228);
#20705=VERTEX_POINT('',#66229);
#20706=VERTEX_POINT('',#66253);
#20707=VERTEX_POINT('',#66310);
#20708=VERTEX_POINT('',#66312);
#20709=VERTEX_POINT('',#66349);
#20710=VERTEX_POINT('',#66350);
#20711=VERTEX_POINT('',#66374);
#20712=VERTEX_POINT('',#66431);
#20713=VERTEX_POINT('',#66433);
#20714=VERTEX_POINT('',#66470);
#20715=VERTEX_POINT('',#66471);
#20716=VERTEX_POINT('',#66495);
#20717=VERTEX_POINT('',#66552);
#20718=VERTEX_POINT('',#66554);
#20719=VERTEX_POINT('',#66591);
#20720=VERTEX_POINT('',#66592);
#20721=VERTEX_POINT('',#66616);
#20722=VERTEX_POINT('',#66673);
#20723=VERTEX_POINT('',#66675);
#20724=VERTEX_POINT('',#66712);
#20725=VERTEX_POINT('',#66713);
#20726=VERTEX_POINT('',#66737);
#20727=VERTEX_POINT('',#66794);
#20728=VERTEX_POINT('',#66796);
#20729=VERTEX_POINT('',#66833);
#20730=VERTEX_POINT('',#66834);
#20731=VERTEX_POINT('',#66855);
#20732=VERTEX_POINT('',#66915);
#20733=VERTEX_POINT('',#66917);
#20734=VERTEX_POINT('',#66954);
#20735=VERTEX_POINT('',#66955);
#20736=VERTEX_POINT('',#66976);
#20737=VERTEX_POINT('',#67036);
#20738=VERTEX_POINT('',#67038);
#20739=VERTEX_POINT('',#67075);
#20740=VERTEX_POINT('',#67076);
#20741=VERTEX_POINT('',#67097);
#20742=VERTEX_POINT('',#67157);
#20743=VERTEX_POINT('',#67159);
#20744=VERTEX_POINT('',#67196);
#20745=VERTEX_POINT('',#67197);
#20746=VERTEX_POINT('',#67218);
#20747=VERTEX_POINT('',#67278);
#20748=VERTEX_POINT('',#67280);
#20749=VERTEX_POINT('',#67317);
#20750=VERTEX_POINT('',#67318);
#20751=VERTEX_POINT('',#67339);
#20752=VERTEX_POINT('',#67399);
#20753=VERTEX_POINT('',#67401);
#20754=VERTEX_POINT('',#67438);
#20755=VERTEX_POINT('',#67439);
#20756=VERTEX_POINT('',#67460);
#20757=VERTEX_POINT('',#67520);
#20758=VERTEX_POINT('',#67522);
#20759=VERTEX_POINT('',#67559);
#20760=VERTEX_POINT('',#67560);
#20761=VERTEX_POINT('',#67582);
#20762=VERTEX_POINT('',#67641);
#20763=VERTEX_POINT('',#67643);
#20764=VERTEX_POINT('',#67680);
#20765=VERTEX_POINT('',#67681);
#20766=VERTEX_POINT('',#67700);
#20767=VERTEX_POINT('',#67762);
#20768=VERTEX_POINT('',#67764);
#20769=VERTEX_POINT('',#67801);
#20770=VERTEX_POINT('',#67802);
#20771=VERTEX_POINT('',#67826);
#20772=VERTEX_POINT('',#67883);
#20773=VERTEX_POINT('',#67885);
#20774=VERTEX_POINT('',#67922);
#20775=VERTEX_POINT('',#67923);
#20776=VERTEX_POINT('',#67942);
#20777=VERTEX_POINT('',#68004);
#20778=VERTEX_POINT('',#68006);
#20779=VERTEX_POINT('',#68043);
#20780=VERTEX_POINT('',#68044);
#20781=VERTEX_POINT('',#68063);
#20782=VERTEX_POINT('',#68125);
#20783=VERTEX_POINT('',#68127);
#20784=VERTEX_POINT('',#68164);
#20785=VERTEX_POINT('',#68165);
#20786=VERTEX_POINT('',#68184);
#20787=VERTEX_POINT('',#68246);
#20788=VERTEX_POINT('',#68248);
#20789=VERTEX_POINT('',#68285);
#20790=VERTEX_POINT('',#68286);
#20791=VERTEX_POINT('',#68305);
#20792=VERTEX_POINT('',#68367);
#20793=VERTEX_POINT('',#68369);
#20794=VERTEX_POINT('',#68406);
#20795=VERTEX_POINT('',#68407);
#20796=VERTEX_POINT('',#68429);
#20797=VERTEX_POINT('',#68488);
#20798=VERTEX_POINT('',#68490);
#20799=VERTEX_POINT('',#68527);
#20800=VERTEX_POINT('',#68528);
#20801=VERTEX_POINT('',#68547);
#20802=VERTEX_POINT('',#68609);
#20803=VERTEX_POINT('',#68611);
#20804=VERTEX_POINT('',#68648);
#20805=VERTEX_POINT('',#68649);
#20806=VERTEX_POINT('',#68668);
#20807=VERTEX_POINT('',#68730);
#20808=VERTEX_POINT('',#68732);
#20809=VERTEX_POINT('',#68769);
#20810=VERTEX_POINT('',#68770);
#20811=VERTEX_POINT('',#68789);
#20812=VERTEX_POINT('',#68851);
#20813=VERTEX_POINT('',#68853);
#20814=VERTEX_POINT('',#68890);
#20815=VERTEX_POINT('',#68891);
#20816=VERTEX_POINT('',#68910);
#20817=VERTEX_POINT('',#68972);
#20818=VERTEX_POINT('',#68974);
#20819=VERTEX_POINT('',#69011);
#20820=VERTEX_POINT('',#69012);
#20821=VERTEX_POINT('',#69031);
#20822=VERTEX_POINT('',#69093);
#20823=VERTEX_POINT('',#69095);
#20824=VERTEX_POINT('',#69132);
#20825=VERTEX_POINT('',#69133);
#20826=VERTEX_POINT('',#69152);
#20827=VERTEX_POINT('',#69214);
#20828=VERTEX_POINT('',#69216);
#20829=VERTEX_POINT('',#69253);
#20830=VERTEX_POINT('',#69254);
#20831=VERTEX_POINT('',#69273);
#20832=VERTEX_POINT('',#69335);
#20833=VERTEX_POINT('',#69337);
#20834=VERTEX_POINT('',#69374);
#20835=VERTEX_POINT('',#69375);
#20836=VERTEX_POINT('',#69394);
#20837=VERTEX_POINT('',#69456);
#20838=VERTEX_POINT('',#69458);
#20839=VERTEX_POINT('',#69495);
#20840=VERTEX_POINT('',#69496);
#20841=VERTEX_POINT('',#69515);
#20842=VERTEX_POINT('',#69579);
#20843=VERTEX_POINT('',#69581);
#20844=VERTEX_POINT('',#69618);
#20845=VERTEX_POINT('',#69619);
#20846=VERTEX_POINT('',#69641);
#20847=VERTEX_POINT('',#69700);
#20848=VERTEX_POINT('',#69702);
#20849=VERTEX_POINT('',#69739);
#20850=VERTEX_POINT('',#69740);
#20851=VERTEX_POINT('',#69759);
#20852=VERTEX_POINT('',#69821);
#20853=VERTEX_POINT('',#69823);
#20854=VERTEX_POINT('',#69860);
#20855=VERTEX_POINT('',#69861);
#20856=VERTEX_POINT('',#69880);
#20857=VERTEX_POINT('',#69942);
#20858=VERTEX_POINT('',#69944);
#20859=VERTEX_POINT('',#69981);
#20860=VERTEX_POINT('',#69982);
#20861=VERTEX_POINT('',#70001);
#20862=VERTEX_POINT('',#70063);
#20863=VERTEX_POINT('',#70065);
#20864=VERTEX_POINT('',#70102);
#20865=VERTEX_POINT('',#70103);
#20866=VERTEX_POINT('',#70122);
#20867=VERTEX_POINT('',#70196);
#20868=VERTEX_POINT('',#70198);
#20869=VERTEX_POINT('',#70235);
#20870=VERTEX_POINT('',#70236);
#20871=VERTEX_POINT('',#70255);
#20872=VERTEX_POINT('',#70317);
#20873=VERTEX_POINT('',#70319);
#20874=VERTEX_POINT('',#70356);
#20875=VERTEX_POINT('',#70358);
#20876=VERTEX_POINT('',#70405);
#20877=VERTEX_POINT('',#70407);
#20878=VERTEX_POINT('',#70411);
#20879=VERTEX_POINT('',#70413);
#20880=VERTEX_POINT('',#70462);
#20881=VERTEX_POINT('',#70464);
#20882=VERTEX_POINT('',#70468);
#20883=VERTEX_POINT('',#70469);
#20884=VERTEX_POINT('',#70488);
#20885=VERTEX_POINT('',#70566);
#20886=VERTEX_POINT('',#70568);
#20887=VERTEX_POINT('',#70605);
#20888=VERTEX_POINT('',#70606);
#20889=VERTEX_POINT('',#70628);
#20890=VERTEX_POINT('',#70705);
#20891=VERTEX_POINT('',#70707);
#20892=VERTEX_POINT('',#70744);
#20893=VERTEX_POINT('',#70746);
#20894=VERTEX_POINT('',#70797);
#20895=VERTEX_POINT('',#70799);
#20896=VERTEX_POINT('',#70803);
#20897=VERTEX_POINT('',#70805);
#20898=VERTEX_POINT('',#70854);
#20899=VERTEX_POINT('',#70856);
#20900=VERTEX_POINT('',#70860);
#20901=VERTEX_POINT('',#70861);
#20902=VERTEX_POINT('',#70883);
#20903=VERTEX_POINT('',#70952);
#20904=VERTEX_POINT('',#70954);
#20905=VERTEX_POINT('',#70991);
#20906=VERTEX_POINT('',#70992);
#20907=VERTEX_POINT('',#71014);
#20908=VERTEX_POINT('',#71087);
#20909=VERTEX_POINT('',#71089);
#20910=VERTEX_POINT('',#71126);
#20911=VERTEX_POINT('',#71128);
#20912=VERTEX_POINT('',#71179);
#20913=VERTEX_POINT('',#71181);
#20914=VERTEX_POINT('',#71185);
#20915=VERTEX_POINT('',#71186);
#20916=VERTEX_POINT('',#71205);
#20917=VERTEX_POINT('',#71277);
#20918=VERTEX_POINT('',#71279);
#20919=VERTEX_POINT('',#71316);
#20920=VERTEX_POINT('',#71317);
#20921=VERTEX_POINT('',#71339);
#20922=VERTEX_POINT('',#71406);
#20923=VERTEX_POINT('',#71408);
#20924=VERTEX_POINT('',#71445);
#20925=VERTEX_POINT('',#71447);
#20926=VERTEX_POINT('',#71500);
#20927=VERTEX_POINT('',#71502);
#20928=VERTEX_POINT('',#71506);
#20929=VERTEX_POINT('',#71507);
#20930=VERTEX_POINT('',#71529);
#20931=VERTEX_POINT('',#71600);
#20932=VERTEX_POINT('',#71602);
#20933=VERTEX_POINT('',#71639);
#20934=VERTEX_POINT('',#71640);
#20935=VERTEX_POINT('',#71659);
#20936=VERTEX_POINT('',#71731);
#20937=VERTEX_POINT('',#71733);
#20938=VERTEX_POINT('',#71770);
#20939=VERTEX_POINT('',#71771);
#20940=VERTEX_POINT('',#71793);
#20941=VERTEX_POINT('',#71868);
#20942=VERTEX_POINT('',#71870);
#20943=VERTEX_POINT('',#71907);
#20944=VERTEX_POINT('',#71908);
#20945=VERTEX_POINT('',#71927);
#20946=VERTEX_POINT('',#72009);
#20947=VERTEX_POINT('',#72011);
#20948=VERTEX_POINT('',#72048);
#20949=VERTEX_POINT('',#72049);
#20950=VERTEX_POINT('',#72071);
#20951=VERTEX_POINT('',#72130);
#20952=VERTEX_POINT('',#72132);
#20953=VERTEX_POINT('',#72169);
#20954=VERTEX_POINT('',#72170);
#20955=VERTEX_POINT('',#72189);
#20956=VERTEX_POINT('',#72265);
#20957=VERTEX_POINT('',#72267);
#20958=VERTEX_POINT('',#72304);
#20959=VERTEX_POINT('',#72305);
#20960=VERTEX_POINT('',#72327);
#20961=VERTEX_POINT('',#72386);
#20962=VERTEX_POINT('',#72388);
#20963=VERTEX_POINT('',#72425);
#20964=VERTEX_POINT('',#72426);
#20965=VERTEX_POINT('',#72448);
#20966=VERTEX_POINT('',#72507);
#20967=VERTEX_POINT('',#72509);
#20968=VERTEX_POINT('',#72546);
#20969=VERTEX_POINT('',#72547);
#20970=VERTEX_POINT('',#72568);
#20971=VERTEX_POINT('',#72628);
#20972=VERTEX_POINT('',#72630);
#20973=VERTEX_POINT('',#72667);
#20974=VERTEX_POINT('',#72668);
#20975=VERTEX_POINT('',#72692);
#20976=VERTEX_POINT('',#72749);
#20977=VERTEX_POINT('',#72751);
#20978=VERTEX_POINT('',#72788);
#20979=VERTEX_POINT('',#72789);
#20980=VERTEX_POINT('',#72813);
#20981=VERTEX_POINT('',#72870);
#20982=VERTEX_POINT('',#72872);
#20983=VERTEX_POINT('',#72909);
#20984=VERTEX_POINT('',#72910);
#20985=VERTEX_POINT('',#72932);
#20986=VERTEX_POINT('',#72991);
#20987=VERTEX_POINT('',#72993);
#20988=VERTEX_POINT('',#73030);
#20989=VERTEX_POINT('',#73031);
#20990=VERTEX_POINT('',#73055);
#20991=VERTEX_POINT('',#73114);
#20992=VERTEX_POINT('',#73116);
#20993=VERTEX_POINT('',#73153);
#20994=VERTEX_POINT('',#73154);
#20995=VERTEX_POINT('',#73178);
#20996=VERTEX_POINT('',#73235);
#20997=VERTEX_POINT('',#73237);
#20998=VERTEX_POINT('',#73274);
#20999=VERTEX_POINT('',#73276);
#21000=VERTEX_POINT('',#73280);
#21001=VERTEX_POINT('',#73282);
#21002=VERTEX_POINT('',#73286);
#21003=VERTEX_POINT('',#73288);
#21004=VERTEX_POINT('',#73292);
#21005=VERTEX_POINT('',#73294);
#21006=VERTEX_POINT('',#73298);
#21007=VERTEX_POINT('',#73300);
#21008=VERTEX_POINT('',#73304);
#21009=VERTEX_POINT('',#73306);
#21010=VERTEX_POINT('',#73310);
#21011=VERTEX_POINT('',#73312);
#21012=VERTEX_POINT('',#73316);
#21013=VERTEX_POINT('',#73318);
#21014=VERTEX_POINT('',#73322);
#21015=VERTEX_POINT('',#73324);
#21016=VERTEX_POINT('',#73328);
#21017=VERTEX_POINT('',#73330);
#21018=VERTEX_POINT('',#73334);
#21019=VERTEX_POINT('',#73336);
#21020=VERTEX_POINT('',#73340);
#21021=VERTEX_POINT('',#73342);
#21022=VERTEX_POINT('',#73346);
#21023=VERTEX_POINT('',#73348);
#21024=VERTEX_POINT('',#73352);
#21025=VERTEX_POINT('',#73354);
#21026=VERTEX_POINT('',#73358);
#21027=VERTEX_POINT('',#73360);
#21028=VERTEX_POINT('',#73364);
#21029=VERTEX_POINT('',#73366);
#21030=VERTEX_POINT('',#73370);
#21031=VERTEX_POINT('',#73372);
#21032=VERTEX_POINT('',#73374);
#21033=VERTEX_POINT('',#73400);
#21034=VERTEX_POINT('',#73411);
#21035=VERTEX_POINT('',#73413);
#21036=VERTEX_POINT('',#73417);
#21037=VERTEX_POINT('',#73419);
#21038=VERTEX_POINT('',#73423);
#21039=VERTEX_POINT('',#73425);
#21040=VERTEX_POINT('',#73429);
#21041=VERTEX_POINT('',#73431);
#21042=VERTEX_POINT('',#73435);
#21043=VERTEX_POINT('',#73437);
#21044=VERTEX_POINT('',#73441);
#21045=VERTEX_POINT('',#73443);
#21046=VERTEX_POINT('',#73447);
#21047=VERTEX_POINT('',#73449);
#21048=VERTEX_POINT('',#73453);
#21049=VERTEX_POINT('',#73455);
#21050=VERTEX_POINT('',#73459);
#21051=VERTEX_POINT('',#73461);
#21052=VERTEX_POINT('',#73465);
#21053=VERTEX_POINT('',#73467);
#21054=VERTEX_POINT('',#73471);
#21055=VERTEX_POINT('',#73473);
#21056=VERTEX_POINT('',#73477);
#21057=VERTEX_POINT('',#73479);
#21058=VERTEX_POINT('',#73483);
#21059=VERTEX_POINT('',#73485);
#21060=VERTEX_POINT('',#73489);
#21061=VERTEX_POINT('',#73491);
#21062=VERTEX_POINT('',#73495);
#21063=VERTEX_POINT('',#73497);
#21064=VERTEX_POINT('',#73501);
#21065=VERTEX_POINT('',#73503);
#21066=VERTEX_POINT('',#73507);
#21067=VERTEX_POINT('',#73509);
#21068=VERTEX_POINT('',#73513);
#21069=VERTEX_POINT('',#73515);
#21070=VERTEX_POINT('',#73517);
#21071=VERTEX_POINT('',#73541);
#21072=VERTEX_POINT('',#73554);
#21073=VERTEX_POINT('',#73556);
#21074=VERTEX_POINT('',#73560);
#21075=VERTEX_POINT('',#73562);
#21076=VERTEX_POINT('',#73566);
#21077=VERTEX_POINT('',#73568);
#21078=VERTEX_POINT('',#73572);
#21079=VERTEX_POINT('',#73574);
#21080=VERTEX_POINT('',#73578);
#21081=VERTEX_POINT('',#73580);
#21082=VERTEX_POINT('',#73584);
#21083=VERTEX_POINT('',#73586);
#21084=VERTEX_POINT('',#73590);
#21085=VERTEX_POINT('',#73592);
#21086=VERTEX_POINT('',#73596);
#21087=VERTEX_POINT('',#73598);
#21088=VERTEX_POINT('',#73602);
#21089=VERTEX_POINT('',#73604);
#21090=VERTEX_POINT('',#73608);
#21091=VERTEX_POINT('',#73610);
#21092=VERTEX_POINT('',#73614);
#21093=VERTEX_POINT('',#73616);
#21094=VERTEX_POINT('',#73620);
#21095=VERTEX_POINT('',#73622);
#21096=VERTEX_POINT('',#73626);
#21097=VERTEX_POINT('',#73628);
#21098=VERTEX_POINT('',#73632);
#21099=VERTEX_POINT('',#73634);
#21100=VERTEX_POINT('',#73638);
#21101=VERTEX_POINT('',#73640);
#21102=VERTEX_POINT('',#73644);
#21103=VERTEX_POINT('',#73646);
#21104=VERTEX_POINT('',#73648);
#21105=VERTEX_POINT('',#73672);
#21106=VERTEX_POINT('',#73685);
#21107=VERTEX_POINT('',#73687);
#21108=VERTEX_POINT('',#73691);
#21109=VERTEX_POINT('',#73693);
#21110=VERTEX_POINT('',#73697);
#21111=VERTEX_POINT('',#73699);
#21112=VERTEX_POINT('',#73703);
#21113=VERTEX_POINT('',#73705);
#21114=VERTEX_POINT('',#73709);
#21115=VERTEX_POINT('',#73711);
#21116=VERTEX_POINT('',#73715);
#21117=VERTEX_POINT('',#73717);
#21118=VERTEX_POINT('',#73721);
#21119=VERTEX_POINT('',#73723);
#21120=VERTEX_POINT('',#73727);
#21121=VERTEX_POINT('',#73729);
#21122=VERTEX_POINT('',#73733);
#21123=VERTEX_POINT('',#73735);
#21124=VERTEX_POINT('',#73739);
#21125=VERTEX_POINT('',#73741);
#21126=VERTEX_POINT('',#73745);
#21127=VERTEX_POINT('',#73747);
#21128=VERTEX_POINT('',#73751);
#21129=VERTEX_POINT('',#73753);
#21130=VERTEX_POINT('',#73757);
#21131=VERTEX_POINT('',#73759);
#21132=VERTEX_POINT('',#73763);
#21133=VERTEX_POINT('',#73765);
#21134=VERTEX_POINT('',#73769);
#21135=VERTEX_POINT('',#73771);
#21136=VERTEX_POINT('',#73775);
#21137=VERTEX_POINT('',#73777);
#21138=VERTEX_POINT('',#73781);
#21139=VERTEX_POINT('',#73783);
#21140=VERTEX_POINT('',#73787);
#21141=VERTEX_POINT('',#73789);
#21142=VERTEX_POINT('',#73791);
#21143=VERTEX_POINT('',#73813);
#21144=VERTEX_POINT('',#73828);
#21145=VERTEX_POINT('',#73830);
#21146=VERTEX_POINT('',#73834);
#21147=VERTEX_POINT('',#73836);
#21148=VERTEX_POINT('',#73840);
#21149=VERTEX_POINT('',#73842);
#21150=VERTEX_POINT('',#73846);
#21151=VERTEX_POINT('',#73848);
#21152=VERTEX_POINT('',#73852);
#21153=VERTEX_POINT('',#73854);
#21154=VERTEX_POINT('',#73858);
#21155=VERTEX_POINT('',#73860);
#21156=VERTEX_POINT('',#73864);
#21157=VERTEX_POINT('',#73866);
#21158=VERTEX_POINT('',#73870);
#21159=VERTEX_POINT('',#73872);
#21160=VERTEX_POINT('',#73876);
#21161=VERTEX_POINT('',#73878);
#21162=VERTEX_POINT('',#73882);
#21163=VERTEX_POINT('',#73884);
#21164=VERTEX_POINT('',#73888);
#21165=VERTEX_POINT('',#73890);
#21166=VERTEX_POINT('',#73894);
#21167=VERTEX_POINT('',#73896);
#21168=VERTEX_POINT('',#73900);
#21169=VERTEX_POINT('',#73902);
#21170=VERTEX_POINT('',#73906);
#21171=VERTEX_POINT('',#73908);
#21172=VERTEX_POINT('',#73912);
#21173=VERTEX_POINT('',#73914);
#21174=VERTEX_POINT('',#73918);
#21175=VERTEX_POINT('',#73920);
#21176=VERTEX_POINT('',#73924);
#21177=VERTEX_POINT('',#73926);
#21178=VERTEX_POINT('',#73930);
#21179=VERTEX_POINT('',#73932);
#21180=VERTEX_POINT('',#73934);
#21181=VERTEX_POINT('',#73956);
#21182=VERTEX_POINT('',#73971);
#21183=VERTEX_POINT('',#73973);
#21184=VERTEX_POINT('',#73977);
#21185=VERTEX_POINT('',#73979);
#21186=VERTEX_POINT('',#73983);
#21187=VERTEX_POINT('',#73985);
#21188=VERTEX_POINT('',#73989);
#21189=VERTEX_POINT('',#73991);
#21190=VERTEX_POINT('',#73995);
#21191=VERTEX_POINT('',#73997);
#21192=VERTEX_POINT('',#74001);
#21193=VERTEX_POINT('',#74003);
#21194=VERTEX_POINT('',#74007);
#21195=VERTEX_POINT('',#74009);
#21196=VERTEX_POINT('',#74013);
#21197=VERTEX_POINT('',#74015);
#21198=VERTEX_POINT('',#74019);
#21199=VERTEX_POINT('',#74021);
#21200=VERTEX_POINT('',#74025);
#21201=VERTEX_POINT('',#74027);
#21202=VERTEX_POINT('',#74031);
#21203=VERTEX_POINT('',#74033);
#21204=VERTEX_POINT('',#74037);
#21205=VERTEX_POINT('',#74039);
#21206=VERTEX_POINT('',#74043);
#21207=VERTEX_POINT('',#74045);
#21208=VERTEX_POINT('',#74049);
#21209=VERTEX_POINT('',#74051);
#21210=VERTEX_POINT('',#74055);
#21211=VERTEX_POINT('',#74057);
#21212=VERTEX_POINT('',#74061);
#21213=VERTEX_POINT('',#74063);
#21214=VERTEX_POINT('',#74067);
#21215=VERTEX_POINT('',#74069);
#21216=VERTEX_POINT('',#74073);
#21217=VERTEX_POINT('',#74075);
#21218=VERTEX_POINT('',#74077);
#21219=VERTEX_POINT('',#74097);
#21220=VERTEX_POINT('',#74114);
#21221=VERTEX_POINT('',#74116);
#21222=VERTEX_POINT('',#74120);
#21223=VERTEX_POINT('',#74122);
#21224=VERTEX_POINT('',#74126);
#21225=VERTEX_POINT('',#74128);
#21226=VERTEX_POINT('',#74132);
#21227=VERTEX_POINT('',#74134);
#21228=VERTEX_POINT('',#74138);
#21229=VERTEX_POINT('',#74140);
#21230=VERTEX_POINT('',#74144);
#21231=VERTEX_POINT('',#74146);
#21232=VERTEX_POINT('',#74150);
#21233=VERTEX_POINT('',#74152);
#21234=VERTEX_POINT('',#74156);
#21235=VERTEX_POINT('',#74158);
#21236=VERTEX_POINT('',#74162);
#21237=VERTEX_POINT('',#74164);
#21238=VERTEX_POINT('',#74168);
#21239=VERTEX_POINT('',#74170);
#21240=VERTEX_POINT('',#74174);
#21241=VERTEX_POINT('',#74176);
#21242=VERTEX_POINT('',#74180);
#21243=VERTEX_POINT('',#74182);
#21244=VERTEX_POINT('',#74186);
#21245=VERTEX_POINT('',#74188);
#21246=VERTEX_POINT('',#74192);
#21247=VERTEX_POINT('',#74194);
#21248=VERTEX_POINT('',#74198);
#21249=VERTEX_POINT('',#74200);
#21250=VERTEX_POINT('',#74204);
#21251=VERTEX_POINT('',#74206);
#21252=VERTEX_POINT('',#74210);
#21253=VERTEX_POINT('',#74212);
#21254=VERTEX_POINT('',#74216);
#21255=VERTEX_POINT('',#74218);
#21256=VERTEX_POINT('',#74220);
#21257=VERTEX_POINT('',#74240);
#21258=VERTEX_POINT('',#74257);
#21259=VERTEX_POINT('',#74259);
#21260=VERTEX_POINT('',#74263);
#21261=VERTEX_POINT('',#74265);
#21262=VERTEX_POINT('',#74269);
#21263=VERTEX_POINT('',#74271);
#21264=VERTEX_POINT('',#74275);
#21265=VERTEX_POINT('',#74277);
#21266=VERTEX_POINT('',#74281);
#21267=VERTEX_POINT('',#74283);
#21268=VERTEX_POINT('',#74287);
#21269=VERTEX_POINT('',#74289);
#21270=VERTEX_POINT('',#74293);
#21271=VERTEX_POINT('',#74295);
#21272=VERTEX_POINT('',#74299);
#21273=VERTEX_POINT('',#74301);
#21274=VERTEX_POINT('',#74305);
#21275=VERTEX_POINT('',#74307);
#21276=VERTEX_POINT('',#74311);
#21277=VERTEX_POINT('',#74313);
#21278=VERTEX_POINT('',#74317);
#21279=VERTEX_POINT('',#74319);
#21280=VERTEX_POINT('',#74323);
#21281=VERTEX_POINT('',#74325);
#21282=VERTEX_POINT('',#74329);
#21283=VERTEX_POINT('',#74331);
#21284=VERTEX_POINT('',#74335);
#21285=VERTEX_POINT('',#74337);
#21286=VERTEX_POINT('',#74341);
#21287=VERTEX_POINT('',#74343);
#21288=VERTEX_POINT('',#74347);
#21289=VERTEX_POINT('',#74349);
#21290=VERTEX_POINT('',#74351);
#21291=VERTEX_POINT('',#74366);
#21292=VERTEX_POINT('',#74388);
#21293=VERTEX_POINT('',#74390);
#21294=VERTEX_POINT('',#74394);
#21295=VERTEX_POINT('',#74396);
#21296=VERTEX_POINT('',#74400);
#21297=VERTEX_POINT('',#74402);
#21298=VERTEX_POINT('',#74406);
#21299=VERTEX_POINT('',#74408);
#21300=VERTEX_POINT('',#74412);
#21301=VERTEX_POINT('',#74414);
#21302=VERTEX_POINT('',#74418);
#21303=VERTEX_POINT('',#74420);
#21304=VERTEX_POINT('',#74424);
#21305=VERTEX_POINT('',#74426);
#21306=VERTEX_POINT('',#74430);
#21307=VERTEX_POINT('',#74432);
#21308=VERTEX_POINT('',#74436);
#21309=VERTEX_POINT('',#74438);
#21310=VERTEX_POINT('',#74442);
#21311=VERTEX_POINT('',#74444);
#21312=VERTEX_POINT('',#74448);
#21313=VERTEX_POINT('',#74450);
#21314=VERTEX_POINT('',#74454);
#21315=VERTEX_POINT('',#74456);
#21316=VERTEX_POINT('',#74460);
#21317=VERTEX_POINT('',#74462);
#21318=VERTEX_POINT('',#74466);
#21319=VERTEX_POINT('',#74468);
#21320=VERTEX_POINT('',#74472);
#21321=VERTEX_POINT('',#74474);
#21322=VERTEX_POINT('',#74478);
#21323=VERTEX_POINT('',#74480);
#21324=VERTEX_POINT('',#74484);
#21325=VERTEX_POINT('',#74486);
#21326=VERTEX_POINT('',#74490);
#21327=VERTEX_POINT('',#74492);
#21328=VERTEX_POINT('',#74494);
#21329=VERTEX_POINT('',#74509);
#21330=VERTEX_POINT('',#74531);
#21331=VERTEX_POINT('',#74533);
#21332=VERTEX_POINT('',#74537);
#21333=VERTEX_POINT('',#74539);
#21334=VERTEX_POINT('',#74543);
#21335=VERTEX_POINT('',#74545);
#21336=VERTEX_POINT('',#74549);
#21337=VERTEX_POINT('',#74551);
#21338=VERTEX_POINT('',#74555);
#21339=VERTEX_POINT('',#74557);
#21340=VERTEX_POINT('',#74561);
#21341=VERTEX_POINT('',#74563);
#21342=VERTEX_POINT('',#74567);
#21343=VERTEX_POINT('',#74569);
#21344=VERTEX_POINT('',#74573);
#21345=VERTEX_POINT('',#74575);
#21346=VERTEX_POINT('',#74579);
#21347=VERTEX_POINT('',#74581);
#21348=VERTEX_POINT('',#74585);
#21349=VERTEX_POINT('',#74587);
#21350=VERTEX_POINT('',#74591);
#21351=VERTEX_POINT('',#74593);
#21352=VERTEX_POINT('',#74597);
#21353=VERTEX_POINT('',#74599);
#21354=VERTEX_POINT('',#74603);
#21355=VERTEX_POINT('',#74605);
#21356=VERTEX_POINT('',#74609);
#21357=VERTEX_POINT('',#74611);
#21358=VERTEX_POINT('',#74615);
#21359=VERTEX_POINT('',#74617);
#21360=VERTEX_POINT('',#74621);
#21361=VERTEX_POINT('',#74623);
#21362=VERTEX_POINT('',#74627);
#21363=VERTEX_POINT('',#74629);
#21364=VERTEX_POINT('',#74633);
#21365=VERTEX_POINT('',#74635);
#21366=VERTEX_POINT('',#74637);
#21367=VERTEX_POINT('',#74650);
#21368=VERTEX_POINT('',#74674);
#21369=VERTEX_POINT('',#74676);
#21370=VERTEX_POINT('',#74680);
#21371=VERTEX_POINT('',#74682);
#21372=VERTEX_POINT('',#74686);
#21373=VERTEX_POINT('',#74688);
#21374=VERTEX_POINT('',#74692);
#21375=VERTEX_POINT('',#74694);
#21376=VERTEX_POINT('',#74698);
#21377=VERTEX_POINT('',#74700);
#21378=VERTEX_POINT('',#74704);
#21379=VERTEX_POINT('',#74706);
#21380=VERTEX_POINT('',#74710);
#21381=VERTEX_POINT('',#74712);
#21382=VERTEX_POINT('',#74716);
#21383=VERTEX_POINT('',#74718);
#21384=VERTEX_POINT('',#74722);
#21385=VERTEX_POINT('',#74724);
#21386=VERTEX_POINT('',#74728);
#21387=VERTEX_POINT('',#74730);
#21388=VERTEX_POINT('',#74734);
#21389=VERTEX_POINT('',#74736);
#21390=VERTEX_POINT('',#74740);
#21391=VERTEX_POINT('',#74742);
#21392=VERTEX_POINT('',#74746);
#21393=VERTEX_POINT('',#74748);
#21394=VERTEX_POINT('',#74752);
#21395=VERTEX_POINT('',#74754);
#21396=VERTEX_POINT('',#74758);
#21397=VERTEX_POINT('',#74760);
#21398=VERTEX_POINT('',#74764);
#21399=VERTEX_POINT('',#74766);
#21400=VERTEX_POINT('',#74770);
#21401=VERTEX_POINT('',#74772);
#21402=VERTEX_POINT('',#74776);
#21403=VERTEX_POINT('',#74778);
#21404=VERTEX_POINT('',#74780);
#21405=VERTEX_POINT('',#74793);
#21406=VERTEX_POINT('',#74817);
#21407=VERTEX_POINT('',#74819);
#21408=VERTEX_POINT('',#74823);
#21409=VERTEX_POINT('',#74825);
#21410=VERTEX_POINT('',#74829);
#21411=VERTEX_POINT('',#74831);
#21412=VERTEX_POINT('',#74835);
#21413=VERTEX_POINT('',#74837);
#21414=VERTEX_POINT('',#74841);
#21415=VERTEX_POINT('',#74843);
#21416=VERTEX_POINT('',#74847);
#21417=VERTEX_POINT('',#74849);
#21418=VERTEX_POINT('',#74853);
#21419=VERTEX_POINT('',#74855);
#21420=VERTEX_POINT('',#74859);
#21421=VERTEX_POINT('',#74861);
#21422=VERTEX_POINT('',#74865);
#21423=VERTEX_POINT('',#74867);
#21424=VERTEX_POINT('',#74871);
#21425=VERTEX_POINT('',#74873);
#21426=VERTEX_POINT('',#74877);
#21427=VERTEX_POINT('',#74879);
#21428=VERTEX_POINT('',#74883);
#21429=VERTEX_POINT('',#74885);
#21430=VERTEX_POINT('',#74889);
#21431=VERTEX_POINT('',#74891);
#21432=VERTEX_POINT('',#74895);
#21433=VERTEX_POINT('',#74897);
#21434=VERTEX_POINT('',#74901);
#21435=VERTEX_POINT('',#74903);
#21436=VERTEX_POINT('',#74907);
#21437=VERTEX_POINT('',#74909);
#21438=VERTEX_POINT('',#74913);
#21439=VERTEX_POINT('',#74915);
#21440=VERTEX_POINT('',#74919);
#21441=VERTEX_POINT('',#74921);
#21442=VERTEX_POINT('',#74923);
#21443=VERTEX_POINT('',#74934);
#21444=VERTEX_POINT('',#74960);
#21445=VERTEX_POINT('',#74962);
#21446=VERTEX_POINT('',#74966);
#21447=VERTEX_POINT('',#74968);
#21448=VERTEX_POINT('',#74972);
#21449=VERTEX_POINT('',#74974);
#21450=VERTEX_POINT('',#74978);
#21451=VERTEX_POINT('',#74980);
#21452=VERTEX_POINT('',#74984);
#21453=VERTEX_POINT('',#74986);
#21454=VERTEX_POINT('',#74990);
#21455=VERTEX_POINT('',#74992);
#21456=VERTEX_POINT('',#74996);
#21457=VERTEX_POINT('',#74998);
#21458=VERTEX_POINT('',#75002);
#21459=VERTEX_POINT('',#75004);
#21460=VERTEX_POINT('',#75008);
#21461=VERTEX_POINT('',#75010);
#21462=VERTEX_POINT('',#75014);
#21463=VERTEX_POINT('',#75016);
#21464=VERTEX_POINT('',#75020);
#21465=VERTEX_POINT('',#75022);
#21466=VERTEX_POINT('',#75026);
#21467=VERTEX_POINT('',#75028);
#21468=VERTEX_POINT('',#75032);
#21469=VERTEX_POINT('',#75034);
#21470=VERTEX_POINT('',#75038);
#21471=VERTEX_POINT('',#75040);
#21472=VERTEX_POINT('',#75044);
#21473=VERTEX_POINT('',#75046);
#21474=VERTEX_POINT('',#75050);
#21475=VERTEX_POINT('',#75052);
#21476=VERTEX_POINT('',#75054);
#21477=VERTEX_POINT('',#75065);
#21478=VERTEX_POINT('',#75091);
#21479=VERTEX_POINT('',#75093);
#21480=VERTEX_POINT('',#75097);
#21481=VERTEX_POINT('',#75099);
#21482=VERTEX_POINT('',#75103);
#21483=VERTEX_POINT('',#75105);
#21484=VERTEX_POINT('',#75109);
#21485=VERTEX_POINT('',#75111);
#21486=VERTEX_POINT('',#75115);
#21487=VERTEX_POINT('',#75117);
#21488=VERTEX_POINT('',#75121);
#21489=VERTEX_POINT('',#75123);
#21490=VERTEX_POINT('',#75127);
#21491=VERTEX_POINT('',#75129);
#21492=VERTEX_POINT('',#75133);
#21493=VERTEX_POINT('',#75135);
#21494=VERTEX_POINT('',#75139);
#21495=VERTEX_POINT('',#75141);
#21496=VERTEX_POINT('',#75145);
#21497=VERTEX_POINT('',#75147);
#21498=VERTEX_POINT('',#75151);
#21499=VERTEX_POINT('',#75153);
#21500=VERTEX_POINT('',#75157);
#21501=VERTEX_POINT('',#75159);
#21502=VERTEX_POINT('',#75163);
#21503=VERTEX_POINT('',#75165);
#21504=VERTEX_POINT('',#75169);
#21505=VERTEX_POINT('',#75171);
#21506=VERTEX_POINT('',#75175);
#21507=VERTEX_POINT('',#75177);
#21508=VERTEX_POINT('',#75181);
#21509=VERTEX_POINT('',#75183);
#21510=VERTEX_POINT('',#75187);
#21511=VERTEX_POINT('',#75189);
#21512=VERTEX_POINT('',#75193);
#21513=VERTEX_POINT('',#75195);
#21514=VERTEX_POINT('',#75197);
#21515=VERTEX_POINT('',#75206);
#21516=VERTEX_POINT('',#75234);
#21517=VERTEX_POINT('',#75236);
#21518=VERTEX_POINT('',#75240);
#21519=VERTEX_POINT('',#75242);
#21520=VERTEX_POINT('',#75246);
#21521=VERTEX_POINT('',#75248);
#21522=VERTEX_POINT('',#75252);
#21523=VERTEX_POINT('',#75254);
#21524=VERTEX_POINT('',#75258);
#21525=VERTEX_POINT('',#75260);
#21526=VERTEX_POINT('',#75264);
#21527=VERTEX_POINT('',#75266);
#21528=VERTEX_POINT('',#75270);
#21529=VERTEX_POINT('',#75272);
#21530=VERTEX_POINT('',#75276);
#21531=VERTEX_POINT('',#75278);
#21532=VERTEX_POINT('',#75282);
#21533=VERTEX_POINT('',#75284);
#21534=VERTEX_POINT('',#75288);
#21535=VERTEX_POINT('',#75290);
#21536=VERTEX_POINT('',#75294);
#21537=VERTEX_POINT('',#75296);
#21538=VERTEX_POINT('',#75300);
#21539=VERTEX_POINT('',#75302);
#21540=VERTEX_POINT('',#75306);
#21541=VERTEX_POINT('',#75308);
#21542=VERTEX_POINT('',#75312);
#21543=VERTEX_POINT('',#75314);
#21544=VERTEX_POINT('',#75318);
#21545=VERTEX_POINT('',#75320);
#21546=VERTEX_POINT('',#75324);
#21547=VERTEX_POINT('',#75326);
#21548=VERTEX_POINT('',#75330);
#21549=VERTEX_POINT('',#75332);
#21550=VERTEX_POINT('',#75336);
#21551=VERTEX_POINT('',#75338);
#21552=VERTEX_POINT('',#75340);
#21553=VERTEX_POINT('',#75349);
#21554=VERTEX_POINT('',#75377);
#21555=VERTEX_POINT('',#75379);
#21556=VERTEX_POINT('',#75383);
#21557=VERTEX_POINT('',#75385);
#21558=VERTEX_POINT('',#75389);
#21559=VERTEX_POINT('',#75391);
#21560=VERTEX_POINT('',#75395);
#21561=VERTEX_POINT('',#75397);
#21562=VERTEX_POINT('',#75401);
#21563=VERTEX_POINT('',#75403);
#21564=VERTEX_POINT('',#75407);
#21565=VERTEX_POINT('',#75409);
#21566=VERTEX_POINT('',#75413);
#21567=VERTEX_POINT('',#75415);
#21568=VERTEX_POINT('',#75419);
#21569=VERTEX_POINT('',#75421);
#21570=VERTEX_POINT('',#75425);
#21571=VERTEX_POINT('',#75427);
#21572=VERTEX_POINT('',#75431);
#21573=VERTEX_POINT('',#75433);
#21574=VERTEX_POINT('',#75437);
#21575=VERTEX_POINT('',#75439);
#21576=VERTEX_POINT('',#75443);
#21577=VERTEX_POINT('',#75445);
#21578=VERTEX_POINT('',#75449);
#21579=VERTEX_POINT('',#75451);
#21580=VERTEX_POINT('',#75455);
#21581=VERTEX_POINT('',#75457);
#21582=VERTEX_POINT('',#75461);
#21583=VERTEX_POINT('',#75463);
#21584=VERTEX_POINT('',#75467);
#21585=VERTEX_POINT('',#75469);
#21586=VERTEX_POINT('',#75473);
#21587=VERTEX_POINT('',#75475);
#21588=VERTEX_POINT('',#75479);
#21589=VERTEX_POINT('',#75481);
#21590=VERTEX_POINT('',#75483);
#21591=VERTEX_POINT('',#75490);
#21592=VERTEX_POINT('',#75520);
#21593=VERTEX_POINT('',#75522);
#21594=VERTEX_POINT('',#75526);
#21595=VERTEX_POINT('',#75528);
#21596=VERTEX_POINT('',#75532);
#21597=VERTEX_POINT('',#75534);
#21598=VERTEX_POINT('',#75538);
#21599=VERTEX_POINT('',#75540);
#21600=VERTEX_POINT('',#75544);
#21601=VERTEX_POINT('',#75546);
#21602=VERTEX_POINT('',#75550);
#21603=VERTEX_POINT('',#75552);
#21604=VERTEX_POINT('',#75556);
#21605=VERTEX_POINT('',#75558);
#21606=VERTEX_POINT('',#75562);
#21607=VERTEX_POINT('',#75564);
#21608=VERTEX_POINT('',#75568);
#21609=VERTEX_POINT('',#75570);
#21610=VERTEX_POINT('',#75574);
#21611=VERTEX_POINT('',#75576);
#21612=VERTEX_POINT('',#75580);
#21613=VERTEX_POINT('',#75582);
#21614=VERTEX_POINT('',#75586);
#21615=VERTEX_POINT('',#75588);
#21616=VERTEX_POINT('',#75592);
#21617=VERTEX_POINT('',#75594);
#21618=VERTEX_POINT('',#75598);
#21619=VERTEX_POINT('',#75600);
#21620=VERTEX_POINT('',#75604);
#21621=VERTEX_POINT('',#75606);
#21622=VERTEX_POINT('',#75610);
#21623=VERTEX_POINT('',#75612);
#21624=VERTEX_POINT('',#75616);
#21625=VERTEX_POINT('',#75618);
#21626=VERTEX_POINT('',#75622);
#21627=VERTEX_POINT('',#75624);
#21628=VERTEX_POINT('',#75626);
#21629=VERTEX_POINT('',#75631);
#21630=VERTEX_POINT('',#75663);
#21631=VERTEX_POINT('',#75665);
#21632=VERTEX_POINT('',#75669);
#21633=VERTEX_POINT('',#75671);
#21634=VERTEX_POINT('',#75675);
#21635=VERTEX_POINT('',#75677);
#21636=VERTEX_POINT('',#75681);
#21637=VERTEX_POINT('',#75683);
#21638=VERTEX_POINT('',#75687);
#21639=VERTEX_POINT('',#75689);
#21640=VERTEX_POINT('',#75693);
#21641=VERTEX_POINT('',#75695);
#21642=VERTEX_POINT('',#75699);
#21643=VERTEX_POINT('',#75701);
#21644=VERTEX_POINT('',#75705);
#21645=VERTEX_POINT('',#75707);
#21646=VERTEX_POINT('',#75711);
#21647=VERTEX_POINT('',#75713);
#21648=VERTEX_POINT('',#75717);
#21649=VERTEX_POINT('',#75719);
#21650=VERTEX_POINT('',#75723);
#21651=VERTEX_POINT('',#75725);
#21652=VERTEX_POINT('',#75729);
#21653=VERTEX_POINT('',#75731);
#21654=VERTEX_POINT('',#75735);
#21655=VERTEX_POINT('',#75737);
#21656=VERTEX_POINT('',#75741);
#21657=VERTEX_POINT('',#75743);
#21658=VERTEX_POINT('',#75747);
#21659=VERTEX_POINT('',#75749);
#21660=VERTEX_POINT('',#75753);
#21661=VERTEX_POINT('',#75755);
#21662=VERTEX_POINT('',#75757);
#21663=VERTEX_POINT('',#75762);
#21664=VERTEX_POINT('',#75794);
#21665=VERTEX_POINT('',#75796);
#21666=VERTEX_POINT('',#75800);
#21667=VERTEX_POINT('',#75802);
#21668=VERTEX_POINT('',#75806);
#21669=VERTEX_POINT('',#75808);
#21670=VERTEX_POINT('',#75812);
#21671=VERTEX_POINT('',#75814);
#21672=VERTEX_POINT('',#75818);
#21673=VERTEX_POINT('',#75820);
#21674=VERTEX_POINT('',#75824);
#21675=VERTEX_POINT('',#75826);
#21676=VERTEX_POINT('',#75830);
#21677=VERTEX_POINT('',#75832);
#21678=VERTEX_POINT('',#75836);
#21679=VERTEX_POINT('',#75838);
#21680=VERTEX_POINT('',#75842);
#21681=VERTEX_POINT('',#75844);
#21682=VERTEX_POINT('',#75848);
#21683=VERTEX_POINT('',#75850);
#21684=VERTEX_POINT('',#75854);
#21685=VERTEX_POINT('',#75856);
#21686=VERTEX_POINT('',#75860);
#21687=VERTEX_POINT('',#75862);
#21688=VERTEX_POINT('',#75866);
#21689=VERTEX_POINT('',#75868);
#21690=VERTEX_POINT('',#75872);
#21691=VERTEX_POINT('',#75874);
#21692=VERTEX_POINT('',#75878);
#21693=VERTEX_POINT('',#75880);
#21694=VERTEX_POINT('',#75884);
#21695=VERTEX_POINT('',#75886);
#21696=VERTEX_POINT('',#75890);
#21697=VERTEX_POINT('',#75892);
#21698=VERTEX_POINT('',#75896);
#21699=VERTEX_POINT('',#75898);
#21700=VERTEX_POINT('',#75900);
#21701=VERTEX_POINT('',#75902);
#21702=VERTEX_POINT('',#75934);
#21703=VERTEX_POINT('',#75936);
#21704=VERTEX_POINT('',#75940);
#21705=VERTEX_POINT('',#75942);
#21706=VERTEX_POINT('',#75946);
#21707=VERTEX_POINT('',#75948);
#21708=VERTEX_POINT('',#75952);
#21709=VERTEX_POINT('',#75954);
#21710=VERTEX_POINT('',#75958);
#21711=VERTEX_POINT('',#75960);
#21712=VERTEX_POINT('',#75964);
#21713=VERTEX_POINT('',#75966);
#21714=VERTEX_POINT('',#75970);
#21715=VERTEX_POINT('',#75972);
#21716=VERTEX_POINT('',#75976);
#21717=VERTEX_POINT('',#75978);
#21718=VERTEX_POINT('',#75982);
#21719=VERTEX_POINT('',#75984);
#21720=VERTEX_POINT('',#75988);
#21721=VERTEX_POINT('',#75990);
#21722=VERTEX_POINT('',#75994);
#21723=VERTEX_POINT('',#75996);
#21724=VERTEX_POINT('',#76000);
#21725=VERTEX_POINT('',#76002);
#21726=VERTEX_POINT('',#76006);
#21727=VERTEX_POINT('',#76008);
#21728=VERTEX_POINT('',#76012);
#21729=VERTEX_POINT('',#76014);
#21730=VERTEX_POINT('',#76018);
#21731=VERTEX_POINT('',#76020);
#21732=VERTEX_POINT('',#76024);
#21733=VERTEX_POINT('',#76026);
#21734=VERTEX_POINT('',#76028);
#21735=VERTEX_POINT('',#76030);
#21736=VERTEX_POINT('',#76045);
#21737=VERTEX_POINT('',#76047);
#21738=VERTEX_POINT('',#76051);
#21739=VERTEX_POINT('',#76053);
#21740=VERTEX_POINT('',#76055);
#21741=VERTEX_POINT('',#76057);
#21742=VERTEX_POINT('',#76096);
#21743=VERTEX_POINT('',#76098);
#21744=VERTEX_POINT('',#76102);
#21745=VERTEX_POINT('',#76104);
#21746=VERTEX_POINT('',#76108);
#21747=VERTEX_POINT('',#76110);
#21748=VERTEX_POINT('',#76114);
#21749=VERTEX_POINT('',#76116);
#21750=VERTEX_POINT('',#76120);
#21751=VERTEX_POINT('',#76122);
#21752=VERTEX_POINT('',#76126);
#21753=VERTEX_POINT('',#76128);
#21754=VERTEX_POINT('',#76132);
#21755=VERTEX_POINT('',#76134);
#21756=VERTEX_POINT('',#76138);
#21757=VERTEX_POINT('',#76140);
#21758=VERTEX_POINT('',#76144);
#21759=VERTEX_POINT('',#76146);
#21760=VERTEX_POINT('',#76150);
#21761=VERTEX_POINT('',#76152);
#21762=VERTEX_POINT('',#76156);
#21763=VERTEX_POINT('',#76158);
#21764=VERTEX_POINT('',#76162);
#21765=VERTEX_POINT('',#76164);
#21766=VERTEX_POINT('',#76168);
#21767=VERTEX_POINT('',#76170);
#21768=VERTEX_POINT('',#76174);
#21769=VERTEX_POINT('',#76176);
#21770=VERTEX_POINT('',#76178);
#21771=VERTEX_POINT('',#76180);
#21772=VERTEX_POINT('',#76197);
#21773=VERTEX_POINT('',#76199);
#21774=VERTEX_POINT('',#76203);
#21775=VERTEX_POINT('',#76205);
#21776=VERTEX_POINT('',#76209);
#21777=VERTEX_POINT('',#76211);
#21778=VERTEX_POINT('',#76215);
#21779=VERTEX_POINT('',#76217);
#21780=VERTEX_POINT('',#76221);
#21781=VERTEX_POINT('',#76223);
#21782=VERTEX_POINT('',#76227);
#21783=VERTEX_POINT('',#76229);
#21784=VERTEX_POINT('',#76233);
#21785=VERTEX_POINT('',#76235);
#21786=VERTEX_POINT('',#76239);
#21787=VERTEX_POINT('',#76241);
#21788=VERTEX_POINT('',#76245);
#21789=VERTEX_POINT('',#76247);
#21790=VERTEX_POINT('',#76251);
#21791=VERTEX_POINT('',#76253);
#21792=VERTEX_POINT('',#76257);
#21793=VERTEX_POINT('',#76259);
#21794=VERTEX_POINT('',#76263);
#21795=VERTEX_POINT('',#76265);
#21796=VERTEX_POINT('',#76269);
#21797=VERTEX_POINT('',#76271);
#21798=VERTEX_POINT('',#76275);
#21799=VERTEX_POINT('',#76277);
#21800=VERTEX_POINT('',#76281);
#21801=VERTEX_POINT('',#76283);
#21802=VERTEX_POINT('',#76287);
#21803=VERTEX_POINT('',#76289);
#21804=VERTEX_POINT('',#76293);
#21805=VERTEX_POINT('',#76295);
#21806=VERTEX_POINT('',#76299);
#21807=VERTEX_POINT('',#76301);
#21808=VERTEX_POINT('',#76305);
#21809=VERTEX_POINT('',#76307);
#21810=VERTEX_POINT('',#76311);
#21811=VERTEX_POINT('',#76313);
#21812=VERTEX_POINT('',#76317);
#21813=VERTEX_POINT('',#76319);
#21814=VERTEX_POINT('',#76323);
#21815=VERTEX_POINT('',#76325);
#21816=VERTEX_POINT('',#76329);
#21817=VERTEX_POINT('',#76331);
#21818=VERTEX_POINT('',#76335);
#21819=VERTEX_POINT('',#76337);
#21820=VERTEX_POINT('',#76341);
#21821=VERTEX_POINT('',#76343);
#21822=VERTEX_POINT('',#76347);
#21823=VERTEX_POINT('',#76349);
#21824=VERTEX_POINT('',#76353);
#21825=VERTEX_POINT('',#76355);
#21826=VERTEX_POINT('',#76359);
#21827=VERTEX_POINT('',#76361);
#21828=VERTEX_POINT('',#76363);
#21829=VERTEX_POINT('',#76365);
#21830=VERTEX_POINT('',#76392);
#21831=VERTEX_POINT('',#76394);
#21832=VERTEX_POINT('',#76398);
#21833=VERTEX_POINT('',#76400);
#21834=VERTEX_POINT('',#76404);
#21835=VERTEX_POINT('',#76406);
#21836=VERTEX_POINT('',#76410);
#21837=VERTEX_POINT('',#76412);
#21838=VERTEX_POINT('',#76416);
#21839=VERTEX_POINT('',#76418);
#21840=VERTEX_POINT('',#76422);
#21841=VERTEX_POINT('',#76424);
#21842=VERTEX_POINT('',#76428);
#21843=VERTEX_POINT('',#76430);
#21844=VERTEX_POINT('',#76434);
#21845=VERTEX_POINT('',#76436);
#21846=VERTEX_POINT('',#76440);
#21847=VERTEX_POINT('',#76442);
#21848=VERTEX_POINT('',#76446);
#21849=VERTEX_POINT('',#76448);
#21850=VERTEX_POINT('',#76452);
#21851=VERTEX_POINT('',#76454);
#21852=VERTEX_POINT('',#76458);
#21853=VERTEX_POINT('',#76460);
#21854=VERTEX_POINT('',#76464);
#21855=VERTEX_POINT('',#76466);
#21856=VERTEX_POINT('',#76470);
#21857=VERTEX_POINT('',#76472);
#21858=VERTEX_POINT('',#76476);
#21859=VERTEX_POINT('',#76478);
#21860=VERTEX_POINT('',#76482);
#21861=VERTEX_POINT('',#76484);
#21862=VERTEX_POINT('',#76488);
#21863=VERTEX_POINT('',#76490);
#21864=VERTEX_POINT('',#76494);
#21865=VERTEX_POINT('',#76496);
#21866=VERTEX_POINT('',#76500);
#21867=VERTEX_POINT('',#76502);
#21868=VERTEX_POINT('',#76506);
#21869=VERTEX_POINT('',#76508);
#21870=VERTEX_POINT('',#76512);
#21871=VERTEX_POINT('',#76514);
#21872=VERTEX_POINT('',#76518);
#21873=VERTEX_POINT('',#76520);
#21874=VERTEX_POINT('',#76524);
#21875=VERTEX_POINT('',#76526);
#21876=VERTEX_POINT('',#76530);
#21877=VERTEX_POINT('',#76532);
#21878=VERTEX_POINT('',#76536);
#21879=VERTEX_POINT('',#76538);
#21880=VERTEX_POINT('',#76542);
#21881=VERTEX_POINT('',#76544);
#21882=VERTEX_POINT('',#76548);
#21883=VERTEX_POINT('',#76550);
#21884=VERTEX_POINT('',#76554);
#21885=VERTEX_POINT('',#76556);
#21886=VERTEX_POINT('',#76560);
#21887=VERTEX_POINT('',#76562);
#21888=VERTEX_POINT('',#76566);
#21889=VERTEX_POINT('',#76568);
#21890=VERTEX_POINT('',#76572);
#21891=VERTEX_POINT('',#76574);
#21892=VERTEX_POINT('',#76578);
#21893=VERTEX_POINT('',#76580);
#21894=VERTEX_POINT('',#76584);
#21895=VERTEX_POINT('',#76586);
#21896=VERTEX_POINT('',#76590);
#21897=VERTEX_POINT('',#76592);
#21898=VERTEX_POINT('',#76594);
#21899=VERTEX_POINT('',#76596);
#21900=VERTEX_POINT('',#76607);
#21901=VERTEX_POINT('',#76638);
#21902=VERTEX_POINT('',#76640);
#21903=VERTEX_POINT('',#76644);
#21904=VERTEX_POINT('',#76646);
#21905=VERTEX_POINT('',#76650);
#21906=VERTEX_POINT('',#76652);
#21907=VERTEX_POINT('',#76656);
#21908=VERTEX_POINT('',#76658);
#21909=VERTEX_POINT('',#76662);
#21910=VERTEX_POINT('',#76664);
#21911=VERTEX_POINT('',#76668);
#21912=VERTEX_POINT('',#76670);
#21913=VERTEX_POINT('',#76674);
#21914=VERTEX_POINT('',#76676);
#21915=VERTEX_POINT('',#76680);
#21916=VERTEX_POINT('',#76682);
#21917=VERTEX_POINT('',#76686);
#21918=VERTEX_POINT('',#76688);
#21919=VERTEX_POINT('',#76692);
#21920=VERTEX_POINT('',#76694);
#21921=VERTEX_POINT('',#76698);
#21922=VERTEX_POINT('',#76700);
#21923=VERTEX_POINT('',#76704);
#21924=VERTEX_POINT('',#76706);
#21925=VERTEX_POINT('',#76710);
#21926=VERTEX_POINT('',#76712);
#21927=VERTEX_POINT('',#76716);
#21928=VERTEX_POINT('',#76718);
#21929=VERTEX_POINT('',#76722);
#21930=VERTEX_POINT('',#76724);
#21931=VERTEX_POINT('',#76728);
#21932=VERTEX_POINT('',#76730);
#21933=VERTEX_POINT('',#76734);
#21934=VERTEX_POINT('',#76736);
#21935=VERTEX_POINT('',#76740);
#21936=VERTEX_POINT('',#76742);
#21937=VERTEX_POINT('',#76744);
#21938=VERTEX_POINT('',#76746);
#21939=VERTEX_POINT('',#76778);
#21940=VERTEX_POINT('',#76780);
#21941=VERTEX_POINT('',#76784);
#21942=VERTEX_POINT('',#76786);
#21943=VERTEX_POINT('',#76790);
#21944=VERTEX_POINT('',#76792);
#21945=VERTEX_POINT('',#76796);
#21946=VERTEX_POINT('',#76798);
#21947=VERTEX_POINT('',#76802);
#21948=VERTEX_POINT('',#76804);
#21949=VERTEX_POINT('',#76808);
#21950=VERTEX_POINT('',#76810);
#21951=VERTEX_POINT('',#76814);
#21952=VERTEX_POINT('',#76816);
#21953=VERTEX_POINT('',#76820);
#21954=VERTEX_POINT('',#76822);
#21955=VERTEX_POINT('',#76826);
#21956=VERTEX_POINT('',#76828);
#21957=VERTEX_POINT('',#76832);
#21958=VERTEX_POINT('',#76834);
#21959=VERTEX_POINT('',#76838);
#21960=VERTEX_POINT('',#76840);
#21961=VERTEX_POINT('',#76844);
#21962=VERTEX_POINT('',#76846);
#21963=VERTEX_POINT('',#76850);
#21964=VERTEX_POINT('',#76852);
#21965=VERTEX_POINT('',#76856);
#21966=VERTEX_POINT('',#76858);
#21967=VERTEX_POINT('',#76862);
#21968=VERTEX_POINT('',#76864);
#21969=VERTEX_POINT('',#76868);
#21970=VERTEX_POINT('',#76870);
#21971=VERTEX_POINT('',#76874);
#21972=VERTEX_POINT('',#76876);
#21973=VERTEX_POINT('',#76880);
#21974=VERTEX_POINT('',#76882);
#21975=VERTEX_POINT('',#76884);
#21976=VERTEX_POINT('',#76914);
#21977=VERTEX_POINT('',#76921);
#21978=VERTEX_POINT('',#76923);
#21979=VERTEX_POINT('',#76927);
#21980=VERTEX_POINT('',#76929);
#21981=VERTEX_POINT('',#76933);
#21982=VERTEX_POINT('',#76935);
#21983=VERTEX_POINT('',#76939);
#21984=VERTEX_POINT('',#76941);
#21985=VERTEX_POINT('',#76945);
#21986=VERTEX_POINT('',#76947);
#21987=VERTEX_POINT('',#76951);
#21988=VERTEX_POINT('',#76953);
#21989=VERTEX_POINT('',#76957);
#21990=VERTEX_POINT('',#76959);
#21991=VERTEX_POINT('',#76963);
#21992=VERTEX_POINT('',#76965);
#21993=VERTEX_POINT('',#76969);
#21994=VERTEX_POINT('',#76971);
#21995=VERTEX_POINT('',#76975);
#21996=VERTEX_POINT('',#76977);
#21997=VERTEX_POINT('',#76981);
#21998=VERTEX_POINT('',#76983);
#21999=VERTEX_POINT('',#76987);
#22000=VERTEX_POINT('',#76989);
#22001=VERTEX_POINT('',#76993);
#22002=VERTEX_POINT('',#76995);
#22003=VERTEX_POINT('',#76999);
#22004=VERTEX_POINT('',#77001);
#22005=VERTEX_POINT('',#77005);
#22006=VERTEX_POINT('',#77007);
#22007=VERTEX_POINT('',#77011);
#22008=VERTEX_POINT('',#77013);
#22009=VERTEX_POINT('',#77015);
#22010=VERTEX_POINT('',#77045);
#22011=VERTEX_POINT('',#77052);
#22012=VERTEX_POINT('',#77054);
#22013=VERTEX_POINT('',#77058);
#22014=VERTEX_POINT('',#77060);
#22015=VERTEX_POINT('',#77064);
#22016=VERTEX_POINT('',#77066);
#22017=VERTEX_POINT('',#77070);
#22018=VERTEX_POINT('',#77072);
#22019=VERTEX_POINT('',#77076);
#22020=VERTEX_POINT('',#77078);
#22021=VERTEX_POINT('',#77082);
#22022=VERTEX_POINT('',#77084);
#22023=VERTEX_POINT('',#77088);
#22024=VERTEX_POINT('',#77090);
#22025=VERTEX_POINT('',#77094);
#22026=VERTEX_POINT('',#77096);
#22027=VERTEX_POINT('',#77100);
#22028=VERTEX_POINT('',#77102);
#22029=VERTEX_POINT('',#77106);
#22030=VERTEX_POINT('',#77108);
#22031=VERTEX_POINT('',#77112);
#22032=VERTEX_POINT('',#77114);
#22033=VERTEX_POINT('',#77118);
#22034=VERTEX_POINT('',#77120);
#22035=VERTEX_POINT('',#77124);
#22036=VERTEX_POINT('',#77126);
#22037=VERTEX_POINT('',#77130);
#22038=VERTEX_POINT('',#77132);
#22039=VERTEX_POINT('',#77136);
#22040=VERTEX_POINT('',#77138);
#22041=VERTEX_POINT('',#77142);
#22042=VERTEX_POINT('',#77144);
#22043=VERTEX_POINT('',#77148);
#22044=VERTEX_POINT('',#77150);
#22045=VERTEX_POINT('',#77154);
#22046=VERTEX_POINT('',#77156);
#22047=VERTEX_POINT('',#77158);
#22048=VERTEX_POINT('',#77186);
#22049=VERTEX_POINT('',#77195);
#22050=VERTEX_POINT('',#77197);
#22051=VERTEX_POINT('',#77201);
#22052=VERTEX_POINT('',#77203);
#22053=VERTEX_POINT('',#77207);
#22054=VERTEX_POINT('',#77209);
#22055=VERTEX_POINT('',#77213);
#22056=VERTEX_POINT('',#77215);
#22057=VERTEX_POINT('',#77219);
#22058=VERTEX_POINT('',#77221);
#22059=VERTEX_POINT('',#77225);
#22060=VERTEX_POINT('',#77227);
#22061=VERTEX_POINT('',#77231);
#22062=VERTEX_POINT('',#77233);
#22063=VERTEX_POINT('',#77237);
#22064=VERTEX_POINT('',#77239);
#22065=VERTEX_POINT('',#77243);
#22066=VERTEX_POINT('',#77245);
#22067=VERTEX_POINT('',#77249);
#22068=VERTEX_POINT('',#77251);
#22069=VERTEX_POINT('',#77255);
#22070=VERTEX_POINT('',#77257);
#22071=VERTEX_POINT('',#77261);
#22072=VERTEX_POINT('',#77263);
#22073=VERTEX_POINT('',#77267);
#22074=VERTEX_POINT('',#77269);
#22075=VERTEX_POINT('',#77273);
#22076=VERTEX_POINT('',#77275);
#22077=VERTEX_POINT('',#77279);
#22078=VERTEX_POINT('',#77281);
#22079=VERTEX_POINT('',#77285);
#22080=VERTEX_POINT('',#77287);
#22081=VERTEX_POINT('',#77291);
#22082=VERTEX_POINT('',#77293);
#22083=VERTEX_POINT('',#77297);
#22084=VERTEX_POINT('',#77299);
#22085=VERTEX_POINT('',#77301);
#22086=VERTEX_POINT('',#77327);
#22087=VERTEX_POINT('',#77338);
#22088=VERTEX_POINT('',#77340);
#22089=VERTEX_POINT('',#77370);
#22090=VERTEX_POINT('',#77371);
#22091=VERTEX_POINT('',#77398);
#22092=VERTEX_POINT('',#77401);
#22093=VERTEX_POINT('',#77402);
#22094=VERTEX_POINT('',#77447);
#22095=VERTEX_POINT('',#77448);
#22096=VERTEX_POINT('',#77450);
#22097=VERTEX_POINT('',#77452);
#22098=VERTEX_POINT('',#77457);
#22099=VERTEX_POINT('',#77462);
#22100=VERTEX_POINT('',#77623);
#22101=VERTEX_POINT('',#77784);
#22102=VERTEX_POINT('',#77789);
#22103=VERTEX_POINT('',#77796);
#22104=VERTEX_POINT('',#77797);
#22105=VERTEX_POINT('',#77799);
#22106=VERTEX_POINT('',#77804);
#22107=VERTEX_POINT('',#77808);
#22108=VERTEX_POINT('',#77810);
#22109=VERTEX_POINT('',#77814);
#22110=VERTEX_POINT('',#77815);
#22111=VERTEX_POINT('',#77817);
#22112=VERTEX_POINT('',#77828);
#22113=VERTEX_POINT('',#77841);
#22114=VERTEX_POINT('',#77842);
#22115=VERTEX_POINT('',#77844);
#22116=VERTEX_POINT('',#77846);
#22117=VERTEX_POINT('',#77850);
#22118=VERTEX_POINT('',#77851);
#22119=VERTEX_POINT('',#77853);
#22120=VERTEX_POINT('',#77855);
#22121=VERTEX_POINT('',#77857);
#22122=VERTEX_POINT('',#77894);
#22123=VERTEX_POINT('',#77895);
#22124=VERTEX_POINT('',#77900);
#22125=VERTEX_POINT('',#77904);
#22126=VERTEX_POINT('',#77906);
#22127=VERTEX_POINT('',#77943);
#22128=VERTEX_POINT('',#77944);
#22129=VERTEX_POINT('',#78002);
#22130=VERTEX_POINT('',#78003);
#22131=VERTEX_POINT('',#78005);
#22132=VERTEX_POINT('',#78028);
#22133=VERTEX_POINT('',#78030);
#22134=VERTEX_POINT('',#78039);
#22135=VERTEX_POINT('',#78043);
#22136=VERTEX_POINT('',#78044);
#22137=VERTEX_POINT('',#78046);
#22138=VERTEX_POINT('',#78071);
#22139=VERTEX_POINT('',#78090);
#22140=VERTEX_POINT('',#78094);
#22141=VERTEX_POINT('',#78095);
#22142=VERTEX_POINT('',#78097);
#22143=VERTEX_POINT('',#78100);
#22144=VERTEX_POINT('',#78104);
#22145=VERTEX_POINT('',#78113);
#22146=VERTEX_POINT('',#78114);
#22147=VERTEX_POINT('',#78147);
#22148=VERTEX_POINT('',#78148);
#22149=VERTEX_POINT('',#78150);
#22150=VERTEX_POINT('',#78152);
#22151=VERTEX_POINT('',#78156);
#22152=VERTEX_POINT('',#78157);
#22153=VERTEX_POINT('',#78159);
#22154=VERTEX_POINT('',#78164);
#22155=VERTEX_POINT('',#78165);
#22156=VERTEX_POINT('',#78170);
#22157=VERTEX_POINT('',#78184);
#22158=VERTEX_POINT('',#78186);
#22159=VERTEX_POINT('',#78188);
#22160=VERTEX_POINT('',#78190);
#22161=VERTEX_POINT('',#78354);
#22162=VERTEX_POINT('',#78356);
#22163=VERTEX_POINT('',#78361);
#22164=VERTEX_POINT('',#78559);
#22165=VERTEX_POINT('',#78560);
#22166=VERTEX_POINT('',#78904);
#22167=VERTEX_POINT('',#78931);
#22168=VERTEX_POINT('',#78984);
#22169=VERTEX_POINT('',#79073);
#22170=VERTEX_POINT('',#79075);
#22171=VERTEX_POINT('',#79080);
#22172=VERTEX_POINT('',#79200);
#22173=VERTEX_POINT('',#79201);
#22174=VERTEX_POINT('',#79203);
#22175=VERTEX_POINT('',#79229);
#22176=VERTEX_POINT('',#79513);
#22177=VERTEX_POINT('',#79566);
#22178=VERTEX_POINT('',#79568);
#22179=VERTEX_POINT('',#79587);
#22180=VERTEX_POINT('',#79588);
#22181=VERTEX_POINT('',#79616);
#22182=VERTEX_POINT('',#79617);
#22183=VERTEX_POINT('',#79678);
#22184=VERTEX_POINT('',#79679);
#22185=VERTEX_POINT('',#79766);
#22186=VERTEX_POINT('',#79880);
#22187=VERTEX_POINT('',#79908);
#22188=VERTEX_POINT('',#79915);
#22189=VERTEX_POINT('',#79923);
#22190=VERTEX_POINT('',#79925);
#22191=VERTEX_POINT('',#80014);
#22192=VERTEX_POINT('',#80130);
#22193=VERTEX_POINT('',#80331);
#22194=VERTEX_POINT('',#80450);
#22195=VERTEX_POINT('',#80714);
#22196=VERTEX_POINT('',#81047);
#22197=VERTEX_POINT('',#81090);
#22198=VERTEX_POINT('',#81091);
#22199=VERTEX_POINT('',#81613);
#22200=VERTEX_POINT('',#81618);
#22201=VERTEX_POINT('',#81626);
#22202=VERTEX_POINT('',#81778);
#24515=EDGE_CURVE('',#20643,#20644,#4315,.T.);
#24516=EDGE_CURVE('',#20643,#20645,#2912,.T.);
#24517=EDGE_CURVE('',#20646,#20645,#4316,.T.);
#24518=EDGE_CURVE('',#20646,#20644,#4317,.T.);
#24519=EDGE_CURVE('',#20646,#20647,#4318,.T.);
#24520=EDGE_CURVE('',#20647,#20648,#17713,.T.);
#24521=EDGE_CURVE('',#20648,#20644,#4319,.T.);
#24522=EDGE_CURVE('',#20643,#20648,#4320,.T.);
#24523=EDGE_CURVE('',#20645,#20647,#4321,.T.);
#24524=EDGE_CURVE('',#20649,#20650,#4322,.T.);
#24525=EDGE_CURVE('',#20649,#20651,#2913,.T.);
#24526=EDGE_CURVE('',#20651,#20652,#4323,.T.);
#24527=EDGE_CURVE('',#20652,#20650,#2914,.T.);
#24528=EDGE_CURVE('',#20651,#20653,#4324,.T.);
#24529=EDGE_CURVE('',#20652,#20653,#4325,.T.);
#24530=EDGE_CURVE('',#20649,#20654,#4326,.T.);
#24531=EDGE_CURVE('',#20654,#20650,#4327,.T.);
#24532=EDGE_CURVE('',#20653,#20654,#17714,.T.);
#24533=EDGE_CURVE('',#20655,#20655,#17715,.T.);
#24534=EDGE_CURVE('',#20655,#20656,#4328,.T.);
#24535=EDGE_CURVE('',#20656,#20656,#17716,.T.);
#24536=EDGE_CURVE('',#20657,#20657,#17717,.T.);
#24537=EDGE_CURVE('',#20657,#20658,#4329,.T.);
#24538=EDGE_CURVE('',#20658,#20658,#17718,.T.);
#24539=EDGE_CURVE('',#20659,#20659,#17719,.T.);
#24540=EDGE_CURVE('',#20659,#20660,#4330,.T.);
#24541=EDGE_CURVE('',#20660,#20660,#17720,.T.);
#24542=EDGE_CURVE('',#20661,#20661,#17721,.T.);
#24543=EDGE_CURVE('',#20661,#20662,#4331,.T.);
#24544=EDGE_CURVE('',#20662,#20662,#17722,.T.);
#24545=EDGE_CURVE('',#20663,#20663,#17723,.T.);
#24546=EDGE_CURVE('',#20663,#20664,#4332,.T.);
#24547=EDGE_CURVE('',#20664,#20664,#17724,.T.);
#24548=EDGE_CURVE('',#20665,#20665,#17725,.T.);
#24549=EDGE_CURVE('',#20665,#20666,#4333,.T.);
#24550=EDGE_CURVE('',#20666,#20666,#17726,.T.);
#24551=EDGE_CURVE('',#20667,#20667,#17727,.T.);
#24552=EDGE_CURVE('',#20667,#20668,#4334,.T.);
#24553=EDGE_CURVE('',#20668,#20668,#17728,.T.);
#24554=EDGE_CURVE('',#20669,#20669,#17729,.T.);
#24555=EDGE_CURVE('',#20669,#20670,#4335,.T.);
#24556=EDGE_CURVE('',#20670,#20670,#17730,.T.);
#24557=EDGE_CURVE('',#20671,#20671,#17731,.T.);
#24558=EDGE_CURVE('',#20671,#20672,#4336,.T.);
#24559=EDGE_CURVE('',#20672,#20672,#17732,.T.);
#24560=EDGE_CURVE('',#20673,#20673,#17733,.T.);
#24561=EDGE_CURVE('',#20673,#20674,#4337,.T.);
#24562=EDGE_CURVE('',#20674,#20674,#17734,.T.);
#24563=EDGE_CURVE('',#20675,#20675,#17735,.T.);
#24564=EDGE_CURVE('',#20675,#20676,#4338,.T.);
#24565=EDGE_CURVE('',#20676,#20676,#17736,.T.);
#24566=EDGE_CURVE('',#20677,#20677,#17737,.T.);
#24567=EDGE_CURVE('',#20677,#20678,#4339,.T.);
#24568=EDGE_CURVE('',#20678,#20678,#17738,.T.);
#24569=EDGE_CURVE('',#20679,#20680,#1808,.T.);
#24570=EDGE_CURVE('',#20680,#20681,#4340,.T.);
#24571=EDGE_CURVE('',#20681,#20681,#1809,.T.);
#24572=EDGE_CURVE('',#20680,#20679,#1810,.T.);
#24573=EDGE_CURVE('',#20682,#20682,#17739,.T.);
#24574=EDGE_CURVE('',#20682,#20683,#4341,.T.);
#24575=EDGE_CURVE('',#20683,#20683,#1811,.T.);
#24576=EDGE_CURVE('',#20684,#20685,#1812,.T.);
#24577=EDGE_CURVE('',#20685,#20686,#4342,.T.);
#24578=EDGE_CURVE('',#20686,#20686,#1813,.T.);
#24579=EDGE_CURVE('',#20685,#20684,#1814,.T.);
#24580=EDGE_CURVE('',#20687,#20687,#17740,.T.);
#24581=EDGE_CURVE('',#20687,#20688,#4343,.T.);
#24582=EDGE_CURVE('',#20688,#20688,#1815,.T.);
#24583=EDGE_CURVE('',#20689,#20690,#1816,.T.);
#24584=EDGE_CURVE('',#20690,#20691,#4344,.T.);
#24585=EDGE_CURVE('',#20691,#20691,#1817,.T.);
#24586=EDGE_CURVE('',#20690,#20689,#1818,.T.);
#24587=EDGE_CURVE('',#20692,#20692,#17741,.T.);
#24588=EDGE_CURVE('',#20692,#20693,#4345,.T.);
#24589=EDGE_CURVE('',#20693,#20693,#1819,.T.);
#24590=EDGE_CURVE('',#20694,#20695,#1820,.T.);
#24591=EDGE_CURVE('',#20695,#20696,#4346,.T.);
#24592=EDGE_CURVE('',#20696,#20696,#1821,.T.);
#24593=EDGE_CURVE('',#20695,#20694,#1822,.T.);
#24594=EDGE_CURVE('',#20697,#20697,#17742,.T.);
#24595=EDGE_CURVE('',#20697,#20698,#4347,.T.);
#24596=EDGE_CURVE('',#20698,#20698,#1823,.T.);
#24597=EDGE_CURVE('',#20699,#20700,#1824,.T.);
#24598=EDGE_CURVE('',#20700,#20701,#4348,.T.);
#24599=EDGE_CURVE('',#20701,#20701,#1825,.T.);
#24600=EDGE_CURVE('',#20700,#20699,#1826,.T.);
#24601=EDGE_CURVE('',#20702,#20702,#17743,.T.);
#24602=EDGE_CURVE('',#20702,#20703,#4349,.T.);
#24603=EDGE_CURVE('',#20703,#20703,#1827,.T.);
#24604=EDGE_CURVE('',#20704,#20705,#1828,.T.);
#24605=EDGE_CURVE('',#20705,#20706,#4350,.T.);
#24606=EDGE_CURVE('',#20706,#20706,#1829,.T.);
#24607=EDGE_CURVE('',#20705,#20704,#1830,.T.);
#24608=EDGE_CURVE('',#20707,#20707,#17744,.T.);
#24609=EDGE_CURVE('',#20707,#20708,#4351,.T.);
#24610=EDGE_CURVE('',#20708,#20708,#1831,.T.);
#24611=EDGE_CURVE('',#20709,#20710,#1832,.T.);
#24612=EDGE_CURVE('',#20710,#20711,#4352,.T.);
#24613=EDGE_CURVE('',#20711,#20711,#1833,.T.);
#24614=EDGE_CURVE('',#20710,#20709,#1834,.T.);
#24615=EDGE_CURVE('',#20712,#20712,#17745,.T.);
#24616=EDGE_CURVE('',#20712,#20713,#4353,.T.);
#24617=EDGE_CURVE('',#20713,#20713,#1835,.T.);
#24618=EDGE_CURVE('',#20714,#20715,#1836,.T.);
#24619=EDGE_CURVE('',#20715,#20716,#4354,.T.);
#24620=EDGE_CURVE('',#20716,#20716,#1837,.T.);
#24621=EDGE_CURVE('',#20715,#20714,#1838,.T.);
#24622=EDGE_CURVE('',#20717,#20717,#17746,.T.);
#24623=EDGE_CURVE('',#20717,#20718,#4355,.T.);
#24624=EDGE_CURVE('',#20718,#20718,#1839,.T.);
#24625=EDGE_CURVE('',#20719,#20720,#1840,.T.);
#24626=EDGE_CURVE('',#20720,#20721,#4356,.T.);
#24627=EDGE_CURVE('',#20721,#20721,#1841,.T.);
#24628=EDGE_CURVE('',#20720,#20719,#1842,.T.);
#24629=EDGE_CURVE('',#20722,#20722,#17747,.T.);
#24630=EDGE_CURVE('',#20722,#20723,#4357,.T.);
#24631=EDGE_CURVE('',#20723,#20723,#1843,.T.);
#24632=EDGE_CURVE('',#20724,#20725,#1844,.T.);
#24633=EDGE_CURVE('',#20725,#20726,#4358,.T.);
#24634=EDGE_CURVE('',#20726,#20726,#1845,.T.);
#24635=EDGE_CURVE('',#20725,#20724,#1846,.T.);
#24636=EDGE_CURVE('',#20727,#20727,#17748,.T.);
#24637=EDGE_CURVE('',#20727,#20728,#4359,.T.);
#24638=EDGE_CURVE('',#20728,#20728,#1847,.T.);
#24639=EDGE_CURVE('',#20729,#20730,#1848,.T.);
#24640=EDGE_CURVE('',#20730,#20731,#4360,.T.);
#24641=EDGE_CURVE('',#20731,#20731,#1849,.T.);
#24642=EDGE_CURVE('',#20730,#20729,#1850,.T.);
#24643=EDGE_CURVE('',#20732,#20732,#17749,.T.);
#24644=EDGE_CURVE('',#20732,#20733,#4361,.T.);
#24645=EDGE_CURVE('',#20733,#20733,#1851,.T.);
#24646=EDGE_CURVE('',#20734,#20735,#1852,.T.);
#24647=EDGE_CURVE('',#20735,#20736,#4362,.T.);
#24648=EDGE_CURVE('',#20736,#20736,#1853,.T.);
#24649=EDGE_CURVE('',#20735,#20734,#1854,.T.);
#24650=EDGE_CURVE('',#20737,#20737,#17750,.T.);
#24651=EDGE_CURVE('',#20737,#20738,#4363,.T.);
#24652=EDGE_CURVE('',#20738,#20738,#1855,.T.);
#24653=EDGE_CURVE('',#20739,#20740,#1856,.T.);
#24654=EDGE_CURVE('',#20740,#20741,#4364,.T.);
#24655=EDGE_CURVE('',#20741,#20741,#1857,.T.);
#24656=EDGE_CURVE('',#20740,#20739,#1858,.T.);
#24657=EDGE_CURVE('',#20742,#20742,#17751,.T.);
#24658=EDGE_CURVE('',#20742,#20743,#4365,.T.);
#24659=EDGE_CURVE('',#20743,#20743,#1859,.T.);
#24660=EDGE_CURVE('',#20744,#20745,#1860,.T.);
#24661=EDGE_CURVE('',#20745,#20746,#4366,.T.);
#24662=EDGE_CURVE('',#20746,#20746,#1861,.T.);
#24663=EDGE_CURVE('',#20745,#20744,#1862,.T.);
#24664=EDGE_CURVE('',#20747,#20747,#17752,.T.);
#24665=EDGE_CURVE('',#20747,#20748,#4367,.T.);
#24666=EDGE_CURVE('',#20748,#20748,#1863,.T.);
#24667=EDGE_CURVE('',#20749,#20750,#1864,.T.);
#24668=EDGE_CURVE('',#20750,#20751,#4368,.T.);
#24669=EDGE_CURVE('',#20751,#20751,#1865,.T.);
#24670=EDGE_CURVE('',#20750,#20749,#1866,.T.);
#24671=EDGE_CURVE('',#20752,#20752,#17753,.T.);
#24672=EDGE_CURVE('',#20752,#20753,#4369,.T.);
#24673=EDGE_CURVE('',#20753,#20753,#1867,.T.);
#24674=EDGE_CURVE('',#20754,#20755,#1868,.T.);
#24675=EDGE_CURVE('',#20755,#20756,#4370,.T.);
#24676=EDGE_CURVE('',#20756,#20756,#1869,.T.);
#24677=EDGE_CURVE('',#20755,#20754,#1870,.T.);
#24678=EDGE_CURVE('',#20757,#20757,#17754,.T.);
#24679=EDGE_CURVE('',#20757,#20758,#4371,.T.);
#24680=EDGE_CURVE('',#20758,#20758,#1871,.T.);
#24681=EDGE_CURVE('',#20759,#20760,#1872,.T.);
#24682=EDGE_CURVE('',#20760,#20761,#4372,.T.);
#24683=EDGE_CURVE('',#20761,#20761,#1873,.T.);
#24684=EDGE_CURVE('',#20760,#20759,#1874,.T.);
#24685=EDGE_CURVE('',#20762,#20762,#17755,.T.);
#24686=EDGE_CURVE('',#20762,#20763,#4373,.T.);
#24687=EDGE_CURVE('',#20763,#20763,#1875,.T.);
#24688=EDGE_CURVE('',#20764,#20765,#1876,.T.);
#24689=EDGE_CURVE('',#20765,#20766,#4374,.T.);
#24690=EDGE_CURVE('',#20766,#20766,#1877,.T.);
#24691=EDGE_CURVE('',#20765,#20764,#1878,.T.);
#24692=EDGE_CURVE('',#20767,#20767,#17756,.T.);
#24693=EDGE_CURVE('',#20767,#20768,#4375,.T.);
#24694=EDGE_CURVE('',#20768,#20768,#1879,.T.);
#24695=EDGE_CURVE('',#20769,#20770,#1880,.T.);
#24696=EDGE_CURVE('',#20770,#20771,#4376,.T.);
#24697=EDGE_CURVE('',#20771,#20771,#1881,.T.);
#24698=EDGE_CURVE('',#20770,#20769,#1882,.T.);
#24699=EDGE_CURVE('',#20772,#20772,#17757,.T.);
#24700=EDGE_CURVE('',#20772,#20773,#4377,.T.);
#24701=EDGE_CURVE('',#20773,#20773,#1883,.T.);
#24702=EDGE_CURVE('',#20774,#20775,#1884,.T.);
#24703=EDGE_CURVE('',#20775,#20776,#4378,.T.);
#24704=EDGE_CURVE('',#20776,#20776,#1885,.T.);
#24705=EDGE_CURVE('',#20775,#20774,#1886,.T.);
#24706=EDGE_CURVE('',#20777,#20777,#17758,.T.);
#24707=EDGE_CURVE('',#20777,#20778,#4379,.T.);
#24708=EDGE_CURVE('',#20778,#20778,#1887,.T.);
#24709=EDGE_CURVE('',#20779,#20780,#1888,.T.);
#24710=EDGE_CURVE('',#20780,#20781,#4380,.T.);
#24711=EDGE_CURVE('',#20781,#20781,#1889,.T.);
#24712=EDGE_CURVE('',#20780,#20779,#1890,.T.);
#24713=EDGE_CURVE('',#20782,#20782,#17759,.T.);
#24714=EDGE_CURVE('',#20782,#20783,#4381,.T.);
#24715=EDGE_CURVE('',#20783,#20783,#1891,.T.);
#24716=EDGE_CURVE('',#20784,#20785,#1892,.T.);
#24717=EDGE_CURVE('',#20785,#20786,#4382,.T.);
#24718=EDGE_CURVE('',#20786,#20786,#1893,.T.);
#24719=EDGE_CURVE('',#20785,#20784,#1894,.T.);
#24720=EDGE_CURVE('',#20787,#20787,#17760,.T.);
#24721=EDGE_CURVE('',#20787,#20788,#4383,.T.);
#24722=EDGE_CURVE('',#20788,#20788,#1895,.T.);
#24723=EDGE_CURVE('',#20789,#20790,#1896,.T.);
#24724=EDGE_CURVE('',#20790,#20791,#4384,.T.);
#24725=EDGE_CURVE('',#20791,#20791,#1897,.T.);
#24726=EDGE_CURVE('',#20790,#20789,#1898,.T.);
#24727=EDGE_CURVE('',#20792,#20792,#17761,.T.);
#24728=EDGE_CURVE('',#20792,#20793,#4385,.T.);
#24729=EDGE_CURVE('',#20793,#20793,#1899,.T.);
#24730=EDGE_CURVE('',#20794,#20795,#1900,.T.);
#24731=EDGE_CURVE('',#20795,#20796,#4386,.T.);
#24732=EDGE_CURVE('',#20796,#20796,#1901,.T.);
#24733=EDGE_CURVE('',#20795,#20794,#1902,.T.);
#24734=EDGE_CURVE('',#20797,#20797,#17762,.T.);
#24735=EDGE_CURVE('',#20797,#20798,#4387,.T.);
#24736=EDGE_CURVE('',#20798,#20798,#1903,.T.);
#24737=EDGE_CURVE('',#20799,#20800,#1904,.T.);
#24738=EDGE_CURVE('',#20800,#20801,#4388,.T.);
#24739=EDGE_CURVE('',#20801,#20801,#1905,.T.);
#24740=EDGE_CURVE('',#20800,#20799,#1906,.T.);
#24741=EDGE_CURVE('',#20802,#20802,#17763,.T.);
#24742=EDGE_CURVE('',#20802,#20803,#4389,.T.);
#24743=EDGE_CURVE('',#20803,#20803,#1907,.T.);
#24744=EDGE_CURVE('',#20804,#20805,#1908,.T.);
#24745=EDGE_CURVE('',#20805,#20806,#4390,.T.);
#24746=EDGE_CURVE('',#20806,#20806,#1909,.T.);
#24747=EDGE_CURVE('',#20805,#20804,#1910,.T.);
#24748=EDGE_CURVE('',#20807,#20807,#17764,.T.);
#24749=EDGE_CURVE('',#20807,#20808,#4391,.T.);
#24750=EDGE_CURVE('',#20808,#20808,#1911,.T.);
#24751=EDGE_CURVE('',#20809,#20810,#1912,.T.);
#24752=EDGE_CURVE('',#20810,#20811,#4392,.T.);
#24753=EDGE_CURVE('',#20811,#20811,#1913,.T.);
#24754=EDGE_CURVE('',#20810,#20809,#1914,.T.);
#24755=EDGE_CURVE('',#20812,#20812,#17765,.T.);
#24756=EDGE_CURVE('',#20812,#20813,#4393,.T.);
#24757=EDGE_CURVE('',#20813,#20813,#1915,.T.);
#24758=EDGE_CURVE('',#20814,#20815,#1916,.T.);
#24759=EDGE_CURVE('',#20815,#20816,#4394,.T.);
#24760=EDGE_CURVE('',#20816,#20816,#1917,.T.);
#24761=EDGE_CURVE('',#20815,#20814,#1918,.T.);
#24762=EDGE_CURVE('',#20817,#20817,#17766,.T.);
#24763=EDGE_CURVE('',#20817,#20818,#4395,.T.);
#24764=EDGE_CURVE('',#20818,#20818,#1919,.T.);
#24765=EDGE_CURVE('',#20819,#20820,#1920,.T.);
#24766=EDGE_CURVE('',#20820,#20821,#4396,.T.);
#24767=EDGE_CURVE('',#20821,#20821,#1921,.T.);
#24768=EDGE_CURVE('',#20820,#20819,#1922,.T.);
#24769=EDGE_CURVE('',#20822,#20822,#17767,.T.);
#24770=EDGE_CURVE('',#20822,#20823,#4397,.T.);
#24771=EDGE_CURVE('',#20823,#20823,#1923,.T.);
#24772=EDGE_CURVE('',#20824,#20825,#1924,.T.);
#24773=EDGE_CURVE('',#20825,#20826,#4398,.T.);
#24774=EDGE_CURVE('',#20826,#20826,#1925,.T.);
#24775=EDGE_CURVE('',#20825,#20824,#1926,.T.);
#24776=EDGE_CURVE('',#20827,#20827,#17768,.T.);
#24777=EDGE_CURVE('',#20827,#20828,#4399,.T.);
#24778=EDGE_CURVE('',#20828,#20828,#1927,.T.);
#24779=EDGE_CURVE('',#20829,#20830,#1928,.T.);
#24780=EDGE_CURVE('',#20830,#20831,#4400,.T.);
#24781=EDGE_CURVE('',#20831,#20831,#1929,.T.);
#24782=EDGE_CURVE('',#20830,#20829,#1930,.T.);
#24783=EDGE_CURVE('',#20832,#20832,#17769,.T.);
#24784=EDGE_CURVE('',#20832,#20833,#4401,.T.);
#24785=EDGE_CURVE('',#20833,#20833,#1931,.T.);
#24786=EDGE_CURVE('',#20834,#20835,#1932,.T.);
#24787=EDGE_CURVE('',#20835,#20836,#4402,.T.);
#24788=EDGE_CURVE('',#20836,#20836,#1933,.T.);
#24789=EDGE_CURVE('',#20835,#20834,#1934,.T.);
#24790=EDGE_CURVE('',#20837,#20837,#17770,.T.);
#24791=EDGE_CURVE('',#20837,#20838,#4403,.T.);
#24792=EDGE_CURVE('',#20838,#20838,#1935,.T.);
#24793=EDGE_CURVE('',#20839,#20840,#1936,.T.);
#24794=EDGE_CURVE('',#20840,#20841,#4404,.T.);
#24795=EDGE_CURVE('',#20841,#20841,#1937,.T.);
#24796=EDGE_CURVE('',#20840,#20839,#1938,.T.);
#24797=EDGE_CURVE('',#20842,#20842,#17771,.T.);
#24798=EDGE_CURVE('',#20842,#20843,#4405,.T.);
#24799=EDGE_CURVE('',#20843,#20843,#1939,.T.);
#24800=EDGE_CURVE('',#20844,#20845,#1940,.T.);
#24801=EDGE_CURVE('',#20845,#20846,#4406,.T.);
#24802=EDGE_CURVE('',#20846,#20846,#1941,.T.);
#24803=EDGE_CURVE('',#20845,#20844,#1942,.T.);
#24804=EDGE_CURVE('',#20847,#20847,#17772,.T.);
#24805=EDGE_CURVE('',#20847,#20848,#4407,.T.);
#24806=EDGE_CURVE('',#20848,#20848,#1943,.T.);
#24807=EDGE_CURVE('',#20849,#20850,#1944,.T.);
#24808=EDGE_CURVE('',#20850,#20851,#4408,.T.);
#24809=EDGE_CURVE('',#20851,#20851,#1945,.T.);
#24810=EDGE_CURVE('',#20850,#20849,#1946,.T.);
#24811=EDGE_CURVE('',#20852,#20852,#17773,.T.);
#24812=EDGE_CURVE('',#20852,#20853,#4409,.T.);
#24813=EDGE_CURVE('',#20853,#20853,#1947,.T.);
#24814=EDGE_CURVE('',#20854,#20855,#1948,.T.);
#24815=EDGE_CURVE('',#20855,#20856,#4410,.T.);
#24816=EDGE_CURVE('',#20856,#20856,#1949,.T.);
#24817=EDGE_CURVE('',#20855,#20854,#1950,.T.);
#24818=EDGE_CURVE('',#20857,#20857,#17774,.T.);
#24819=EDGE_CURVE('',#20857,#20858,#4411,.T.);
#24820=EDGE_CURVE('',#20858,#20858,#1951,.T.);
#24821=EDGE_CURVE('',#20859,#20860,#1952,.T.);
#24822=EDGE_CURVE('',#20860,#20861,#4412,.T.);
#24823=EDGE_CURVE('',#20861,#20861,#1953,.T.);
#24824=EDGE_CURVE('',#20860,#20859,#1954,.T.);
#24825=EDGE_CURVE('',#20862,#20862,#17775,.T.);
#24826=EDGE_CURVE('',#20862,#20863,#4413,.T.);
#24827=EDGE_CURVE('',#20863,#20863,#1955,.T.);
#24828=EDGE_CURVE('',#20864,#20865,#1956,.T.);
#24829=EDGE_CURVE('',#20865,#20866,#4414,.T.);
#24830=EDGE_CURVE('',#20866,#20866,#1957,.T.);
#24831=EDGE_CURVE('',#20865,#20864,#1958,.T.);
#24832=EDGE_CURVE('',#20867,#20867,#17776,.T.);
#24833=EDGE_CURVE('',#20867,#20868,#4415,.T.);
#24834=EDGE_CURVE('',#20868,#20868,#1959,.T.);
#24835=EDGE_CURVE('',#20869,#20870,#1960,.T.);
#24836=EDGE_CURVE('',#20870,#20871,#4416,.T.);
#24837=EDGE_CURVE('',#20871,#20871,#1961,.T.);
#24838=EDGE_CURVE('',#20870,#20869,#1962,.T.);
#24839=EDGE_CURVE('',#20872,#20872,#17777,.T.);
#24840=EDGE_CURVE('',#20872,#20873,#4417,.T.);
#24841=EDGE_CURVE('',#20873,#20873,#1963,.T.);
#24842=EDGE_CURVE('',#20874,#20874,#17778,.T.);
#24843=EDGE_CURVE('',#20874,#20875,#4418,.T.);
#24844=EDGE_CURVE('',#20875,#20875,#1964,.T.);
#24845=EDGE_CURVE('',#20876,#20876,#17779,.T.);
#24846=EDGE_CURVE('',#20876,#20877,#4419,.T.);
#24847=EDGE_CURVE('',#20877,#20877,#17780,.T.);
#24848=EDGE_CURVE('',#20878,#20878,#17781,.T.);
#24849=EDGE_CURVE('',#20878,#20879,#4420,.T.);
#24850=EDGE_CURVE('',#20879,#20879,#1965,.T.);
#24851=EDGE_CURVE('',#20880,#20880,#17782,.T.);
#24852=EDGE_CURVE('',#20880,#20881,#4421,.T.);
#24853=EDGE_CURVE('',#20881,#20881,#17783,.T.);
#24854=EDGE_CURVE('',#20882,#20883,#1966,.T.);
#24855=EDGE_CURVE('',#20883,#20884,#4422,.T.);
#24856=EDGE_CURVE('',#20884,#20884,#1967,.T.);
#24857=EDGE_CURVE('',#20883,#20882,#1968,.T.);
#24858=EDGE_CURVE('',#20885,#20885,#17784,.T.);
#24859=EDGE_CURVE('',#20885,#20886,#4423,.T.);
#24860=EDGE_CURVE('',#20886,#20886,#1969,.T.);
#24861=EDGE_CURVE('',#20887,#20888,#1970,.T.);
#24862=EDGE_CURVE('',#20888,#20889,#4424,.T.);
#24863=EDGE_CURVE('',#20889,#20889,#1971,.T.);
#24864=EDGE_CURVE('',#20888,#20887,#1972,.T.);
#24865=EDGE_CURVE('',#20890,#20890,#17785,.T.);
#24866=EDGE_CURVE('',#20890,#20891,#4425,.T.);
#24867=EDGE_CURVE('',#20891,#20891,#1973,.T.);
#24868=EDGE_CURVE('',#20892,#20892,#17786,.T.);
#24869=EDGE_CURVE('',#20892,#20893,#4426,.T.);
#24870=EDGE_CURVE('',#20893,#20893,#1974,.T.);
#24871=EDGE_CURVE('',#20894,#20894,#17787,.T.);
#24872=EDGE_CURVE('',#20894,#20895,#4427,.T.);
#24873=EDGE_CURVE('',#20895,#20895,#17788,.T.);
#24874=EDGE_CURVE('',#20896,#20896,#17789,.T.);
#24875=EDGE_CURVE('',#20896,#20897,#4428,.T.);
#24876=EDGE_CURVE('',#20897,#20897,#1975,.T.);
#24877=EDGE_CURVE('',#20898,#20898,#17790,.T.);
#24878=EDGE_CURVE('',#20898,#20899,#4429,.T.);
#24879=EDGE_CURVE('',#20899,#20899,#17791,.T.);
#24880=EDGE_CURVE('',#20900,#20901,#1976,.T.);
#24881=EDGE_CURVE('',#20901,#20902,#4430,.T.);
#24882=EDGE_CURVE('',#20902,#20902,#1977,.T.);
#24883=EDGE_CURVE('',#20901,#20900,#1978,.T.);
#24884=EDGE_CURVE('',#20903,#20903,#17792,.T.);
#24885=EDGE_CURVE('',#20903,#20904,#4431,.T.);
#24886=EDGE_CURVE('',#20904,#20904,#1979,.T.);
#24887=EDGE_CURVE('',#20905,#20906,#1980,.T.);
#24888=EDGE_CURVE('',#20906,#20907,#4432,.T.);
#24889=EDGE_CURVE('',#20907,#20907,#1981,.T.);
#24890=EDGE_CURVE('',#20906,#20905,#1982,.T.);
#24891=EDGE_CURVE('',#20908,#20908,#17793,.T.);
#24892=EDGE_CURVE('',#20908,#20909,#4433,.T.);
#24893=EDGE_CURVE('',#20909,#20909,#1983,.T.);
#24894=EDGE_CURVE('',#20910,#20910,#17794,.T.);
#24895=EDGE_CURVE('',#20910,#20911,#4434,.T.);
#24896=EDGE_CURVE('',#20911,#20911,#1984,.T.);
#24897=EDGE_CURVE('',#20912,#20912,#17795,.T.);
#24898=EDGE_CURVE('',#20912,#20913,#4435,.T.);
#24899=EDGE_CURVE('',#20913,#20913,#17796,.T.);
#24900=EDGE_CURVE('',#20914,#20915,#1985,.T.);
#24901=EDGE_CURVE('',#20915,#20916,#4436,.T.);
#24902=EDGE_CURVE('',#20916,#20916,#1986,.T.);
#24903=EDGE_CURVE('',#20915,#20914,#1987,.T.);
#24904=EDGE_CURVE('',#20917,#20917,#17797,.T.);
#24905=EDGE_CURVE('',#20917,#20918,#4437,.T.);
#24906=EDGE_CURVE('',#20918,#20918,#1988,.T.);
#24907=EDGE_CURVE('',#20919,#20920,#1989,.T.);
#24908=EDGE_CURVE('',#20920,#20921,#4438,.T.);
#24909=EDGE_CURVE('',#20921,#20921,#1990,.T.);
#24910=EDGE_CURVE('',#20920,#20919,#1991,.T.);
#24911=EDGE_CURVE('',#20922,#20922,#17798,.T.);
#24912=EDGE_CURVE('',#20922,#20923,#4439,.T.);
#24913=EDGE_CURVE('',#20923,#20923,#1992,.T.);
#24914=EDGE_CURVE('',#20924,#20924,#17799,.T.);
#24915=EDGE_CURVE('',#20924,#20925,#4440,.T.);
#24916=EDGE_CURVE('',#20925,#20925,#1993,.T.);
#24917=EDGE_CURVE('',#20926,#20926,#17800,.T.);
#24918=EDGE_CURVE('',#20926,#20927,#4441,.T.);
#24919=EDGE_CURVE('',#20927,#20927,#17801,.T.);
#24920=EDGE_CURVE('',#20928,#20929,#1994,.T.);
#24921=EDGE_CURVE('',#20929,#20930,#4442,.T.);
#24922=EDGE_CURVE('',#20930,#20930,#1995,.T.);
#24923=EDGE_CURVE('',#20929,#20928,#1996,.T.);
#24924=EDGE_CURVE('',#20931,#20931,#17802,.T.);
#24925=EDGE_CURVE('',#20931,#20932,#4443,.T.);
#24926=EDGE_CURVE('',#20932,#20932,#1997,.T.);
#24927=EDGE_CURVE('',#20933,#20934,#1998,.T.);
#24928=EDGE_CURVE('',#20934,#20935,#4444,.T.);
#24929=EDGE_CURVE('',#20935,#20935,#1999,.T.);
#24930=EDGE_CURVE('',#20934,#20933,#2000,.T.);
#24931=EDGE_CURVE('',#20936,#20936,#17803,.T.);
#24932=EDGE_CURVE('',#20936,#20937,#4445,.T.);
#24933=EDGE_CURVE('',#20937,#20937,#2001,.T.);
#24934=EDGE_CURVE('',#20938,#20939,#2002,.T.);
#24935=EDGE_CURVE('',#20939,#20940,#4446,.T.);
#24936=EDGE_CURVE('',#20940,#20940,#2003,.T.);
#24937=EDGE_CURVE('',#20939,#20938,#2004,.T.);
#24938=EDGE_CURVE('',#20941,#20941,#17804,.T.);
#24939=EDGE_CURVE('',#20941,#20942,#4447,.T.);
#24940=EDGE_CURVE('',#20942,#20942,#2005,.T.);
#24941=EDGE_CURVE('',#20943,#20944,#2006,.T.);
#24942=EDGE_CURVE('',#20944,#20945,#4448,.T.);
#24943=EDGE_CURVE('',#20945,#20945,#2007,.T.);
#24944=EDGE_CURVE('',#20944,#20943,#2008,.T.);
#24945=EDGE_CURVE('',#20946,#20946,#17805,.T.);
#24946=EDGE_CURVE('',#20946,#20947,#4449,.T.);
#24947=EDGE_CURVE('',#20947,#20947,#2009,.T.);
#24948=EDGE_CURVE('',#20948,#20949,#2010,.T.);
#24949=EDGE_CURVE('',#20949,#20950,#4450,.T.);
#24950=EDGE_CURVE('',#20950,#20950,#2011,.T.);
#24951=EDGE_CURVE('',#20949,#20948,#2012,.T.);
#24952=EDGE_CURVE('',#20951,#20951,#17806,.T.);
#24953=EDGE_CURVE('',#20951,#20952,#4451,.T.);
#24954=EDGE_CURVE('',#20952,#20952,#2013,.T.);
#24955=EDGE_CURVE('',#20953,#20954,#2014,.T.);
#24956=EDGE_CURVE('',#20954,#20955,#4452,.T.);
#24957=EDGE_CURVE('',#20955,#20955,#2015,.T.);
#24958=EDGE_CURVE('',#20954,#20953,#2016,.T.);
#24959=EDGE_CURVE('',#20956,#20956,#17807,.T.);
#24960=EDGE_CURVE('',#20956,#20957,#4453,.T.);
#24961=EDGE_CURVE('',#20957,#20957,#2017,.T.);
#24962=EDGE_CURVE('',#20958,#20959,#2018,.T.);
#24963=EDGE_CURVE('',#20959,#20960,#4454,.T.);
#24964=EDGE_CURVE('',#20960,#20960,#2019,.T.);
#24965=EDGE_CURVE('',#20959,#20958,#2020,.T.);
#24966=EDGE_CURVE('',#20961,#20961,#17808,.T.);
#24967=EDGE_CURVE('',#20961,#20962,#4455,.T.);
#24968=EDGE_CURVE('',#20962,#20962,#2021,.T.);
#24969=EDGE_CURVE('',#20963,#20964,#2022,.T.);
#24970=EDGE_CURVE('',#20964,#20965,#4456,.T.);
#24971=EDGE_CURVE('',#20965,#20965,#2023,.T.);
#24972=EDGE_CURVE('',#20964,#20963,#2024,.T.);
#24973=EDGE_CURVE('',#20966,#20966,#17809,.T.);
#24974=EDGE_CURVE('',#20966,#20967,#4457,.T.);
#24975=EDGE_CURVE('',#20967,#20967,#2025,.T.);
#24976=EDGE_CURVE('',#20968,#20969,#2026,.T.);
#24977=EDGE_CURVE('',#20969,#20970,#4458,.T.);
#24978=EDGE_CURVE('',#20970,#20970,#2027,.T.);
#24979=EDGE_CURVE('',#20969,#20968,#2028,.T.);
#24980=EDGE_CURVE('',#20971,#20971,#17810,.T.);
#24981=EDGE_CURVE('',#20971,#20972,#4459,.T.);
#24982=EDGE_CURVE('',#20972,#20972,#2029,.T.);
#24983=EDGE_CURVE('',#20973,#20974,#2030,.T.);
#24984=EDGE_CURVE('',#20974,#20975,#4460,.T.);
#24985=EDGE_CURVE('',#20975,#20975,#2031,.T.);
#24986=EDGE_CURVE('',#20974,#20973,#2032,.T.);
#24987=EDGE_CURVE('',#20976,#20976,#17811,.T.);
#24988=EDGE_CURVE('',#20976,#20977,#4461,.T.);
#24989=EDGE_CURVE('',#20977,#20977,#2033,.T.);
#24990=EDGE_CURVE('',#20978,#20979,#2034,.T.);
#24991=EDGE_CURVE('',#20979,#20980,#4462,.T.);
#24992=EDGE_CURVE('',#20980,#20980,#2035,.T.);
#24993=EDGE_CURVE('',#20979,#20978,#2036,.T.);
#24994=EDGE_CURVE('',#20981,#20981,#17812,.T.);
#24995=EDGE_CURVE('',#20981,#20982,#4463,.T.);
#24996=EDGE_CURVE('',#20982,#20982,#2037,.T.);
#24997=EDGE_CURVE('',#20983,#20984,#2038,.T.);
#24998=EDGE_CURVE('',#20984,#20985,#4464,.T.);
#24999=EDGE_CURVE('',#20985,#20985,#2039,.T.);
#25000=EDGE_CURVE('',#20984,#20983,#2040,.T.);
#25001=EDGE_CURVE('',#20986,#20986,#17813,.T.);
#25002=EDGE_CURVE('',#20986,#20987,#4465,.T.);
#25003=EDGE_CURVE('',#20987,#20987,#2041,.T.);
#25004=EDGE_CURVE('',#20988,#20989,#2042,.T.);
#25005=EDGE_CURVE('',#20989,#20990,#4466,.T.);
#25006=EDGE_CURVE('',#20990,#20990,#2043,.T.);
#25007=EDGE_CURVE('',#20989,#20988,#2044,.T.);
#25008=EDGE_CURVE('',#20991,#20991,#17814,.T.);
#25009=EDGE_CURVE('',#20991,#20992,#4467,.T.);
#25010=EDGE_CURVE('',#20992,#20992,#2045,.T.);
#25011=EDGE_CURVE('',#20993,#20994,#2046,.T.);
#25012=EDGE_CURVE('',#20994,#20995,#4468,.T.);
#25013=EDGE_CURVE('',#20995,#20995,#2047,.T.);
#25014=EDGE_CURVE('',#20994,#20993,#2048,.T.);
#25015=EDGE_CURVE('',#20996,#20996,#17815,.T.);
#25016=EDGE_CURVE('',#20996,#20997,#4469,.T.);
#25017=EDGE_CURVE('',#20997,#20997,#2049,.T.);
#25018=EDGE_CURVE('',#20998,#20998,#17816,.T.);
#25019=EDGE_CURVE('',#20998,#20999,#4470,.T.);
#25020=EDGE_CURVE('',#20999,#20999,#17817,.T.);
#25021=EDGE_CURVE('',#21000,#21000,#17818,.T.);
#25022=EDGE_CURVE('',#21000,#21001,#4471,.T.);
#25023=EDGE_CURVE('',#21001,#21001,#17819,.T.);
#25024=EDGE_CURVE('',#21002,#21002,#17820,.T.);
#25025=EDGE_CURVE('',#21002,#21003,#4472,.T.);
#25026=EDGE_CURVE('',#21003,#21003,#17821,.T.);
#25027=EDGE_CURVE('',#21004,#21004,#17822,.T.);
#25028=EDGE_CURVE('',#21004,#21005,#4473,.T.);
#25029=EDGE_CURVE('',#21005,#21005,#17823,.T.);
#25030=EDGE_CURVE('',#21006,#21006,#17824,.T.);
#25031=EDGE_CURVE('',#21006,#21007,#4474,.T.);
#25032=EDGE_CURVE('',#21007,#21007,#17825,.T.);
#25033=EDGE_CURVE('',#21008,#21008,#17826,.T.);
#25034=EDGE_CURVE('',#21008,#21009,#4475,.T.);
#25035=EDGE_CURVE('',#21009,#21009,#17827,.T.);
#25036=EDGE_CURVE('',#21010,#21010,#17828,.T.);
#25037=EDGE_CURVE('',#21010,#21011,#4476,.T.);
#25038=EDGE_CURVE('',#21011,#21011,#17829,.T.);
#25039=EDGE_CURVE('',#21012,#21012,#17830,.T.);
#25040=EDGE_CURVE('',#21012,#21013,#4477,.T.);
#25041=EDGE_CURVE('',#21013,#21013,#17831,.T.);
#25042=EDGE_CURVE('',#21014,#21014,#17832,.T.);
#25043=EDGE_CURVE('',#21014,#21015,#4478,.T.);
#25044=EDGE_CURVE('',#21015,#21015,#17833,.T.);
#25045=EDGE_CURVE('',#21016,#21016,#17834,.T.);
#25046=EDGE_CURVE('',#21016,#21017,#4479,.T.);
#25047=EDGE_CURVE('',#21017,#21017,#17835,.T.);
#25048=EDGE_CURVE('',#21018,#21018,#17836,.T.);
#25049=EDGE_CURVE('',#21018,#21019,#4480,.T.);
#25050=EDGE_CURVE('',#21019,#21019,#17837,.T.);
#25051=EDGE_CURVE('',#21020,#21020,#17838,.T.);
#25052=EDGE_CURVE('',#21020,#21021,#4481,.T.);
#25053=EDGE_CURVE('',#21021,#21021,#17839,.T.);
#25054=EDGE_CURVE('',#21022,#21022,#17840,.T.);
#25055=EDGE_CURVE('',#21022,#21023,#4482,.T.);
#25056=EDGE_CURVE('',#21023,#21023,#17841,.T.);
#25057=EDGE_CURVE('',#21024,#21024,#17842,.T.);
#25058=EDGE_CURVE('',#21024,#21025,#4483,.T.);
#25059=EDGE_CURVE('',#21025,#21025,#17843,.T.);
#25060=EDGE_CURVE('',#21026,#21026,#17844,.T.);
#25061=EDGE_CURVE('',#21026,#21027,#4484,.T.);
#25062=EDGE_CURVE('',#21027,#21027,#17845,.T.);
#25063=EDGE_CURVE('',#21028,#21028,#17846,.T.);
#25064=EDGE_CURVE('',#21028,#21029,#4485,.T.);
#25065=EDGE_CURVE('',#21029,#21029,#17847,.T.);
#25066=EDGE_CURVE('',#21030,#21030,#17848,.T.);
#25067=EDGE_CURVE('',#21030,#21031,#4486,.T.);
#25068=EDGE_CURVE('',#21032,#21031,#2050,.F.);
#25069=EDGE_CURVE('',#21032,#21033,#17849,.T.);
#25070=EDGE_CURVE('',#21031,#21033,#2051,.F.);
#25071=EDGE_CURVE('',#21034,#21034,#17850,.T.);
#25072=EDGE_CURVE('',#21034,#21035,#4487,.T.);
#25073=EDGE_CURVE('',#21035,#21035,#17851,.T.);
#25074=EDGE_CURVE('',#21036,#21036,#17852,.T.);
#25075=EDGE_CURVE('',#21036,#21037,#4488,.T.);
#25076=EDGE_CURVE('',#21037,#21037,#17853,.T.);
#25077=EDGE_CURVE('',#21038,#21038,#17854,.T.);
#25078=EDGE_CURVE('',#21038,#21039,#4489,.T.);
#25079=EDGE_CURVE('',#21039,#21039,#17855,.T.);
#25080=EDGE_CURVE('',#21040,#21040,#17856,.T.);
#25081=EDGE_CURVE('',#21040,#21041,#4490,.T.);
#25082=EDGE_CURVE('',#21041,#21041,#17857,.T.);
#25083=EDGE_CURVE('',#21042,#21042,#17858,.T.);
#25084=EDGE_CURVE('',#21042,#21043,#4491,.T.);
#25085=EDGE_CURVE('',#21043,#21043,#17859,.T.);
#25086=EDGE_CURVE('',#21044,#21044,#17860,.T.);
#25087=EDGE_CURVE('',#21044,#21045,#4492,.T.);
#25088=EDGE_CURVE('',#21045,#21045,#17861,.T.);
#25089=EDGE_CURVE('',#21046,#21046,#17862,.T.);
#25090=EDGE_CURVE('',#21046,#21047,#4493,.T.);
#25091=EDGE_CURVE('',#21047,#21047,#17863,.T.);
#25092=EDGE_CURVE('',#21048,#21048,#17864,.T.);
#25093=EDGE_CURVE('',#21048,#21049,#4494,.T.);
#25094=EDGE_CURVE('',#21049,#21049,#17865,.T.);
#25095=EDGE_CURVE('',#21050,#21050,#17866,.T.);
#25096=EDGE_CURVE('',#21050,#21051,#4495,.T.);
#25097=EDGE_CURVE('',#21051,#21051,#17867,.T.);
#25098=EDGE_CURVE('',#21052,#21052,#17868,.T.);
#25099=EDGE_CURVE('',#21052,#21053,#4496,.T.);
#25100=EDGE_CURVE('',#21053,#21053,#17869,.T.);
#25101=EDGE_CURVE('',#21054,#21054,#17870,.T.);
#25102=EDGE_CURVE('',#21054,#21055,#4497,.T.);
#25103=EDGE_CURVE('',#21055,#21055,#17871,.T.);
#25104=EDGE_CURVE('',#21056,#21056,#17872,.T.);
#25105=EDGE_CURVE('',#21056,#21057,#4498,.T.);
#25106=EDGE_CURVE('',#21057,#21057,#17873,.T.);
#25107=EDGE_CURVE('',#21058,#21058,#17874,.T.);
#25108=EDGE_CURVE('',#21058,#21059,#4499,.T.);
#25109=EDGE_CURVE('',#21059,#21059,#17875,.T.);
#25110=EDGE_CURVE('',#21060,#21060,#17876,.T.);
#25111=EDGE_CURVE('',#21060,#21061,#4500,.T.);
#25112=EDGE_CURVE('',#21061,#21061,#17877,.T.);
#25113=EDGE_CURVE('',#21062,#21062,#17878,.T.);
#25114=EDGE_CURVE('',#21062,#21063,#4501,.T.);
#25115=EDGE_CURVE('',#21063,#21063,#17879,.T.);
#25116=EDGE_CURVE('',#21064,#21064,#17880,.T.);
#25117=EDGE_CURVE('',#21064,#21065,#4502,.T.);
#25118=EDGE_CURVE('',#21065,#21065,#17881,.T.);
#25119=EDGE_CURVE('',#21066,#21066,#17882,.T.);
#25120=EDGE_CURVE('',#21066,#21067,#4503,.T.);
#25121=EDGE_CURVE('',#21067,#21067,#17883,.T.);
#25122=EDGE_CURVE('',#21068,#21068,#17884,.T.);
#25123=EDGE_CURVE('',#21068,#21069,#4504,.T.);
#25124=EDGE_CURVE('',#21070,#21069,#2052,.F.);
#25125=EDGE_CURVE('',#21070,#21071,#17885,.T.);
#25126=EDGE_CURVE('',#21069,#21071,#2053,.F.);
#25127=EDGE_CURVE('',#21072,#21072,#17886,.T.);
#25128=EDGE_CURVE('',#21072,#21073,#4505,.T.);
#25129=EDGE_CURVE('',#21073,#21073,#17887,.T.);
#25130=EDGE_CURVE('',#21074,#21074,#17888,.T.);
#25131=EDGE_CURVE('',#21074,#21075,#4506,.T.);
#25132=EDGE_CURVE('',#21075,#21075,#17889,.T.);
#25133=EDGE_CURVE('',#21076,#21076,#17890,.T.);
#25134=EDGE_CURVE('',#21076,#21077,#4507,.T.);
#25135=EDGE_CURVE('',#21077,#21077,#17891,.T.);
#25136=EDGE_CURVE('',#21078,#21078,#17892,.T.);
#25137=EDGE_CURVE('',#21078,#21079,#4508,.T.);
#25138=EDGE_CURVE('',#21079,#21079,#17893,.T.);
#25139=EDGE_CURVE('',#21080,#21080,#17894,.T.);
#25140=EDGE_CURVE('',#21080,#21081,#4509,.T.);
#25141=EDGE_CURVE('',#21081,#21081,#17895,.T.);
#25142=EDGE_CURVE('',#21082,#21082,#17896,.T.);
#25143=EDGE_CURVE('',#21082,#21083,#4510,.T.);
#25144=EDGE_CURVE('',#21083,#21083,#17897,.T.);
#25145=EDGE_CURVE('',#21084,#21084,#17898,.T.);
#25146=EDGE_CURVE('',#21084,#21085,#4511,.T.);
#25147=EDGE_CURVE('',#21085,#21085,#17899,.T.);
#25148=EDGE_CURVE('',#21086,#21086,#17900,.T.);
#25149=EDGE_CURVE('',#21086,#21087,#4512,.T.);
#25150=EDGE_CURVE('',#21087,#21087,#17901,.T.);
#25151=EDGE_CURVE('',#21088,#21088,#17902,.T.);
#25152=EDGE_CURVE('',#21088,#21089,#4513,.T.);
#25153=EDGE_CURVE('',#21089,#21089,#17903,.T.);
#25154=EDGE_CURVE('',#21090,#21090,#17904,.T.);
#25155=EDGE_CURVE('',#21090,#21091,#4514,.T.);
#25156=EDGE_CURVE('',#21091,#21091,#17905,.T.);
#25157=EDGE_CURVE('',#21092,#21092,#17906,.T.);
#25158=EDGE_CURVE('',#21092,#21093,#4515,.T.);
#25159=EDGE_CURVE('',#21093,#21093,#17907,.T.);
#25160=EDGE_CURVE('',#21094,#21094,#17908,.T.);
#25161=EDGE_CURVE('',#21094,#21095,#4516,.T.);
#25162=EDGE_CURVE('',#21095,#21095,#17909,.T.);
#25163=EDGE_CURVE('',#21096,#21096,#17910,.T.);
#25164=EDGE_CURVE('',#21096,#21097,#4517,.T.);
#25165=EDGE_CURVE('',#21097,#21097,#17911,.T.);
#25166=EDGE_CURVE('',#21098,#21098,#17912,.T.);
#25167=EDGE_CURVE('',#21098,#21099,#4518,.T.);
#25168=EDGE_CURVE('',#21099,#21099,#17913,.T.);
#25169=EDGE_CURVE('',#21100,#21100,#17914,.T.);
#25170=EDGE_CURVE('',#21100,#21101,#4519,.T.);
#25171=EDGE_CURVE('',#21101,#21101,#17915,.T.);
#25172=EDGE_CURVE('',#21102,#21102,#17916,.T.);
#25173=EDGE_CURVE('',#21102,#21103,#4520,.T.);
#25174=EDGE_CURVE('',#21104,#21103,#2054,.F.);
#25175=EDGE_CURVE('',#21104,#21105,#17917,.T.);
#25176=EDGE_CURVE('',#21103,#21105,#2055,.F.);
#25177=EDGE_CURVE('',#21106,#21106,#17918,.T.);
#25178=EDGE_CURVE('',#21106,#21107,#4521,.T.);
#25179=EDGE_CURVE('',#21107,#21107,#17919,.T.);
#25180=EDGE_CURVE('',#21108,#21108,#17920,.T.);
#25181=EDGE_CURVE('',#21108,#21109,#4522,.T.);
#25182=EDGE_CURVE('',#21109,#21109,#17921,.T.);
#25183=EDGE_CURVE('',#21110,#21110,#17922,.T.);
#25184=EDGE_CURVE('',#21110,#21111,#4523,.T.);
#25185=EDGE_CURVE('',#21111,#21111,#17923,.T.);
#25186=EDGE_CURVE('',#21112,#21112,#17924,.T.);
#25187=EDGE_CURVE('',#21112,#21113,#4524,.T.);
#25188=EDGE_CURVE('',#21113,#21113,#17925,.T.);
#25189=EDGE_CURVE('',#21114,#21114,#17926,.T.);
#25190=EDGE_CURVE('',#21114,#21115,#4525,.T.);
#25191=EDGE_CURVE('',#21115,#21115,#17927,.T.);
#25192=EDGE_CURVE('',#21116,#21116,#17928,.T.);
#25193=EDGE_CURVE('',#21116,#21117,#4526,.T.);
#25194=EDGE_CURVE('',#21117,#21117,#17929,.T.);
#25195=EDGE_CURVE('',#21118,#21118,#17930,.T.);
#25196=EDGE_CURVE('',#21118,#21119,#4527,.T.);
#25197=EDGE_CURVE('',#21119,#21119,#17931,.T.);
#25198=EDGE_CURVE('',#21120,#21120,#17932,.T.);
#25199=EDGE_CURVE('',#21120,#21121,#4528,.T.);
#25200=EDGE_CURVE('',#21121,#21121,#17933,.T.);
#25201=EDGE_CURVE('',#21122,#21122,#17934,.T.);
#25202=EDGE_CURVE('',#21122,#21123,#4529,.T.);
#25203=EDGE_CURVE('',#21123,#21123,#17935,.T.);
#25204=EDGE_CURVE('',#21124,#21124,#17936,.T.);
#25205=EDGE_CURVE('',#21124,#21125,#4530,.T.);
#25206=EDGE_CURVE('',#21125,#21125,#17937,.T.);
#25207=EDGE_CURVE('',#21126,#21126,#17938,.T.);
#25208=EDGE_CURVE('',#21126,#21127,#4531,.T.);
#25209=EDGE_CURVE('',#21127,#21127,#17939,.T.);
#25210=EDGE_CURVE('',#21128,#21128,#17940,.T.);
#25211=EDGE_CURVE('',#21128,#21129,#4532,.T.);
#25212=EDGE_CURVE('',#21129,#21129,#17941,.T.);
#25213=EDGE_CURVE('',#21130,#21130,#17942,.T.);
#25214=EDGE_CURVE('',#21130,#21131,#4533,.T.);
#25215=EDGE_CURVE('',#21131,#21131,#17943,.T.);
#25216=EDGE_CURVE('',#21132,#21132,#17944,.T.);
#25217=EDGE_CURVE('',#21132,#21133,#4534,.T.);
#25218=EDGE_CURVE('',#21133,#21133,#17945,.T.);
#25219=EDGE_CURVE('',#21134,#21134,#17946,.T.);
#25220=EDGE_CURVE('',#21134,#21135,#4535,.T.);
#25221=EDGE_CURVE('',#21135,#21135,#17947,.T.);
#25222=EDGE_CURVE('',#21136,#21136,#17948,.T.);
#25223=EDGE_CURVE('',#21136,#21137,#4536,.T.);
#25224=EDGE_CURVE('',#21137,#21137,#17949,.T.);
#25225=EDGE_CURVE('',#21138,#21138,#17950,.T.);
#25226=EDGE_CURVE('',#21138,#21139,#4537,.T.);
#25227=EDGE_CURVE('',#21139,#21139,#17951,.T.);
#25228=EDGE_CURVE('',#21140,#21140,#17952,.T.);
#25229=EDGE_CURVE('',#21140,#21141,#4538,.T.);
#25230=EDGE_CURVE('',#21142,#21141,#2056,.F.);
#25231=EDGE_CURVE('',#21142,#21143,#17953,.T.);
#25232=EDGE_CURVE('',#21141,#21143,#2057,.F.);
#25233=EDGE_CURVE('',#21144,#21144,#17954,.T.);
#25234=EDGE_CURVE('',#21144,#21145,#4539,.T.);
#25235=EDGE_CURVE('',#21145,#21145,#17955,.T.);
#25236=EDGE_CURVE('',#21146,#21146,#17956,.T.);
#25237=EDGE_CURVE('',#21146,#21147,#4540,.T.);
#25238=EDGE_CURVE('',#21147,#21147,#17957,.T.);
#25239=EDGE_CURVE('',#21148,#21148,#17958,.T.);
#25240=EDGE_CURVE('',#21148,#21149,#4541,.T.);
#25241=EDGE_CURVE('',#21149,#21149,#17959,.T.);
#25242=EDGE_CURVE('',#21150,#21150,#17960,.T.);
#25243=EDGE_CURVE('',#21150,#21151,#4542,.T.);
#25244=EDGE_CURVE('',#21151,#21151,#17961,.T.);
#25245=EDGE_CURVE('',#21152,#21152,#17962,.T.);
#25246=EDGE_CURVE('',#21152,#21153,#4543,.T.);
#25247=EDGE_CURVE('',#21153,#21153,#17963,.T.);
#25248=EDGE_CURVE('',#21154,#21154,#17964,.T.);
#25249=EDGE_CURVE('',#21154,#21155,#4544,.T.);
#25250=EDGE_CURVE('',#21155,#21155,#17965,.T.);
#25251=EDGE_CURVE('',#21156,#21156,#17966,.T.);
#25252=EDGE_CURVE('',#21156,#21157,#4545,.T.);
#25253=EDGE_CURVE('',#21157,#21157,#17967,.T.);
#25254=EDGE_CURVE('',#21158,#21158,#17968,.T.);
#25255=EDGE_CURVE('',#21158,#21159,#4546,.T.);
#25256=EDGE_CURVE('',#21159,#21159,#17969,.T.);
#25257=EDGE_CURVE('',#21160,#21160,#17970,.T.);
#25258=EDGE_CURVE('',#21160,#21161,#4547,.T.);
#25259=EDGE_CURVE('',#21161,#21161,#17971,.T.);
#25260=EDGE_CURVE('',#21162,#21162,#17972,.T.);
#25261=EDGE_CURVE('',#21162,#21163,#4548,.T.);
#25262=EDGE_CURVE('',#21163,#21163,#17973,.T.);
#25263=EDGE_CURVE('',#21164,#21164,#17974,.T.);
#25264=EDGE_CURVE('',#21164,#21165,#4549,.T.);
#25265=EDGE_CURVE('',#21165,#21165,#17975,.T.);
#25266=EDGE_CURVE('',#21166,#21166,#17976,.T.);
#25267=EDGE_CURVE('',#21166,#21167,#4550,.T.);
#25268=EDGE_CURVE('',#21167,#21167,#17977,.T.);
#25269=EDGE_CURVE('',#21168,#21168,#17978,.T.);
#25270=EDGE_CURVE('',#21168,#21169,#4551,.T.);
#25271=EDGE_CURVE('',#21169,#21169,#17979,.T.);
#25272=EDGE_CURVE('',#21170,#21170,#17980,.T.);
#25273=EDGE_CURVE('',#21170,#21171,#4552,.T.);
#25274=EDGE_CURVE('',#21171,#21171,#17981,.T.);
#25275=EDGE_CURVE('',#21172,#21172,#17982,.T.);
#25276=EDGE_CURVE('',#21172,#21173,#4553,.T.);
#25277=EDGE_CURVE('',#21173,#21173,#17983,.T.);
#25278=EDGE_CURVE('',#21174,#21174,#17984,.T.);
#25279=EDGE_CURVE('',#21174,#21175,#4554,.T.);
#25280=EDGE_CURVE('',#21175,#21175,#17985,.T.);
#25281=EDGE_CURVE('',#21176,#21176,#17986,.T.);
#25282=EDGE_CURVE('',#21176,#21177,#4555,.T.);
#25283=EDGE_CURVE('',#21177,#21177,#17987,.T.);
#25284=EDGE_CURVE('',#21178,#21178,#17988,.T.);
#25285=EDGE_CURVE('',#21178,#21179,#4556,.T.);
#25286=EDGE_CURVE('',#21180,#21179,#2058,.F.);
#25287=EDGE_CURVE('',#21180,#21181,#17989,.T.);
#25288=EDGE_CURVE('',#21179,#21181,#2059,.F.);
#25289=EDGE_CURVE('',#21182,#21182,#17990,.T.);
#25290=EDGE_CURVE('',#21182,#21183,#4557,.T.);
#25291=EDGE_CURVE('',#21183,#21183,#17991,.T.);
#25292=EDGE_CURVE('',#21184,#21184,#17992,.T.);
#25293=EDGE_CURVE('',#21184,#21185,#4558,.T.);
#25294=EDGE_CURVE('',#21185,#21185,#17993,.T.);
#25295=EDGE_CURVE('',#21186,#21186,#17994,.T.);
#25296=EDGE_CURVE('',#21186,#21187,#4559,.T.);
#25297=EDGE_CURVE('',#21187,#21187,#17995,.T.);
#25298=EDGE_CURVE('',#21188,#21188,#17996,.T.);
#25299=EDGE_CURVE('',#21188,#21189,#4560,.T.);
#25300=EDGE_CURVE('',#21189,#21189,#17997,.T.);
#25301=EDGE_CURVE('',#21190,#21190,#17998,.T.);
#25302=EDGE_CURVE('',#21190,#21191,#4561,.T.);
#25303=EDGE_CURVE('',#21191,#21191,#17999,.T.);
#25304=EDGE_CURVE('',#21192,#21192,#18000,.T.);
#25305=EDGE_CURVE('',#21192,#21193,#4562,.T.);
#25306=EDGE_CURVE('',#21193,#21193,#18001,.T.);
#25307=EDGE_CURVE('',#21194,#21194,#18002,.T.);
#25308=EDGE_CURVE('',#21194,#21195,#4563,.T.);
#25309=EDGE_CURVE('',#21195,#21195,#18003,.T.);
#25310=EDGE_CURVE('',#21196,#21196,#18004,.T.);
#25311=EDGE_CURVE('',#21196,#21197,#4564,.T.);
#25312=EDGE_CURVE('',#21197,#21197,#18005,.T.);
#25313=EDGE_CURVE('',#21198,#21198,#18006,.T.);
#25314=EDGE_CURVE('',#21198,#21199,#4565,.T.);
#25315=EDGE_CURVE('',#21199,#21199,#18007,.T.);
#25316=EDGE_CURVE('',#21200,#21200,#18008,.T.);
#25317=EDGE_CURVE('',#21200,#21201,#4566,.T.);
#25318=EDGE_CURVE('',#21201,#21201,#18009,.T.);
#25319=EDGE_CURVE('',#21202,#21202,#18010,.T.);
#25320=EDGE_CURVE('',#21202,#21203,#4567,.T.);
#25321=EDGE_CURVE('',#21203,#21203,#18011,.T.);
#25322=EDGE_CURVE('',#21204,#21204,#18012,.T.);
#25323=EDGE_CURVE('',#21204,#21205,#4568,.T.);
#25324=EDGE_CURVE('',#21205,#21205,#18013,.T.);
#25325=EDGE_CURVE('',#21206,#21206,#18014,.T.);
#25326=EDGE_CURVE('',#21206,#21207,#4569,.T.);
#25327=EDGE_CURVE('',#21207,#21207,#18015,.T.);
#25328=EDGE_CURVE('',#21208,#21208,#18016,.T.);
#25329=EDGE_CURVE('',#21208,#21209,#4570,.T.);
#25330=EDGE_CURVE('',#21209,#21209,#18017,.T.);
#25331=EDGE_CURVE('',#21210,#21210,#18018,.T.);
#25332=EDGE_CURVE('',#21210,#21211,#4571,.T.);
#25333=EDGE_CURVE('',#21211,#21211,#18019,.T.);
#25334=EDGE_CURVE('',#21212,#21212,#18020,.T.);
#25335=EDGE_CURVE('',#21212,#21213,#4572,.T.);
#25336=EDGE_CURVE('',#21213,#21213,#18021,.T.);
#25337=EDGE_CURVE('',#21214,#21214,#18022,.T.);
#25338=EDGE_CURVE('',#21214,#21215,#4573,.T.);
#25339=EDGE_CURVE('',#21215,#21215,#18023,.T.);
#25340=EDGE_CURVE('',#21216,#21216,#18024,.T.);
#25341=EDGE_CURVE('',#21216,#21217,#4574,.T.);
#25342=EDGE_CURVE('',#21218,#21217,#2060,.F.);
#25343=EDGE_CURVE('',#21218,#21219,#18025,.T.);
#25344=EDGE_CURVE('',#21217,#21219,#2061,.F.);
#25345=EDGE_CURVE('',#21220,#21220,#18026,.T.);
#25346=EDGE_CURVE('',#21220,#21221,#4575,.T.);
#25347=EDGE_CURVE('',#21221,#21221,#18027,.T.);
#25348=EDGE_CURVE('',#21222,#21222,#18028,.T.);
#25349=EDGE_CURVE('',#21222,#21223,#4576,.T.);
#25350=EDGE_CURVE('',#21223,#21223,#18029,.T.);
#25351=EDGE_CURVE('',#21224,#21224,#18030,.T.);
#25352=EDGE_CURVE('',#21224,#21225,#4577,.T.);
#25353=EDGE_CURVE('',#21225,#21225,#18031,.T.);
#25354=EDGE_CURVE('',#21226,#21226,#18032,.T.);
#25355=EDGE_CURVE('',#21226,#21227,#4578,.T.);
#25356=EDGE_CURVE('',#21227,#21227,#18033,.T.);
#25357=EDGE_CURVE('',#21228,#21228,#18034,.T.);
#25358=EDGE_CURVE('',#21228,#21229,#4579,.T.);
#25359=EDGE_CURVE('',#21229,#21229,#18035,.T.);
#25360=EDGE_CURVE('',#21230,#21230,#18036,.T.);
#25361=EDGE_CURVE('',#21230,#21231,#4580,.T.);
#25362=EDGE_CURVE('',#21231,#21231,#18037,.T.);
#25363=EDGE_CURVE('',#21232,#21232,#18038,.T.);
#25364=EDGE_CURVE('',#21232,#21233,#4581,.T.);
#25365=EDGE_CURVE('',#21233,#21233,#18039,.T.);
#25366=EDGE_CURVE('',#21234,#21234,#18040,.T.);
#25367=EDGE_CURVE('',#21234,#21235,#4582,.T.);
#25368=EDGE_CURVE('',#21235,#21235,#18041,.T.);
#25369=EDGE_CURVE('',#21236,#21236,#18042,.T.);
#25370=EDGE_CURVE('',#21236,#21237,#4583,.T.);
#25371=EDGE_CURVE('',#21237,#21237,#18043,.T.);
#25372=EDGE_CURVE('',#21238,#21238,#18044,.T.);
#25373=EDGE_CURVE('',#21238,#21239,#4584,.T.);
#25374=EDGE_CURVE('',#21239,#21239,#18045,.T.);
#25375=EDGE_CURVE('',#21240,#21240,#18046,.T.);
#25376=EDGE_CURVE('',#21240,#21241,#4585,.T.);
#25377=EDGE_CURVE('',#21241,#21241,#18047,.T.);
#25378=EDGE_CURVE('',#21242,#21242,#18048,.T.);
#25379=EDGE_CURVE('',#21242,#21243,#4586,.T.);
#25380=EDGE_CURVE('',#21243,#21243,#18049,.T.);
#25381=EDGE_CURVE('',#21244,#21244,#18050,.T.);
#25382=EDGE_CURVE('',#21244,#21245,#4587,.T.);
#25383=EDGE_CURVE('',#21245,#21245,#18051,.T.);
#25384=EDGE_CURVE('',#21246,#21246,#18052,.T.);
#25385=EDGE_CURVE('',#21246,#21247,#4588,.T.);
#25386=EDGE_CURVE('',#21247,#21247,#18053,.T.);
#25387=EDGE_CURVE('',#21248,#21248,#18054,.T.);
#25388=EDGE_CURVE('',#21248,#21249,#4589,.T.);
#25389=EDGE_CURVE('',#21249,#21249,#18055,.T.);
#25390=EDGE_CURVE('',#21250,#21250,#18056,.T.);
#25391=EDGE_CURVE('',#21250,#21251,#4590,.T.);
#25392=EDGE_CURVE('',#21251,#21251,#18057,.T.);
#25393=EDGE_CURVE('',#21252,#21252,#18058,.T.);
#25394=EDGE_CURVE('',#21252,#21253,#4591,.T.);
#25395=EDGE_CURVE('',#21253,#21253,#18059,.T.);
#25396=EDGE_CURVE('',#21254,#21254,#18060,.T.);
#25397=EDGE_CURVE('',#21254,#21255,#4592,.T.);
#25398=EDGE_CURVE('',#21256,#21255,#2062,.F.);
#25399=EDGE_CURVE('',#21256,#21257,#18061,.T.);
#25400=EDGE_CURVE('',#21255,#21257,#2063,.F.);
#25401=EDGE_CURVE('',#21258,#21258,#18062,.T.);
#25402=EDGE_CURVE('',#21258,#21259,#4593,.T.);
#25403=EDGE_CURVE('',#21259,#21259,#18063,.T.);
#25404=EDGE_CURVE('',#21260,#21260,#18064,.T.);
#25405=EDGE_CURVE('',#21260,#21261,#4594,.T.);
#25406=EDGE_CURVE('',#21261,#21261,#18065,.T.);
#25407=EDGE_CURVE('',#21262,#21262,#18066,.T.);
#25408=EDGE_CURVE('',#21262,#21263,#4595,.T.);
#25409=EDGE_CURVE('',#21263,#21263,#18067,.T.);
#25410=EDGE_CURVE('',#21264,#21264,#18068,.T.);
#25411=EDGE_CURVE('',#21264,#21265,#4596,.T.);
#25412=EDGE_CURVE('',#21265,#21265,#18069,.T.);
#25413=EDGE_CURVE('',#21266,#21266,#18070,.T.);
#25414=EDGE_CURVE('',#21266,#21267,#4597,.T.);
#25415=EDGE_CURVE('',#21267,#21267,#18071,.T.);
#25416=EDGE_CURVE('',#21268,#21268,#18072,.T.);
#25417=EDGE_CURVE('',#21268,#21269,#4598,.T.);
#25418=EDGE_CURVE('',#21269,#21269,#18073,.T.);
#25419=EDGE_CURVE('',#21270,#21270,#18074,.T.);
#25420=EDGE_CURVE('',#21270,#21271,#4599,.T.);
#25421=EDGE_CURVE('',#21271,#21271,#18075,.T.);
#25422=EDGE_CURVE('',#21272,#21272,#18076,.T.);
#25423=EDGE_CURVE('',#21272,#21273,#4600,.T.);
#25424=EDGE_CURVE('',#21273,#21273,#18077,.T.);
#25425=EDGE_CURVE('',#21274,#21274,#18078,.T.);
#25426=EDGE_CURVE('',#21274,#21275,#4601,.T.);
#25427=EDGE_CURVE('',#21275,#21275,#18079,.T.);
#25428=EDGE_CURVE('',#21276,#21276,#18080,.T.);
#25429=EDGE_CURVE('',#21276,#21277,#4602,.T.);
#25430=EDGE_CURVE('',#21277,#21277,#18081,.T.);
#25431=EDGE_CURVE('',#21278,#21278,#18082,.T.);
#25432=EDGE_CURVE('',#21278,#21279,#4603,.T.);
#25433=EDGE_CURVE('',#21279,#21279,#18083,.T.);
#25434=EDGE_CURVE('',#21280,#21280,#18084,.T.);
#25435=EDGE_CURVE('',#21280,#21281,#4604,.T.);
#25436=EDGE_CURVE('',#21281,#21281,#18085,.T.);
#25437=EDGE_CURVE('',#21282,#21282,#18086,.T.);
#25438=EDGE_CURVE('',#21282,#21283,#4605,.T.);
#25439=EDGE_CURVE('',#21283,#21283,#18087,.T.);
#25440=EDGE_CURVE('',#21284,#21284,#18088,.T.);
#25441=EDGE_CURVE('',#21284,#21285,#4606,.T.);
#25442=EDGE_CURVE('',#21285,#21285,#18089,.T.);
#25443=EDGE_CURVE('',#21286,#21286,#18090,.T.);
#25444=EDGE_CURVE('',#21286,#21287,#4607,.T.);
#25445=EDGE_CURVE('',#21287,#21287,#18091,.T.);
#25446=EDGE_CURVE('',#21288,#21288,#18092,.T.);
#25447=EDGE_CURVE('',#21288,#21289,#4608,.T.);
#25448=EDGE_CURVE('',#21290,#21289,#2064,.F.);
#25449=EDGE_CURVE('',#21290,#21291,#18093,.T.);
#25450=EDGE_CURVE('',#21289,#21291,#2065,.F.);
#25451=EDGE_CURVE('',#21292,#21292,#18094,.T.);
#25452=EDGE_CURVE('',#21292,#21293,#4609,.T.);
#25453=EDGE_CURVE('',#21293,#21293,#18095,.T.);
#25454=EDGE_CURVE('',#21294,#21294,#18096,.T.);
#25455=EDGE_CURVE('',#21294,#21295,#4610,.T.);
#25456=EDGE_CURVE('',#21295,#21295,#18097,.T.);
#25457=EDGE_CURVE('',#21296,#21296,#18098,.T.);
#25458=EDGE_CURVE('',#21296,#21297,#4611,.T.);
#25459=EDGE_CURVE('',#21297,#21297,#18099,.T.);
#25460=EDGE_CURVE('',#21298,#21298,#18100,.T.);
#25461=EDGE_CURVE('',#21298,#21299,#4612,.T.);
#25462=EDGE_CURVE('',#21299,#21299,#18101,.T.);
#25463=EDGE_CURVE('',#21300,#21300,#18102,.T.);
#25464=EDGE_CURVE('',#21300,#21301,#4613,.T.);
#25465=EDGE_CURVE('',#21301,#21301,#18103,.T.);
#25466=EDGE_CURVE('',#21302,#21302,#18104,.T.);
#25467=EDGE_CURVE('',#21302,#21303,#4614,.T.);
#25468=EDGE_CURVE('',#21303,#21303,#18105,.T.);
#25469=EDGE_CURVE('',#21304,#21304,#18106,.T.);
#25470=EDGE_CURVE('',#21304,#21305,#4615,.T.);
#25471=EDGE_CURVE('',#21305,#21305,#18107,.T.);
#25472=EDGE_CURVE('',#21306,#21306,#18108,.T.);
#25473=EDGE_CURVE('',#21306,#21307,#4616,.T.);
#25474=EDGE_CURVE('',#21307,#21307,#18109,.T.);
#25475=EDGE_CURVE('',#21308,#21308,#18110,.T.);
#25476=EDGE_CURVE('',#21308,#21309,#4617,.T.);
#25477=EDGE_CURVE('',#21309,#21309,#18111,.T.);
#25478=EDGE_CURVE('',#21310,#21310,#18112,.T.);
#25479=EDGE_CURVE('',#21310,#21311,#4618,.T.);
#25480=EDGE_CURVE('',#21311,#21311,#18113,.T.);
#25481=EDGE_CURVE('',#21312,#21312,#18114,.T.);
#25482=EDGE_CURVE('',#21312,#21313,#4619,.T.);
#25483=EDGE_CURVE('',#21313,#21313,#18115,.T.);
#25484=EDGE_CURVE('',#21314,#21314,#18116,.T.);
#25485=EDGE_CURVE('',#21314,#21315,#4620,.T.);
#25486=EDGE_CURVE('',#21315,#21315,#18117,.T.);
#25487=EDGE_CURVE('',#21316,#21316,#18118,.T.);
#25488=EDGE_CURVE('',#21316,#21317,#4621,.T.);
#25489=EDGE_CURVE('',#21317,#21317,#18119,.T.);
#25490=EDGE_CURVE('',#21318,#21318,#18120,.T.);
#25491=EDGE_CURVE('',#21318,#21319,#4622,.T.);
#25492=EDGE_CURVE('',#21319,#21319,#18121,.T.);
#25493=EDGE_CURVE('',#21320,#21320,#18122,.T.);
#25494=EDGE_CURVE('',#21320,#21321,#4623,.T.);
#25495=EDGE_CURVE('',#21321,#21321,#18123,.T.);
#25496=EDGE_CURVE('',#21322,#21322,#18124,.T.);
#25497=EDGE_CURVE('',#21322,#21323,#4624,.T.);
#25498=EDGE_CURVE('',#21323,#21323,#18125,.T.);
#25499=EDGE_CURVE('',#21324,#21324,#18126,.T.);
#25500=EDGE_CURVE('',#21324,#21325,#4625,.T.);
#25501=EDGE_CURVE('',#21325,#21325,#18127,.T.);
#25502=EDGE_CURVE('',#21326,#21326,#18128,.T.);
#25503=EDGE_CURVE('',#21326,#21327,#4626,.T.);
#25504=EDGE_CURVE('',#21328,#21327,#2066,.F.);
#25505=EDGE_CURVE('',#21328,#21329,#18129,.T.);
#25506=EDGE_CURVE('',#21327,#21329,#2067,.F.);
#25507=EDGE_CURVE('',#21330,#21330,#18130,.T.);
#25508=EDGE_CURVE('',#21330,#21331,#4627,.T.);
#25509=EDGE_CURVE('',#21331,#21331,#18131,.T.);
#25510=EDGE_CURVE('',#21332,#21332,#18132,.T.);
#25511=EDGE_CURVE('',#21332,#21333,#4628,.T.);
#25512=EDGE_CURVE('',#21333,#21333,#18133,.T.);
#25513=EDGE_CURVE('',#21334,#21334,#18134,.T.);
#25514=EDGE_CURVE('',#21334,#21335,#4629,.T.);
#25515=EDGE_CURVE('',#21335,#21335,#18135,.T.);
#25516=EDGE_CURVE('',#21336,#21336,#18136,.T.);
#25517=EDGE_CURVE('',#21336,#21337,#4630,.T.);
#25518=EDGE_CURVE('',#21337,#21337,#18137,.T.);
#25519=EDGE_CURVE('',#21338,#21338,#18138,.T.);
#25520=EDGE_CURVE('',#21338,#21339,#4631,.T.);
#25521=EDGE_CURVE('',#21339,#21339,#18139,.T.);
#25522=EDGE_CURVE('',#21340,#21340,#18140,.T.);
#25523=EDGE_CURVE('',#21340,#21341,#4632,.T.);
#25524=EDGE_CURVE('',#21341,#21341,#18141,.T.);
#25525=EDGE_CURVE('',#21342,#21342,#18142,.T.);
#25526=EDGE_CURVE('',#21342,#21343,#4633,.T.);
#25527=EDGE_CURVE('',#21343,#21343,#18143,.T.);
#25528=EDGE_CURVE('',#21344,#21344,#18144,.T.);
#25529=EDGE_CURVE('',#21344,#21345,#4634,.T.);
#25530=EDGE_CURVE('',#21345,#21345,#18145,.T.);
#25531=EDGE_CURVE('',#21346,#21346,#18146,.T.);
#25532=EDGE_CURVE('',#21346,#21347,#4635,.T.);
#25533=EDGE_CURVE('',#21347,#21347,#18147,.T.);
#25534=EDGE_CURVE('',#21348,#21348,#18148,.T.);
#25535=EDGE_CURVE('',#21348,#21349,#4636,.T.);
#25536=EDGE_CURVE('',#21349,#21349,#18149,.T.);
#25537=EDGE_CURVE('',#21350,#21350,#18150,.T.);
#25538=EDGE_CURVE('',#21350,#21351,#4637,.T.);
#25539=EDGE_CURVE('',#21351,#21351,#18151,.T.);
#25540=EDGE_CURVE('',#21352,#21352,#18152,.T.);
#25541=EDGE_CURVE('',#21352,#21353,#4638,.T.);
#25542=EDGE_CURVE('',#21353,#21353,#18153,.T.);
#25543=EDGE_CURVE('',#21354,#21354,#18154,.T.);
#25544=EDGE_CURVE('',#21354,#21355,#4639,.T.);
#25545=EDGE_CURVE('',#21355,#21355,#18155,.T.);
#25546=EDGE_CURVE('',#21356,#21356,#18156,.T.);
#25547=EDGE_CURVE('',#21356,#21357,#4640,.T.);
#25548=EDGE_CURVE('',#21357,#21357,#18157,.T.);
#25549=EDGE_CURVE('',#21358,#21358,#18158,.T.);
#25550=EDGE_CURVE('',#21358,#21359,#4641,.T.);
#25551=EDGE_CURVE('',#21359,#21359,#18159,.T.);
#25552=EDGE_CURVE('',#21360,#21360,#18160,.T.);
#25553=EDGE_CURVE('',#21360,#21361,#4642,.T.);
#25554=EDGE_CURVE('',#21361,#21361,#18161,.T.);
#25555=EDGE_CURVE('',#21362,#21362,#18162,.T.);
#25556=EDGE_CURVE('',#21362,#21363,#4643,.T.);
#25557=EDGE_CURVE('',#21363,#21363,#18163,.T.);
#25558=EDGE_CURVE('',#21364,#21364,#18164,.T.);
#25559=EDGE_CURVE('',#21364,#21365,#4644,.T.);
#25560=EDGE_CURVE('',#21366,#21365,#2068,.F.);
#25561=EDGE_CURVE('',#21366,#21367,#18165,.T.);
#25562=EDGE_CURVE('',#21365,#21367,#2069,.F.);
#25563=EDGE_CURVE('',#21368,#21368,#18166,.T.);
#25564=EDGE_CURVE('',#21368,#21369,#4645,.T.);
#25565=EDGE_CURVE('',#21369,#21369,#18167,.T.);
#25566=EDGE_CURVE('',#21370,#21370,#18168,.T.);
#25567=EDGE_CURVE('',#21370,#21371,#4646,.T.);
#25568=EDGE_CURVE('',#21371,#21371,#18169,.T.);
#25569=EDGE_CURVE('',#21372,#21372,#18170,.T.);
#25570=EDGE_CURVE('',#21372,#21373,#4647,.T.);
#25571=EDGE_CURVE('',#21373,#21373,#18171,.T.);
#25572=EDGE_CURVE('',#21374,#21374,#18172,.T.);
#25573=EDGE_CURVE('',#21374,#21375,#4648,.T.);
#25574=EDGE_CURVE('',#21375,#21375,#18173,.T.);
#25575=EDGE_CURVE('',#21376,#21376,#18174,.T.);
#25576=EDGE_CURVE('',#21376,#21377,#4649,.T.);
#25577=EDGE_CURVE('',#21377,#21377,#18175,.T.);
#25578=EDGE_CURVE('',#21378,#21378,#18176,.T.);
#25579=EDGE_CURVE('',#21378,#21379,#4650,.T.);
#25580=EDGE_CURVE('',#21379,#21379,#18177,.T.);
#25581=EDGE_CURVE('',#21380,#21380,#18178,.T.);
#25582=EDGE_CURVE('',#21380,#21381,#4651,.T.);
#25583=EDGE_CURVE('',#21381,#21381,#18179,.T.);
#25584=EDGE_CURVE('',#21382,#21382,#18180,.T.);
#25585=EDGE_CURVE('',#21382,#21383,#4652,.T.);
#25586=EDGE_CURVE('',#21383,#21383,#18181,.T.);
#25587=EDGE_CURVE('',#21384,#21384,#18182,.T.);
#25588=EDGE_CURVE('',#21384,#21385,#4653,.T.);
#25589=EDGE_CURVE('',#21385,#21385,#18183,.T.);
#25590=EDGE_CURVE('',#21386,#21386,#18184,.T.);
#25591=EDGE_CURVE('',#21386,#21387,#4654,.T.);
#25592=EDGE_CURVE('',#21387,#21387,#18185,.T.);
#25593=EDGE_CURVE('',#21388,#21388,#18186,.T.);
#25594=EDGE_CURVE('',#21388,#21389,#4655,.T.);
#25595=EDGE_CURVE('',#21389,#21389,#18187,.T.);
#25596=EDGE_CURVE('',#21390,#21390,#18188,.T.);
#25597=EDGE_CURVE('',#21390,#21391,#4656,.T.);
#25598=EDGE_CURVE('',#21391,#21391,#18189,.T.);
#25599=EDGE_CURVE('',#21392,#21392,#18190,.T.);
#25600=EDGE_CURVE('',#21392,#21393,#4657,.T.);
#25601=EDGE_CURVE('',#21393,#21393,#18191,.T.);
#25602=EDGE_CURVE('',#21394,#21394,#18192,.T.);
#25603=EDGE_CURVE('',#21394,#21395,#4658,.T.);
#25604=EDGE_CURVE('',#21395,#21395,#18193,.T.);
#25605=EDGE_CURVE('',#21396,#21396,#18194,.T.);
#25606=EDGE_CURVE('',#21396,#21397,#4659,.T.);
#25607=EDGE_CURVE('',#21397,#21397,#18195,.T.);
#25608=EDGE_CURVE('',#21398,#21398,#18196,.T.);
#25609=EDGE_CURVE('',#21398,#21399,#4660,.T.);
#25610=EDGE_CURVE('',#21399,#21399,#18197,.T.);
#25611=EDGE_CURVE('',#21400,#21400,#18198,.T.);
#25612=EDGE_CURVE('',#21400,#21401,#4661,.T.);
#25613=EDGE_CURVE('',#21401,#21401,#18199,.T.);
#25614=EDGE_CURVE('',#21402,#21402,#18200,.T.);
#25615=EDGE_CURVE('',#21402,#21403,#4662,.T.);
#25616=EDGE_CURVE('',#21404,#21403,#2070,.F.);
#25617=EDGE_CURVE('',#21404,#21405,#18201,.T.);
#25618=EDGE_CURVE('',#21403,#21405,#2071,.F.);
#25619=EDGE_CURVE('',#21406,#21406,#18202,.T.);
#25620=EDGE_CURVE('',#21406,#21407,#4663,.T.);
#25621=EDGE_CURVE('',#21407,#21407,#18203,.T.);
#25622=EDGE_CURVE('',#21408,#21408,#18204,.T.);
#25623=EDGE_CURVE('',#21408,#21409,#4664,.T.);
#25624=EDGE_CURVE('',#21409,#21409,#18205,.T.);
#25625=EDGE_CURVE('',#21410,#21410,#18206,.T.);
#25626=EDGE_CURVE('',#21410,#21411,#4665,.T.);
#25627=EDGE_CURVE('',#21411,#21411,#18207,.T.);
#25628=EDGE_CURVE('',#21412,#21412,#18208,.T.);
#25629=EDGE_CURVE('',#21412,#21413,#4666,.T.);
#25630=EDGE_CURVE('',#21413,#21413,#18209,.T.);
#25631=EDGE_CURVE('',#21414,#21414,#18210,.T.);
#25632=EDGE_CURVE('',#21414,#21415,#4667,.T.);
#25633=EDGE_CURVE('',#21415,#21415,#18211,.T.);
#25634=EDGE_CURVE('',#21416,#21416,#18212,.T.);
#25635=EDGE_CURVE('',#21416,#21417,#4668,.T.);
#25636=EDGE_CURVE('',#21417,#21417,#18213,.T.);
#25637=EDGE_CURVE('',#21418,#21418,#18214,.T.);
#25638=EDGE_CURVE('',#21418,#21419,#4669,.T.);
#25639=EDGE_CURVE('',#21419,#21419,#18215,.T.);
#25640=EDGE_CURVE('',#21420,#21420,#18216,.T.);
#25641=EDGE_CURVE('',#21420,#21421,#4670,.T.);
#25642=EDGE_CURVE('',#21421,#21421,#18217,.T.);
#25643=EDGE_CURVE('',#21422,#21422,#18218,.T.);
#25644=EDGE_CURVE('',#21422,#21423,#4671,.T.);
#25645=EDGE_CURVE('',#21423,#21423,#18219,.T.);
#25646=EDGE_CURVE('',#21424,#21424,#18220,.T.);
#25647=EDGE_CURVE('',#21424,#21425,#4672,.T.);
#25648=EDGE_CURVE('',#21425,#21425,#18221,.T.);
#25649=EDGE_CURVE('',#21426,#21426,#18222,.T.);
#25650=EDGE_CURVE('',#21426,#21427,#4673,.T.);
#25651=EDGE_CURVE('',#21427,#21427,#18223,.T.);
#25652=EDGE_CURVE('',#21428,#21428,#18224,.T.);
#25653=EDGE_CURVE('',#21428,#21429,#4674,.T.);
#25654=EDGE_CURVE('',#21429,#21429,#18225,.T.);
#25655=EDGE_CURVE('',#21430,#21430,#18226,.T.);
#25656=EDGE_CURVE('',#21430,#21431,#4675,.T.);
#25657=EDGE_CURVE('',#21431,#21431,#18227,.T.);
#25658=EDGE_CURVE('',#21432,#21432,#18228,.T.);
#25659=EDGE_CURVE('',#21432,#21433,#4676,.T.);
#25660=EDGE_CURVE('',#21433,#21433,#18229,.T.);
#25661=EDGE_CURVE('',#21434,#21434,#18230,.T.);
#25662=EDGE_CURVE('',#21434,#21435,#4677,.T.);
#25663=EDGE_CURVE('',#21435,#21435,#18231,.T.);
#25664=EDGE_CURVE('',#21436,#21436,#18232,.T.);
#25665=EDGE_CURVE('',#21436,#21437,#4678,.T.);
#25666=EDGE_CURVE('',#21437,#21437,#18233,.T.);
#25667=EDGE_CURVE('',#21438,#21438,#18234,.T.);
#25668=EDGE_CURVE('',#21438,#21439,#4679,.T.);
#25669=EDGE_CURVE('',#21439,#21439,#18235,.T.);
#25670=EDGE_CURVE('',#21440,#21440,#18236,.T.);
#25671=EDGE_CURVE('',#21440,#21441,#4680,.T.);
#25672=EDGE_CURVE('',#21442,#21441,#2072,.F.);
#25673=EDGE_CURVE('',#21442,#21443,#18237,.T.);
#25674=EDGE_CURVE('',#21441,#21443,#2073,.F.);
#25675=EDGE_CURVE('',#21444,#21444,#18238,.T.);
#25676=EDGE_CURVE('',#21444,#21445,#4681,.T.);
#25677=EDGE_CURVE('',#21445,#21445,#18239,.T.);
#25678=EDGE_CURVE('',#21446,#21446,#18240,.T.);
#25679=EDGE_CURVE('',#21446,#21447,#4682,.T.);
#25680=EDGE_CURVE('',#21447,#21447,#18241,.T.);
#25681=EDGE_CURVE('',#21448,#21448,#18242,.T.);
#25682=EDGE_CURVE('',#21448,#21449,#4683,.T.);
#25683=EDGE_CURVE('',#21449,#21449,#18243,.T.);
#25684=EDGE_CURVE('',#21450,#21450,#18244,.T.);
#25685=EDGE_CURVE('',#21450,#21451,#4684,.T.);
#25686=EDGE_CURVE('',#21451,#21451,#18245,.T.);
#25687=EDGE_CURVE('',#21452,#21452,#18246,.T.);
#25688=EDGE_CURVE('',#21452,#21453,#4685,.T.);
#25689=EDGE_CURVE('',#21453,#21453,#18247,.T.);
#25690=EDGE_CURVE('',#21454,#21454,#18248,.T.);
#25691=EDGE_CURVE('',#21454,#21455,#4686,.T.);
#25692=EDGE_CURVE('',#21455,#21455,#18249,.T.);
#25693=EDGE_CURVE('',#21456,#21456,#18250,.T.);
#25694=EDGE_CURVE('',#21456,#21457,#4687,.T.);
#25695=EDGE_CURVE('',#21457,#21457,#18251,.T.);
#25696=EDGE_CURVE('',#21458,#21458,#18252,.T.);
#25697=EDGE_CURVE('',#21458,#21459,#4688,.T.);
#25698=EDGE_CURVE('',#21459,#21459,#18253,.T.);
#25699=EDGE_CURVE('',#21460,#21460,#18254,.T.);
#25700=EDGE_CURVE('',#21460,#21461,#4689,.T.);
#25701=EDGE_CURVE('',#21461,#21461,#18255,.T.);
#25702=EDGE_CURVE('',#21462,#21462,#18256,.T.);
#25703=EDGE_CURVE('',#21462,#21463,#4690,.T.);
#25704=EDGE_CURVE('',#21463,#21463,#18257,.T.);
#25705=EDGE_CURVE('',#21464,#21464,#18258,.T.);
#25706=EDGE_CURVE('',#21464,#21465,#4691,.T.);
#25707=EDGE_CURVE('',#21465,#21465,#18259,.T.);
#25708=EDGE_CURVE('',#21466,#21466,#18260,.T.);
#25709=EDGE_CURVE('',#21466,#21467,#4692,.T.);
#25710=EDGE_CURVE('',#21467,#21467,#18261,.T.);
#25711=EDGE_CURVE('',#21468,#21468,#18262,.T.);
#25712=EDGE_CURVE('',#21468,#21469,#4693,.T.);
#25713=EDGE_CURVE('',#21469,#21469,#18263,.T.);
#25714=EDGE_CURVE('',#21470,#21470,#18264,.T.);
#25715=EDGE_CURVE('',#21470,#21471,#4694,.T.);
#25716=EDGE_CURVE('',#21471,#21471,#18265,.T.);
#25717=EDGE_CURVE('',#21472,#21472,#18266,.T.);
#25718=EDGE_CURVE('',#21472,#21473,#4695,.T.);
#25719=EDGE_CURVE('',#21473,#21473,#18267,.T.);
#25720=EDGE_CURVE('',#21474,#21474,#18268,.T.);
#25721=EDGE_CURVE('',#21474,#21475,#4696,.T.);
#25722=EDGE_CURVE('',#21476,#21475,#2074,.F.);
#25723=EDGE_CURVE('',#21476,#21477,#18269,.T.);
#25724=EDGE_CURVE('',#21475,#21477,#2075,.F.);
#25725=EDGE_CURVE('',#21478,#21478,#18270,.T.);
#25726=EDGE_CURVE('',#21478,#21479,#4697,.T.);
#25727=EDGE_CURVE('',#21479,#21479,#18271,.T.);
#25728=EDGE_CURVE('',#21480,#21480,#18272,.T.);
#25729=EDGE_CURVE('',#21480,#21481,#4698,.T.);
#25730=EDGE_CURVE('',#21481,#21481,#18273,.T.);
#25731=EDGE_CURVE('',#21482,#21482,#18274,.T.);
#25732=EDGE_CURVE('',#21482,#21483,#4699,.T.);
#25733=EDGE_CURVE('',#21483,#21483,#18275,.T.);
#25734=EDGE_CURVE('',#21484,#21484,#18276,.T.);
#25735=EDGE_CURVE('',#21484,#21485,#4700,.T.);
#25736=EDGE_CURVE('',#21485,#21485,#18277,.T.);
#25737=EDGE_CURVE('',#21486,#21486,#18278,.T.);
#25738=EDGE_CURVE('',#21486,#21487,#4701,.T.);
#25739=EDGE_CURVE('',#21487,#21487,#18279,.T.);
#25740=EDGE_CURVE('',#21488,#21488,#18280,.T.);
#25741=EDGE_CURVE('',#21488,#21489,#4702,.T.);
#25742=EDGE_CURVE('',#21489,#21489,#18281,.T.);
#25743=EDGE_CURVE('',#21490,#21490,#18282,.T.);
#25744=EDGE_CURVE('',#21490,#21491,#4703,.T.);
#25745=EDGE_CURVE('',#21491,#21491,#18283,.T.);
#25746=EDGE_CURVE('',#21492,#21492,#18284,.T.);
#25747=EDGE_CURVE('',#21492,#21493,#4704,.T.);
#25748=EDGE_CURVE('',#21493,#21493,#18285,.T.);
#25749=EDGE_CURVE('',#21494,#21494,#18286,.T.);
#25750=EDGE_CURVE('',#21494,#21495,#4705,.T.);
#25751=EDGE_CURVE('',#21495,#21495,#18287,.T.);
#25752=EDGE_CURVE('',#21496,#21496,#18288,.T.);
#25753=EDGE_CURVE('',#21496,#21497,#4706,.T.);
#25754=EDGE_CURVE('',#21497,#21497,#18289,.T.);
#25755=EDGE_CURVE('',#21498,#21498,#18290,.T.);
#25756=EDGE_CURVE('',#21498,#21499,#4707,.T.);
#25757=EDGE_CURVE('',#21499,#21499,#18291,.T.);
#25758=EDGE_CURVE('',#21500,#21500,#18292,.T.);
#25759=EDGE_CURVE('',#21500,#21501,#4708,.T.);
#25760=EDGE_CURVE('',#21501,#21501,#18293,.T.);
#25761=EDGE_CURVE('',#21502,#21502,#18294,.T.);
#25762=EDGE_CURVE('',#21502,#21503,#4709,.T.);
#25763=EDGE_CURVE('',#21503,#21503,#18295,.T.);
#25764=EDGE_CURVE('',#21504,#21504,#18296,.T.);
#25765=EDGE_CURVE('',#21504,#21505,#4710,.T.);
#25766=EDGE_CURVE('',#21505,#21505,#18297,.T.);
#25767=EDGE_CURVE('',#21506,#21506,#18298,.T.);
#25768=EDGE_CURVE('',#21506,#21507,#4711,.T.);
#25769=EDGE_CURVE('',#21507,#21507,#18299,.T.);
#25770=EDGE_CURVE('',#21508,#21508,#18300,.T.);
#25771=EDGE_CURVE('',#21508,#21509,#4712,.T.);
#25772=EDGE_CURVE('',#21509,#21509,#18301,.T.);
#25773=EDGE_CURVE('',#21510,#21510,#18302,.T.);
#25774=EDGE_CURVE('',#21510,#21511,#4713,.T.);
#25775=EDGE_CURVE('',#21511,#21511,#18303,.T.);
#25776=EDGE_CURVE('',#21512,#21512,#18304,.T.);
#25777=EDGE_CURVE('',#21512,#21513,#4714,.T.);
#25778=EDGE_CURVE('',#21514,#21513,#2076,.F.);
#25779=EDGE_CURVE('',#21514,#21515,#18305,.T.);
#25780=EDGE_CURVE('',#21513,#21515,#2077,.F.);
#25781=EDGE_CURVE('',#21516,#21516,#18306,.T.);
#25782=EDGE_CURVE('',#21516,#21517,#4715,.T.);
#25783=EDGE_CURVE('',#21517,#21517,#18307,.T.);
#25784=EDGE_CURVE('',#21518,#21518,#18308,.T.);
#25785=EDGE_CURVE('',#21518,#21519,#4716,.T.);
#25786=EDGE_CURVE('',#21519,#21519,#18309,.T.);
#25787=EDGE_CURVE('',#21520,#21520,#18310,.T.);
#25788=EDGE_CURVE('',#21520,#21521,#4717,.T.);
#25789=EDGE_CURVE('',#21521,#21521,#18311,.T.);
#25790=EDGE_CURVE('',#21522,#21522,#18312,.T.);
#25791=EDGE_CURVE('',#21522,#21523,#4718,.T.);
#25792=EDGE_CURVE('',#21523,#21523,#18313,.T.);
#25793=EDGE_CURVE('',#21524,#21524,#18314,.T.);
#25794=EDGE_CURVE('',#21524,#21525,#4719,.T.);
#25795=EDGE_CURVE('',#21525,#21525,#18315,.T.);
#25796=EDGE_CURVE('',#21526,#21526,#18316,.T.);
#25797=EDGE_CURVE('',#21526,#21527,#4720,.T.);
#25798=EDGE_CURVE('',#21527,#21527,#18317,.T.);
#25799=EDGE_CURVE('',#21528,#21528,#18318,.T.);
#25800=EDGE_CURVE('',#21528,#21529,#4721,.T.);
#25801=EDGE_CURVE('',#21529,#21529,#18319,.T.);
#25802=EDGE_CURVE('',#21530,#21530,#18320,.T.);
#25803=EDGE_CURVE('',#21530,#21531,#4722,.T.);
#25804=EDGE_CURVE('',#21531,#21531,#18321,.T.);
#25805=EDGE_CURVE('',#21532,#21532,#18322,.T.);
#25806=EDGE_CURVE('',#21532,#21533,#4723,.T.);
#25807=EDGE_CURVE('',#21533,#21533,#18323,.T.);
#25808=EDGE_CURVE('',#21534,#21534,#18324,.T.);
#25809=EDGE_CURVE('',#21534,#21535,#4724,.T.);
#25810=EDGE_CURVE('',#21535,#21535,#18325,.T.);
#25811=EDGE_CURVE('',#21536,#21536,#18326,.T.);
#25812=EDGE_CURVE('',#21536,#21537,#4725,.T.);
#25813=EDGE_CURVE('',#21537,#21537,#18327,.T.);
#25814=EDGE_CURVE('',#21538,#21538,#18328,.T.);
#25815=EDGE_CURVE('',#21538,#21539,#4726,.T.);
#25816=EDGE_CURVE('',#21539,#21539,#18329,.T.);
#25817=EDGE_CURVE('',#21540,#21540,#18330,.T.);
#25818=EDGE_CURVE('',#21540,#21541,#4727,.T.);
#25819=EDGE_CURVE('',#21541,#21541,#18331,.T.);
#25820=EDGE_CURVE('',#21542,#21542,#18332,.T.);
#25821=EDGE_CURVE('',#21542,#21543,#4728,.T.);
#25822=EDGE_CURVE('',#21543,#21543,#18333,.T.);
#25823=EDGE_CURVE('',#21544,#21544,#18334,.T.);
#25824=EDGE_CURVE('',#21544,#21545,#4729,.T.);
#25825=EDGE_CURVE('',#21545,#21545,#18335,.T.);
#25826=EDGE_CURVE('',#21546,#21546,#18336,.T.);
#25827=EDGE_CURVE('',#21546,#21547,#4730,.T.);
#25828=EDGE_CURVE('',#21547,#21547,#18337,.T.);
#25829=EDGE_CURVE('',#21548,#21548,#18338,.T.);
#25830=EDGE_CURVE('',#21548,#21549,#4731,.T.);
#25831=EDGE_CURVE('',#21549,#21549,#18339,.T.);
#25832=EDGE_CURVE('',#21550,#21550,#18340,.T.);
#25833=EDGE_CURVE('',#21550,#21551,#4732,.T.);
#25834=EDGE_CURVE('',#21552,#21551,#2078,.F.);
#25835=EDGE_CURVE('',#21552,#21553,#18341,.T.);
#25836=EDGE_CURVE('',#21551,#21553,#2079,.F.);
#25837=EDGE_CURVE('',#21554,#21554,#18342,.T.);
#25838=EDGE_CURVE('',#21554,#21555,#4733,.T.);
#25839=EDGE_CURVE('',#21555,#21555,#18343,.T.);
#25840=EDGE_CURVE('',#21556,#21556,#18344,.T.);
#25841=EDGE_CURVE('',#21556,#21557,#4734,.T.);
#25842=EDGE_CURVE('',#21557,#21557,#18345,.T.);
#25843=EDGE_CURVE('',#21558,#21558,#18346,.T.);
#25844=EDGE_CURVE('',#21558,#21559,#4735,.T.);
#25845=EDGE_CURVE('',#21559,#21559,#18347,.T.);
#25846=EDGE_CURVE('',#21560,#21560,#18348,.T.);
#25847=EDGE_CURVE('',#21560,#21561,#4736,.T.);
#25848=EDGE_CURVE('',#21561,#21561,#18349,.T.);
#25849=EDGE_CURVE('',#21562,#21562,#18350,.T.);
#25850=EDGE_CURVE('',#21562,#21563,#4737,.T.);
#25851=EDGE_CURVE('',#21563,#21563,#18351,.T.);
#25852=EDGE_CURVE('',#21564,#21564,#18352,.T.);
#25853=EDGE_CURVE('',#21564,#21565,#4738,.T.);
#25854=EDGE_CURVE('',#21565,#21565,#18353,.T.);
#25855=EDGE_CURVE('',#21566,#21566,#18354,.T.);
#25856=EDGE_CURVE('',#21566,#21567,#4739,.T.);
#25857=EDGE_CURVE('',#21567,#21567,#18355,.T.);
#25858=EDGE_CURVE('',#21568,#21568,#18356,.T.);
#25859=EDGE_CURVE('',#21568,#21569,#4740,.T.);
#25860=EDGE_CURVE('',#21569,#21569,#18357,.T.);
#25861=EDGE_CURVE('',#21570,#21570,#18358,.T.);
#25862=EDGE_CURVE('',#21570,#21571,#4741,.T.);
#25863=EDGE_CURVE('',#21571,#21571,#18359,.T.);
#25864=EDGE_CURVE('',#21572,#21572,#18360,.T.);
#25865=EDGE_CURVE('',#21572,#21573,#4742,.T.);
#25866=EDGE_CURVE('',#21573,#21573,#18361,.T.);
#25867=EDGE_CURVE('',#21574,#21574,#18362,.T.);
#25868=EDGE_CURVE('',#21574,#21575,#4743,.T.);
#25869=EDGE_CURVE('',#21575,#21575,#18363,.T.);
#25870=EDGE_CURVE('',#21576,#21576,#18364,.T.);
#25871=EDGE_CURVE('',#21576,#21577,#4744,.T.);
#25872=EDGE_CURVE('',#21577,#21577,#18365,.T.);
#25873=EDGE_CURVE('',#21578,#21578,#18366,.T.);
#25874=EDGE_CURVE('',#21578,#21579,#4745,.T.);
#25875=EDGE_CURVE('',#21579,#21579,#18367,.T.);
#25876=EDGE_CURVE('',#21580,#21580,#18368,.T.);
#25877=EDGE_CURVE('',#21580,#21581,#4746,.T.);
#25878=EDGE_CURVE('',#21581,#21581,#18369,.T.);
#25879=EDGE_CURVE('',#21582,#21582,#18370,.T.);
#25880=EDGE_CURVE('',#21582,#21583,#4747,.T.);
#25881=EDGE_CURVE('',#21583,#21583,#18371,.T.);
#25882=EDGE_CURVE('',#21584,#21584,#18372,.T.);
#25883=EDGE_CURVE('',#21584,#21585,#4748,.T.);
#25884=EDGE_CURVE('',#21585,#21585,#18373,.T.);
#25885=EDGE_CURVE('',#21586,#21586,#18374,.T.);
#25886=EDGE_CURVE('',#21586,#21587,#4749,.T.);
#25887=EDGE_CURVE('',#21587,#21587,#18375,.T.);
#25888=EDGE_CURVE('',#21588,#21588,#18376,.T.);
#25889=EDGE_CURVE('',#21588,#21589,#4750,.T.);
#25890=EDGE_CURVE('',#21590,#21589,#2080,.F.);
#25891=EDGE_CURVE('',#21590,#21591,#18377,.T.);
#25892=EDGE_CURVE('',#21589,#21591,#2081,.F.);
#25893=EDGE_CURVE('',#21592,#21592,#18378,.T.);
#25894=EDGE_CURVE('',#21592,#21593,#4751,.T.);
#25895=EDGE_CURVE('',#21593,#21593,#18379,.T.);
#25896=EDGE_CURVE('',#21594,#21594,#18380,.T.);
#25897=EDGE_CURVE('',#21594,#21595,#4752,.T.);
#25898=EDGE_CURVE('',#21595,#21595,#18381,.T.);
#25899=EDGE_CURVE('',#21596,#21596,#18382,.T.);
#25900=EDGE_CURVE('',#21596,#21597,#4753,.T.);
#25901=EDGE_CURVE('',#21597,#21597,#18383,.T.);
#25902=EDGE_CURVE('',#21598,#21598,#18384,.T.);
#25903=EDGE_CURVE('',#21598,#21599,#4754,.T.);
#25904=EDGE_CURVE('',#21599,#21599,#18385,.T.);
#25905=EDGE_CURVE('',#21600,#21600,#18386,.T.);
#25906=EDGE_CURVE('',#21600,#21601,#4755,.T.);
#25907=EDGE_CURVE('',#21601,#21601,#18387,.T.);
#25908=EDGE_CURVE('',#21602,#21602,#18388,.T.);
#25909=EDGE_CURVE('',#21602,#21603,#4756,.T.);
#25910=EDGE_CURVE('',#21603,#21603,#18389,.T.);
#25911=EDGE_CURVE('',#21604,#21604,#18390,.T.);
#25912=EDGE_CURVE('',#21604,#21605,#4757,.T.);
#25913=EDGE_CURVE('',#21605,#21605,#18391,.T.);
#25914=EDGE_CURVE('',#21606,#21606,#18392,.T.);
#25915=EDGE_CURVE('',#21606,#21607,#4758,.T.);
#25916=EDGE_CURVE('',#21607,#21607,#18393,.T.);
#25917=EDGE_CURVE('',#21608,#21608,#18394,.T.);
#25918=EDGE_CURVE('',#21608,#21609,#4759,.T.);
#25919=EDGE_CURVE('',#21609,#21609,#18395,.T.);
#25920=EDGE_CURVE('',#21610,#21610,#18396,.T.);
#25921=EDGE_CURVE('',#21610,#21611,#4760,.T.);
#25922=EDGE_CURVE('',#21611,#21611,#18397,.T.);
#25923=EDGE_CURVE('',#21612,#21612,#18398,.T.);
#25924=EDGE_CURVE('',#21612,#21613,#4761,.T.);
#25925=EDGE_CURVE('',#21613,#21613,#18399,.T.);
#25926=EDGE_CURVE('',#21614,#21614,#18400,.T.);
#25927=EDGE_CURVE('',#21614,#21615,#4762,.T.);
#25928=EDGE_CURVE('',#21615,#21615,#18401,.T.);
#25929=EDGE_CURVE('',#21616,#21616,#18402,.T.);
#25930=EDGE_CURVE('',#21616,#21617,#4763,.T.);
#25931=EDGE_CURVE('',#21617,#21617,#18403,.T.);
#25932=EDGE_CURVE('',#21618,#21618,#18404,.T.);
#25933=EDGE_CURVE('',#21618,#21619,#4764,.T.);
#25934=EDGE_CURVE('',#21619,#21619,#18405,.T.);
#25935=EDGE_CURVE('',#21620,#21620,#18406,.T.);
#25936=EDGE_CURVE('',#21620,#21621,#4765,.T.);
#25937=EDGE_CURVE('',#21621,#21621,#18407,.T.);
#25938=EDGE_CURVE('',#21622,#21622,#18408,.T.);
#25939=EDGE_CURVE('',#21622,#21623,#4766,.T.);
#25940=EDGE_CURVE('',#21623,#21623,#18409,.T.);
#25941=EDGE_CURVE('',#21624,#21624,#18410,.T.);
#25942=EDGE_CURVE('',#21624,#21625,#4767,.T.);
#25943=EDGE_CURVE('',#21625,#21625,#18411,.T.);
#25944=EDGE_CURVE('',#21626,#21626,#18412,.T.);
#25945=EDGE_CURVE('',#21626,#21627,#4768,.T.);
#25946=EDGE_CURVE('',#21628,#21627,#2082,.F.);
#25947=EDGE_CURVE('',#21628,#21629,#18413,.T.);
#25948=EDGE_CURVE('',#21627,#21629,#2083,.F.);
#25949=EDGE_CURVE('',#21630,#21630,#18414,.T.);
#25950=EDGE_CURVE('',#21630,#21631,#4769,.T.);
#25951=EDGE_CURVE('',#21631,#21631,#18415,.T.);
#25952=EDGE_CURVE('',#21632,#21632,#18416,.T.);
#25953=EDGE_CURVE('',#21632,#21633,#4770,.T.);
#25954=EDGE_CURVE('',#21633,#21633,#18417,.T.);
#25955=EDGE_CURVE('',#21634,#21634,#18418,.T.);
#25956=EDGE_CURVE('',#21634,#21635,#4771,.T.);
#25957=EDGE_CURVE('',#21635,#21635,#18419,.T.);
#25958=EDGE_CURVE('',#21636,#21636,#18420,.T.);
#25959=EDGE_CURVE('',#21636,#21637,#4772,.T.);
#25960=EDGE_CURVE('',#21637,#21637,#18421,.T.);
#25961=EDGE_CURVE('',#21638,#21638,#18422,.T.);
#25962=EDGE_CURVE('',#21638,#21639,#4773,.T.);
#25963=EDGE_CURVE('',#21639,#21639,#18423,.T.);
#25964=EDGE_CURVE('',#21640,#21640,#18424,.T.);
#25965=EDGE_CURVE('',#21640,#21641,#4774,.T.);
#25966=EDGE_CURVE('',#21641,#21641,#18425,.T.);
#25967=EDGE_CURVE('',#21642,#21642,#18426,.T.);
#25968=EDGE_CURVE('',#21642,#21643,#4775,.T.);
#25969=EDGE_CURVE('',#21643,#21643,#18427,.T.);
#25970=EDGE_CURVE('',#21644,#21644,#18428,.T.);
#25971=EDGE_CURVE('',#21644,#21645,#4776,.T.);
#25972=EDGE_CURVE('',#21645,#21645,#18429,.T.);
#25973=EDGE_CURVE('',#21646,#21646,#18430,.T.);
#25974=EDGE_CURVE('',#21646,#21647,#4777,.T.);
#25975=EDGE_CURVE('',#21647,#21647,#18431,.T.);
#25976=EDGE_CURVE('',#21648,#21648,#18432,.T.);
#25977=EDGE_CURVE('',#21648,#21649,#4778,.T.);
#25978=EDGE_CURVE('',#21649,#21649,#18433,.T.);
#25979=EDGE_CURVE('',#21650,#21650,#18434,.T.);
#25980=EDGE_CURVE('',#21650,#21651,#4779,.T.);
#25981=EDGE_CURVE('',#21651,#21651,#18435,.T.);
#25982=EDGE_CURVE('',#21652,#21652,#18436,.T.);
#25983=EDGE_CURVE('',#21652,#21653,#4780,.T.);
#25984=EDGE_CURVE('',#21653,#21653,#18437,.T.);
#25985=EDGE_CURVE('',#21654,#21654,#18438,.T.);
#25986=EDGE_CURVE('',#21654,#21655,#4781,.T.);
#25987=EDGE_CURVE('',#21655,#21655,#18439,.T.);
#25988=EDGE_CURVE('',#21656,#21656,#18440,.T.);
#25989=EDGE_CURVE('',#21656,#21657,#4782,.T.);
#25990=EDGE_CURVE('',#21657,#21657,#18441,.T.);
#25991=EDGE_CURVE('',#21658,#21658,#18442,.T.);
#25992=EDGE_CURVE('',#21658,#21659,#4783,.T.);
#25993=EDGE_CURVE('',#21659,#21659,#18443,.T.);
#25994=EDGE_CURVE('',#21660,#21660,#18444,.T.);
#25995=EDGE_CURVE('',#21660,#21661,#4784,.T.);
#25996=EDGE_CURVE('',#21662,#21661,#2084,.F.);
#25997=EDGE_CURVE('',#21662,#21663,#18445,.T.);
#25998=EDGE_CURVE('',#21661,#21663,#2085,.F.);
#25999=EDGE_CURVE('',#21664,#21664,#18446,.T.);
#26000=EDGE_CURVE('',#21664,#21665,#4785,.T.);
#26001=EDGE_CURVE('',#21665,#21665,#18447,.T.);
#26002=EDGE_CURVE('',#21666,#21666,#18448,.T.);
#26003=EDGE_CURVE('',#21666,#21667,#4786,.T.);
#26004=EDGE_CURVE('',#21667,#21667,#18449,.T.);
#26005=EDGE_CURVE('',#21668,#21668,#18450,.T.);
#26006=EDGE_CURVE('',#21668,#21669,#4787,.T.);
#26007=EDGE_CURVE('',#21669,#21669,#18451,.T.);
#26008=EDGE_CURVE('',#21670,#21670,#18452,.T.);
#26009=EDGE_CURVE('',#21670,#21671,#4788,.T.);
#26010=EDGE_CURVE('',#21671,#21671,#18453,.T.);
#26011=EDGE_CURVE('',#21672,#21672,#18454,.T.);
#26012=EDGE_CURVE('',#21672,#21673,#4789,.T.);
#26013=EDGE_CURVE('',#21673,#21673,#18455,.T.);
#26014=EDGE_CURVE('',#21674,#21674,#18456,.T.);
#26015=EDGE_CURVE('',#21674,#21675,#4790,.T.);
#26016=EDGE_CURVE('',#21675,#21675,#18457,.T.);
#26017=EDGE_CURVE('',#21676,#21676,#18458,.T.);
#26018=EDGE_CURVE('',#21676,#21677,#4791,.T.);
#26019=EDGE_CURVE('',#21677,#21677,#18459,.T.);
#26020=EDGE_CURVE('',#21678,#21678,#18460,.T.);
#26021=EDGE_CURVE('',#21678,#21679,#4792,.T.);
#26022=EDGE_CURVE('',#21679,#21679,#18461,.T.);
#26023=EDGE_CURVE('',#21680,#21680,#18462,.T.);
#26024=EDGE_CURVE('',#21680,#21681,#4793,.T.);
#26025=EDGE_CURVE('',#21681,#21681,#18463,.T.);
#26026=EDGE_CURVE('',#21682,#21682,#18464,.T.);
#26027=EDGE_CURVE('',#21682,#21683,#4794,.T.);
#26028=EDGE_CURVE('',#21683,#21683,#18465,.T.);
#26029=EDGE_CURVE('',#21684,#21684,#18466,.T.);
#26030=EDGE_CURVE('',#21684,#21685,#4795,.T.);
#26031=EDGE_CURVE('',#21685,#21685,#18467,.T.);
#26032=EDGE_CURVE('',#21686,#21686,#18468,.T.);
#26033=EDGE_CURVE('',#21686,#21687,#4796,.T.);
#26034=EDGE_CURVE('',#21687,#21687,#18469,.T.);
#26035=EDGE_CURVE('',#21688,#21688,#18470,.T.);
#26036=EDGE_CURVE('',#21688,#21689,#4797,.T.);
#26037=EDGE_CURVE('',#21689,#21689,#18471,.T.);
#26038=EDGE_CURVE('',#21690,#21690,#18472,.T.);
#26039=EDGE_CURVE('',#21690,#21691,#4798,.T.);
#26040=EDGE_CURVE('',#21691,#21691,#18473,.T.);
#26041=EDGE_CURVE('',#21692,#21692,#18474,.T.);
#26042=EDGE_CURVE('',#21692,#21693,#4799,.T.);
#26043=EDGE_CURVE('',#21693,#21693,#18475,.T.);
#26044=EDGE_CURVE('',#21694,#21694,#18476,.T.);
#26045=EDGE_CURVE('',#21694,#21695,#4800,.T.);
#26046=EDGE_CURVE('',#21695,#21695,#18477,.T.);
#26047=EDGE_CURVE('',#21696,#21696,#18478,.T.);
#26048=EDGE_CURVE('',#21696,#21697,#4801,.T.);
#26049=EDGE_CURVE('',#21697,#21697,#18479,.T.);
#26050=EDGE_CURVE('',#21698,#21698,#18480,.T.);
#26051=EDGE_CURVE('',#21698,#21699,#4802,.T.);
#26052=EDGE_CURVE('',#21699,#21700,#18481,.T.);
#26053=EDGE_CURVE('',#21701,#21700,#2086,.T.);
#26054=EDGE_CURVE('',#21701,#21699,#18482,.T.);
#26055=EDGE_CURVE('',#21702,#21702,#18483,.T.);
#26056=EDGE_CURVE('',#21702,#21703,#4803,.T.);
#26057=EDGE_CURVE('',#21703,#21703,#18484,.T.);
#26058=EDGE_CURVE('',#21704,#21704,#18485,.T.);
#26059=EDGE_CURVE('',#21704,#21705,#4804,.T.);
#26060=EDGE_CURVE('',#21705,#21705,#18486,.T.);
#26061=EDGE_CURVE('',#21706,#21706,#18487,.T.);
#26062=EDGE_CURVE('',#21706,#21707,#4805,.T.);
#26063=EDGE_CURVE('',#21707,#21707,#18488,.T.);
#26064=EDGE_CURVE('',#21708,#21708,#18489,.T.);
#26065=EDGE_CURVE('',#21708,#21709,#4806,.T.);
#26066=EDGE_CURVE('',#21709,#21709,#18490,.T.);
#26067=EDGE_CURVE('',#21710,#21710,#18491,.T.);
#26068=EDGE_CURVE('',#21710,#21711,#4807,.T.);
#26069=EDGE_CURVE('',#21711,#21711,#18492,.T.);
#26070=EDGE_CURVE('',#21712,#21712,#18493,.T.);
#26071=EDGE_CURVE('',#21712,#21713,#4808,.T.);
#26072=EDGE_CURVE('',#21713,#21713,#18494,.T.);
#26073=EDGE_CURVE('',#21714,#21714,#18495,.T.);
#26074=EDGE_CURVE('',#21714,#21715,#4809,.T.);
#26075=EDGE_CURVE('',#21715,#21715,#18496,.T.);
#26076=EDGE_CURVE('',#21716,#21716,#18497,.T.);
#26077=EDGE_CURVE('',#21716,#21717,#4810,.T.);
#26078=EDGE_CURVE('',#21717,#21717,#18498,.T.);
#26079=EDGE_CURVE('',#21718,#21718,#18499,.T.);
#26080=EDGE_CURVE('',#21718,#21719,#4811,.T.);
#26081=EDGE_CURVE('',#21719,#21719,#18500,.T.);
#26082=EDGE_CURVE('',#21720,#21720,#18501,.T.);
#26083=EDGE_CURVE('',#21720,#21721,#4812,.T.);
#26084=EDGE_CURVE('',#21721,#21721,#18502,.T.);
#26085=EDGE_CURVE('',#21722,#21722,#18503,.T.);
#26086=EDGE_CURVE('',#21722,#21723,#4813,.T.);
#26087=EDGE_CURVE('',#21723,#21723,#18504,.T.);
#26088=EDGE_CURVE('',#21724,#21724,#18505,.T.);
#26089=EDGE_CURVE('',#21724,#21725,#4814,.T.);
#26090=EDGE_CURVE('',#21725,#21725,#18506,.T.);
#26091=EDGE_CURVE('',#21726,#21726,#18507,.T.);
#26092=EDGE_CURVE('',#21726,#21727,#4815,.T.);
#26093=EDGE_CURVE('',#21727,#21727,#18508,.T.);
#26094=EDGE_CURVE('',#21728,#21728,#18509,.T.);
#26095=EDGE_CURVE('',#21728,#21729,#4816,.T.);
#26096=EDGE_CURVE('',#21729,#21729,#18510,.T.);
#26097=EDGE_CURVE('',#21730,#21730,#18511,.T.);
#26098=EDGE_CURVE('',#21730,#21731,#4817,.T.);
#26099=EDGE_CURVE('',#21731,#21731,#18512,.T.);
#26100=EDGE_CURVE('',#21732,#21732,#18513,.T.);
#26101=EDGE_CURVE('',#21732,#21733,#4818,.T.);
#26102=EDGE_CURVE('',#21733,#21734,#18514,.T.);
#26103=EDGE_CURVE('',#21735,#21734,#2087,.T.);
#26104=EDGE_CURVE('',#21735,#21733,#18515,.T.);
#26105=EDGE_CURVE('',#21736,#21736,#18516,.T.);
#26106=EDGE_CURVE('',#21736,#21737,#4819,.T.);
#26107=EDGE_CURVE('',#21737,#21737,#18517,.T.);
#26108=EDGE_CURVE('',#21738,#21738,#18518,.T.);
#26109=EDGE_CURVE('',#21738,#21739,#4820,.T.);
#26110=EDGE_CURVE('',#21739,#21740,#18519,.T.);
#26111=EDGE_CURVE('',#21741,#21740,#2088,.T.);
#26112=EDGE_CURVE('',#21741,#21739,#18520,.T.);
#26113=EDGE_CURVE('',#21742,#21742,#18521,.T.);
#26114=EDGE_CURVE('',#21742,#21743,#4821,.T.);
#26115=EDGE_CURVE('',#21743,#21743,#18522,.T.);
#26116=EDGE_CURVE('',#21744,#21744,#18523,.T.);
#26117=EDGE_CURVE('',#21744,#21745,#4822,.T.);
#26118=EDGE_CURVE('',#21745,#21745,#18524,.T.);
#26119=EDGE_CURVE('',#21746,#21746,#18525,.T.);
#26120=EDGE_CURVE('',#21746,#21747,#4823,.T.);
#26121=EDGE_CURVE('',#21747,#21747,#18526,.T.);
#26122=EDGE_CURVE('',#21748,#21748,#18527,.T.);
#26123=EDGE_CURVE('',#21748,#21749,#4824,.T.);
#26124=EDGE_CURVE('',#21749,#21749,#18528,.T.);
#26125=EDGE_CURVE('',#21750,#21750,#18529,.T.);
#26126=EDGE_CURVE('',#21750,#21751,#4825,.T.);
#26127=EDGE_CURVE('',#21751,#21751,#18530,.T.);
#26128=EDGE_CURVE('',#21752,#21752,#18531,.T.);
#26129=EDGE_CURVE('',#21752,#21753,#4826,.T.);
#26130=EDGE_CURVE('',#21753,#21753,#18532,.T.);
#26131=EDGE_CURVE('',#21754,#21754,#18533,.T.);
#26132=EDGE_CURVE('',#21754,#21755,#4827,.T.);
#26133=EDGE_CURVE('',#21755,#21755,#18534,.T.);
#26134=EDGE_CURVE('',#21756,#21756,#18535,.T.);
#26135=EDGE_CURVE('',#21756,#21757,#4828,.T.);
#26136=EDGE_CURVE('',#21757,#21757,#18536,.T.);
#26137=EDGE_CURVE('',#21758,#21758,#18537,.T.);
#26138=EDGE_CURVE('',#21758,#21759,#4829,.T.);
#26139=EDGE_CURVE('',#21759,#21759,#18538,.T.);
#26140=EDGE_CURVE('',#21760,#21760,#18539,.T.);
#26141=EDGE_CURVE('',#21760,#21761,#4830,.T.);
#26142=EDGE_CURVE('',#21761,#21761,#18540,.T.);
#26143=EDGE_CURVE('',#21762,#21762,#18541,.T.);
#26144=EDGE_CURVE('',#21762,#21763,#4831,.T.);
#26145=EDGE_CURVE('',#21763,#21763,#18542,.T.);
#26146=EDGE_CURVE('',#21764,#21764,#18543,.T.);
#26147=EDGE_CURVE('',#21764,#21765,#4832,.T.);
#26148=EDGE_CURVE('',#21765,#21765,#18544,.T.);
#26149=EDGE_CURVE('',#21766,#21766,#18545,.T.);
#26150=EDGE_CURVE('',#21766,#21767,#4833,.T.);
#26151=EDGE_CURVE('',#21767,#21767,#18546,.T.);
#26152=EDGE_CURVE('',#21768,#21768,#18547,.T.);
#26153=EDGE_CURVE('',#21768,#21769,#4834,.T.);
#26154=EDGE_CURVE('',#21769,#21770,#18548,.T.);
#26155=EDGE_CURVE('',#21771,#21770,#2089,.T.);
#26156=EDGE_CURVE('',#21771,#21769,#18549,.T.);
#26157=EDGE_CURVE('',#21772,#21772,#18550,.T.);
#26158=EDGE_CURVE('',#21772,#21773,#4835,.T.);
#26159=EDGE_CURVE('',#21773,#21773,#18551,.T.);
#26160=EDGE_CURVE('',#21774,#21774,#18552,.T.);
#26161=EDGE_CURVE('',#21774,#21775,#4836,.T.);
#26162=EDGE_CURVE('',#21775,#21775,#18553,.T.);
#26163=EDGE_CURVE('',#21776,#21776,#18554,.T.);
#26164=EDGE_CURVE('',#21776,#21777,#4837,.T.);
#26165=EDGE_CURVE('',#21777,#21777,#18555,.T.);
#26166=EDGE_CURVE('',#21778,#21778,#18556,.T.);
#26167=EDGE_CURVE('',#21778,#21779,#4838,.T.);
#26168=EDGE_CURVE('',#21779,#21779,#18557,.T.);
#26169=EDGE_CURVE('',#21780,#21780,#18558,.T.);
#26170=EDGE_CURVE('',#21780,#21781,#4839,.T.);
#26171=EDGE_CURVE('',#21781,#21781,#18559,.T.);
#26172=EDGE_CURVE('',#21782,#21782,#18560,.T.);
#26173=EDGE_CURVE('',#21782,#21783,#4840,.T.);
#26174=EDGE_CURVE('',#21783,#21783,#18561,.T.);
#26175=EDGE_CURVE('',#21784,#21784,#18562,.T.);
#26176=EDGE_CURVE('',#21784,#21785,#4841,.T.);
#26177=EDGE_CURVE('',#21785,#21785,#18563,.T.);
#26178=EDGE_CURVE('',#21786,#21786,#18564,.T.);
#26179=EDGE_CURVE('',#21786,#21787,#4842,.T.);
#26180=EDGE_CURVE('',#21787,#21787,#18565,.T.);
#26181=EDGE_CURVE('',#21788,#21788,#18566,.T.);
#26182=EDGE_CURVE('',#21788,#21789,#4843,.T.);
#26183=EDGE_CURVE('',#21789,#21789,#18567,.T.);
#26184=EDGE_CURVE('',#21790,#21790,#18568,.T.);
#26185=EDGE_CURVE('',#21790,#21791,#4844,.T.);
#26186=EDGE_CURVE('',#21791,#21791,#18569,.T.);
#26187=EDGE_CURVE('',#21792,#21792,#18570,.T.);
#26188=EDGE_CURVE('',#21792,#21793,#4845,.T.);
#26189=EDGE_CURVE('',#21793,#21793,#18571,.T.);
#26190=EDGE_CURVE('',#21794,#21794,#18572,.T.);
#26191=EDGE_CURVE('',#21794,#21795,#4846,.T.);
#26192=EDGE_CURVE('',#21795,#21795,#18573,.T.);
#26193=EDGE_CURVE('',#21796,#21796,#18574,.T.);
#26194=EDGE_CURVE('',#21796,#21797,#4847,.T.);
#26195=EDGE_CURVE('',#21797,#21797,#18575,.T.);
#26196=EDGE_CURVE('',#21798,#21798,#18576,.T.);
#26197=EDGE_CURVE('',#21798,#21799,#4848,.T.);
#26198=EDGE_CURVE('',#21799,#21799,#18577,.T.);
#26199=EDGE_CURVE('',#21800,#21800,#18578,.T.);
#26200=EDGE_CURVE('',#21800,#21801,#4849,.T.);
#26201=EDGE_CURVE('',#21801,#21801,#18579,.T.);
#26202=EDGE_CURVE('',#21802,#21802,#18580,.T.);
#26203=EDGE_CURVE('',#21802,#21803,#4850,.T.);
#26204=EDGE_CURVE('',#21803,#21803,#18581,.T.);
#26205=EDGE_CURVE('',#21804,#21804,#18582,.T.);
#26206=EDGE_CURVE('',#21804,#21805,#4851,.T.);
#26207=EDGE_CURVE('',#21805,#21805,#18583,.T.);
#26208=EDGE_CURVE('',#21806,#21806,#18584,.T.);
#26209=EDGE_CURVE('',#21806,#21807,#4852,.T.);
#26210=EDGE_CURVE('',#21807,#21807,#18585,.T.);
#26211=EDGE_CURVE('',#21808,#21808,#18586,.T.);
#26212=EDGE_CURVE('',#21808,#21809,#4853,.T.);
#26213=EDGE_CURVE('',#21809,#21809,#18587,.T.);
#26214=EDGE_CURVE('',#21810,#21810,#18588,.T.);
#26215=EDGE_CURVE('',#21810,#21811,#4854,.T.);
#26216=EDGE_CURVE('',#21811,#21811,#18589,.T.);
#26217=EDGE_CURVE('',#21812,#21812,#18590,.T.);
#26218=EDGE_CURVE('',#21812,#21813,#4855,.T.);
#26219=EDGE_CURVE('',#21813,#21813,#18591,.T.);
#26220=EDGE_CURVE('',#21814,#21814,#18592,.T.);
#26221=EDGE_CURVE('',#21814,#21815,#4856,.T.);
#26222=EDGE_CURVE('',#21815,#21815,#18593,.T.);
#26223=EDGE_CURVE('',#21816,#21816,#18594,.T.);
#26224=EDGE_CURVE('',#21816,#21817,#4857,.T.);
#26225=EDGE_CURVE('',#21817,#21817,#18595,.T.);
#26226=EDGE_CURVE('',#21818,#21818,#18596,.T.);
#26227=EDGE_CURVE('',#21818,#21819,#4858,.T.);
#26228=EDGE_CURVE('',#21819,#21819,#18597,.T.);
#26229=EDGE_CURVE('',#21820,#21820,#18598,.T.);
#26230=EDGE_CURVE('',#21820,#21821,#4859,.T.);
#26231=EDGE_CURVE('',#21821,#21821,#18599,.T.);
#26232=EDGE_CURVE('',#21822,#21822,#18600,.T.);
#26233=EDGE_CURVE('',#21822,#21823,#4860,.T.);
#26234=EDGE_CURVE('',#21823,#21823,#18601,.T.);
#26235=EDGE_CURVE('',#21824,#21824,#18602,.T.);
#26236=EDGE_CURVE('',#21824,#21825,#4861,.T.);
#26237=EDGE_CURVE('',#21825,#21825,#18603,.T.);
#26238=EDGE_CURVE('',#21826,#21826,#18604,.T.);
#26239=EDGE_CURVE('',#21826,#21827,#4862,.T.);
#26240=EDGE_CURVE('',#21827,#21828,#18605,.T.);
#26241=EDGE_CURVE('',#21829,#21828,#2090,.T.);
#26242=EDGE_CURVE('',#21829,#21827,#18606,.T.);
#26243=EDGE_CURVE('',#21830,#21830,#18607,.T.);
#26244=EDGE_CURVE('',#21830,#21831,#4863,.T.);
#26245=EDGE_CURVE('',#21831,#21831,#18608,.T.);
#26246=EDGE_CURVE('',#21832,#21832,#18609,.T.);
#26247=EDGE_CURVE('',#21832,#21833,#4864,.T.);
#26248=EDGE_CURVE('',#21833,#21833,#18610,.T.);
#26249=EDGE_CURVE('',#21834,#21834,#18611,.T.);
#26250=EDGE_CURVE('',#21834,#21835,#4865,.T.);
#26251=EDGE_CURVE('',#21835,#21835,#18612,.T.);
#26252=EDGE_CURVE('',#21836,#21836,#18613,.T.);
#26253=EDGE_CURVE('',#21836,#21837,#4866,.T.);
#26254=EDGE_CURVE('',#21837,#21837,#18614,.T.);
#26255=EDGE_CURVE('',#21838,#21838,#18615,.T.);
#26256=EDGE_CURVE('',#21838,#21839,#4867,.T.);
#26257=EDGE_CURVE('',#21839,#21839,#18616,.T.);
#26258=EDGE_CURVE('',#21840,#21840,#18617,.T.);
#26259=EDGE_CURVE('',#21840,#21841,#4868,.T.);
#26260=EDGE_CURVE('',#21841,#21841,#18618,.T.);
#26261=EDGE_CURVE('',#21842,#21842,#18619,.T.);
#26262=EDGE_CURVE('',#21842,#21843,#4869,.T.);
#26263=EDGE_CURVE('',#21843,#21843,#18620,.T.);
#26264=EDGE_CURVE('',#21844,#21844,#18621,.T.);
#26265=EDGE_CURVE('',#21844,#21845,#4870,.T.);
#26266=EDGE_CURVE('',#21845,#21845,#18622,.T.);
#26267=EDGE_CURVE('',#21846,#21846,#18623,.T.);
#26268=EDGE_CURVE('',#21846,#21847,#4871,.T.);
#26269=EDGE_CURVE('',#21847,#21847,#18624,.T.);
#26270=EDGE_CURVE('',#21848,#21848,#18625,.T.);
#26271=EDGE_CURVE('',#21848,#21849,#4872,.T.);
#26272=EDGE_CURVE('',#21849,#21849,#18626,.T.);
#26273=EDGE_CURVE('',#21850,#21850,#18627,.T.);
#26274=EDGE_CURVE('',#21850,#21851,#4873,.T.);
#26275=EDGE_CURVE('',#21851,#21851,#18628,.T.);
#26276=EDGE_CURVE('',#21852,#21852,#18629,.T.);
#26277=EDGE_CURVE('',#21852,#21853,#4874,.T.);
#26278=EDGE_CURVE('',#21853,#21853,#18630,.T.);
#26279=EDGE_CURVE('',#21854,#21854,#18631,.T.);
#26280=EDGE_CURVE('',#21854,#21855,#4875,.T.);
#26281=EDGE_CURVE('',#21855,#21855,#18632,.T.);
#26282=EDGE_CURVE('',#21856,#21856,#18633,.T.);
#26283=EDGE_CURVE('',#21856,#21857,#4876,.T.);
#26284=EDGE_CURVE('',#21857,#21857,#18634,.T.);
#26285=EDGE_CURVE('',#21858,#21858,#18635,.T.);
#26286=EDGE_CURVE('',#21858,#21859,#4877,.T.);
#26287=EDGE_CURVE('',#21859,#21859,#18636,.T.);
#26288=EDGE_CURVE('',#21860,#21860,#18637,.T.);
#26289=EDGE_CURVE('',#21860,#21861,#4878,.T.);
#26290=EDGE_CURVE('',#21861,#21861,#18638,.T.);
#26291=EDGE_CURVE('',#21862,#21862,#18639,.T.);
#26292=EDGE_CURVE('',#21862,#21863,#4879,.T.);
#26293=EDGE_CURVE('',#21863,#21863,#18640,.T.);
#26294=EDGE_CURVE('',#21864,#21864,#18641,.T.);
#26295=EDGE_CURVE('',#21864,#21865,#4880,.T.);
#26296=EDGE_CURVE('',#21865,#21865,#18642,.T.);
#26297=EDGE_CURVE('',#21866,#21866,#18643,.T.);
#26298=EDGE_CURVE('',#21866,#21867,#4881,.T.);
#26299=EDGE_CURVE('',#21867,#21867,#18644,.T.);
#26300=EDGE_CURVE('',#21868,#21868,#18645,.T.);
#26301=EDGE_CURVE('',#21868,#21869,#4882,.T.);
#26302=EDGE_CURVE('',#21869,#21869,#18646,.T.);
#26303=EDGE_CURVE('',#21870,#21870,#18647,.T.);
#26304=EDGE_CURVE('',#21870,#21871,#4883,.T.);
#26305=EDGE_CURVE('',#21871,#21871,#18648,.T.);
#26306=EDGE_CURVE('',#21872,#21872,#18649,.T.);
#26307=EDGE_CURVE('',#21872,#21873,#4884,.T.);
#26308=EDGE_CURVE('',#21873,#21873,#18650,.T.);
#26309=EDGE_CURVE('',#21874,#21874,#18651,.T.);
#26310=EDGE_CURVE('',#21874,#21875,#4885,.T.);
#26311=EDGE_CURVE('',#21875,#21875,#18652,.T.);
#26312=EDGE_CURVE('',#21876,#21876,#18653,.T.);
#26313=EDGE_CURVE('',#21876,#21877,#4886,.T.);
#26314=EDGE_CURVE('',#21877,#21877,#18654,.T.);
#26315=EDGE_CURVE('',#21878,#21878,#18655,.T.);
#26316=EDGE_CURVE('',#21878,#21879,#4887,.T.);
#26317=EDGE_CURVE('',#21879,#21879,#18656,.T.);
#26318=EDGE_CURVE('',#21880,#21880,#18657,.T.);
#26319=EDGE_CURVE('',#21880,#21881,#4888,.T.);
#26320=EDGE_CURVE('',#21881,#21881,#18658,.T.);
#26321=EDGE_CURVE('',#21882,#21882,#18659,.T.);
#26322=EDGE_CURVE('',#21882,#21883,#4889,.T.);
#26323=EDGE_CURVE('',#21883,#21883,#18660,.T.);
#26324=EDGE_CURVE('',#21884,#21884,#18661,.T.);
#26325=EDGE_CURVE('',#21884,#21885,#4890,.T.);
#26326=EDGE_CURVE('',#21885,#21885,#18662,.T.);
#26327=EDGE_CURVE('',#21886,#21886,#18663,.T.);
#26328=EDGE_CURVE('',#21886,#21887,#4891,.T.);
#26329=EDGE_CURVE('',#21887,#21887,#18664,.T.);
#26330=EDGE_CURVE('',#21888,#21888,#18665,.T.);
#26331=EDGE_CURVE('',#21888,#21889,#4892,.T.);
#26332=EDGE_CURVE('',#21889,#21889,#18666,.T.);
#26333=EDGE_CURVE('',#21890,#21890,#18667,.T.);
#26334=EDGE_CURVE('',#21890,#21891,#4893,.T.);
#26335=EDGE_CURVE('',#21891,#21891,#18668,.T.);
#26336=EDGE_CURVE('',#21892,#21892,#18669,.T.);
#26337=EDGE_CURVE('',#21892,#21893,#4894,.T.);
#26338=EDGE_CURVE('',#21893,#21893,#18670,.T.);
#26339=EDGE_CURVE('',#21894,#21894,#18671,.T.);
#26340=EDGE_CURVE('',#21894,#21895,#4895,.T.);
#26341=EDGE_CURVE('',#21895,#21895,#18672,.T.);
#26342=EDGE_CURVE('',#21896,#21896,#18673,.T.);
#26343=EDGE_CURVE('',#21896,#21897,#4896,.T.);
#26344=EDGE_CURVE('',#21897,#21898,#18674,.T.);
#26345=EDGE_CURVE('',#21899,#21898,#2091,.T.);
#26346=EDGE_CURVE('',#21900,#21899,#2092,.T.);
#26347=EDGE_CURVE('',#21900,#21897,#18675,.T.);
#26348=EDGE_CURVE('',#21901,#21901,#18676,.T.);
#26349=EDGE_CURVE('',#21901,#21902,#4897,.T.);
#26350=EDGE_CURVE('',#21902,#21902,#18677,.T.);
#26351=EDGE_CURVE('',#21903,#21903,#18678,.T.);
#26352=EDGE_CURVE('',#21903,#21904,#4898,.T.);
#26353=EDGE_CURVE('',#21904,#21904,#18679,.T.);
#26354=EDGE_CURVE('',#21905,#21905,#18680,.T.);
#26355=EDGE_CURVE('',#21905,#21906,#4899,.T.);
#26356=EDGE_CURVE('',#21906,#21906,#18681,.T.);
#26357=EDGE_CURVE('',#21907,#21907,#18682,.T.);
#26358=EDGE_CURVE('',#21907,#21908,#4900,.T.);
#26359=EDGE_CURVE('',#21908,#21908,#18683,.T.);
#26360=EDGE_CURVE('',#21909,#21909,#18684,.T.);
#26361=EDGE_CURVE('',#21909,#21910,#4901,.T.);
#26362=EDGE_CURVE('',#21910,#21910,#18685,.T.);
#26363=EDGE_CURVE('',#21911,#21911,#18686,.T.);
#26364=EDGE_CURVE('',#21911,#21912,#4902,.T.);
#26365=EDGE_CURVE('',#21912,#21912,#18687,.T.);
#26366=EDGE_CURVE('',#21913,#21913,#18688,.T.);
#26367=EDGE_CURVE('',#21913,#21914,#4903,.T.);
#26368=EDGE_CURVE('',#21914,#21914,#18689,.T.);
#26369=EDGE_CURVE('',#21915,#21915,#18690,.T.);
#26370=EDGE_CURVE('',#21915,#21916,#4904,.T.);
#26371=EDGE_CURVE('',#21916,#21916,#18691,.T.);
#26372=EDGE_CURVE('',#21917,#21917,#18692,.T.);
#26373=EDGE_CURVE('',#21917,#21918,#4905,.T.);
#26374=EDGE_CURVE('',#21918,#21918,#18693,.T.);
#26375=EDGE_CURVE('',#21919,#21919,#18694,.T.);
#26376=EDGE_CURVE('',#21919,#21920,#4906,.T.);
#26377=EDGE_CURVE('',#21920,#21920,#18695,.T.);
#26378=EDGE_CURVE('',#21921,#21921,#18696,.T.);
#26379=EDGE_CURVE('',#21921,#21922,#4907,.T.);
#26380=EDGE_CURVE('',#21922,#21922,#18697,.T.);
#26381=EDGE_CURVE('',#21923,#21923,#18698,.T.);
#26382=EDGE_CURVE('',#21923,#21924,#4908,.T.);
#26383=EDGE_CURVE('',#21924,#21924,#18699,.T.);
#26384=EDGE_CURVE('',#21925,#21925,#18700,.T.);
#26385=EDGE_CURVE('',#21925,#21926,#4909,.T.);
#26386=EDGE_CURVE('',#21926,#21926,#18701,.T.);
#26387=EDGE_CURVE('',#21927,#21927,#18702,.T.);
#26388=EDGE_CURVE('',#21927,#21928,#4910,.T.);
#26389=EDGE_CURVE('',#21928,#21928,#18703,.T.);
#26390=EDGE_CURVE('',#21929,#21929,#18704,.T.);
#26391=EDGE_CURVE('',#21929,#21930,#4911,.T.);
#26392=EDGE_CURVE('',#21930,#21930,#18705,.T.);
#26393=EDGE_CURVE('',#21931,#21931,#18706,.T.);
#26394=EDGE_CURVE('',#21931,#21932,#4912,.T.);
#26395=EDGE_CURVE('',#21932,#21932,#18707,.T.);
#26396=EDGE_CURVE('',#21933,#21933,#18708,.T.);
#26397=EDGE_CURVE('',#21933,#21934,#4913,.T.);
#26398=EDGE_CURVE('',#21934,#21934,#18709,.T.);
#26399=EDGE_CURVE('',#21935,#21935,#18710,.T.);
#26400=EDGE_CURVE('',#21935,#21936,#4914,.T.);
#26401=EDGE_CURVE('',#21936,#21937,#18711,.T.);
#26402=EDGE_CURVE('',#21938,#21937,#2093,.T.);
#26403=EDGE_CURVE('',#21938,#21936,#18712,.T.);
#26404=EDGE_CURVE('',#21939,#21939,#18713,.T.);
#26405=EDGE_CURVE('',#21939,#21940,#4915,.T.);
#26406=EDGE_CURVE('',#21940,#21940,#18714,.T.);
#26407=EDGE_CURVE('',#21941,#21941,#18715,.T.);
#26408=EDGE_CURVE('',#21941,#21942,#4916,.T.);
#26409=EDGE_CURVE('',#21942,#21942,#18716,.T.);
#26410=EDGE_CURVE('',#21943,#21943,#18717,.T.);
#26411=EDGE_CURVE('',#21943,#21944,#4917,.T.);
#26412=EDGE_CURVE('',#21944,#21944,#18718,.T.);
#26413=EDGE_CURVE('',#21945,#21945,#18719,.T.);
#26414=EDGE_CURVE('',#21945,#21946,#4918,.T.);
#26415=EDGE_CURVE('',#21946,#21946,#18720,.T.);
#26416=EDGE_CURVE('',#21947,#21947,#18721,.T.);
#26417=EDGE_CURVE('',#21947,#21948,#4919,.T.);
#26418=EDGE_CURVE('',#21948,#21948,#18722,.T.);
#26419=EDGE_CURVE('',#21949,#21949,#18723,.T.);
#26420=EDGE_CURVE('',#21949,#21950,#4920,.T.);
#26421=EDGE_CURVE('',#21950,#21950,#18724,.T.);
#26422=EDGE_CURVE('',#21951,#21951,#18725,.T.);
#26423=EDGE_CURVE('',#21951,#21952,#4921,.T.);
#26424=EDGE_CURVE('',#21952,#21952,#18726,.T.);
#26425=EDGE_CURVE('',#21953,#21953,#18727,.T.);
#26426=EDGE_CURVE('',#21953,#21954,#4922,.T.);
#26427=EDGE_CURVE('',#21954,#21954,#18728,.T.);
#26428=EDGE_CURVE('',#21955,#21955,#18729,.T.);
#26429=EDGE_CURVE('',#21955,#21956,#4923,.T.);
#26430=EDGE_CURVE('',#21956,#21956,#18730,.T.);
#26431=EDGE_CURVE('',#21957,#21957,#18731,.T.);
#26432=EDGE_CURVE('',#21957,#21958,#4924,.T.);
#26433=EDGE_CURVE('',#21958,#21958,#18732,.T.);
#26434=EDGE_CURVE('',#21959,#21959,#18733,.T.);
#26435=EDGE_CURVE('',#21959,#21960,#4925,.T.);
#26436=EDGE_CURVE('',#21960,#21960,#18734,.T.);
#26437=EDGE_CURVE('',#21961,#21961,#18735,.T.);
#26438=EDGE_CURVE('',#21961,#21962,#4926,.T.);
#26439=EDGE_CURVE('',#21962,#21962,#18736,.T.);
#26440=EDGE_CURVE('',#21963,#21963,#18737,.T.);
#26441=EDGE_CURVE('',#21963,#21964,#4927,.T.);
#26442=EDGE_CURVE('',#21964,#21964,#18738,.T.);
#26443=EDGE_CURVE('',#21965,#21965,#18739,.T.);
#26444=EDGE_CURVE('',#21965,#21966,#4928,.T.);
#26445=EDGE_CURVE('',#21966,#21966,#18740,.T.);
#26446=EDGE_CURVE('',#21967,#21967,#18741,.T.);
#26447=EDGE_CURVE('',#21967,#21968,#4929,.T.);
#26448=EDGE_CURVE('',#21968,#21968,#18742,.T.);
#26449=EDGE_CURVE('',#21969,#21969,#18743,.T.);
#26450=EDGE_CURVE('',#21969,#21970,#4930,.T.);
#26451=EDGE_CURVE('',#21970,#21970,#18744,.T.);
#26452=EDGE_CURVE('',#21971,#21971,#18745,.T.);
#26453=EDGE_CURVE('',#21971,#21972,#4931,.T.);
#26454=EDGE_CURVE('',#21972,#21972,#18746,.T.);
#26455=EDGE_CURVE('',#21973,#21973,#18747,.T.);
#26456=EDGE_CURVE('',#21973,#21974,#4932,.T.);
#26457=EDGE_CURVE('',#21975,#21974,#2094,.F.);
#26458=EDGE_CURVE('',#21975,#21976,#18748,.T.);
#26459=EDGE_CURVE('',#21974,#21976,#2095,.F.);
#26460=EDGE_CURVE('',#21977,#21977,#18749,.T.);
#26461=EDGE_CURVE('',#21977,#21978,#4933,.T.);
#26462=EDGE_CURVE('',#21978,#21978,#18750,.T.);
#26463=EDGE_CURVE('',#21979,#21979,#18751,.T.);
#26464=EDGE_CURVE('',#21979,#21980,#4934,.T.);
#26465=EDGE_CURVE('',#21980,#21980,#18752,.T.);
#26466=EDGE_CURVE('',#21981,#21981,#18753,.T.);
#26467=EDGE_CURVE('',#21981,#21982,#4935,.T.);
#26468=EDGE_CURVE('',#21982,#21982,#18754,.T.);
#26469=EDGE_CURVE('',#21983,#21983,#18755,.T.);
#26470=EDGE_CURVE('',#21983,#21984,#4936,.T.);
#26471=EDGE_CURVE('',#21984,#21984,#18756,.T.);
#26472=EDGE_CURVE('',#21985,#21985,#18757,.T.);
#26473=EDGE_CURVE('',#21985,#21986,#4937,.T.);
#26474=EDGE_CURVE('',#21986,#21986,#18758,.T.);
#26475=EDGE_CURVE('',#21987,#21987,#18759,.T.);
#26476=EDGE_CURVE('',#21987,#21988,#4938,.T.);
#26477=EDGE_CURVE('',#21988,#21988,#18760,.T.);
#26478=EDGE_CURVE('',#21989,#21989,#18761,.T.);
#26479=EDGE_CURVE('',#21989,#21990,#4939,.T.);
#26480=EDGE_CURVE('',#21990,#21990,#18762,.T.);
#26481=EDGE_CURVE('',#21991,#21991,#18763,.T.);
#26482=EDGE_CURVE('',#21991,#21992,#4940,.T.);
#26483=EDGE_CURVE('',#21992,#21992,#18764,.T.);
#26484=EDGE_CURVE('',#21993,#21993,#18765,.T.);
#26485=EDGE_CURVE('',#21993,#21994,#4941,.T.);
#26486=EDGE_CURVE('',#21994,#21994,#18766,.T.);
#26487=EDGE_CURVE('',#21995,#21995,#18767,.T.);
#26488=EDGE_CURVE('',#21995,#21996,#4942,.T.);
#26489=EDGE_CURVE('',#21996,#21996,#18768,.T.);
#26490=EDGE_CURVE('',#21997,#21997,#18769,.T.);
#26491=EDGE_CURVE('',#21997,#21998,#4943,.T.);
#26492=EDGE_CURVE('',#21998,#21998,#18770,.T.);
#26493=EDGE_CURVE('',#21999,#21999,#18771,.T.);
#26494=EDGE_CURVE('',#21999,#22000,#4944,.T.);
#26495=EDGE_CURVE('',#22000,#22000,#18772,.T.);
#26496=EDGE_CURVE('',#22001,#22001,#18773,.T.);
#26497=EDGE_CURVE('',#22001,#22002,#4945,.T.);
#26498=EDGE_CURVE('',#22002,#22002,#18774,.T.);
#26499=EDGE_CURVE('',#22003,#22003,#18775,.T.);
#26500=EDGE_CURVE('',#22003,#22004,#4946,.T.);
#26501=EDGE_CURVE('',#22004,#22004,#18776,.T.);
#26502=EDGE_CURVE('',#22005,#22005,#18777,.T.);
#26503=EDGE_CURVE('',#22005,#22006,#4947,.T.);
#26504=EDGE_CURVE('',#22006,#22006,#18778,.T.);
#26505=EDGE_CURVE('',#22007,#22007,#18779,.T.);
#26506=EDGE_CURVE('',#22007,#22008,#4948,.T.);
#26507=EDGE_CURVE('',#22009,#22008,#2096,.F.);
#26508=EDGE_CURVE('',#22009,#22010,#18780,.T.);
#26509=EDGE_CURVE('',#22008,#22010,#2097,.F.);
#26510=EDGE_CURVE('',#22011,#22011,#18781,.T.);
#26511=EDGE_CURVE('',#22011,#22012,#4949,.T.);
#26512=EDGE_CURVE('',#22012,#22012,#18782,.T.);
#26513=EDGE_CURVE('',#22013,#22013,#18783,.T.);
#26514=EDGE_CURVE('',#22013,#22014,#4950,.T.);
#26515=EDGE_CURVE('',#22014,#22014,#18784,.T.);
#26516=EDGE_CURVE('',#22015,#22015,#18785,.T.);
#26517=EDGE_CURVE('',#22015,#22016,#4951,.T.);
#26518=EDGE_CURVE('',#22016,#22016,#18786,.T.);
#26519=EDGE_CURVE('',#22017,#22017,#18787,.T.);
#26520=EDGE_CURVE('',#22017,#22018,#4952,.T.);
#26521=EDGE_CURVE('',#22018,#22018,#18788,.T.);
#26522=EDGE_CURVE('',#22019,#22019,#18789,.T.);
#26523=EDGE_CURVE('',#22019,#22020,#4953,.T.);
#26524=EDGE_CURVE('',#22020,#22020,#18790,.T.);
#26525=EDGE_CURVE('',#22021,#22021,#18791,.T.);
#26526=EDGE_CURVE('',#22021,#22022,#4954,.T.);
#26527=EDGE_CURVE('',#22022,#22022,#18792,.T.);
#26528=EDGE_CURVE('',#22023,#22023,#18793,.T.);
#26529=EDGE_CURVE('',#22023,#22024,#4955,.T.);
#26530=EDGE_CURVE('',#22024,#22024,#18794,.T.);
#26531=EDGE_CURVE('',#22025,#22025,#18795,.T.);
#26532=EDGE_CURVE('',#22025,#22026,#4956,.T.);
#26533=EDGE_CURVE('',#22026,#22026,#18796,.T.);
#26534=EDGE_CURVE('',#22027,#22027,#18797,.T.);
#26535=EDGE_CURVE('',#22027,#22028,#4957,.T.);
#26536=EDGE_CURVE('',#22028,#22028,#18798,.T.);
#26537=EDGE_CURVE('',#22029,#22029,#18799,.T.);
#26538=EDGE_CURVE('',#22029,#22030,#4958,.T.);
#26539=EDGE_CURVE('',#22030,#22030,#18800,.T.);
#26540=EDGE_CURVE('',#22031,#22031,#18801,.T.);
#26541=EDGE_CURVE('',#22031,#22032,#4959,.T.);
#26542=EDGE_CURVE('',#22032,#22032,#18802,.T.);
#26543=EDGE_CURVE('',#22033,#22033,#18803,.T.);
#26544=EDGE_CURVE('',#22033,#22034,#4960,.T.);
#26545=EDGE_CURVE('',#22034,#22034,#18804,.T.);
#26546=EDGE_CURVE('',#22035,#22035,#18805,.T.);
#26547=EDGE_CURVE('',#22035,#22036,#4961,.T.);
#26548=EDGE_CURVE('',#22036,#22036,#18806,.T.);
#26549=EDGE_CURVE('',#22037,#22037,#18807,.T.);
#26550=EDGE_CURVE('',#22037,#22038,#4962,.T.);
#26551=EDGE_CURVE('',#22038,#22038,#18808,.T.);
#26552=EDGE_CURVE('',#22039,#22039,#18809,.T.);
#26553=EDGE_CURVE('',#22039,#22040,#4963,.T.);
#26554=EDGE_CURVE('',#22040,#22040,#18810,.T.);
#26555=EDGE_CURVE('',#22041,#22041,#18811,.T.);
#26556=EDGE_CURVE('',#22041,#22042,#4964,.T.);
#26557=EDGE_CURVE('',#22042,#22042,#18812,.T.);
#26558=EDGE_CURVE('',#22043,#22043,#18813,.T.);
#26559=EDGE_CURVE('',#22043,#22044,#4965,.T.);
#26560=EDGE_CURVE('',#22044,#22044,#18814,.T.);
#26561=EDGE_CURVE('',#22045,#22045,#18815,.T.);
#26562=EDGE_CURVE('',#22045,#22046,#4966,.T.);
#26563=EDGE_CURVE('',#22047,#22046,#2098,.F.);
#26564=EDGE_CURVE('',#22047,#22048,#18816,.T.);
#26565=EDGE_CURVE('',#22046,#22048,#2099,.F.);
#26566=EDGE_CURVE('',#22049,#22049,#18817,.T.);
#26567=EDGE_CURVE('',#22049,#22050,#4967,.T.);
#26568=EDGE_CURVE('',#22050,#22050,#18818,.T.);
#26569=EDGE_CURVE('',#22051,#22051,#18819,.T.);
#26570=EDGE_CURVE('',#22051,#22052,#4968,.T.);
#26571=EDGE_CURVE('',#22052,#22052,#18820,.T.);
#26572=EDGE_CURVE('',#22053,#22053,#18821,.T.);
#26573=EDGE_CURVE('',#22053,#22054,#4969,.T.);
#26574=EDGE_CURVE('',#22054,#22054,#18822,.T.);
#26575=EDGE_CURVE('',#22055,#22055,#18823,.T.);
#26576=EDGE_CURVE('',#22055,#22056,#4970,.T.);
#26577=EDGE_CURVE('',#22056,#22056,#18824,.T.);
#26578=EDGE_CURVE('',#22057,#22057,#18825,.T.);
#26579=EDGE_CURVE('',#22057,#22058,#4971,.T.);
#26580=EDGE_CURVE('',#22058,#22058,#18826,.T.);
#26581=EDGE_CURVE('',#22059,#22059,#18827,.T.);
#26582=EDGE_CURVE('',#22059,#22060,#4972,.T.);
#26583=EDGE_CURVE('',#22060,#22060,#18828,.T.);
#26584=EDGE_CURVE('',#22061,#22061,#18829,.T.);
#26585=EDGE_CURVE('',#22061,#22062,#4973,.T.);
#26586=EDGE_CURVE('',#22062,#22062,#18830,.T.);
#26587=EDGE_CURVE('',#22063,#22063,#18831,.T.);
#26588=EDGE_CURVE('',#22063,#22064,#4974,.T.);
#26589=EDGE_CURVE('',#22064,#22064,#18832,.T.);
#26590=EDGE_CURVE('',#22065,#22065,#18833,.T.);
#26591=EDGE_CURVE('',#22065,#22066,#4975,.T.);
#26592=EDGE_CURVE('',#22066,#22066,#18834,.T.);
#26593=EDGE_CURVE('',#22067,#22067,#18835,.T.);
#26594=EDGE_CURVE('',#22067,#22068,#4976,.T.);
#26595=EDGE_CURVE('',#22068,#22068,#18836,.T.);
#26596=EDGE_CURVE('',#22069,#22069,#18837,.T.);
#26597=EDGE_CURVE('',#22069,#22070,#4977,.T.);
#26598=EDGE_CURVE('',#22070,#22070,#18838,.T.);
#26599=EDGE_CURVE('',#22071,#22071,#18839,.T.);
#26600=EDGE_CURVE('',#22071,#22072,#4978,.T.);
#26601=EDGE_CURVE('',#22072,#22072,#18840,.T.);
#26602=EDGE_CURVE('',#22073,#22073,#18841,.T.);
#26603=EDGE_CURVE('',#22073,#22074,#4979,.T.);
#26604=EDGE_CURVE('',#22074,#22074,#18842,.T.);
#26605=EDGE_CURVE('',#22075,#22075,#18843,.T.);
#26606=EDGE_CURVE('',#22075,#22076,#4980,.T.);
#26607=EDGE_CURVE('',#22076,#22076,#18844,.T.);
#26608=EDGE_CURVE('',#22077,#22077,#18845,.T.);
#26609=EDGE_CURVE('',#22077,#22078,#4981,.T.);
#26610=EDGE_CURVE('',#22078,#22078,#18846,.T.);
#26611=EDGE_CURVE('',#22079,#22079,#18847,.T.);
#26612=EDGE_CURVE('',#22079,#22080,#4982,.T.);
#26613=EDGE_CURVE('',#22080,#22080,#18848,.T.);
#26614=EDGE_CURVE('',#22081,#22081,#18849,.T.);
#26615=EDGE_CURVE('',#22081,#22082,#4983,.T.);
#26616=EDGE_CURVE('',#22082,#22082,#18850,.T.);
#26617=EDGE_CURVE('',#22083,#22083,#18851,.T.);
#26618=EDGE_CURVE('',#22083,#22084,#4984,.T.);
#26619=EDGE_CURVE('',#22085,#22084,#2100,.F.);
#26620=EDGE_CURVE('',#22085,#22086,#18852,.T.);
#26621=EDGE_CURVE('',#22084,#22086,#2101,.F.);
#26622=EDGE_CURVE('',#22087,#22087,#18853,.T.);
#26623=EDGE_CURVE('',#22087,#22088,#4985,.T.);
#26624=EDGE_CURVE('',#22088,#22088,#18854,.T.);
#26625=EDGE_CURVE('',#22089,#22090,#18855,.T.);
#26626=EDGE_CURVE('',#21899,#22089,#18856,.T.);
#26627=EDGE_CURVE('',#21938,#21898,#18857,.T.);
#26628=EDGE_CURVE('',#21975,#21937,#18858,.T.);
#26629=EDGE_CURVE('',#22009,#21976,#18859,.T.);
#26630=EDGE_CURVE('',#22047,#22010,#18860,.T.);
#26631=EDGE_CURVE('',#22085,#22048,#18861,.T.);
#26632=EDGE_CURVE('',#21032,#22086,#18862,.T.);
#26633=EDGE_CURVE('',#21070,#21033,#18863,.T.);
#26634=EDGE_CURVE('',#21104,#21071,#18864,.T.);
#26635=EDGE_CURVE('',#21142,#21105,#18865,.T.);
#26636=EDGE_CURVE('',#21180,#21143,#18866,.T.);
#26637=EDGE_CURVE('',#21218,#21181,#18867,.T.);
#26638=EDGE_CURVE('',#21256,#21219,#18868,.T.);
#26639=EDGE_CURVE('',#21290,#21257,#18869,.T.);
#26640=EDGE_CURVE('',#21328,#21291,#18870,.T.);
#26641=EDGE_CURVE('',#21366,#21329,#18871,.T.);
#26642=EDGE_CURVE('',#21404,#21367,#18872,.T.);
#26643=EDGE_CURVE('',#21442,#21405,#18873,.T.);
#26644=EDGE_CURVE('',#21476,#21443,#18874,.T.);
#26645=EDGE_CURVE('',#21514,#21477,#18875,.T.);
#26646=EDGE_CURVE('',#21552,#21515,#18876,.T.);
#26647=EDGE_CURVE('',#21590,#21553,#18877,.T.);
#26648=EDGE_CURVE('',#21628,#21591,#18878,.T.);
#26649=EDGE_CURVE('',#21662,#21629,#18879,.T.);
#26650=EDGE_CURVE('',#21701,#21663,#18880,.T.);
#26651=EDGE_CURVE('',#22091,#21700,#18881,.T.);
#26652=EDGE_CURVE('',#22090,#22091,#18882,.T.);
#26653=EDGE_CURVE('',#22092,#22093,#2102,.T.);
#26654=EDGE_CURVE('',#22093,#22092,#2103,.T.);
#26655=EDGE_CURVE('',#22094,#22095,#18883,.T.);
#26656=EDGE_CURVE('',#22096,#22094,#18884,.T.);
#26657=EDGE_CURVE('',#22096,#22097,#2104,.T.);
#26658=EDGE_CURVE('',#22097,#22098,#2105,.T.);
#26659=EDGE_CURVE('',#22098,#22099,#2106,.T.);
#26660=EDGE_CURVE('',#22099,#22100,#2107,.T.);
#26661=EDGE_CURVE('',#22100,#22101,#2108,.T.);
#26662=EDGE_CURVE('',#22101,#22102,#2109,.T.);
#26663=EDGE_CURVE('',#22095,#22102,#18885,.T.);
#26664=EDGE_CURVE('',#22103,#22104,#18886,.T.);
#26665=EDGE_CURVE('',#22104,#22105,#4986,.T.);
#26666=EDGE_CURVE('',#22105,#22105,#18887,.T.);
#26667=EDGE_CURVE('',#22104,#22103,#18888,.T.);
#26668=EDGE_CURVE('',#22105,#22106,#18889,.T.);
#26669=EDGE_CURVE('',#22106,#22106,#18890,.T.);
#26670=EDGE_CURVE('',#22103,#22107,#18891,.T.);
#26671=EDGE_CURVE('',#22108,#22107,#18892,.T.);
#26672=EDGE_CURVE('',#22107,#22108,#18893,.T.);
#26673=EDGE_CURVE('',#22109,#22110,#18894,.T.);
#26674=EDGE_CURVE('',#22111,#22110,#2110,.T.);
#26675=EDGE_CURVE('',#22112,#22111,#18895,.T.);
#26676=EDGE_CURVE('',#22112,#22109,#2111,.T.);
#26677=EDGE_CURVE('',#22113,#22114,#18896,.T.);
#26678=EDGE_CURVE('',#22115,#22113,#18897,.T.);
#26679=EDGE_CURVE('',#22116,#22115,#18898,.T.);
#26680=EDGE_CURVE('',#22116,#22114,#18899,.T.);
#26681=EDGE_CURVE('',#22117,#22118,#18900,.T.);
#26682=EDGE_CURVE('',#22118,#22119,#18901,.T.);
#26683=EDGE_CURVE('',#22120,#22119,#4987,.T.);
#26684=EDGE_CURVE('',#22121,#22120,#18902,.T.);
#26685=EDGE_CURVE('',#22117,#22121,#4988,.T.);
#26686=EDGE_CURVE('',#22098,#22110,#2112,.T.);
#26687=EDGE_CURVE('',#22100,#22109,#18903,.T.);
#26688=EDGE_CURVE('',#22122,#22123,#18904,.T.);
#26689=EDGE_CURVE('',#22123,#22108,#4989,.T.);
#26690=EDGE_CURVE('',#22123,#22122,#18905,.T.);
#26691=EDGE_CURVE('',#22122,#22124,#18906,.T.);
#26692=EDGE_CURVE('',#22124,#22124,#18907,.T.);
#26693=EDGE_CURVE('',#22125,#22125,#18908,.T.);
#26694=EDGE_CURVE('',#22125,#22126,#4990,.T.);
#26695=EDGE_CURVE('',#22126,#22126,#2113,.T.);
#26696=EDGE_CURVE('',#22127,#22128,#2114,.T.);
#26697=EDGE_CURVE('',#22128,#22093,#4991,.T.);
#26698=EDGE_CURVE('',#22128,#22127,#2115,.T.);
#26699=EDGE_CURVE('',#22129,#22130,#4992,.T.);
#26700=EDGE_CURVE('',#22130,#22131,#2116,.T.);
#26701=EDGE_CURVE('',#22131,#22132,#4993,.T.);
#26702=EDGE_CURVE('',#22132,#22133,#2117,.T.);
#26703=EDGE_CURVE('',#22134,#22133,#4994,.T.);
#26704=EDGE_CURVE('',#22134,#22129,#4995,.T.);
#26705=EDGE_CURVE('',#22135,#22136,#18909,.T.);
#26706=EDGE_CURVE('',#22136,#22137,#2118,.T.);
#26707=EDGE_CURVE('',#22135,#22137,#4996,.T.);
#26708=EDGE_CURVE('',#22136,#22138,#2119,.T.);
#26709=EDGE_CURVE('',#22139,#22135,#18910,.T.);
#26710=EDGE_CURVE('',#22138,#22139,#18911,.T.);
#26711=EDGE_CURVE('',#22140,#22141,#4997,.T.);
#26712=EDGE_CURVE('',#22141,#22142,#2915,.T.);
#26713=EDGE_CURVE('',#22130,#22142,#4998,.T.);
#26714=EDGE_CURVE('',#22129,#22143,#18912,.T.);
#26715=EDGE_CURVE('',#22143,#22140,#4999,.T.);
#26716=EDGE_CURVE('',#22133,#22144,#2120,.T.);
#26717=EDGE_CURVE('',#22144,#22134,#18913,.T.);
#26718=EDGE_CURVE('',#22145,#22146,#5000,.T.);
#26719=EDGE_CURVE('',#22146,#22140,#2121,.T.);
#26720=EDGE_CURVE('',#22143,#22135,#5001,.T.);
#26721=EDGE_CURVE('',#22137,#22145,#2122,.T.);
#26722=EDGE_CURVE('',#22147,#22148,#5002,.T.);
#26723=EDGE_CURVE('',#22148,#22149,#18914,.T.);
#26724=EDGE_CURVE('',#22149,#22150,#5003,.T.);
#26725=EDGE_CURVE('',#22150,#22147,#18915,.T.);
#26726=EDGE_CURVE('',#22151,#22152,#5004,.T.);
#26727=EDGE_CURVE('',#22151,#22153,#5005,.T.);
#26728=EDGE_CURVE('',#22139,#22153,#5006,.T.);
#26729=EDGE_CURVE('',#22139,#22152,#5007,.T.);
#26730=EDGE_CURVE('',#22154,#22155,#5008,.T.);
#26731=EDGE_CURVE('',#22154,#22151,#18916,.T.);
#26732=EDGE_CURVE('',#22152,#22155,#18917,.T.);
#26733=EDGE_CURVE('',#22138,#22156,#2123,.T.);
#26734=EDGE_CURVE('',#22153,#22157,#18918,.T.);
#26735=EDGE_CURVE('',#22158,#22157,#5009,.T.);
#26736=EDGE_CURVE('',#22158,#22159,#18919,.T.);
#26737=EDGE_CURVE('',#22160,#22159,#2124,.T.);
#26738=EDGE_CURVE('',#22156,#22160,#2125,.T.);
#26739=EDGE_CURVE('',#22157,#22154,#5010,.T.);
#26740=EDGE_CURVE('',#22155,#22158,#5011,.T.);
#26741=EDGE_CURVE('',#22151,#22150,#18920,.T.);
#26742=EDGE_CURVE('',#22147,#22154,#18921,.T.);
#26743=EDGE_CURVE('',#22148,#22157,#18922,.T.);
#26744=EDGE_CURVE('',#22153,#22149,#18923,.T.);
#26745=EDGE_CURVE('',#22159,#22144,#2126,.T.);
#26746=EDGE_CURVE('',#22134,#22158,#18924,.T.);
#26747=EDGE_CURVE('',#22129,#22155,#18925,.T.);
#26748=EDGE_CURVE('',#22152,#22143,#18926,.T.);
#26749=EDGE_CURVE('',#22161,#22131,#18927,.T.);
#26750=EDGE_CURVE('',#22162,#22130,#2127,.T.);
#26751=EDGE_CURVE('',#22162,#22163,#18928,.T.);
#26752=EDGE_CURVE('',#22161,#22163,#2128,.T.);
#26753=EDGE_CURVE('',#22164,#22165,#18929,.T.);
#26754=EDGE_CURVE('',#22163,#22165,#2129,.T.);
#26755=EDGE_CURVE('',#22164,#22162,#2130,.T.);
#26756=EDGE_CURVE('',#22166,#22132,#18930,.T.);
#26757=EDGE_CURVE('',#22166,#22161,#5012,.T.);
#26758=EDGE_CURVE('',#22146,#22167,#18931,.T.);
#26759=EDGE_CURVE('',#22165,#22167,#2131,.T.);
#26760=EDGE_CURVE('',#22140,#22164,#2132,.T.);
#26761=EDGE_CURVE('',#22168,#22145,#18932,.T.);
#26762=EDGE_CURVE('',#22167,#22168,#5013,.T.);
#26763=EDGE_CURVE('',#22160,#22156,#2133,.T.);
#26764=EDGE_CURVE('',#22101,#22169,#18933,.T.);
#26765=EDGE_CURVE('',#22170,#22169,#2134,.T.);
#26766=EDGE_CURVE('',#22170,#22171,#18934,.T.);
#26767=EDGE_CURVE('',#22171,#22102,#2135,.T.);
#26768=EDGE_CURVE('',#22172,#22173,#18935,.T.);
#26769=EDGE_CURVE('',#22174,#22173,#2136,.T.);
#26770=EDGE_CURVE('',#22175,#22174,#2137,.T.);
#26771=EDGE_CURVE('',#22171,#22175,#2138,.T.);
#26772=EDGE_CURVE('',#22172,#22170,#2139,.T.);
#26773=EDGE_CURVE('',#22169,#22109,#2140,.T.);
#26774=EDGE_CURVE('',#22176,#22097,#18936,.T.);
#26775=EDGE_CURVE('',#22096,#22173,#2141,.T.);
#26776=EDGE_CURVE('',#22176,#22172,#2142,.T.);
#26777=EDGE_CURVE('',#22110,#22176,#2143,.T.);
#26778=EDGE_CURVE('',#22177,#22120,#18937,.T.);
#26779=EDGE_CURVE('',#22177,#22178,#18938,.T.);
#26780=EDGE_CURVE('',#22121,#22178,#2144,.T.);
#26781=EDGE_CURVE('',#22179,#22180,#18939,.T.);
#26782=EDGE_CURVE('',#22178,#22180,#18940,.T.);
#26783=EDGE_CURVE('',#22179,#22177,#18941,.T.);
#26784=EDGE_CURVE('',#22181,#22182,#18942,.T.);
#26785=EDGE_CURVE('',#22180,#22182,#2145,.T.);
#26786=EDGE_CURVE('',#22181,#22179,#18943,.T.);
#26787=EDGE_CURVE('',#22119,#22113,#18944,.T.);
#26788=EDGE_CURVE('',#22115,#22117,#2146,.T.);
#26789=EDGE_CURVE('',#22183,#22184,#18945,.T.);
#26790=EDGE_CURVE('',#22182,#22184,#5014,.T.);
#26791=EDGE_CURVE('',#22183,#22181,#5015,.T.);
#26792=EDGE_CURVE('',#22114,#22183,#18946,.T.);
#26793=EDGE_CURVE('',#22184,#22116,#2147,.T.);
#26794=EDGE_CURVE('',#22185,#22169,#2148,.T.);
#26795=EDGE_CURVE('',#22185,#22112,#2149,.T.);
#26796=EDGE_CURVE('',#22186,#22176,#18947,.T.);
#26797=EDGE_CURVE('',#22111,#22186,#2150,.T.);
#26798=EDGE_CURVE('',#22111,#22187,#2151,.T.);
#26799=EDGE_CURVE('',#22187,#22188,#2152,.T.);
#26800=EDGE_CURVE('',#22188,#22189,#18948,.T.);
#26801=EDGE_CURVE('',#22189,#22190,#2153,.T.);
#26802=EDGE_CURVE('',#22190,#22112,#2154,.T.);
#26803=EDGE_CURVE('',#22170,#22191,#2155,.T.);
#26804=EDGE_CURVE('',#22192,#22185,#2156,.T.);
#26805=EDGE_CURVE('',#22192,#22191,#18949,.T.);
#26806=EDGE_CURVE('',#22193,#22172,#2157,.T.);
#26807=EDGE_CURVE('',#22194,#22193,#18950,.T.);
#26808=EDGE_CURVE('',#22186,#22194,#2158,.T.);
#26809=EDGE_CURVE('',#22190,#22195,#2159,.T.);
#26810=EDGE_CURVE('',#22195,#22192,#5016,.T.);
#26811=EDGE_CURVE('',#22196,#22194,#5017,.T.);
#26812=EDGE_CURVE('',#22196,#22187,#2160,.T.);
#26813=EDGE_CURVE('',#22197,#22198,#2161,.T.);
#26814=EDGE_CURVE('',#22198,#22197,#18951,.T.);
#26815=EDGE_CURVE('',#22199,#22198,#2162,.T.);
#26816=EDGE_CURVE('',#22197,#22200,#2163,.T.);
#26817=EDGE_CURVE('',#22200,#22201,#2164,.T.);
#26818=EDGE_CURVE('',#22201,#22202,#2165,.T.);
#26819=EDGE_CURVE('',#22202,#22199,#2166,.T.);
#26820=EDGE_CURVE('',#22198,#22189,#2167,.T.);
#26821=EDGE_CURVE('',#22197,#22188,#18952,.T.);
#26822=EDGE_CURVE('',#22200,#22187,#2168,.T.);
#26823=EDGE_CURVE('',#22201,#22196,#18953,.T.);
#26824=EDGE_CURVE('',#22201,#22113,#2169,.T.);
#26825=EDGE_CURVE('',#22114,#22202,#2170,.T.);
#26826=EDGE_CURVE('',#22202,#22195,#18954,.T.);
#26827=EDGE_CURVE('',#22199,#22190,#2171,.T.);
#26828=EDGE_CURVE('',#22181,#22192,#2172,.T.);
#26829=EDGE_CURVE('',#22191,#22179,#2173,.T.);
#26830=EDGE_CURVE('',#22177,#22193,#2174,.T.);
#26831=EDGE_CURVE('',#22194,#22120,#2175,.T.);
#26832=EDGE_CURVE('',#22119,#22196,#2176,.T.);
#26833=EDGE_CURVE('',#22195,#22183,#2177,.T.);
#26834=EDGE_CURVE('',#22161,#22191,#2916,.T.);
#26835=EDGE_CURVE('',#22193,#22167,#2917,.T.);
#26836=EDGE_CURVE('',#22168,#22166,#2178,.T.);
#26837=EDGE_CURVE('',#22095,#22094,#2179,.T.);
#26838=EDGE_CURVE('',#21771,#21734,#2180,.T.);
#26839=EDGE_CURVE('',#21829,#21770,#2181,.T.);
#26840=EDGE_CURVE('',#21900,#21828,#2182,.T.);
#26841=EDGE_CURVE('',#22089,#22090,#2183,.T.);
#26842=EDGE_CURVE('',#21741,#22091,#2184,.T.);
#26843=EDGE_CURVE('',#21735,#21740,#2185,.T.);
#26844=EDGE_CURVE('',#22090,#22094,#18955,.T.);
#26845=EDGE_CURVE('',#22095,#22089,#18956,.T.);
#26846=EDGE_CURVE('',#22164,#22141,#5018,.T.);
#26847=EDGE_CURVE('',#22162,#22142,#5019,.T.);
#30342=ORIENTED_EDGE('',*,*,#24515,.F.);
#30343=ORIENTED_EDGE('',*,*,#24516,.T.);
#30344=ORIENTED_EDGE('',*,*,#24517,.F.);
#30345=ORIENTED_EDGE('',*,*,#24518,.T.);
#30346=ORIENTED_EDGE('',*,*,#24518,.F.);
#30347=ORIENTED_EDGE('',*,*,#24519,.T.);
#30348=ORIENTED_EDGE('',*,*,#24520,.T.);
#30349=ORIENTED_EDGE('',*,*,#24521,.T.);
#30350=ORIENTED_EDGE('',*,*,#24516,.F.);
#30351=ORIENTED_EDGE('',*,*,#24522,.T.);
#30352=ORIENTED_EDGE('',*,*,#24520,.F.);
#30353=ORIENTED_EDGE('',*,*,#24523,.F.);
#30354=ORIENTED_EDGE('',*,*,#24519,.F.);
#30355=ORIENTED_EDGE('',*,*,#24517,.T.);
#30356=ORIENTED_EDGE('',*,*,#24523,.T.);
#30357=ORIENTED_EDGE('',*,*,#24522,.F.);
#30358=ORIENTED_EDGE('',*,*,#24515,.T.);
#30359=ORIENTED_EDGE('',*,*,#24521,.F.);
#30360=ORIENTED_EDGE('',*,*,#24524,.F.);
#30361=ORIENTED_EDGE('',*,*,#24525,.T.);
#30362=ORIENTED_EDGE('',*,*,#24526,.T.);
#30363=ORIENTED_EDGE('',*,*,#24527,.T.);
#30364=ORIENTED_EDGE('',*,*,#24526,.F.);
#30365=ORIENTED_EDGE('',*,*,#24528,.T.);
#30366=ORIENTED_EDGE('',*,*,#24529,.F.);
#30367=ORIENTED_EDGE('',*,*,#24530,.F.);
#30368=ORIENTED_EDGE('',*,*,#24524,.T.);
#30369=ORIENTED_EDGE('',*,*,#24531,.F.);
#30370=ORIENTED_EDGE('',*,*,#24527,.F.);
#30371=ORIENTED_EDGE('',*,*,#24529,.T.);
#30372=ORIENTED_EDGE('',*,*,#24532,.T.);
#30373=ORIENTED_EDGE('',*,*,#24531,.T.);
#30374=ORIENTED_EDGE('',*,*,#24525,.F.);
#30375=ORIENTED_EDGE('',*,*,#24530,.T.);
#30376=ORIENTED_EDGE('',*,*,#24532,.F.);
#30377=ORIENTED_EDGE('',*,*,#24528,.F.);
#30378=ORIENTED_EDGE('',*,*,#24533,.T.);
#30379=ORIENTED_EDGE('',*,*,#24534,.T.);
#30380=ORIENTED_EDGE('',*,*,#24535,.F.);
#30381=ORIENTED_EDGE('',*,*,#24534,.F.);
#30382=ORIENTED_EDGE('',*,*,#24536,.T.);
#30383=ORIENTED_EDGE('',*,*,#24537,.T.);
#30384=ORIENTED_EDGE('',*,*,#24538,.F.);
#30385=ORIENTED_EDGE('',*,*,#24537,.F.);
#30386=ORIENTED_EDGE('',*,*,#24539,.T.);
#30387=ORIENTED_EDGE('',*,*,#24540,.T.);
#30388=ORIENTED_EDGE('',*,*,#24541,.F.);
#30389=ORIENTED_EDGE('',*,*,#24540,.F.);
#30390=ORIENTED_EDGE('',*,*,#24542,.T.);
#30391=ORIENTED_EDGE('',*,*,#24543,.T.);
#30392=ORIENTED_EDGE('',*,*,#24544,.F.);
#30393=ORIENTED_EDGE('',*,*,#24543,.F.);
#30394=ORIENTED_EDGE('',*,*,#24545,.T.);
#30395=ORIENTED_EDGE('',*,*,#24546,.T.);
#30396=ORIENTED_EDGE('',*,*,#24547,.F.);
#30397=ORIENTED_EDGE('',*,*,#24546,.F.);
#30398=ORIENTED_EDGE('',*,*,#24548,.T.);
#30399=ORIENTED_EDGE('',*,*,#24549,.T.);
#30400=ORIENTED_EDGE('',*,*,#24550,.F.);
#30401=ORIENTED_EDGE('',*,*,#24549,.F.);
#30402=ORIENTED_EDGE('',*,*,#24551,.T.);
#30403=ORIENTED_EDGE('',*,*,#24552,.T.);
#30404=ORIENTED_EDGE('',*,*,#24553,.F.);
#30405=ORIENTED_EDGE('',*,*,#24552,.F.);
#30406=ORIENTED_EDGE('',*,*,#24554,.T.);
#30407=ORIENTED_EDGE('',*,*,#24555,.T.);
#30408=ORIENTED_EDGE('',*,*,#24556,.F.);
#30409=ORIENTED_EDGE('',*,*,#24555,.F.);
#30410=ORIENTED_EDGE('',*,*,#24557,.T.);
#30411=ORIENTED_EDGE('',*,*,#24558,.T.);
#30412=ORIENTED_EDGE('',*,*,#24559,.F.);
#30413=ORIENTED_EDGE('',*,*,#24558,.F.);
#30414=ORIENTED_EDGE('',*,*,#24560,.T.);
#30415=ORIENTED_EDGE('',*,*,#24561,.T.);
#30416=ORIENTED_EDGE('',*,*,#24562,.F.);
#30417=ORIENTED_EDGE('',*,*,#24561,.F.);
#30418=ORIENTED_EDGE('',*,*,#24563,.T.);
#30419=ORIENTED_EDGE('',*,*,#24564,.T.);
#30420=ORIENTED_EDGE('',*,*,#24565,.F.);
#30421=ORIENTED_EDGE('',*,*,#24564,.F.);
#30422=ORIENTED_EDGE('',*,*,#24566,.T.);
#30423=ORIENTED_EDGE('',*,*,#24567,.T.);
#30424=ORIENTED_EDGE('',*,*,#24568,.F.);
#30425=ORIENTED_EDGE('',*,*,#24567,.F.);
#30426=ORIENTED_EDGE('',*,*,#24569,.T.);
#30427=ORIENTED_EDGE('',*,*,#24570,.T.);
#30428=ORIENTED_EDGE('',*,*,#24571,.F.);
#30429=ORIENTED_EDGE('',*,*,#24570,.F.);
#30430=ORIENTED_EDGE('',*,*,#24572,.T.);
#30431=ORIENTED_EDGE('',*,*,#24573,.T.);
#30432=ORIENTED_EDGE('',*,*,#24574,.T.);
#30433=ORIENTED_EDGE('',*,*,#24575,.F.);
#30434=ORIENTED_EDGE('',*,*,#24574,.F.);
#30435=ORIENTED_EDGE('',*,*,#24576,.T.);
#30436=ORIENTED_EDGE('',*,*,#24577,.T.);
#30437=ORIENTED_EDGE('',*,*,#24578,.F.);
#30438=ORIENTED_EDGE('',*,*,#24577,.F.);
#30439=ORIENTED_EDGE('',*,*,#24579,.T.);
#30440=ORIENTED_EDGE('',*,*,#24580,.T.);
#30441=ORIENTED_EDGE('',*,*,#24581,.T.);
#30442=ORIENTED_EDGE('',*,*,#24582,.F.);
#30443=ORIENTED_EDGE('',*,*,#24581,.F.);
#30444=ORIENTED_EDGE('',*,*,#24583,.T.);
#30445=ORIENTED_EDGE('',*,*,#24584,.T.);
#30446=ORIENTED_EDGE('',*,*,#24585,.F.);
#30447=ORIENTED_EDGE('',*,*,#24584,.F.);
#30448=ORIENTED_EDGE('',*,*,#24586,.T.);
#30449=ORIENTED_EDGE('',*,*,#24587,.T.);
#30450=ORIENTED_EDGE('',*,*,#24588,.T.);
#30451=ORIENTED_EDGE('',*,*,#24589,.F.);
#30452=ORIENTED_EDGE('',*,*,#24588,.F.);
#30453=ORIENTED_EDGE('',*,*,#24590,.T.);
#30454=ORIENTED_EDGE('',*,*,#24591,.T.);
#30455=ORIENTED_EDGE('',*,*,#24592,.F.);
#30456=ORIENTED_EDGE('',*,*,#24591,.F.);
#30457=ORIENTED_EDGE('',*,*,#24593,.T.);
#30458=ORIENTED_EDGE('',*,*,#24594,.T.);
#30459=ORIENTED_EDGE('',*,*,#24595,.T.);
#30460=ORIENTED_EDGE('',*,*,#24596,.F.);
#30461=ORIENTED_EDGE('',*,*,#24595,.F.);
#30462=ORIENTED_EDGE('',*,*,#24597,.T.);
#30463=ORIENTED_EDGE('',*,*,#24598,.T.);
#30464=ORIENTED_EDGE('',*,*,#24599,.F.);
#30465=ORIENTED_EDGE('',*,*,#24598,.F.);
#30466=ORIENTED_EDGE('',*,*,#24600,.T.);
#30467=ORIENTED_EDGE('',*,*,#24601,.T.);
#30468=ORIENTED_EDGE('',*,*,#24602,.T.);
#30469=ORIENTED_EDGE('',*,*,#24603,.F.);
#30470=ORIENTED_EDGE('',*,*,#24602,.F.);
#30471=ORIENTED_EDGE('',*,*,#24604,.T.);
#30472=ORIENTED_EDGE('',*,*,#24605,.T.);
#30473=ORIENTED_EDGE('',*,*,#24606,.F.);
#30474=ORIENTED_EDGE('',*,*,#24605,.F.);
#30475=ORIENTED_EDGE('',*,*,#24607,.T.);
#30476=ORIENTED_EDGE('',*,*,#24608,.T.);
#30477=ORIENTED_EDGE('',*,*,#24609,.T.);
#30478=ORIENTED_EDGE('',*,*,#24610,.F.);
#30479=ORIENTED_EDGE('',*,*,#24609,.F.);
#30480=ORIENTED_EDGE('',*,*,#24611,.T.);
#30481=ORIENTED_EDGE('',*,*,#24612,.T.);
#30482=ORIENTED_EDGE('',*,*,#24613,.F.);
#30483=ORIENTED_EDGE('',*,*,#24612,.F.);
#30484=ORIENTED_EDGE('',*,*,#24614,.T.);
#30485=ORIENTED_EDGE('',*,*,#24615,.T.);
#30486=ORIENTED_EDGE('',*,*,#24616,.T.);
#30487=ORIENTED_EDGE('',*,*,#24617,.F.);
#30488=ORIENTED_EDGE('',*,*,#24616,.F.);
#30489=ORIENTED_EDGE('',*,*,#24618,.T.);
#30490=ORIENTED_EDGE('',*,*,#24619,.T.);
#30491=ORIENTED_EDGE('',*,*,#24620,.F.);
#30492=ORIENTED_EDGE('',*,*,#24619,.F.);
#30493=ORIENTED_EDGE('',*,*,#24621,.T.);
#30494=ORIENTED_EDGE('',*,*,#24622,.T.);
#30495=ORIENTED_EDGE('',*,*,#24623,.T.);
#30496=ORIENTED_EDGE('',*,*,#24624,.F.);
#30497=ORIENTED_EDGE('',*,*,#24623,.F.);
#30498=ORIENTED_EDGE('',*,*,#24625,.T.);
#30499=ORIENTED_EDGE('',*,*,#24626,.T.);
#30500=ORIENTED_EDGE('',*,*,#24627,.F.);
#30501=ORIENTED_EDGE('',*,*,#24626,.F.);
#30502=ORIENTED_EDGE('',*,*,#24628,.T.);
#30503=ORIENTED_EDGE('',*,*,#24629,.T.);
#30504=ORIENTED_EDGE('',*,*,#24630,.T.);
#30505=ORIENTED_EDGE('',*,*,#24631,.F.);
#30506=ORIENTED_EDGE('',*,*,#24630,.F.);
#30507=ORIENTED_EDGE('',*,*,#24632,.T.);
#30508=ORIENTED_EDGE('',*,*,#24633,.T.);
#30509=ORIENTED_EDGE('',*,*,#24634,.F.);
#30510=ORIENTED_EDGE('',*,*,#24633,.F.);
#30511=ORIENTED_EDGE('',*,*,#24635,.T.);
#30512=ORIENTED_EDGE('',*,*,#24636,.T.);
#30513=ORIENTED_EDGE('',*,*,#24637,.T.);
#30514=ORIENTED_EDGE('',*,*,#24638,.F.);
#30515=ORIENTED_EDGE('',*,*,#24637,.F.);
#30516=ORIENTED_EDGE('',*,*,#24639,.T.);
#30517=ORIENTED_EDGE('',*,*,#24640,.T.);
#30518=ORIENTED_EDGE('',*,*,#24641,.F.);
#30519=ORIENTED_EDGE('',*,*,#24640,.F.);
#30520=ORIENTED_EDGE('',*,*,#24642,.T.);
#30521=ORIENTED_EDGE('',*,*,#24643,.T.);
#30522=ORIENTED_EDGE('',*,*,#24644,.T.);
#30523=ORIENTED_EDGE('',*,*,#24645,.F.);
#30524=ORIENTED_EDGE('',*,*,#24644,.F.);
#30525=ORIENTED_EDGE('',*,*,#24646,.T.);
#30526=ORIENTED_EDGE('',*,*,#24647,.T.);
#30527=ORIENTED_EDGE('',*,*,#24648,.F.);
#30528=ORIENTED_EDGE('',*,*,#24647,.F.);
#30529=ORIENTED_EDGE('',*,*,#24649,.T.);
#30530=ORIENTED_EDGE('',*,*,#24650,.T.);
#30531=ORIENTED_EDGE('',*,*,#24651,.T.);
#30532=ORIENTED_EDGE('',*,*,#24652,.F.);
#30533=ORIENTED_EDGE('',*,*,#24651,.F.);
#30534=ORIENTED_EDGE('',*,*,#24653,.T.);
#30535=ORIENTED_EDGE('',*,*,#24654,.T.);
#30536=ORIENTED_EDGE('',*,*,#24655,.F.);
#30537=ORIENTED_EDGE('',*,*,#24654,.F.);
#30538=ORIENTED_EDGE('',*,*,#24656,.T.);
#30539=ORIENTED_EDGE('',*,*,#24657,.T.);
#30540=ORIENTED_EDGE('',*,*,#24658,.T.);
#30541=ORIENTED_EDGE('',*,*,#24659,.F.);
#30542=ORIENTED_EDGE('',*,*,#24658,.F.);
#30543=ORIENTED_EDGE('',*,*,#24660,.T.);
#30544=ORIENTED_EDGE('',*,*,#24661,.T.);
#30545=ORIENTED_EDGE('',*,*,#24662,.F.);
#30546=ORIENTED_EDGE('',*,*,#24661,.F.);
#30547=ORIENTED_EDGE('',*,*,#24663,.T.);
#30548=ORIENTED_EDGE('',*,*,#24664,.T.);
#30549=ORIENTED_EDGE('',*,*,#24665,.T.);
#30550=ORIENTED_EDGE('',*,*,#24666,.F.);
#30551=ORIENTED_EDGE('',*,*,#24665,.F.);
#30552=ORIENTED_EDGE('',*,*,#24667,.T.);
#30553=ORIENTED_EDGE('',*,*,#24668,.T.);
#30554=ORIENTED_EDGE('',*,*,#24669,.F.);
#30555=ORIENTED_EDGE('',*,*,#24668,.F.);
#30556=ORIENTED_EDGE('',*,*,#24670,.T.);
#30557=ORIENTED_EDGE('',*,*,#24671,.T.);
#30558=ORIENTED_EDGE('',*,*,#24672,.T.);
#30559=ORIENTED_EDGE('',*,*,#24673,.F.);
#30560=ORIENTED_EDGE('',*,*,#24672,.F.);
#30561=ORIENTED_EDGE('',*,*,#24674,.T.);
#30562=ORIENTED_EDGE('',*,*,#24675,.T.);
#30563=ORIENTED_EDGE('',*,*,#24676,.F.);
#30564=ORIENTED_EDGE('',*,*,#24675,.F.);
#30565=ORIENTED_EDGE('',*,*,#24677,.T.);
#30566=ORIENTED_EDGE('',*,*,#24678,.T.);
#30567=ORIENTED_EDGE('',*,*,#24679,.T.);
#30568=ORIENTED_EDGE('',*,*,#24680,.F.);
#30569=ORIENTED_EDGE('',*,*,#24679,.F.);
#30570=ORIENTED_EDGE('',*,*,#24681,.T.);
#30571=ORIENTED_EDGE('',*,*,#24682,.T.);
#30572=ORIENTED_EDGE('',*,*,#24683,.F.);
#30573=ORIENTED_EDGE('',*,*,#24682,.F.);
#30574=ORIENTED_EDGE('',*,*,#24684,.T.);
#30575=ORIENTED_EDGE('',*,*,#24685,.T.);
#30576=ORIENTED_EDGE('',*,*,#24686,.T.);
#30577=ORIENTED_EDGE('',*,*,#24687,.F.);
#30578=ORIENTED_EDGE('',*,*,#24686,.F.);
#30579=ORIENTED_EDGE('',*,*,#24688,.T.);
#30580=ORIENTED_EDGE('',*,*,#24689,.T.);
#30581=ORIENTED_EDGE('',*,*,#24690,.F.);
#30582=ORIENTED_EDGE('',*,*,#24689,.F.);
#30583=ORIENTED_EDGE('',*,*,#24691,.T.);
#30584=ORIENTED_EDGE('',*,*,#24692,.T.);
#30585=ORIENTED_EDGE('',*,*,#24693,.T.);
#30586=ORIENTED_EDGE('',*,*,#24694,.F.);
#30587=ORIENTED_EDGE('',*,*,#24693,.F.);
#30588=ORIENTED_EDGE('',*,*,#24695,.T.);
#30589=ORIENTED_EDGE('',*,*,#24696,.T.);
#30590=ORIENTED_EDGE('',*,*,#24697,.F.);
#30591=ORIENTED_EDGE('',*,*,#24696,.F.);
#30592=ORIENTED_EDGE('',*,*,#24698,.T.);
#30593=ORIENTED_EDGE('',*,*,#24699,.T.);
#30594=ORIENTED_EDGE('',*,*,#24700,.T.);
#30595=ORIENTED_EDGE('',*,*,#24701,.F.);
#30596=ORIENTED_EDGE('',*,*,#24700,.F.);
#30597=ORIENTED_EDGE('',*,*,#24702,.T.);
#30598=ORIENTED_EDGE('',*,*,#24703,.T.);
#30599=ORIENTED_EDGE('',*,*,#24704,.F.);
#30600=ORIENTED_EDGE('',*,*,#24703,.F.);
#30601=ORIENTED_EDGE('',*,*,#24705,.T.);
#30602=ORIENTED_EDGE('',*,*,#24706,.T.);
#30603=ORIENTED_EDGE('',*,*,#24707,.T.);
#30604=ORIENTED_EDGE('',*,*,#24708,.F.);
#30605=ORIENTED_EDGE('',*,*,#24707,.F.);
#30606=ORIENTED_EDGE('',*,*,#24709,.T.);
#30607=ORIENTED_EDGE('',*,*,#24710,.T.);
#30608=ORIENTED_EDGE('',*,*,#24711,.F.);
#30609=ORIENTED_EDGE('',*,*,#24710,.F.);
#30610=ORIENTED_EDGE('',*,*,#24712,.T.);
#30611=ORIENTED_EDGE('',*,*,#24713,.T.);
#30612=ORIENTED_EDGE('',*,*,#24714,.T.);
#30613=ORIENTED_EDGE('',*,*,#24715,.F.);
#30614=ORIENTED_EDGE('',*,*,#24714,.F.);
#30615=ORIENTED_EDGE('',*,*,#24716,.T.);
#30616=ORIENTED_EDGE('',*,*,#24717,.T.);
#30617=ORIENTED_EDGE('',*,*,#24718,.F.);
#30618=ORIENTED_EDGE('',*,*,#24717,.F.);
#30619=ORIENTED_EDGE('',*,*,#24719,.T.);
#30620=ORIENTED_EDGE('',*,*,#24720,.T.);
#30621=ORIENTED_EDGE('',*,*,#24721,.T.);
#30622=ORIENTED_EDGE('',*,*,#24722,.F.);
#30623=ORIENTED_EDGE('',*,*,#24721,.F.);
#30624=ORIENTED_EDGE('',*,*,#24723,.T.);
#30625=ORIENTED_EDGE('',*,*,#24724,.T.);
#30626=ORIENTED_EDGE('',*,*,#24725,.F.);
#30627=ORIENTED_EDGE('',*,*,#24724,.F.);
#30628=ORIENTED_EDGE('',*,*,#24726,.T.);
#30629=ORIENTED_EDGE('',*,*,#24727,.T.);
#30630=ORIENTED_EDGE('',*,*,#24728,.T.);
#30631=ORIENTED_EDGE('',*,*,#24729,.F.);
#30632=ORIENTED_EDGE('',*,*,#24728,.F.);
#30633=ORIENTED_EDGE('',*,*,#24730,.T.);
#30634=ORIENTED_EDGE('',*,*,#24731,.T.);
#30635=ORIENTED_EDGE('',*,*,#24732,.F.);
#30636=ORIENTED_EDGE('',*,*,#24731,.F.);
#30637=ORIENTED_EDGE('',*,*,#24733,.T.);
#30638=ORIENTED_EDGE('',*,*,#24734,.T.);
#30639=ORIENTED_EDGE('',*,*,#24735,.T.);
#30640=ORIENTED_EDGE('',*,*,#24736,.F.);
#30641=ORIENTED_EDGE('',*,*,#24735,.F.);
#30642=ORIENTED_EDGE('',*,*,#24737,.T.);
#30643=ORIENTED_EDGE('',*,*,#24738,.T.);
#30644=ORIENTED_EDGE('',*,*,#24739,.F.);
#30645=ORIENTED_EDGE('',*,*,#24738,.F.);
#30646=ORIENTED_EDGE('',*,*,#24740,.T.);
#30647=ORIENTED_EDGE('',*,*,#24741,.T.);
#30648=ORIENTED_EDGE('',*,*,#24742,.T.);
#30649=ORIENTED_EDGE('',*,*,#24743,.F.);
#30650=ORIENTED_EDGE('',*,*,#24742,.F.);
#30651=ORIENTED_EDGE('',*,*,#24744,.T.);
#30652=ORIENTED_EDGE('',*,*,#24745,.T.);
#30653=ORIENTED_EDGE('',*,*,#24746,.F.);
#30654=ORIENTED_EDGE('',*,*,#24745,.F.);
#30655=ORIENTED_EDGE('',*,*,#24747,.T.);
#30656=ORIENTED_EDGE('',*,*,#24748,.T.);
#30657=ORIENTED_EDGE('',*,*,#24749,.T.);
#30658=ORIENTED_EDGE('',*,*,#24750,.F.);
#30659=ORIENTED_EDGE('',*,*,#24749,.F.);
#30660=ORIENTED_EDGE('',*,*,#24751,.T.);
#30661=ORIENTED_EDGE('',*,*,#24752,.T.);
#30662=ORIENTED_EDGE('',*,*,#24753,.F.);
#30663=ORIENTED_EDGE('',*,*,#24752,.F.);
#30664=ORIENTED_EDGE('',*,*,#24754,.T.);
#30665=ORIENTED_EDGE('',*,*,#24755,.T.);
#30666=ORIENTED_EDGE('',*,*,#24756,.T.);
#30667=ORIENTED_EDGE('',*,*,#24757,.F.);
#30668=ORIENTED_EDGE('',*,*,#24756,.F.);
#30669=ORIENTED_EDGE('',*,*,#24758,.T.);
#30670=ORIENTED_EDGE('',*,*,#24759,.T.);
#30671=ORIENTED_EDGE('',*,*,#24760,.F.);
#30672=ORIENTED_EDGE('',*,*,#24759,.F.);
#30673=ORIENTED_EDGE('',*,*,#24761,.T.);
#30674=ORIENTED_EDGE('',*,*,#24762,.T.);
#30675=ORIENTED_EDGE('',*,*,#24763,.T.);
#30676=ORIENTED_EDGE('',*,*,#24764,.F.);
#30677=ORIENTED_EDGE('',*,*,#24763,.F.);
#30678=ORIENTED_EDGE('',*,*,#24765,.T.);
#30679=ORIENTED_EDGE('',*,*,#24766,.T.);
#30680=ORIENTED_EDGE('',*,*,#24767,.F.);
#30681=ORIENTED_EDGE('',*,*,#24766,.F.);
#30682=ORIENTED_EDGE('',*,*,#24768,.T.);
#30683=ORIENTED_EDGE('',*,*,#24769,.T.);
#30684=ORIENTED_EDGE('',*,*,#24770,.T.);
#30685=ORIENTED_EDGE('',*,*,#24771,.F.);
#30686=ORIENTED_EDGE('',*,*,#24770,.F.);
#30687=ORIENTED_EDGE('',*,*,#24772,.T.);
#30688=ORIENTED_EDGE('',*,*,#24773,.T.);
#30689=ORIENTED_EDGE('',*,*,#24774,.F.);
#30690=ORIENTED_EDGE('',*,*,#24773,.F.);
#30691=ORIENTED_EDGE('',*,*,#24775,.T.);
#30692=ORIENTED_EDGE('',*,*,#24776,.T.);
#30693=ORIENTED_EDGE('',*,*,#24777,.T.);
#30694=ORIENTED_EDGE('',*,*,#24778,.F.);
#30695=ORIENTED_EDGE('',*,*,#24777,.F.);
#30696=ORIENTED_EDGE('',*,*,#24779,.T.);
#30697=ORIENTED_EDGE('',*,*,#24780,.T.);
#30698=ORIENTED_EDGE('',*,*,#24781,.F.);
#30699=ORIENTED_EDGE('',*,*,#24780,.F.);
#30700=ORIENTED_EDGE('',*,*,#24782,.T.);
#30701=ORIENTED_EDGE('',*,*,#24783,.T.);
#30702=ORIENTED_EDGE('',*,*,#24784,.T.);
#30703=ORIENTED_EDGE('',*,*,#24785,.F.);
#30704=ORIENTED_EDGE('',*,*,#24784,.F.);
#30705=ORIENTED_EDGE('',*,*,#24786,.T.);
#30706=ORIENTED_EDGE('',*,*,#24787,.T.);
#30707=ORIENTED_EDGE('',*,*,#24788,.F.);
#30708=ORIENTED_EDGE('',*,*,#24787,.F.);
#30709=ORIENTED_EDGE('',*,*,#24789,.T.);
#30710=ORIENTED_EDGE('',*,*,#24790,.T.);
#30711=ORIENTED_EDGE('',*,*,#24791,.T.);
#30712=ORIENTED_EDGE('',*,*,#24792,.F.);
#30713=ORIENTED_EDGE('',*,*,#24791,.F.);
#30714=ORIENTED_EDGE('',*,*,#24793,.T.);
#30715=ORIENTED_EDGE('',*,*,#24794,.T.);
#30716=ORIENTED_EDGE('',*,*,#24795,.F.);
#30717=ORIENTED_EDGE('',*,*,#24794,.F.);
#30718=ORIENTED_EDGE('',*,*,#24796,.T.);
#30719=ORIENTED_EDGE('',*,*,#24797,.T.);
#30720=ORIENTED_EDGE('',*,*,#24798,.T.);
#30721=ORIENTED_EDGE('',*,*,#24799,.F.);
#30722=ORIENTED_EDGE('',*,*,#24798,.F.);
#30723=ORIENTED_EDGE('',*,*,#24800,.T.);
#30724=ORIENTED_EDGE('',*,*,#24801,.T.);
#30725=ORIENTED_EDGE('',*,*,#24802,.F.);
#30726=ORIENTED_EDGE('',*,*,#24801,.F.);
#30727=ORIENTED_EDGE('',*,*,#24803,.T.);
#30728=ORIENTED_EDGE('',*,*,#24804,.T.);
#30729=ORIENTED_EDGE('',*,*,#24805,.T.);
#30730=ORIENTED_EDGE('',*,*,#24806,.F.);
#30731=ORIENTED_EDGE('',*,*,#24805,.F.);
#30732=ORIENTED_EDGE('',*,*,#24807,.T.);
#30733=ORIENTED_EDGE('',*,*,#24808,.T.);
#30734=ORIENTED_EDGE('',*,*,#24809,.F.);
#30735=ORIENTED_EDGE('',*,*,#24808,.F.);
#30736=ORIENTED_EDGE('',*,*,#24810,.T.);
#30737=ORIENTED_EDGE('',*,*,#24811,.T.);
#30738=ORIENTED_EDGE('',*,*,#24812,.T.);
#30739=ORIENTED_EDGE('',*,*,#24813,.F.);
#30740=ORIENTED_EDGE('',*,*,#24812,.F.);
#30741=ORIENTED_EDGE('',*,*,#24814,.T.);
#30742=ORIENTED_EDGE('',*,*,#24815,.T.);
#30743=ORIENTED_EDGE('',*,*,#24816,.F.);
#30744=ORIENTED_EDGE('',*,*,#24815,.F.);
#30745=ORIENTED_EDGE('',*,*,#24817,.T.);
#30746=ORIENTED_EDGE('',*,*,#24818,.T.);
#30747=ORIENTED_EDGE('',*,*,#24819,.T.);
#30748=ORIENTED_EDGE('',*,*,#24820,.F.);
#30749=ORIENTED_EDGE('',*,*,#24819,.F.);
#30750=ORIENTED_EDGE('',*,*,#24821,.T.);
#30751=ORIENTED_EDGE('',*,*,#24822,.T.);
#30752=ORIENTED_EDGE('',*,*,#24823,.F.);
#30753=ORIENTED_EDGE('',*,*,#24822,.F.);
#30754=ORIENTED_EDGE('',*,*,#24824,.T.);
#30755=ORIENTED_EDGE('',*,*,#24825,.T.);
#30756=ORIENTED_EDGE('',*,*,#24826,.T.);
#30757=ORIENTED_EDGE('',*,*,#24827,.F.);
#30758=ORIENTED_EDGE('',*,*,#24826,.F.);
#30759=ORIENTED_EDGE('',*,*,#24828,.T.);
#30760=ORIENTED_EDGE('',*,*,#24829,.T.);
#30761=ORIENTED_EDGE('',*,*,#24830,.F.);
#30762=ORIENTED_EDGE('',*,*,#24829,.F.);
#30763=ORIENTED_EDGE('',*,*,#24831,.T.);
#30764=ORIENTED_EDGE('',*,*,#24832,.T.);
#30765=ORIENTED_EDGE('',*,*,#24833,.T.);
#30766=ORIENTED_EDGE('',*,*,#24834,.F.);
#30767=ORIENTED_EDGE('',*,*,#24833,.F.);
#30768=ORIENTED_EDGE('',*,*,#24835,.T.);
#30769=ORIENTED_EDGE('',*,*,#24836,.T.);
#30770=ORIENTED_EDGE('',*,*,#24837,.F.);
#30771=ORIENTED_EDGE('',*,*,#24836,.F.);
#30772=ORIENTED_EDGE('',*,*,#24838,.T.);
#30773=ORIENTED_EDGE('',*,*,#24839,.T.);
#30774=ORIENTED_EDGE('',*,*,#24840,.T.);
#30775=ORIENTED_EDGE('',*,*,#24841,.F.);
#30776=ORIENTED_EDGE('',*,*,#24840,.F.);
#30777=ORIENTED_EDGE('',*,*,#24842,.T.);
#30778=ORIENTED_EDGE('',*,*,#24843,.T.);
#30779=ORIENTED_EDGE('',*,*,#24844,.F.);
#30780=ORIENTED_EDGE('',*,*,#24843,.F.);
#30781=ORIENTED_EDGE('',*,*,#24845,.T.);
#30782=ORIENTED_EDGE('',*,*,#24846,.T.);
#30783=ORIENTED_EDGE('',*,*,#24847,.F.);
#30784=ORIENTED_EDGE('',*,*,#24846,.F.);
#30785=ORIENTED_EDGE('',*,*,#24848,.T.);
#30786=ORIENTED_EDGE('',*,*,#24849,.T.);
#30787=ORIENTED_EDGE('',*,*,#24850,.F.);
#30788=ORIENTED_EDGE('',*,*,#24849,.F.);
#30789=ORIENTED_EDGE('',*,*,#24851,.T.);
#30790=ORIENTED_EDGE('',*,*,#24852,.T.);
#30791=ORIENTED_EDGE('',*,*,#24853,.F.);
#30792=ORIENTED_EDGE('',*,*,#24852,.F.);
#30793=ORIENTED_EDGE('',*,*,#24854,.T.);
#30794=ORIENTED_EDGE('',*,*,#24855,.T.);
#30795=ORIENTED_EDGE('',*,*,#24856,.F.);
#30796=ORIENTED_EDGE('',*,*,#24855,.F.);
#30797=ORIENTED_EDGE('',*,*,#24857,.T.);
#30798=ORIENTED_EDGE('',*,*,#24858,.T.);
#30799=ORIENTED_EDGE('',*,*,#24859,.T.);
#30800=ORIENTED_EDGE('',*,*,#24860,.F.);
#30801=ORIENTED_EDGE('',*,*,#24859,.F.);
#30802=ORIENTED_EDGE('',*,*,#24861,.T.);
#30803=ORIENTED_EDGE('',*,*,#24862,.T.);
#30804=ORIENTED_EDGE('',*,*,#24863,.F.);
#30805=ORIENTED_EDGE('',*,*,#24862,.F.);
#30806=ORIENTED_EDGE('',*,*,#24864,.T.);
#30807=ORIENTED_EDGE('',*,*,#24865,.T.);
#30808=ORIENTED_EDGE('',*,*,#24866,.T.);
#30809=ORIENTED_EDGE('',*,*,#24867,.F.);
#30810=ORIENTED_EDGE('',*,*,#24866,.F.);
#30811=ORIENTED_EDGE('',*,*,#24868,.T.);
#30812=ORIENTED_EDGE('',*,*,#24869,.T.);
#30813=ORIENTED_EDGE('',*,*,#24870,.F.);
#30814=ORIENTED_EDGE('',*,*,#24869,.F.);
#30815=ORIENTED_EDGE('',*,*,#24871,.T.);
#30816=ORIENTED_EDGE('',*,*,#24872,.T.);
#30817=ORIENTED_EDGE('',*,*,#24873,.F.);
#30818=ORIENTED_EDGE('',*,*,#24872,.F.);
#30819=ORIENTED_EDGE('',*,*,#24874,.T.);
#30820=ORIENTED_EDGE('',*,*,#24875,.T.);
#30821=ORIENTED_EDGE('',*,*,#24876,.F.);
#30822=ORIENTED_EDGE('',*,*,#24875,.F.);
#30823=ORIENTED_EDGE('',*,*,#24877,.T.);
#30824=ORIENTED_EDGE('',*,*,#24878,.T.);
#30825=ORIENTED_EDGE('',*,*,#24879,.F.);
#30826=ORIENTED_EDGE('',*,*,#24878,.F.);
#30827=ORIENTED_EDGE('',*,*,#24880,.T.);
#30828=ORIENTED_EDGE('',*,*,#24881,.T.);
#30829=ORIENTED_EDGE('',*,*,#24882,.F.);
#30830=ORIENTED_EDGE('',*,*,#24881,.F.);
#30831=ORIENTED_EDGE('',*,*,#24883,.T.);
#30832=ORIENTED_EDGE('',*,*,#24884,.T.);
#30833=ORIENTED_EDGE('',*,*,#24885,.T.);
#30834=ORIENTED_EDGE('',*,*,#24886,.F.);
#30835=ORIENTED_EDGE('',*,*,#24885,.F.);
#30836=ORIENTED_EDGE('',*,*,#24887,.T.);
#30837=ORIENTED_EDGE('',*,*,#24888,.T.);
#30838=ORIENTED_EDGE('',*,*,#24889,.F.);
#30839=ORIENTED_EDGE('',*,*,#24888,.F.);
#30840=ORIENTED_EDGE('',*,*,#24890,.T.);
#30841=ORIENTED_EDGE('',*,*,#24891,.T.);
#30842=ORIENTED_EDGE('',*,*,#24892,.T.);
#30843=ORIENTED_EDGE('',*,*,#24893,.F.);
#30844=ORIENTED_EDGE('',*,*,#24892,.F.);
#30845=ORIENTED_EDGE('',*,*,#24894,.T.);
#30846=ORIENTED_EDGE('',*,*,#24895,.T.);
#30847=ORIENTED_EDGE('',*,*,#24896,.F.);
#30848=ORIENTED_EDGE('',*,*,#24895,.F.);
#30849=ORIENTED_EDGE('',*,*,#24897,.T.);
#30850=ORIENTED_EDGE('',*,*,#24898,.T.);
#30851=ORIENTED_EDGE('',*,*,#24899,.F.);
#30852=ORIENTED_EDGE('',*,*,#24898,.F.);
#30853=ORIENTED_EDGE('',*,*,#24900,.T.);
#30854=ORIENTED_EDGE('',*,*,#24901,.T.);
#30855=ORIENTED_EDGE('',*,*,#24902,.F.);
#30856=ORIENTED_EDGE('',*,*,#24901,.F.);
#30857=ORIENTED_EDGE('',*,*,#24903,.T.);
#30858=ORIENTED_EDGE('',*,*,#24904,.T.);
#30859=ORIENTED_EDGE('',*,*,#24905,.T.);
#30860=ORIENTED_EDGE('',*,*,#24906,.F.);
#30861=ORIENTED_EDGE('',*,*,#24905,.F.);
#30862=ORIENTED_EDGE('',*,*,#24907,.T.);
#30863=ORIENTED_EDGE('',*,*,#24908,.T.);
#30864=ORIENTED_EDGE('',*,*,#24909,.F.);
#30865=ORIENTED_EDGE('',*,*,#24908,.F.);
#30866=ORIENTED_EDGE('',*,*,#24910,.T.);
#30867=ORIENTED_EDGE('',*,*,#24911,.T.);
#30868=ORIENTED_EDGE('',*,*,#24912,.T.);
#30869=ORIENTED_EDGE('',*,*,#24913,.F.);
#30870=ORIENTED_EDGE('',*,*,#24912,.F.);
#30871=ORIENTED_EDGE('',*,*,#24914,.T.);
#30872=ORIENTED_EDGE('',*,*,#24915,.T.);
#30873=ORIENTED_EDGE('',*,*,#24916,.F.);
#30874=ORIENTED_EDGE('',*,*,#24915,.F.);
#30875=ORIENTED_EDGE('',*,*,#24917,.T.);
#30876=ORIENTED_EDGE('',*,*,#24918,.T.);
#30877=ORIENTED_EDGE('',*,*,#24919,.F.);
#30878=ORIENTED_EDGE('',*,*,#24918,.F.);
#30879=ORIENTED_EDGE('',*,*,#24920,.T.);
#30880=ORIENTED_EDGE('',*,*,#24921,.T.);
#30881=ORIENTED_EDGE('',*,*,#24922,.F.);
#30882=ORIENTED_EDGE('',*,*,#24921,.F.);
#30883=ORIENTED_EDGE('',*,*,#24923,.T.);
#30884=ORIENTED_EDGE('',*,*,#24924,.T.);
#30885=ORIENTED_EDGE('',*,*,#24925,.T.);
#30886=ORIENTED_EDGE('',*,*,#24926,.F.);
#30887=ORIENTED_EDGE('',*,*,#24925,.F.);
#30888=ORIENTED_EDGE('',*,*,#24927,.T.);
#30889=ORIENTED_EDGE('',*,*,#24928,.T.);
#30890=ORIENTED_EDGE('',*,*,#24929,.F.);
#30891=ORIENTED_EDGE('',*,*,#24928,.F.);
#30892=ORIENTED_EDGE('',*,*,#24930,.T.);
#30893=ORIENTED_EDGE('',*,*,#24931,.T.);
#30894=ORIENTED_EDGE('',*,*,#24932,.T.);
#30895=ORIENTED_EDGE('',*,*,#24933,.F.);
#30896=ORIENTED_EDGE('',*,*,#24932,.F.);
#30897=ORIENTED_EDGE('',*,*,#24934,.T.);
#30898=ORIENTED_EDGE('',*,*,#24935,.T.);
#30899=ORIENTED_EDGE('',*,*,#24936,.F.);
#30900=ORIENTED_EDGE('',*,*,#24935,.F.);
#30901=ORIENTED_EDGE('',*,*,#24937,.T.);
#30902=ORIENTED_EDGE('',*,*,#24938,.T.);
#30903=ORIENTED_EDGE('',*,*,#24939,.T.);
#30904=ORIENTED_EDGE('',*,*,#24940,.F.);
#30905=ORIENTED_EDGE('',*,*,#24939,.F.);
#30906=ORIENTED_EDGE('',*,*,#24941,.T.);
#30907=ORIENTED_EDGE('',*,*,#24942,.T.);
#30908=ORIENTED_EDGE('',*,*,#24943,.F.);
#30909=ORIENTED_EDGE('',*,*,#24942,.F.);
#30910=ORIENTED_EDGE('',*,*,#24944,.T.);
#30911=ORIENTED_EDGE('',*,*,#24945,.T.);
#30912=ORIENTED_EDGE('',*,*,#24946,.T.);
#30913=ORIENTED_EDGE('',*,*,#24947,.F.);
#30914=ORIENTED_EDGE('',*,*,#24946,.F.);
#30915=ORIENTED_EDGE('',*,*,#24948,.T.);
#30916=ORIENTED_EDGE('',*,*,#24949,.T.);
#30917=ORIENTED_EDGE('',*,*,#24950,.F.);
#30918=ORIENTED_EDGE('',*,*,#24949,.F.);
#30919=ORIENTED_EDGE('',*,*,#24951,.T.);
#30920=ORIENTED_EDGE('',*,*,#24952,.T.);
#30921=ORIENTED_EDGE('',*,*,#24953,.T.);
#30922=ORIENTED_EDGE('',*,*,#24954,.F.);
#30923=ORIENTED_EDGE('',*,*,#24953,.F.);
#30924=ORIENTED_EDGE('',*,*,#24955,.T.);
#30925=ORIENTED_EDGE('',*,*,#24956,.T.);
#30926=ORIENTED_EDGE('',*,*,#24957,.F.);
#30927=ORIENTED_EDGE('',*,*,#24956,.F.);
#30928=ORIENTED_EDGE('',*,*,#24958,.T.);
#30929=ORIENTED_EDGE('',*,*,#24959,.T.);
#30930=ORIENTED_EDGE('',*,*,#24960,.T.);
#30931=ORIENTED_EDGE('',*,*,#24961,.F.);
#30932=ORIENTED_EDGE('',*,*,#24960,.F.);
#30933=ORIENTED_EDGE('',*,*,#24962,.T.);
#30934=ORIENTED_EDGE('',*,*,#24963,.T.);
#30935=ORIENTED_EDGE('',*,*,#24964,.F.);
#30936=ORIENTED_EDGE('',*,*,#24963,.F.);
#30937=ORIENTED_EDGE('',*,*,#24965,.T.);
#30938=ORIENTED_EDGE('',*,*,#24966,.T.);
#30939=ORIENTED_EDGE('',*,*,#24967,.T.);
#30940=ORIENTED_EDGE('',*,*,#24968,.F.);
#30941=ORIENTED_EDGE('',*,*,#24967,.F.);
#30942=ORIENTED_EDGE('',*,*,#24969,.T.);
#30943=ORIENTED_EDGE('',*,*,#24970,.T.);
#30944=ORIENTED_EDGE('',*,*,#24971,.F.);
#30945=ORIENTED_EDGE('',*,*,#24970,.F.);
#30946=ORIENTED_EDGE('',*,*,#24972,.T.);
#30947=ORIENTED_EDGE('',*,*,#24973,.T.);
#30948=ORIENTED_EDGE('',*,*,#24974,.T.);
#30949=ORIENTED_EDGE('',*,*,#24975,.F.);
#30950=ORIENTED_EDGE('',*,*,#24974,.F.);
#30951=ORIENTED_EDGE('',*,*,#24976,.T.);
#30952=ORIENTED_EDGE('',*,*,#24977,.T.);
#30953=ORIENTED_EDGE('',*,*,#24978,.F.);
#30954=ORIENTED_EDGE('',*,*,#24977,.F.);
#30955=ORIENTED_EDGE('',*,*,#24979,.T.);
#30956=ORIENTED_EDGE('',*,*,#24980,.T.);
#30957=ORIENTED_EDGE('',*,*,#24981,.T.);
#30958=ORIENTED_EDGE('',*,*,#24982,.F.);
#30959=ORIENTED_EDGE('',*,*,#24981,.F.);
#30960=ORIENTED_EDGE('',*,*,#24983,.T.);
#30961=ORIENTED_EDGE('',*,*,#24984,.T.);
#30962=ORIENTED_EDGE('',*,*,#24985,.F.);
#30963=ORIENTED_EDGE('',*,*,#24984,.F.);
#30964=ORIENTED_EDGE('',*,*,#24986,.T.);
#30965=ORIENTED_EDGE('',*,*,#24987,.T.);
#30966=ORIENTED_EDGE('',*,*,#24988,.T.);
#30967=ORIENTED_EDGE('',*,*,#24989,.F.);
#30968=ORIENTED_EDGE('',*,*,#24988,.F.);
#30969=ORIENTED_EDGE('',*,*,#24990,.T.);
#30970=ORIENTED_EDGE('',*,*,#24991,.T.);
#30971=ORIENTED_EDGE('',*,*,#24992,.F.);
#30972=ORIENTED_EDGE('',*,*,#24991,.F.);
#30973=ORIENTED_EDGE('',*,*,#24993,.T.);
#30974=ORIENTED_EDGE('',*,*,#24994,.T.);
#30975=ORIENTED_EDGE('',*,*,#24995,.T.);
#30976=ORIENTED_EDGE('',*,*,#24996,.F.);
#30977=ORIENTED_EDGE('',*,*,#24995,.F.);
#30978=ORIENTED_EDGE('',*,*,#24997,.T.);
#30979=ORIENTED_EDGE('',*,*,#24998,.T.);
#30980=ORIENTED_EDGE('',*,*,#24999,.F.);
#30981=ORIENTED_EDGE('',*,*,#24998,.F.);
#30982=ORIENTED_EDGE('',*,*,#25000,.T.);
#30983=ORIENTED_EDGE('',*,*,#25001,.T.);
#30984=ORIENTED_EDGE('',*,*,#25002,.T.);
#30985=ORIENTED_EDGE('',*,*,#25003,.F.);
#30986=ORIENTED_EDGE('',*,*,#25002,.F.);
#30987=ORIENTED_EDGE('',*,*,#25004,.T.);
#30988=ORIENTED_EDGE('',*,*,#25005,.T.);
#30989=ORIENTED_EDGE('',*,*,#25006,.F.);
#30990=ORIENTED_EDGE('',*,*,#25005,.F.);
#30991=ORIENTED_EDGE('',*,*,#25007,.T.);
#30992=ORIENTED_EDGE('',*,*,#25008,.T.);
#30993=ORIENTED_EDGE('',*,*,#25009,.T.);
#30994=ORIENTED_EDGE('',*,*,#25010,.F.);
#30995=ORIENTED_EDGE('',*,*,#25009,.F.);
#30996=ORIENTED_EDGE('',*,*,#25011,.T.);
#30997=ORIENTED_EDGE('',*,*,#25012,.T.);
#30998=ORIENTED_EDGE('',*,*,#25013,.F.);
#30999=ORIENTED_EDGE('',*,*,#25012,.F.);
#31000=ORIENTED_EDGE('',*,*,#25014,.T.);
#31001=ORIENTED_EDGE('',*,*,#25015,.T.);
#31002=ORIENTED_EDGE('',*,*,#25016,.T.);
#31003=ORIENTED_EDGE('',*,*,#25017,.F.);
#31004=ORIENTED_EDGE('',*,*,#25016,.F.);
#31005=ORIENTED_EDGE('',*,*,#25018,.T.);
#31006=ORIENTED_EDGE('',*,*,#25019,.T.);
#31007=ORIENTED_EDGE('',*,*,#25020,.F.);
#31008=ORIENTED_EDGE('',*,*,#25019,.F.);
#31009=ORIENTED_EDGE('',*,*,#25021,.T.);
#31010=ORIENTED_EDGE('',*,*,#25022,.T.);
#31011=ORIENTED_EDGE('',*,*,#25023,.F.);
#31012=ORIENTED_EDGE('',*,*,#25022,.F.);
#31013=ORIENTED_EDGE('',*,*,#25024,.T.);
#31014=ORIENTED_EDGE('',*,*,#25025,.T.);
#31015=ORIENTED_EDGE('',*,*,#25026,.F.);
#31016=ORIENTED_EDGE('',*,*,#25025,.F.);
#31017=ORIENTED_EDGE('',*,*,#25027,.T.);
#31018=ORIENTED_EDGE('',*,*,#25028,.T.);
#31019=ORIENTED_EDGE('',*,*,#25029,.F.);
#31020=ORIENTED_EDGE('',*,*,#25028,.F.);
#31021=ORIENTED_EDGE('',*,*,#25030,.T.);
#31022=ORIENTED_EDGE('',*,*,#25031,.T.);
#31023=ORIENTED_EDGE('',*,*,#25032,.F.);
#31024=ORIENTED_EDGE('',*,*,#25031,.F.);
#31025=ORIENTED_EDGE('',*,*,#25033,.T.);
#31026=ORIENTED_EDGE('',*,*,#25034,.T.);
#31027=ORIENTED_EDGE('',*,*,#25035,.F.);
#31028=ORIENTED_EDGE('',*,*,#25034,.F.);
#31029=ORIENTED_EDGE('',*,*,#25036,.T.);
#31030=ORIENTED_EDGE('',*,*,#25037,.T.);
#31031=ORIENTED_EDGE('',*,*,#25038,.F.);
#31032=ORIENTED_EDGE('',*,*,#25037,.F.);
#31033=ORIENTED_EDGE('',*,*,#25039,.T.);
#31034=ORIENTED_EDGE('',*,*,#25040,.T.);
#31035=ORIENTED_EDGE('',*,*,#25041,.F.);
#31036=ORIENTED_EDGE('',*,*,#25040,.F.);
#31037=ORIENTED_EDGE('',*,*,#25042,.T.);
#31038=ORIENTED_EDGE('',*,*,#25043,.T.);
#31039=ORIENTED_EDGE('',*,*,#25044,.F.);
#31040=ORIENTED_EDGE('',*,*,#25043,.F.);
#31041=ORIENTED_EDGE('',*,*,#25045,.T.);
#31042=ORIENTED_EDGE('',*,*,#25046,.T.);
#31043=ORIENTED_EDGE('',*,*,#25047,.F.);
#31044=ORIENTED_EDGE('',*,*,#25046,.F.);
#31045=ORIENTED_EDGE('',*,*,#25048,.T.);
#31046=ORIENTED_EDGE('',*,*,#25049,.T.);
#31047=ORIENTED_EDGE('',*,*,#25050,.F.);
#31048=ORIENTED_EDGE('',*,*,#25049,.F.);
#31049=ORIENTED_EDGE('',*,*,#25051,.T.);
#31050=ORIENTED_EDGE('',*,*,#25052,.T.);
#31051=ORIENTED_EDGE('',*,*,#25053,.F.);
#31052=ORIENTED_EDGE('',*,*,#25052,.F.);
#31053=ORIENTED_EDGE('',*,*,#25054,.T.);
#31054=ORIENTED_EDGE('',*,*,#25055,.T.);
#31055=ORIENTED_EDGE('',*,*,#25056,.F.);
#31056=ORIENTED_EDGE('',*,*,#25055,.F.);
#31057=ORIENTED_EDGE('',*,*,#25057,.T.);
#31058=ORIENTED_EDGE('',*,*,#25058,.T.);
#31059=ORIENTED_EDGE('',*,*,#25059,.F.);
#31060=ORIENTED_EDGE('',*,*,#25058,.F.);
#31061=ORIENTED_EDGE('',*,*,#25060,.T.);
#31062=ORIENTED_EDGE('',*,*,#25061,.T.);
#31063=ORIENTED_EDGE('',*,*,#25062,.F.);
#31064=ORIENTED_EDGE('',*,*,#25061,.F.);
#31065=ORIENTED_EDGE('',*,*,#25063,.T.);
#31066=ORIENTED_EDGE('',*,*,#25064,.T.);
#31067=ORIENTED_EDGE('',*,*,#25065,.F.);
#31068=ORIENTED_EDGE('',*,*,#25064,.F.);
#31069=ORIENTED_EDGE('',*,*,#25066,.T.);
#31070=ORIENTED_EDGE('',*,*,#25067,.T.);
#31071=ORIENTED_EDGE('',*,*,#25068,.F.);
#31072=ORIENTED_EDGE('',*,*,#25069,.T.);
#31073=ORIENTED_EDGE('',*,*,#25070,.F.);
#31074=ORIENTED_EDGE('',*,*,#25067,.F.);
#31075=ORIENTED_EDGE('',*,*,#25071,.T.);
#31076=ORIENTED_EDGE('',*,*,#25072,.T.);
#31077=ORIENTED_EDGE('',*,*,#25073,.F.);
#31078=ORIENTED_EDGE('',*,*,#25072,.F.);
#31079=ORIENTED_EDGE('',*,*,#25074,.T.);
#31080=ORIENTED_EDGE('',*,*,#25075,.T.);
#31081=ORIENTED_EDGE('',*,*,#25076,.F.);
#31082=ORIENTED_EDGE('',*,*,#25075,.F.);
#31083=ORIENTED_EDGE('',*,*,#25077,.T.);
#31084=ORIENTED_EDGE('',*,*,#25078,.T.);
#31085=ORIENTED_EDGE('',*,*,#25079,.F.);
#31086=ORIENTED_EDGE('',*,*,#25078,.F.);
#31087=ORIENTED_EDGE('',*,*,#25080,.T.);
#31088=ORIENTED_EDGE('',*,*,#25081,.T.);
#31089=ORIENTED_EDGE('',*,*,#25082,.F.);
#31090=ORIENTED_EDGE('',*,*,#25081,.F.);
#31091=ORIENTED_EDGE('',*,*,#25083,.T.);
#31092=ORIENTED_EDGE('',*,*,#25084,.T.);
#31093=ORIENTED_EDGE('',*,*,#25085,.F.);
#31094=ORIENTED_EDGE('',*,*,#25084,.F.);
#31095=ORIENTED_EDGE('',*,*,#25086,.T.);
#31096=ORIENTED_EDGE('',*,*,#25087,.T.);
#31097=ORIENTED_EDGE('',*,*,#25088,.F.);
#31098=ORIENTED_EDGE('',*,*,#25087,.F.);
#31099=ORIENTED_EDGE('',*,*,#25089,.T.);
#31100=ORIENTED_EDGE('',*,*,#25090,.T.);
#31101=ORIENTED_EDGE('',*,*,#25091,.F.);
#31102=ORIENTED_EDGE('',*,*,#25090,.F.);
#31103=ORIENTED_EDGE('',*,*,#25092,.T.);
#31104=ORIENTED_EDGE('',*,*,#25093,.T.);
#31105=ORIENTED_EDGE('',*,*,#25094,.F.);
#31106=ORIENTED_EDGE('',*,*,#25093,.F.);
#31107=ORIENTED_EDGE('',*,*,#25095,.T.);
#31108=ORIENTED_EDGE('',*,*,#25096,.T.);
#31109=ORIENTED_EDGE('',*,*,#25097,.F.);
#31110=ORIENTED_EDGE('',*,*,#25096,.F.);
#31111=ORIENTED_EDGE('',*,*,#25098,.T.);
#31112=ORIENTED_EDGE('',*,*,#25099,.T.);
#31113=ORIENTED_EDGE('',*,*,#25100,.F.);
#31114=ORIENTED_EDGE('',*,*,#25099,.F.);
#31115=ORIENTED_EDGE('',*,*,#25101,.T.);
#31116=ORIENTED_EDGE('',*,*,#25102,.T.);
#31117=ORIENTED_EDGE('',*,*,#25103,.F.);
#31118=ORIENTED_EDGE('',*,*,#25102,.F.);
#31119=ORIENTED_EDGE('',*,*,#25104,.T.);
#31120=ORIENTED_EDGE('',*,*,#25105,.T.);
#31121=ORIENTED_EDGE('',*,*,#25106,.F.);
#31122=ORIENTED_EDGE('',*,*,#25105,.F.);
#31123=ORIENTED_EDGE('',*,*,#25107,.T.);
#31124=ORIENTED_EDGE('',*,*,#25108,.T.);
#31125=ORIENTED_EDGE('',*,*,#25109,.F.);
#31126=ORIENTED_EDGE('',*,*,#25108,.F.);
#31127=ORIENTED_EDGE('',*,*,#25110,.T.);
#31128=ORIENTED_EDGE('',*,*,#25111,.T.);
#31129=ORIENTED_EDGE('',*,*,#25112,.F.);
#31130=ORIENTED_EDGE('',*,*,#25111,.F.);
#31131=ORIENTED_EDGE('',*,*,#25113,.T.);
#31132=ORIENTED_EDGE('',*,*,#25114,.T.);
#31133=ORIENTED_EDGE('',*,*,#25115,.F.);
#31134=ORIENTED_EDGE('',*,*,#25114,.F.);
#31135=ORIENTED_EDGE('',*,*,#25116,.T.);
#31136=ORIENTED_EDGE('',*,*,#25117,.T.);
#31137=ORIENTED_EDGE('',*,*,#25118,.F.);
#31138=ORIENTED_EDGE('',*,*,#25117,.F.);
#31139=ORIENTED_EDGE('',*,*,#25119,.T.);
#31140=ORIENTED_EDGE('',*,*,#25120,.T.);
#31141=ORIENTED_EDGE('',*,*,#25121,.F.);
#31142=ORIENTED_EDGE('',*,*,#25120,.F.);
#31143=ORIENTED_EDGE('',*,*,#25122,.T.);
#31144=ORIENTED_EDGE('',*,*,#25123,.T.);
#31145=ORIENTED_EDGE('',*,*,#25124,.F.);
#31146=ORIENTED_EDGE('',*,*,#25125,.T.);
#31147=ORIENTED_EDGE('',*,*,#25126,.F.);
#31148=ORIENTED_EDGE('',*,*,#25123,.F.);
#31149=ORIENTED_EDGE('',*,*,#25127,.T.);
#31150=ORIENTED_EDGE('',*,*,#25128,.T.);
#31151=ORIENTED_EDGE('',*,*,#25129,.F.);
#31152=ORIENTED_EDGE('',*,*,#25128,.F.);
#31153=ORIENTED_EDGE('',*,*,#25130,.T.);
#31154=ORIENTED_EDGE('',*,*,#25131,.T.);
#31155=ORIENTED_EDGE('',*,*,#25132,.F.);
#31156=ORIENTED_EDGE('',*,*,#25131,.F.);
#31157=ORIENTED_EDGE('',*,*,#25133,.T.);
#31158=ORIENTED_EDGE('',*,*,#25134,.T.);
#31159=ORIENTED_EDGE('',*,*,#25135,.F.);
#31160=ORIENTED_EDGE('',*,*,#25134,.F.);
#31161=ORIENTED_EDGE('',*,*,#25136,.T.);
#31162=ORIENTED_EDGE('',*,*,#25137,.T.);
#31163=ORIENTED_EDGE('',*,*,#25138,.F.);
#31164=ORIENTED_EDGE('',*,*,#25137,.F.);
#31165=ORIENTED_EDGE('',*,*,#25139,.T.);
#31166=ORIENTED_EDGE('',*,*,#25140,.T.);
#31167=ORIENTED_EDGE('',*,*,#25141,.F.);
#31168=ORIENTED_EDGE('',*,*,#25140,.F.);
#31169=ORIENTED_EDGE('',*,*,#25142,.T.);
#31170=ORIENTED_EDGE('',*,*,#25143,.T.);
#31171=ORIENTED_EDGE('',*,*,#25144,.F.);
#31172=ORIENTED_EDGE('',*,*,#25143,.F.);
#31173=ORIENTED_EDGE('',*,*,#25145,.T.);
#31174=ORIENTED_EDGE('',*,*,#25146,.T.);
#31175=ORIENTED_EDGE('',*,*,#25147,.F.);
#31176=ORIENTED_EDGE('',*,*,#25146,.F.);
#31177=ORIENTED_EDGE('',*,*,#25148,.T.);
#31178=ORIENTED_EDGE('',*,*,#25149,.T.);
#31179=ORIENTED_EDGE('',*,*,#25150,.F.);
#31180=ORIENTED_EDGE('',*,*,#25149,.F.);
#31181=ORIENTED_EDGE('',*,*,#25151,.T.);
#31182=ORIENTED_EDGE('',*,*,#25152,.T.);
#31183=ORIENTED_EDGE('',*,*,#25153,.F.);
#31184=ORIENTED_EDGE('',*,*,#25152,.F.);
#31185=ORIENTED_EDGE('',*,*,#25154,.T.);
#31186=ORIENTED_EDGE('',*,*,#25155,.T.);
#31187=ORIENTED_EDGE('',*,*,#25156,.F.);
#31188=ORIENTED_EDGE('',*,*,#25155,.F.);
#31189=ORIENTED_EDGE('',*,*,#25157,.T.);
#31190=ORIENTED_EDGE('',*,*,#25158,.T.);
#31191=ORIENTED_EDGE('',*,*,#25159,.F.);
#31192=ORIENTED_EDGE('',*,*,#25158,.F.);
#31193=ORIENTED_EDGE('',*,*,#25160,.T.);
#31194=ORIENTED_EDGE('',*,*,#25161,.T.);
#31195=ORIENTED_EDGE('',*,*,#25162,.F.);
#31196=ORIENTED_EDGE('',*,*,#25161,.F.);
#31197=ORIENTED_EDGE('',*,*,#25163,.T.);
#31198=ORIENTED_EDGE('',*,*,#25164,.T.);
#31199=ORIENTED_EDGE('',*,*,#25165,.F.);
#31200=ORIENTED_EDGE('',*,*,#25164,.F.);
#31201=ORIENTED_EDGE('',*,*,#25166,.T.);
#31202=ORIENTED_EDGE('',*,*,#25167,.T.);
#31203=ORIENTED_EDGE('',*,*,#25168,.F.);
#31204=ORIENTED_EDGE('',*,*,#25167,.F.);
#31205=ORIENTED_EDGE('',*,*,#25169,.T.);
#31206=ORIENTED_EDGE('',*,*,#25170,.T.);
#31207=ORIENTED_EDGE('',*,*,#25171,.F.);
#31208=ORIENTED_EDGE('',*,*,#25170,.F.);
#31209=ORIENTED_EDGE('',*,*,#25172,.T.);
#31210=ORIENTED_EDGE('',*,*,#25173,.T.);
#31211=ORIENTED_EDGE('',*,*,#25174,.F.);
#31212=ORIENTED_EDGE('',*,*,#25175,.T.);
#31213=ORIENTED_EDGE('',*,*,#25176,.F.);
#31214=ORIENTED_EDGE('',*,*,#25173,.F.);
#31215=ORIENTED_EDGE('',*,*,#25177,.T.);
#31216=ORIENTED_EDGE('',*,*,#25178,.T.);
#31217=ORIENTED_EDGE('',*,*,#25179,.F.);
#31218=ORIENTED_EDGE('',*,*,#25178,.F.);
#31219=ORIENTED_EDGE('',*,*,#25180,.T.);
#31220=ORIENTED_EDGE('',*,*,#25181,.T.);
#31221=ORIENTED_EDGE('',*,*,#25182,.F.);
#31222=ORIENTED_EDGE('',*,*,#25181,.F.);
#31223=ORIENTED_EDGE('',*,*,#25183,.T.);
#31224=ORIENTED_EDGE('',*,*,#25184,.T.);
#31225=ORIENTED_EDGE('',*,*,#25185,.F.);
#31226=ORIENTED_EDGE('',*,*,#25184,.F.);
#31227=ORIENTED_EDGE('',*,*,#25186,.T.);
#31228=ORIENTED_EDGE('',*,*,#25187,.T.);
#31229=ORIENTED_EDGE('',*,*,#25188,.F.);
#31230=ORIENTED_EDGE('',*,*,#25187,.F.);
#31231=ORIENTED_EDGE('',*,*,#25189,.T.);
#31232=ORIENTED_EDGE('',*,*,#25190,.T.);
#31233=ORIENTED_EDGE('',*,*,#25191,.F.);
#31234=ORIENTED_EDGE('',*,*,#25190,.F.);
#31235=ORIENTED_EDGE('',*,*,#25192,.T.);
#31236=ORIENTED_EDGE('',*,*,#25193,.T.);
#31237=ORIENTED_EDGE('',*,*,#25194,.F.);
#31238=ORIENTED_EDGE('',*,*,#25193,.F.);
#31239=ORIENTED_EDGE('',*,*,#25195,.T.);
#31240=ORIENTED_EDGE('',*,*,#25196,.T.);
#31241=ORIENTED_EDGE('',*,*,#25197,.F.);
#31242=ORIENTED_EDGE('',*,*,#25196,.F.);
#31243=ORIENTED_EDGE('',*,*,#25198,.T.);
#31244=ORIENTED_EDGE('',*,*,#25199,.T.);
#31245=ORIENTED_EDGE('',*,*,#25200,.F.);
#31246=ORIENTED_EDGE('',*,*,#25199,.F.);
#31247=ORIENTED_EDGE('',*,*,#25201,.T.);
#31248=ORIENTED_EDGE('',*,*,#25202,.T.);
#31249=ORIENTED_EDGE('',*,*,#25203,.F.);
#31250=ORIENTED_EDGE('',*,*,#25202,.F.);
#31251=ORIENTED_EDGE('',*,*,#25204,.T.);
#31252=ORIENTED_EDGE('',*,*,#25205,.T.);
#31253=ORIENTED_EDGE('',*,*,#25206,.F.);
#31254=ORIENTED_EDGE('',*,*,#25205,.F.);
#31255=ORIENTED_EDGE('',*,*,#25207,.T.);
#31256=ORIENTED_EDGE('',*,*,#25208,.T.);
#31257=ORIENTED_EDGE('',*,*,#25209,.F.);
#31258=ORIENTED_EDGE('',*,*,#25208,.F.);
#31259=ORIENTED_EDGE('',*,*,#25210,.T.);
#31260=ORIENTED_EDGE('',*,*,#25211,.T.);
#31261=ORIENTED_EDGE('',*,*,#25212,.F.);
#31262=ORIENTED_EDGE('',*,*,#25211,.F.);
#31263=ORIENTED_EDGE('',*,*,#25213,.T.);
#31264=ORIENTED_EDGE('',*,*,#25214,.T.);
#31265=ORIENTED_EDGE('',*,*,#25215,.F.);
#31266=ORIENTED_EDGE('',*,*,#25214,.F.);
#31267=ORIENTED_EDGE('',*,*,#25216,.T.);
#31268=ORIENTED_EDGE('',*,*,#25217,.T.);
#31269=ORIENTED_EDGE('',*,*,#25218,.F.);
#31270=ORIENTED_EDGE('',*,*,#25217,.F.);
#31271=ORIENTED_EDGE('',*,*,#25219,.T.);
#31272=ORIENTED_EDGE('',*,*,#25220,.T.);
#31273=ORIENTED_EDGE('',*,*,#25221,.F.);
#31274=ORIENTED_EDGE('',*,*,#25220,.F.);
#31275=ORIENTED_EDGE('',*,*,#25222,.T.);
#31276=ORIENTED_EDGE('',*,*,#25223,.T.);
#31277=ORIENTED_EDGE('',*,*,#25224,.F.);
#31278=ORIENTED_EDGE('',*,*,#25223,.F.);
#31279=ORIENTED_EDGE('',*,*,#25225,.T.);
#31280=ORIENTED_EDGE('',*,*,#25226,.T.);
#31281=ORIENTED_EDGE('',*,*,#25227,.F.);
#31282=ORIENTED_EDGE('',*,*,#25226,.F.);
#31283=ORIENTED_EDGE('',*,*,#25228,.T.);
#31284=ORIENTED_EDGE('',*,*,#25229,.T.);
#31285=ORIENTED_EDGE('',*,*,#25230,.F.);
#31286=ORIENTED_EDGE('',*,*,#25231,.T.);
#31287=ORIENTED_EDGE('',*,*,#25232,.F.);
#31288=ORIENTED_EDGE('',*,*,#25229,.F.);
#31289=ORIENTED_EDGE('',*,*,#25233,.T.);
#31290=ORIENTED_EDGE('',*,*,#25234,.T.);
#31291=ORIENTED_EDGE('',*,*,#25235,.F.);
#31292=ORIENTED_EDGE('',*,*,#25234,.F.);
#31293=ORIENTED_EDGE('',*,*,#25236,.T.);
#31294=ORIENTED_EDGE('',*,*,#25237,.T.);
#31295=ORIENTED_EDGE('',*,*,#25238,.F.);
#31296=ORIENTED_EDGE('',*,*,#25237,.F.);
#31297=ORIENTED_EDGE('',*,*,#25239,.T.);
#31298=ORIENTED_EDGE('',*,*,#25240,.T.);
#31299=ORIENTED_EDGE('',*,*,#25241,.F.);
#31300=ORIENTED_EDGE('',*,*,#25240,.F.);
#31301=ORIENTED_EDGE('',*,*,#25242,.T.);
#31302=ORIENTED_EDGE('',*,*,#25243,.T.);
#31303=ORIENTED_EDGE('',*,*,#25244,.F.);
#31304=ORIENTED_EDGE('',*,*,#25243,.F.);
#31305=ORIENTED_EDGE('',*,*,#25245,.T.);
#31306=ORIENTED_EDGE('',*,*,#25246,.T.);
#31307=ORIENTED_EDGE('',*,*,#25247,.F.);
#31308=ORIENTED_EDGE('',*,*,#25246,.F.);
#31309=ORIENTED_EDGE('',*,*,#25248,.T.);
#31310=ORIENTED_EDGE('',*,*,#25249,.T.);
#31311=ORIENTED_EDGE('',*,*,#25250,.F.);
#31312=ORIENTED_EDGE('',*,*,#25249,.F.);
#31313=ORIENTED_EDGE('',*,*,#25251,.T.);
#31314=ORIENTED_EDGE('',*,*,#25252,.T.);
#31315=ORIENTED_EDGE('',*,*,#25253,.F.);
#31316=ORIENTED_EDGE('',*,*,#25252,.F.);
#31317=ORIENTED_EDGE('',*,*,#25254,.T.);
#31318=ORIENTED_EDGE('',*,*,#25255,.T.);
#31319=ORIENTED_EDGE('',*,*,#25256,.F.);
#31320=ORIENTED_EDGE('',*,*,#25255,.F.);
#31321=ORIENTED_EDGE('',*,*,#25257,.T.);
#31322=ORIENTED_EDGE('',*,*,#25258,.T.);
#31323=ORIENTED_EDGE('',*,*,#25259,.F.);
#31324=ORIENTED_EDGE('',*,*,#25258,.F.);
#31325=ORIENTED_EDGE('',*,*,#25260,.T.);
#31326=ORIENTED_EDGE('',*,*,#25261,.T.);
#31327=ORIENTED_EDGE('',*,*,#25262,.F.);
#31328=ORIENTED_EDGE('',*,*,#25261,.F.);
#31329=ORIENTED_EDGE('',*,*,#25263,.T.);
#31330=ORIENTED_EDGE('',*,*,#25264,.T.);
#31331=ORIENTED_EDGE('',*,*,#25265,.F.);
#31332=ORIENTED_EDGE('',*,*,#25264,.F.);
#31333=ORIENTED_EDGE('',*,*,#25266,.T.);
#31334=ORIENTED_EDGE('',*,*,#25267,.T.);
#31335=ORIENTED_EDGE('',*,*,#25268,.F.);
#31336=ORIENTED_EDGE('',*,*,#25267,.F.);
#31337=ORIENTED_EDGE('',*,*,#25269,.T.);
#31338=ORIENTED_EDGE('',*,*,#25270,.T.);
#31339=ORIENTED_EDGE('',*,*,#25271,.F.);
#31340=ORIENTED_EDGE('',*,*,#25270,.F.);
#31341=ORIENTED_EDGE('',*,*,#25272,.T.);
#31342=ORIENTED_EDGE('',*,*,#25273,.T.);
#31343=ORIENTED_EDGE('',*,*,#25274,.F.);
#31344=ORIENTED_EDGE('',*,*,#25273,.F.);
#31345=ORIENTED_EDGE('',*,*,#25275,.T.);
#31346=ORIENTED_EDGE('',*,*,#25276,.T.);
#31347=ORIENTED_EDGE('',*,*,#25277,.F.);
#31348=ORIENTED_EDGE('',*,*,#25276,.F.);
#31349=ORIENTED_EDGE('',*,*,#25278,.T.);
#31350=ORIENTED_EDGE('',*,*,#25279,.T.);
#31351=ORIENTED_EDGE('',*,*,#25280,.F.);
#31352=ORIENTED_EDGE('',*,*,#25279,.F.);
#31353=ORIENTED_EDGE('',*,*,#25281,.T.);
#31354=ORIENTED_EDGE('',*,*,#25282,.T.);
#31355=ORIENTED_EDGE('',*,*,#25283,.F.);
#31356=ORIENTED_EDGE('',*,*,#25282,.F.);
#31357=ORIENTED_EDGE('',*,*,#25284,.T.);
#31358=ORIENTED_EDGE('',*,*,#25285,.T.);
#31359=ORIENTED_EDGE('',*,*,#25286,.F.);
#31360=ORIENTED_EDGE('',*,*,#25287,.T.);
#31361=ORIENTED_EDGE('',*,*,#25288,.F.);
#31362=ORIENTED_EDGE('',*,*,#25285,.F.);
#31363=ORIENTED_EDGE('',*,*,#25289,.T.);
#31364=ORIENTED_EDGE('',*,*,#25290,.T.);
#31365=ORIENTED_EDGE('',*,*,#25291,.F.);
#31366=ORIENTED_EDGE('',*,*,#25290,.F.);
#31367=ORIENTED_EDGE('',*,*,#25292,.T.);
#31368=ORIENTED_EDGE('',*,*,#25293,.T.);
#31369=ORIENTED_EDGE('',*,*,#25294,.F.);
#31370=ORIENTED_EDGE('',*,*,#25293,.F.);
#31371=ORIENTED_EDGE('',*,*,#25295,.T.);
#31372=ORIENTED_EDGE('',*,*,#25296,.T.);
#31373=ORIENTED_EDGE('',*,*,#25297,.F.);
#31374=ORIENTED_EDGE('',*,*,#25296,.F.);
#31375=ORIENTED_EDGE('',*,*,#25298,.T.);
#31376=ORIENTED_EDGE('',*,*,#25299,.T.);
#31377=ORIENTED_EDGE('',*,*,#25300,.F.);
#31378=ORIENTED_EDGE('',*,*,#25299,.F.);
#31379=ORIENTED_EDGE('',*,*,#25301,.T.);
#31380=ORIENTED_EDGE('',*,*,#25302,.T.);
#31381=ORIENTED_EDGE('',*,*,#25303,.F.);
#31382=ORIENTED_EDGE('',*,*,#25302,.F.);
#31383=ORIENTED_EDGE('',*,*,#25304,.T.);
#31384=ORIENTED_EDGE('',*,*,#25305,.T.);
#31385=ORIENTED_EDGE('',*,*,#25306,.F.);
#31386=ORIENTED_EDGE('',*,*,#25305,.F.);
#31387=ORIENTED_EDGE('',*,*,#25307,.T.);
#31388=ORIENTED_EDGE('',*,*,#25308,.T.);
#31389=ORIENTED_EDGE('',*,*,#25309,.F.);
#31390=ORIENTED_EDGE('',*,*,#25308,.F.);
#31391=ORIENTED_EDGE('',*,*,#25310,.T.);
#31392=ORIENTED_EDGE('',*,*,#25311,.T.);
#31393=ORIENTED_EDGE('',*,*,#25312,.F.);
#31394=ORIENTED_EDGE('',*,*,#25311,.F.);
#31395=ORIENTED_EDGE('',*,*,#25313,.T.);
#31396=ORIENTED_EDGE('',*,*,#25314,.T.);
#31397=ORIENTED_EDGE('',*,*,#25315,.F.);
#31398=ORIENTED_EDGE('',*,*,#25314,.F.);
#31399=ORIENTED_EDGE('',*,*,#25316,.T.);
#31400=ORIENTED_EDGE('',*,*,#25317,.T.);
#31401=ORIENTED_EDGE('',*,*,#25318,.F.);
#31402=ORIENTED_EDGE('',*,*,#25317,.F.);
#31403=ORIENTED_EDGE('',*,*,#25319,.T.);
#31404=ORIENTED_EDGE('',*,*,#25320,.T.);
#31405=ORIENTED_EDGE('',*,*,#25321,.F.);
#31406=ORIENTED_EDGE('',*,*,#25320,.F.);
#31407=ORIENTED_EDGE('',*,*,#25322,.T.);
#31408=ORIENTED_EDGE('',*,*,#25323,.T.);
#31409=ORIENTED_EDGE('',*,*,#25324,.F.);
#31410=ORIENTED_EDGE('',*,*,#25323,.F.);
#31411=ORIENTED_EDGE('',*,*,#25325,.T.);
#31412=ORIENTED_EDGE('',*,*,#25326,.T.);
#31413=ORIENTED_EDGE('',*,*,#25327,.F.);
#31414=ORIENTED_EDGE('',*,*,#25326,.F.);
#31415=ORIENTED_EDGE('',*,*,#25328,.T.);
#31416=ORIENTED_EDGE('',*,*,#25329,.T.);
#31417=ORIENTED_EDGE('',*,*,#25330,.F.);
#31418=ORIENTED_EDGE('',*,*,#25329,.F.);
#31419=ORIENTED_EDGE('',*,*,#25331,.T.);
#31420=ORIENTED_EDGE('',*,*,#25332,.T.);
#31421=ORIENTED_EDGE('',*,*,#25333,.F.);
#31422=ORIENTED_EDGE('',*,*,#25332,.F.);
#31423=ORIENTED_EDGE('',*,*,#25334,.T.);
#31424=ORIENTED_EDGE('',*,*,#25335,.T.);
#31425=ORIENTED_EDGE('',*,*,#25336,.F.);
#31426=ORIENTED_EDGE('',*,*,#25335,.F.);
#31427=ORIENTED_EDGE('',*,*,#25337,.T.);
#31428=ORIENTED_EDGE('',*,*,#25338,.T.);
#31429=ORIENTED_EDGE('',*,*,#25339,.F.);
#31430=ORIENTED_EDGE('',*,*,#25338,.F.);
#31431=ORIENTED_EDGE('',*,*,#25340,.T.);
#31432=ORIENTED_EDGE('',*,*,#25341,.T.);
#31433=ORIENTED_EDGE('',*,*,#25342,.F.);
#31434=ORIENTED_EDGE('',*,*,#25343,.T.);
#31435=ORIENTED_EDGE('',*,*,#25344,.F.);
#31436=ORIENTED_EDGE('',*,*,#25341,.F.);
#31437=ORIENTED_EDGE('',*,*,#25345,.T.);
#31438=ORIENTED_EDGE('',*,*,#25346,.T.);
#31439=ORIENTED_EDGE('',*,*,#25347,.F.);
#31440=ORIENTED_EDGE('',*,*,#25346,.F.);
#31441=ORIENTED_EDGE('',*,*,#25348,.T.);
#31442=ORIENTED_EDGE('',*,*,#25349,.T.);
#31443=ORIENTED_EDGE('',*,*,#25350,.F.);
#31444=ORIENTED_EDGE('',*,*,#25349,.F.);
#31445=ORIENTED_EDGE('',*,*,#25351,.T.);
#31446=ORIENTED_EDGE('',*,*,#25352,.T.);
#31447=ORIENTED_EDGE('',*,*,#25353,.F.);
#31448=ORIENTED_EDGE('',*,*,#25352,.F.);
#31449=ORIENTED_EDGE('',*,*,#25354,.T.);
#31450=ORIENTED_EDGE('',*,*,#25355,.T.);
#31451=ORIENTED_EDGE('',*,*,#25356,.F.);
#31452=ORIENTED_EDGE('',*,*,#25355,.F.);
#31453=ORIENTED_EDGE('',*,*,#25357,.T.);
#31454=ORIENTED_EDGE('',*,*,#25358,.T.);
#31455=ORIENTED_EDGE('',*,*,#25359,.F.);
#31456=ORIENTED_EDGE('',*,*,#25358,.F.);
#31457=ORIENTED_EDGE('',*,*,#25360,.T.);
#31458=ORIENTED_EDGE('',*,*,#25361,.T.);
#31459=ORIENTED_EDGE('',*,*,#25362,.F.);
#31460=ORIENTED_EDGE('',*,*,#25361,.F.);
#31461=ORIENTED_EDGE('',*,*,#25363,.T.);
#31462=ORIENTED_EDGE('',*,*,#25364,.T.);
#31463=ORIENTED_EDGE('',*,*,#25365,.F.);
#31464=ORIENTED_EDGE('',*,*,#25364,.F.);
#31465=ORIENTED_EDGE('',*,*,#25366,.T.);
#31466=ORIENTED_EDGE('',*,*,#25367,.T.);
#31467=ORIENTED_EDGE('',*,*,#25368,.F.);
#31468=ORIENTED_EDGE('',*,*,#25367,.F.);
#31469=ORIENTED_EDGE('',*,*,#25369,.T.);
#31470=ORIENTED_EDGE('',*,*,#25370,.T.);
#31471=ORIENTED_EDGE('',*,*,#25371,.F.);
#31472=ORIENTED_EDGE('',*,*,#25370,.F.);
#31473=ORIENTED_EDGE('',*,*,#25372,.T.);
#31474=ORIENTED_EDGE('',*,*,#25373,.T.);
#31475=ORIENTED_EDGE('',*,*,#25374,.F.);
#31476=ORIENTED_EDGE('',*,*,#25373,.F.);
#31477=ORIENTED_EDGE('',*,*,#25375,.T.);
#31478=ORIENTED_EDGE('',*,*,#25376,.T.);
#31479=ORIENTED_EDGE('',*,*,#25377,.F.);
#31480=ORIENTED_EDGE('',*,*,#25376,.F.);
#31481=ORIENTED_EDGE('',*,*,#25378,.T.);
#31482=ORIENTED_EDGE('',*,*,#25379,.T.);
#31483=ORIENTED_EDGE('',*,*,#25380,.F.);
#31484=ORIENTED_EDGE('',*,*,#25379,.F.);
#31485=ORIENTED_EDGE('',*,*,#25381,.T.);
#31486=ORIENTED_EDGE('',*,*,#25382,.T.);
#31487=ORIENTED_EDGE('',*,*,#25383,.F.);
#31488=ORIENTED_EDGE('',*,*,#25382,.F.);
#31489=ORIENTED_EDGE('',*,*,#25384,.T.);
#31490=ORIENTED_EDGE('',*,*,#25385,.T.);
#31491=ORIENTED_EDGE('',*,*,#25386,.F.);
#31492=ORIENTED_EDGE('',*,*,#25385,.F.);
#31493=ORIENTED_EDGE('',*,*,#25387,.T.);
#31494=ORIENTED_EDGE('',*,*,#25388,.T.);
#31495=ORIENTED_EDGE('',*,*,#25389,.F.);
#31496=ORIENTED_EDGE('',*,*,#25388,.F.);
#31497=ORIENTED_EDGE('',*,*,#25390,.T.);
#31498=ORIENTED_EDGE('',*,*,#25391,.T.);
#31499=ORIENTED_EDGE('',*,*,#25392,.F.);
#31500=ORIENTED_EDGE('',*,*,#25391,.F.);
#31501=ORIENTED_EDGE('',*,*,#25393,.T.);
#31502=ORIENTED_EDGE('',*,*,#25394,.T.);
#31503=ORIENTED_EDGE('',*,*,#25395,.F.);
#31504=ORIENTED_EDGE('',*,*,#25394,.F.);
#31505=ORIENTED_EDGE('',*,*,#25396,.T.);
#31506=ORIENTED_EDGE('',*,*,#25397,.T.);
#31507=ORIENTED_EDGE('',*,*,#25398,.F.);
#31508=ORIENTED_EDGE('',*,*,#25399,.T.);
#31509=ORIENTED_EDGE('',*,*,#25400,.F.);
#31510=ORIENTED_EDGE('',*,*,#25397,.F.);
#31511=ORIENTED_EDGE('',*,*,#25401,.T.);
#31512=ORIENTED_EDGE('',*,*,#25402,.T.);
#31513=ORIENTED_EDGE('',*,*,#25403,.F.);
#31514=ORIENTED_EDGE('',*,*,#25402,.F.);
#31515=ORIENTED_EDGE('',*,*,#25404,.T.);
#31516=ORIENTED_EDGE('',*,*,#25405,.T.);
#31517=ORIENTED_EDGE('',*,*,#25406,.F.);
#31518=ORIENTED_EDGE('',*,*,#25405,.F.);
#31519=ORIENTED_EDGE('',*,*,#25407,.T.);
#31520=ORIENTED_EDGE('',*,*,#25408,.T.);
#31521=ORIENTED_EDGE('',*,*,#25409,.F.);
#31522=ORIENTED_EDGE('',*,*,#25408,.F.);
#31523=ORIENTED_EDGE('',*,*,#25410,.T.);
#31524=ORIENTED_EDGE('',*,*,#25411,.T.);
#31525=ORIENTED_EDGE('',*,*,#25412,.F.);
#31526=ORIENTED_EDGE('',*,*,#25411,.F.);
#31527=ORIENTED_EDGE('',*,*,#25413,.T.);
#31528=ORIENTED_EDGE('',*,*,#25414,.T.);
#31529=ORIENTED_EDGE('',*,*,#25415,.F.);
#31530=ORIENTED_EDGE('',*,*,#25414,.F.);
#31531=ORIENTED_EDGE('',*,*,#25416,.T.);
#31532=ORIENTED_EDGE('',*,*,#25417,.T.);
#31533=ORIENTED_EDGE('',*,*,#25418,.F.);
#31534=ORIENTED_EDGE('',*,*,#25417,.F.);
#31535=ORIENTED_EDGE('',*,*,#25419,.T.);
#31536=ORIENTED_EDGE('',*,*,#25420,.T.);
#31537=ORIENTED_EDGE('',*,*,#25421,.F.);
#31538=ORIENTED_EDGE('',*,*,#25420,.F.);
#31539=ORIENTED_EDGE('',*,*,#25422,.T.);
#31540=ORIENTED_EDGE('',*,*,#25423,.T.);
#31541=ORIENTED_EDGE('',*,*,#25424,.F.);
#31542=ORIENTED_EDGE('',*,*,#25423,.F.);
#31543=ORIENTED_EDGE('',*,*,#25425,.T.);
#31544=ORIENTED_EDGE('',*,*,#25426,.T.);
#31545=ORIENTED_EDGE('',*,*,#25427,.F.);
#31546=ORIENTED_EDGE('',*,*,#25426,.F.);
#31547=ORIENTED_EDGE('',*,*,#25428,.T.);
#31548=ORIENTED_EDGE('',*,*,#25429,.T.);
#31549=ORIENTED_EDGE('',*,*,#25430,.F.);
#31550=ORIENTED_EDGE('',*,*,#25429,.F.);
#31551=ORIENTED_EDGE('',*,*,#25431,.T.);
#31552=ORIENTED_EDGE('',*,*,#25432,.T.);
#31553=ORIENTED_EDGE('',*,*,#25433,.F.);
#31554=ORIENTED_EDGE('',*,*,#25432,.F.);
#31555=ORIENTED_EDGE('',*,*,#25434,.T.);
#31556=ORIENTED_EDGE('',*,*,#25435,.T.);
#31557=ORIENTED_EDGE('',*,*,#25436,.F.);
#31558=ORIENTED_EDGE('',*,*,#25435,.F.);
#31559=ORIENTED_EDGE('',*,*,#25437,.T.);
#31560=ORIENTED_EDGE('',*,*,#25438,.T.);
#31561=ORIENTED_EDGE('',*,*,#25439,.F.);
#31562=ORIENTED_EDGE('',*,*,#25438,.F.);
#31563=ORIENTED_EDGE('',*,*,#25440,.T.);
#31564=ORIENTED_EDGE('',*,*,#25441,.T.);
#31565=ORIENTED_EDGE('',*,*,#25442,.F.);
#31566=ORIENTED_EDGE('',*,*,#25441,.F.);
#31567=ORIENTED_EDGE('',*,*,#25443,.T.);
#31568=ORIENTED_EDGE('',*,*,#25444,.T.);
#31569=ORIENTED_EDGE('',*,*,#25445,.F.);
#31570=ORIENTED_EDGE('',*,*,#25444,.F.);
#31571=ORIENTED_EDGE('',*,*,#25446,.T.);
#31572=ORIENTED_EDGE('',*,*,#25447,.T.);
#31573=ORIENTED_EDGE('',*,*,#25448,.F.);
#31574=ORIENTED_EDGE('',*,*,#25449,.T.);
#31575=ORIENTED_EDGE('',*,*,#25450,.F.);
#31576=ORIENTED_EDGE('',*,*,#25447,.F.);
#31577=ORIENTED_EDGE('',*,*,#25451,.T.);
#31578=ORIENTED_EDGE('',*,*,#25452,.T.);
#31579=ORIENTED_EDGE('',*,*,#25453,.F.);
#31580=ORIENTED_EDGE('',*,*,#25452,.F.);
#31581=ORIENTED_EDGE('',*,*,#25454,.T.);
#31582=ORIENTED_EDGE('',*,*,#25455,.T.);
#31583=ORIENTED_EDGE('',*,*,#25456,.F.);
#31584=ORIENTED_EDGE('',*,*,#25455,.F.);
#31585=ORIENTED_EDGE('',*,*,#25457,.T.);
#31586=ORIENTED_EDGE('',*,*,#25458,.T.);
#31587=ORIENTED_EDGE('',*,*,#25459,.F.);
#31588=ORIENTED_EDGE('',*,*,#25458,.F.);
#31589=ORIENTED_EDGE('',*,*,#25460,.T.);
#31590=ORIENTED_EDGE('',*,*,#25461,.T.);
#31591=ORIENTED_EDGE('',*,*,#25462,.F.);
#31592=ORIENTED_EDGE('',*,*,#25461,.F.);
#31593=ORIENTED_EDGE('',*,*,#25463,.T.);
#31594=ORIENTED_EDGE('',*,*,#25464,.T.);
#31595=ORIENTED_EDGE('',*,*,#25465,.F.);
#31596=ORIENTED_EDGE('',*,*,#25464,.F.);
#31597=ORIENTED_EDGE('',*,*,#25466,.T.);
#31598=ORIENTED_EDGE('',*,*,#25467,.T.);
#31599=ORIENTED_EDGE('',*,*,#25468,.F.);
#31600=ORIENTED_EDGE('',*,*,#25467,.F.);
#31601=ORIENTED_EDGE('',*,*,#25469,.T.);
#31602=ORIENTED_EDGE('',*,*,#25470,.T.);
#31603=ORIENTED_EDGE('',*,*,#25471,.F.);
#31604=ORIENTED_EDGE('',*,*,#25470,.F.);
#31605=ORIENTED_EDGE('',*,*,#25472,.T.);
#31606=ORIENTED_EDGE('',*,*,#25473,.T.);
#31607=ORIENTED_EDGE('',*,*,#25474,.F.);
#31608=ORIENTED_EDGE('',*,*,#25473,.F.);
#31609=ORIENTED_EDGE('',*,*,#25475,.T.);
#31610=ORIENTED_EDGE('',*,*,#25476,.T.);
#31611=ORIENTED_EDGE('',*,*,#25477,.F.);
#31612=ORIENTED_EDGE('',*,*,#25476,.F.);
#31613=ORIENTED_EDGE('',*,*,#25478,.T.);
#31614=ORIENTED_EDGE('',*,*,#25479,.T.);
#31615=ORIENTED_EDGE('',*,*,#25480,.F.);
#31616=ORIENTED_EDGE('',*,*,#25479,.F.);
#31617=ORIENTED_EDGE('',*,*,#25481,.T.);
#31618=ORIENTED_EDGE('',*,*,#25482,.T.);
#31619=ORIENTED_EDGE('',*,*,#25483,.F.);
#31620=ORIENTED_EDGE('',*,*,#25482,.F.);
#31621=ORIENTED_EDGE('',*,*,#25484,.T.);
#31622=ORIENTED_EDGE('',*,*,#25485,.T.);
#31623=ORIENTED_EDGE('',*,*,#25486,.F.);
#31624=ORIENTED_EDGE('',*,*,#25485,.F.);
#31625=ORIENTED_EDGE('',*,*,#25487,.T.);
#31626=ORIENTED_EDGE('',*,*,#25488,.T.);
#31627=ORIENTED_EDGE('',*,*,#25489,.F.);
#31628=ORIENTED_EDGE('',*,*,#25488,.F.);
#31629=ORIENTED_EDGE('',*,*,#25490,.T.);
#31630=ORIENTED_EDGE('',*,*,#25491,.T.);
#31631=ORIENTED_EDGE('',*,*,#25492,.F.);
#31632=ORIENTED_EDGE('',*,*,#25491,.F.);
#31633=ORIENTED_EDGE('',*,*,#25493,.T.);
#31634=ORIENTED_EDGE('',*,*,#25494,.T.);
#31635=ORIENTED_EDGE('',*,*,#25495,.F.);
#31636=ORIENTED_EDGE('',*,*,#25494,.F.);
#31637=ORIENTED_EDGE('',*,*,#25496,.T.);
#31638=ORIENTED_EDGE('',*,*,#25497,.T.);
#31639=ORIENTED_EDGE('',*,*,#25498,.F.);
#31640=ORIENTED_EDGE('',*,*,#25497,.F.);
#31641=ORIENTED_EDGE('',*,*,#25499,.T.);
#31642=ORIENTED_EDGE('',*,*,#25500,.T.);
#31643=ORIENTED_EDGE('',*,*,#25501,.F.);
#31644=ORIENTED_EDGE('',*,*,#25500,.F.);
#31645=ORIENTED_EDGE('',*,*,#25502,.T.);
#31646=ORIENTED_EDGE('',*,*,#25503,.T.);
#31647=ORIENTED_EDGE('',*,*,#25504,.F.);
#31648=ORIENTED_EDGE('',*,*,#25505,.T.);
#31649=ORIENTED_EDGE('',*,*,#25506,.F.);
#31650=ORIENTED_EDGE('',*,*,#25503,.F.);
#31651=ORIENTED_EDGE('',*,*,#25507,.T.);
#31652=ORIENTED_EDGE('',*,*,#25508,.T.);
#31653=ORIENTED_EDGE('',*,*,#25509,.F.);
#31654=ORIENTED_EDGE('',*,*,#25508,.F.);
#31655=ORIENTED_EDGE('',*,*,#25510,.T.);
#31656=ORIENTED_EDGE('',*,*,#25511,.T.);
#31657=ORIENTED_EDGE('',*,*,#25512,.F.);
#31658=ORIENTED_EDGE('',*,*,#25511,.F.);
#31659=ORIENTED_EDGE('',*,*,#25513,.T.);
#31660=ORIENTED_EDGE('',*,*,#25514,.T.);
#31661=ORIENTED_EDGE('',*,*,#25515,.F.);
#31662=ORIENTED_EDGE('',*,*,#25514,.F.);
#31663=ORIENTED_EDGE('',*,*,#25516,.T.);
#31664=ORIENTED_EDGE('',*,*,#25517,.T.);
#31665=ORIENTED_EDGE('',*,*,#25518,.F.);
#31666=ORIENTED_EDGE('',*,*,#25517,.F.);
#31667=ORIENTED_EDGE('',*,*,#25519,.T.);
#31668=ORIENTED_EDGE('',*,*,#25520,.T.);
#31669=ORIENTED_EDGE('',*,*,#25521,.F.);
#31670=ORIENTED_EDGE('',*,*,#25520,.F.);
#31671=ORIENTED_EDGE('',*,*,#25522,.T.);
#31672=ORIENTED_EDGE('',*,*,#25523,.T.);
#31673=ORIENTED_EDGE('',*,*,#25524,.F.);
#31674=ORIENTED_EDGE('',*,*,#25523,.F.);
#31675=ORIENTED_EDGE('',*,*,#25525,.T.);
#31676=ORIENTED_EDGE('',*,*,#25526,.T.);
#31677=ORIENTED_EDGE('',*,*,#25527,.F.);
#31678=ORIENTED_EDGE('',*,*,#25526,.F.);
#31679=ORIENTED_EDGE('',*,*,#25528,.T.);
#31680=ORIENTED_EDGE('',*,*,#25529,.T.);
#31681=ORIENTED_EDGE('',*,*,#25530,.F.);
#31682=ORIENTED_EDGE('',*,*,#25529,.F.);
#31683=ORIENTED_EDGE('',*,*,#25531,.T.);
#31684=ORIENTED_EDGE('',*,*,#25532,.T.);
#31685=ORIENTED_EDGE('',*,*,#25533,.F.);
#31686=ORIENTED_EDGE('',*,*,#25532,.F.);
#31687=ORIENTED_EDGE('',*,*,#25534,.T.);
#31688=ORIENTED_EDGE('',*,*,#25535,.T.);
#31689=ORIENTED_EDGE('',*,*,#25536,.F.);
#31690=ORIENTED_EDGE('',*,*,#25535,.F.);
#31691=ORIENTED_EDGE('',*,*,#25537,.T.);
#31692=ORIENTED_EDGE('',*,*,#25538,.T.);
#31693=ORIENTED_EDGE('',*,*,#25539,.F.);
#31694=ORIENTED_EDGE('',*,*,#25538,.F.);
#31695=ORIENTED_EDGE('',*,*,#25540,.T.);
#31696=ORIENTED_EDGE('',*,*,#25541,.T.);
#31697=ORIENTED_EDGE('',*,*,#25542,.F.);
#31698=ORIENTED_EDGE('',*,*,#25541,.F.);
#31699=ORIENTED_EDGE('',*,*,#25543,.T.);
#31700=ORIENTED_EDGE('',*,*,#25544,.T.);
#31701=ORIENTED_EDGE('',*,*,#25545,.F.);
#31702=ORIENTED_EDGE('',*,*,#25544,.F.);
#31703=ORIENTED_EDGE('',*,*,#25546,.T.);
#31704=ORIENTED_EDGE('',*,*,#25547,.T.);
#31705=ORIENTED_EDGE('',*,*,#25548,.F.);
#31706=ORIENTED_EDGE('',*,*,#25547,.F.);
#31707=ORIENTED_EDGE('',*,*,#25549,.T.);
#31708=ORIENTED_EDGE('',*,*,#25550,.T.);
#31709=ORIENTED_EDGE('',*,*,#25551,.F.);
#31710=ORIENTED_EDGE('',*,*,#25550,.F.);
#31711=ORIENTED_EDGE('',*,*,#25552,.T.);
#31712=ORIENTED_EDGE('',*,*,#25553,.T.);
#31713=ORIENTED_EDGE('',*,*,#25554,.F.);
#31714=ORIENTED_EDGE('',*,*,#25553,.F.);
#31715=ORIENTED_EDGE('',*,*,#25555,.T.);
#31716=ORIENTED_EDGE('',*,*,#25556,.T.);
#31717=ORIENTED_EDGE('',*,*,#25557,.F.);
#31718=ORIENTED_EDGE('',*,*,#25556,.F.);
#31719=ORIENTED_EDGE('',*,*,#25558,.T.);
#31720=ORIENTED_EDGE('',*,*,#25559,.T.);
#31721=ORIENTED_EDGE('',*,*,#25560,.F.);
#31722=ORIENTED_EDGE('',*,*,#25561,.T.);
#31723=ORIENTED_EDGE('',*,*,#25562,.F.);
#31724=ORIENTED_EDGE('',*,*,#25559,.F.);
#31725=ORIENTED_EDGE('',*,*,#25563,.T.);
#31726=ORIENTED_EDGE('',*,*,#25564,.T.);
#31727=ORIENTED_EDGE('',*,*,#25565,.F.);
#31728=ORIENTED_EDGE('',*,*,#25564,.F.);
#31729=ORIENTED_EDGE('',*,*,#25566,.T.);
#31730=ORIENTED_EDGE('',*,*,#25567,.T.);
#31731=ORIENTED_EDGE('',*,*,#25568,.F.);
#31732=ORIENTED_EDGE('',*,*,#25567,.F.);
#31733=ORIENTED_EDGE('',*,*,#25569,.T.);
#31734=ORIENTED_EDGE('',*,*,#25570,.T.);
#31735=ORIENTED_EDGE('',*,*,#25571,.F.);
#31736=ORIENTED_EDGE('',*,*,#25570,.F.);
#31737=ORIENTED_EDGE('',*,*,#25572,.T.);
#31738=ORIENTED_EDGE('',*,*,#25573,.T.);
#31739=ORIENTED_EDGE('',*,*,#25574,.F.);
#31740=ORIENTED_EDGE('',*,*,#25573,.F.);
#31741=ORIENTED_EDGE('',*,*,#25575,.T.);
#31742=ORIENTED_EDGE('',*,*,#25576,.T.);
#31743=ORIENTED_EDGE('',*,*,#25577,.F.);
#31744=ORIENTED_EDGE('',*,*,#25576,.F.);
#31745=ORIENTED_EDGE('',*,*,#25578,.T.);
#31746=ORIENTED_EDGE('',*,*,#25579,.T.);
#31747=ORIENTED_EDGE('',*,*,#25580,.F.);
#31748=ORIENTED_EDGE('',*,*,#25579,.F.);
#31749=ORIENTED_EDGE('',*,*,#25581,.T.);
#31750=ORIENTED_EDGE('',*,*,#25582,.T.);
#31751=ORIENTED_EDGE('',*,*,#25583,.F.);
#31752=ORIENTED_EDGE('',*,*,#25582,.F.);
#31753=ORIENTED_EDGE('',*,*,#25584,.T.);
#31754=ORIENTED_EDGE('',*,*,#25585,.T.);
#31755=ORIENTED_EDGE('',*,*,#25586,.F.);
#31756=ORIENTED_EDGE('',*,*,#25585,.F.);
#31757=ORIENTED_EDGE('',*,*,#25587,.T.);
#31758=ORIENTED_EDGE('',*,*,#25588,.T.);
#31759=ORIENTED_EDGE('',*,*,#25589,.F.);
#31760=ORIENTED_EDGE('',*,*,#25588,.F.);
#31761=ORIENTED_EDGE('',*,*,#25590,.T.);
#31762=ORIENTED_EDGE('',*,*,#25591,.T.);
#31763=ORIENTED_EDGE('',*,*,#25592,.F.);
#31764=ORIENTED_EDGE('',*,*,#25591,.F.);
#31765=ORIENTED_EDGE('',*,*,#25593,.T.);
#31766=ORIENTED_EDGE('',*,*,#25594,.T.);
#31767=ORIENTED_EDGE('',*,*,#25595,.F.);
#31768=ORIENTED_EDGE('',*,*,#25594,.F.);
#31769=ORIENTED_EDGE('',*,*,#25596,.T.);
#31770=ORIENTED_EDGE('',*,*,#25597,.T.);
#31771=ORIENTED_EDGE('',*,*,#25598,.F.);
#31772=ORIENTED_EDGE('',*,*,#25597,.F.);
#31773=ORIENTED_EDGE('',*,*,#25599,.T.);
#31774=ORIENTED_EDGE('',*,*,#25600,.T.);
#31775=ORIENTED_EDGE('',*,*,#25601,.F.);
#31776=ORIENTED_EDGE('',*,*,#25600,.F.);
#31777=ORIENTED_EDGE('',*,*,#25602,.T.);
#31778=ORIENTED_EDGE('',*,*,#25603,.T.);
#31779=ORIENTED_EDGE('',*,*,#25604,.F.);
#31780=ORIENTED_EDGE('',*,*,#25603,.F.);
#31781=ORIENTED_EDGE('',*,*,#25605,.T.);
#31782=ORIENTED_EDGE('',*,*,#25606,.T.);
#31783=ORIENTED_EDGE('',*,*,#25607,.F.);
#31784=ORIENTED_EDGE('',*,*,#25606,.F.);
#31785=ORIENTED_EDGE('',*,*,#25608,.T.);
#31786=ORIENTED_EDGE('',*,*,#25609,.T.);
#31787=ORIENTED_EDGE('',*,*,#25610,.F.);
#31788=ORIENTED_EDGE('',*,*,#25609,.F.);
#31789=ORIENTED_EDGE('',*,*,#25611,.T.);
#31790=ORIENTED_EDGE('',*,*,#25612,.T.);
#31791=ORIENTED_EDGE('',*,*,#25613,.F.);
#31792=ORIENTED_EDGE('',*,*,#25612,.F.);
#31793=ORIENTED_EDGE('',*,*,#25614,.T.);
#31794=ORIENTED_EDGE('',*,*,#25615,.T.);
#31795=ORIENTED_EDGE('',*,*,#25616,.F.);
#31796=ORIENTED_EDGE('',*,*,#25617,.T.);
#31797=ORIENTED_EDGE('',*,*,#25618,.F.);
#31798=ORIENTED_EDGE('',*,*,#25615,.F.);
#31799=ORIENTED_EDGE('',*,*,#25619,.T.);
#31800=ORIENTED_EDGE('',*,*,#25620,.T.);
#31801=ORIENTED_EDGE('',*,*,#25621,.F.);
#31802=ORIENTED_EDGE('',*,*,#25620,.F.);
#31803=ORIENTED_EDGE('',*,*,#25622,.T.);
#31804=ORIENTED_EDGE('',*,*,#25623,.T.);
#31805=ORIENTED_EDGE('',*,*,#25624,.F.);
#31806=ORIENTED_EDGE('',*,*,#25623,.F.);
#31807=ORIENTED_EDGE('',*,*,#25625,.T.);
#31808=ORIENTED_EDGE('',*,*,#25626,.T.);
#31809=ORIENTED_EDGE('',*,*,#25627,.F.);
#31810=ORIENTED_EDGE('',*,*,#25626,.F.);
#31811=ORIENTED_EDGE('',*,*,#25628,.T.);
#31812=ORIENTED_EDGE('',*,*,#25629,.T.);
#31813=ORIENTED_EDGE('',*,*,#25630,.F.);
#31814=ORIENTED_EDGE('',*,*,#25629,.F.);
#31815=ORIENTED_EDGE('',*,*,#25631,.T.);
#31816=ORIENTED_EDGE('',*,*,#25632,.T.);
#31817=ORIENTED_EDGE('',*,*,#25633,.F.);
#31818=ORIENTED_EDGE('',*,*,#25632,.F.);
#31819=ORIENTED_EDGE('',*,*,#25634,.T.);
#31820=ORIENTED_EDGE('',*,*,#25635,.T.);
#31821=ORIENTED_EDGE('',*,*,#25636,.F.);
#31822=ORIENTED_EDGE('',*,*,#25635,.F.);
#31823=ORIENTED_EDGE('',*,*,#25637,.T.);
#31824=ORIENTED_EDGE('',*,*,#25638,.T.);
#31825=ORIENTED_EDGE('',*,*,#25639,.F.);
#31826=ORIENTED_EDGE('',*,*,#25638,.F.);
#31827=ORIENTED_EDGE('',*,*,#25640,.T.);
#31828=ORIENTED_EDGE('',*,*,#25641,.T.);
#31829=ORIENTED_EDGE('',*,*,#25642,.F.);
#31830=ORIENTED_EDGE('',*,*,#25641,.F.);
#31831=ORIENTED_EDGE('',*,*,#25643,.T.);
#31832=ORIENTED_EDGE('',*,*,#25644,.T.);
#31833=ORIENTED_EDGE('',*,*,#25645,.F.);
#31834=ORIENTED_EDGE('',*,*,#25644,.F.);
#31835=ORIENTED_EDGE('',*,*,#25646,.T.);
#31836=ORIENTED_EDGE('',*,*,#25647,.T.);
#31837=ORIENTED_EDGE('',*,*,#25648,.F.);
#31838=ORIENTED_EDGE('',*,*,#25647,.F.);
#31839=ORIENTED_EDGE('',*,*,#25649,.T.);
#31840=ORIENTED_EDGE('',*,*,#25650,.T.);
#31841=ORIENTED_EDGE('',*,*,#25651,.F.);
#31842=ORIENTED_EDGE('',*,*,#25650,.F.);
#31843=ORIENTED_EDGE('',*,*,#25652,.T.);
#31844=ORIENTED_EDGE('',*,*,#25653,.T.);
#31845=ORIENTED_EDGE('',*,*,#25654,.F.);
#31846=ORIENTED_EDGE('',*,*,#25653,.F.);
#31847=ORIENTED_EDGE('',*,*,#25655,.T.);
#31848=ORIENTED_EDGE('',*,*,#25656,.T.);
#31849=ORIENTED_EDGE('',*,*,#25657,.F.);
#31850=ORIENTED_EDGE('',*,*,#25656,.F.);
#31851=ORIENTED_EDGE('',*,*,#25658,.T.);
#31852=ORIENTED_EDGE('',*,*,#25659,.T.);
#31853=ORIENTED_EDGE('',*,*,#25660,.F.);
#31854=ORIENTED_EDGE('',*,*,#25659,.F.);
#31855=ORIENTED_EDGE('',*,*,#25661,.T.);
#31856=ORIENTED_EDGE('',*,*,#25662,.T.);
#31857=ORIENTED_EDGE('',*,*,#25663,.F.);
#31858=ORIENTED_EDGE('',*,*,#25662,.F.);
#31859=ORIENTED_EDGE('',*,*,#25664,.T.);
#31860=ORIENTED_EDGE('',*,*,#25665,.T.);
#31861=ORIENTED_EDGE('',*,*,#25666,.F.);
#31862=ORIENTED_EDGE('',*,*,#25665,.F.);
#31863=ORIENTED_EDGE('',*,*,#25667,.T.);
#31864=ORIENTED_EDGE('',*,*,#25668,.T.);
#31865=ORIENTED_EDGE('',*,*,#25669,.F.);
#31866=ORIENTED_EDGE('',*,*,#25668,.F.);
#31867=ORIENTED_EDGE('',*,*,#25670,.T.);
#31868=ORIENTED_EDGE('',*,*,#25671,.T.);
#31869=ORIENTED_EDGE('',*,*,#25672,.F.);
#31870=ORIENTED_EDGE('',*,*,#25673,.T.);
#31871=ORIENTED_EDGE('',*,*,#25674,.F.);
#31872=ORIENTED_EDGE('',*,*,#25671,.F.);
#31873=ORIENTED_EDGE('',*,*,#25675,.T.);
#31874=ORIENTED_EDGE('',*,*,#25676,.T.);
#31875=ORIENTED_EDGE('',*,*,#25677,.F.);
#31876=ORIENTED_EDGE('',*,*,#25676,.F.);
#31877=ORIENTED_EDGE('',*,*,#25678,.T.);
#31878=ORIENTED_EDGE('',*,*,#25679,.T.);
#31879=ORIENTED_EDGE('',*,*,#25680,.F.);
#31880=ORIENTED_EDGE('',*,*,#25679,.F.);
#31881=ORIENTED_EDGE('',*,*,#25681,.T.);
#31882=ORIENTED_EDGE('',*,*,#25682,.T.);
#31883=ORIENTED_EDGE('',*,*,#25683,.F.);
#31884=ORIENTED_EDGE('',*,*,#25682,.F.);
#31885=ORIENTED_EDGE('',*,*,#25684,.T.);
#31886=ORIENTED_EDGE('',*,*,#25685,.T.);
#31887=ORIENTED_EDGE('',*,*,#25686,.F.);
#31888=ORIENTED_EDGE('',*,*,#25685,.F.);
#31889=ORIENTED_EDGE('',*,*,#25687,.T.);
#31890=ORIENTED_EDGE('',*,*,#25688,.T.);
#31891=ORIENTED_EDGE('',*,*,#25689,.F.);
#31892=ORIENTED_EDGE('',*,*,#25688,.F.);
#31893=ORIENTED_EDGE('',*,*,#25690,.T.);
#31894=ORIENTED_EDGE('',*,*,#25691,.T.);
#31895=ORIENTED_EDGE('',*,*,#25692,.F.);
#31896=ORIENTED_EDGE('',*,*,#25691,.F.);
#31897=ORIENTED_EDGE('',*,*,#25693,.T.);
#31898=ORIENTED_EDGE('',*,*,#25694,.T.);
#31899=ORIENTED_EDGE('',*,*,#25695,.F.);
#31900=ORIENTED_EDGE('',*,*,#25694,.F.);
#31901=ORIENTED_EDGE('',*,*,#25696,.T.);
#31902=ORIENTED_EDGE('',*,*,#25697,.T.);
#31903=ORIENTED_EDGE('',*,*,#25698,.F.);
#31904=ORIENTED_EDGE('',*,*,#25697,.F.);
#31905=ORIENTED_EDGE('',*,*,#25699,.T.);
#31906=ORIENTED_EDGE('',*,*,#25700,.T.);
#31907=ORIENTED_EDGE('',*,*,#25701,.F.);
#31908=ORIENTED_EDGE('',*,*,#25700,.F.);
#31909=ORIENTED_EDGE('',*,*,#25702,.T.);
#31910=ORIENTED_EDGE('',*,*,#25703,.T.);
#31911=ORIENTED_EDGE('',*,*,#25704,.F.);
#31912=ORIENTED_EDGE('',*,*,#25703,.F.);
#31913=ORIENTED_EDGE('',*,*,#25705,.T.);
#31914=ORIENTED_EDGE('',*,*,#25706,.T.);
#31915=ORIENTED_EDGE('',*,*,#25707,.F.);
#31916=ORIENTED_EDGE('',*,*,#25706,.F.);
#31917=ORIENTED_EDGE('',*,*,#25708,.T.);
#31918=ORIENTED_EDGE('',*,*,#25709,.T.);
#31919=ORIENTED_EDGE('',*,*,#25710,.F.);
#31920=ORIENTED_EDGE('',*,*,#25709,.F.);
#31921=ORIENTED_EDGE('',*,*,#25711,.T.);
#31922=ORIENTED_EDGE('',*,*,#25712,.T.);
#31923=ORIENTED_EDGE('',*,*,#25713,.F.);
#31924=ORIENTED_EDGE('',*,*,#25712,.F.);
#31925=ORIENTED_EDGE('',*,*,#25714,.T.);
#31926=ORIENTED_EDGE('',*,*,#25715,.T.);
#31927=ORIENTED_EDGE('',*,*,#25716,.F.);
#31928=ORIENTED_EDGE('',*,*,#25715,.F.);
#31929=ORIENTED_EDGE('',*,*,#25717,.T.);
#31930=ORIENTED_EDGE('',*,*,#25718,.T.);
#31931=ORIENTED_EDGE('',*,*,#25719,.F.);
#31932=ORIENTED_EDGE('',*,*,#25718,.F.);
#31933=ORIENTED_EDGE('',*,*,#25720,.T.);
#31934=ORIENTED_EDGE('',*,*,#25721,.T.);
#31935=ORIENTED_EDGE('',*,*,#25722,.F.);
#31936=ORIENTED_EDGE('',*,*,#25723,.T.);
#31937=ORIENTED_EDGE('',*,*,#25724,.F.);
#31938=ORIENTED_EDGE('',*,*,#25721,.F.);
#31939=ORIENTED_EDGE('',*,*,#25725,.T.);
#31940=ORIENTED_EDGE('',*,*,#25726,.T.);
#31941=ORIENTED_EDGE('',*,*,#25727,.F.);
#31942=ORIENTED_EDGE('',*,*,#25726,.F.);
#31943=ORIENTED_EDGE('',*,*,#25728,.T.);
#31944=ORIENTED_EDGE('',*,*,#25729,.T.);
#31945=ORIENTED_EDGE('',*,*,#25730,.F.);
#31946=ORIENTED_EDGE('',*,*,#25729,.F.);
#31947=ORIENTED_EDGE('',*,*,#25731,.T.);
#31948=ORIENTED_EDGE('',*,*,#25732,.T.);
#31949=ORIENTED_EDGE('',*,*,#25733,.F.);
#31950=ORIENTED_EDGE('',*,*,#25732,.F.);
#31951=ORIENTED_EDGE('',*,*,#25734,.T.);
#31952=ORIENTED_EDGE('',*,*,#25735,.T.);
#31953=ORIENTED_EDGE('',*,*,#25736,.F.);
#31954=ORIENTED_EDGE('',*,*,#25735,.F.);
#31955=ORIENTED_EDGE('',*,*,#25737,.T.);
#31956=ORIENTED_EDGE('',*,*,#25738,.T.);
#31957=ORIENTED_EDGE('',*,*,#25739,.F.);
#31958=ORIENTED_EDGE('',*,*,#25738,.F.);
#31959=ORIENTED_EDGE('',*,*,#25740,.T.);
#31960=ORIENTED_EDGE('',*,*,#25741,.T.);
#31961=ORIENTED_EDGE('',*,*,#25742,.F.);
#31962=ORIENTED_EDGE('',*,*,#25741,.F.);
#31963=ORIENTED_EDGE('',*,*,#25743,.T.);
#31964=ORIENTED_EDGE('',*,*,#25744,.T.);
#31965=ORIENTED_EDGE('',*,*,#25745,.F.);
#31966=ORIENTED_EDGE('',*,*,#25744,.F.);
#31967=ORIENTED_EDGE('',*,*,#25746,.T.);
#31968=ORIENTED_EDGE('',*,*,#25747,.T.);
#31969=ORIENTED_EDGE('',*,*,#25748,.F.);
#31970=ORIENTED_EDGE('',*,*,#25747,.F.);
#31971=ORIENTED_EDGE('',*,*,#25749,.T.);
#31972=ORIENTED_EDGE('',*,*,#25750,.T.);
#31973=ORIENTED_EDGE('',*,*,#25751,.F.);
#31974=ORIENTED_EDGE('',*,*,#25750,.F.);
#31975=ORIENTED_EDGE('',*,*,#25752,.T.);
#31976=ORIENTED_EDGE('',*,*,#25753,.T.);
#31977=ORIENTED_EDGE('',*,*,#25754,.F.);
#31978=ORIENTED_EDGE('',*,*,#25753,.F.);
#31979=ORIENTED_EDGE('',*,*,#25755,.T.);
#31980=ORIENTED_EDGE('',*,*,#25756,.T.);
#31981=ORIENTED_EDGE('',*,*,#25757,.F.);
#31982=ORIENTED_EDGE('',*,*,#25756,.F.);
#31983=ORIENTED_EDGE('',*,*,#25758,.T.);
#31984=ORIENTED_EDGE('',*,*,#25759,.T.);
#31985=ORIENTED_EDGE('',*,*,#25760,.F.);
#31986=ORIENTED_EDGE('',*,*,#25759,.F.);
#31987=ORIENTED_EDGE('',*,*,#25761,.T.);
#31988=ORIENTED_EDGE('',*,*,#25762,.T.);
#31989=ORIENTED_EDGE('',*,*,#25763,.F.);
#31990=ORIENTED_EDGE('',*,*,#25762,.F.);
#31991=ORIENTED_EDGE('',*,*,#25764,.T.);
#31992=ORIENTED_EDGE('',*,*,#25765,.T.);
#31993=ORIENTED_EDGE('',*,*,#25766,.F.);
#31994=ORIENTED_EDGE('',*,*,#25765,.F.);
#31995=ORIENTED_EDGE('',*,*,#25767,.T.);
#31996=ORIENTED_EDGE('',*,*,#25768,.T.);
#31997=ORIENTED_EDGE('',*,*,#25769,.F.);
#31998=ORIENTED_EDGE('',*,*,#25768,.F.);
#31999=ORIENTED_EDGE('',*,*,#25770,.T.);
#32000=ORIENTED_EDGE('',*,*,#25771,.T.);
#32001=ORIENTED_EDGE('',*,*,#25772,.F.);
#32002=ORIENTED_EDGE('',*,*,#25771,.F.);
#32003=ORIENTED_EDGE('',*,*,#25773,.T.);
#32004=ORIENTED_EDGE('',*,*,#25774,.T.);
#32005=ORIENTED_EDGE('',*,*,#25775,.F.);
#32006=ORIENTED_EDGE('',*,*,#25774,.F.);
#32007=ORIENTED_EDGE('',*,*,#25776,.T.);
#32008=ORIENTED_EDGE('',*,*,#25777,.T.);
#32009=ORIENTED_EDGE('',*,*,#25778,.F.);
#32010=ORIENTED_EDGE('',*,*,#25779,.T.);
#32011=ORIENTED_EDGE('',*,*,#25780,.F.);
#32012=ORIENTED_EDGE('',*,*,#25777,.F.);
#32013=ORIENTED_EDGE('',*,*,#25781,.T.);
#32014=ORIENTED_EDGE('',*,*,#25782,.T.);
#32015=ORIENTED_EDGE('',*,*,#25783,.F.);
#32016=ORIENTED_EDGE('',*,*,#25782,.F.);
#32017=ORIENTED_EDGE('',*,*,#25784,.T.);
#32018=ORIENTED_EDGE('',*,*,#25785,.T.);
#32019=ORIENTED_EDGE('',*,*,#25786,.F.);
#32020=ORIENTED_EDGE('',*,*,#25785,.F.);
#32021=ORIENTED_EDGE('',*,*,#25787,.T.);
#32022=ORIENTED_EDGE('',*,*,#25788,.T.);
#32023=ORIENTED_EDGE('',*,*,#25789,.F.);
#32024=ORIENTED_EDGE('',*,*,#25788,.F.);
#32025=ORIENTED_EDGE('',*,*,#25790,.T.);
#32026=ORIENTED_EDGE('',*,*,#25791,.T.);
#32027=ORIENTED_EDGE('',*,*,#25792,.F.);
#32028=ORIENTED_EDGE('',*,*,#25791,.F.);
#32029=ORIENTED_EDGE('',*,*,#25793,.T.);
#32030=ORIENTED_EDGE('',*,*,#25794,.T.);
#32031=ORIENTED_EDGE('',*,*,#25795,.F.);
#32032=ORIENTED_EDGE('',*,*,#25794,.F.);
#32033=ORIENTED_EDGE('',*,*,#25796,.T.);
#32034=ORIENTED_EDGE('',*,*,#25797,.T.);
#32035=ORIENTED_EDGE('',*,*,#25798,.F.);
#32036=ORIENTED_EDGE('',*,*,#25797,.F.);
#32037=ORIENTED_EDGE('',*,*,#25799,.T.);
#32038=ORIENTED_EDGE('',*,*,#25800,.T.);
#32039=ORIENTED_EDGE('',*,*,#25801,.F.);
#32040=ORIENTED_EDGE('',*,*,#25800,.F.);
#32041=ORIENTED_EDGE('',*,*,#25802,.T.);
#32042=ORIENTED_EDGE('',*,*,#25803,.T.);
#32043=ORIENTED_EDGE('',*,*,#25804,.F.);
#32044=ORIENTED_EDGE('',*,*,#25803,.F.);
#32045=ORIENTED_EDGE('',*,*,#25805,.T.);
#32046=ORIENTED_EDGE('',*,*,#25806,.T.);
#32047=ORIENTED_EDGE('',*,*,#25807,.F.);
#32048=ORIENTED_EDGE('',*,*,#25806,.F.);
#32049=ORIENTED_EDGE('',*,*,#25808,.T.);
#32050=ORIENTED_EDGE('',*,*,#25809,.T.);
#32051=ORIENTED_EDGE('',*,*,#25810,.F.);
#32052=ORIENTED_EDGE('',*,*,#25809,.F.);
#32053=ORIENTED_EDGE('',*,*,#25811,.T.);
#32054=ORIENTED_EDGE('',*,*,#25812,.T.);
#32055=ORIENTED_EDGE('',*,*,#25813,.F.);
#32056=ORIENTED_EDGE('',*,*,#25812,.F.);
#32057=ORIENTED_EDGE('',*,*,#25814,.T.);
#32058=ORIENTED_EDGE('',*,*,#25815,.T.);
#32059=ORIENTED_EDGE('',*,*,#25816,.F.);
#32060=ORIENTED_EDGE('',*,*,#25815,.F.);
#32061=ORIENTED_EDGE('',*,*,#25817,.T.);
#32062=ORIENTED_EDGE('',*,*,#25818,.T.);
#32063=ORIENTED_EDGE('',*,*,#25819,.F.);
#32064=ORIENTED_EDGE('',*,*,#25818,.F.);
#32065=ORIENTED_EDGE('',*,*,#25820,.T.);
#32066=ORIENTED_EDGE('',*,*,#25821,.T.);
#32067=ORIENTED_EDGE('',*,*,#25822,.F.);
#32068=ORIENTED_EDGE('',*,*,#25821,.F.);
#32069=ORIENTED_EDGE('',*,*,#25823,.T.);
#32070=ORIENTED_EDGE('',*,*,#25824,.T.);
#32071=ORIENTED_EDGE('',*,*,#25825,.F.);
#32072=ORIENTED_EDGE('',*,*,#25824,.F.);
#32073=ORIENTED_EDGE('',*,*,#25826,.T.);
#32074=ORIENTED_EDGE('',*,*,#25827,.T.);
#32075=ORIENTED_EDGE('',*,*,#25828,.F.);
#32076=ORIENTED_EDGE('',*,*,#25827,.F.);
#32077=ORIENTED_EDGE('',*,*,#25829,.T.);
#32078=ORIENTED_EDGE('',*,*,#25830,.T.);
#32079=ORIENTED_EDGE('',*,*,#25831,.F.);
#32080=ORIENTED_EDGE('',*,*,#25830,.F.);
#32081=ORIENTED_EDGE('',*,*,#25832,.T.);
#32082=ORIENTED_EDGE('',*,*,#25833,.T.);
#32083=ORIENTED_EDGE('',*,*,#25834,.F.);
#32084=ORIENTED_EDGE('',*,*,#25835,.T.);
#32085=ORIENTED_EDGE('',*,*,#25836,.F.);
#32086=ORIENTED_EDGE('',*,*,#25833,.F.);
#32087=ORIENTED_EDGE('',*,*,#25837,.T.);
#32088=ORIENTED_EDGE('',*,*,#25838,.T.);
#32089=ORIENTED_EDGE('',*,*,#25839,.F.);
#32090=ORIENTED_EDGE('',*,*,#25838,.F.);
#32091=ORIENTED_EDGE('',*,*,#25840,.T.);
#32092=ORIENTED_EDGE('',*,*,#25841,.T.);
#32093=ORIENTED_EDGE('',*,*,#25842,.F.);
#32094=ORIENTED_EDGE('',*,*,#25841,.F.);
#32095=ORIENTED_EDGE('',*,*,#25843,.T.);
#32096=ORIENTED_EDGE('',*,*,#25844,.T.);
#32097=ORIENTED_EDGE('',*,*,#25845,.F.);
#32098=ORIENTED_EDGE('',*,*,#25844,.F.);
#32099=ORIENTED_EDGE('',*,*,#25846,.T.);
#32100=ORIENTED_EDGE('',*,*,#25847,.T.);
#32101=ORIENTED_EDGE('',*,*,#25848,.F.);
#32102=ORIENTED_EDGE('',*,*,#25847,.F.);
#32103=ORIENTED_EDGE('',*,*,#25849,.T.);
#32104=ORIENTED_EDGE('',*,*,#25850,.T.);
#32105=ORIENTED_EDGE('',*,*,#25851,.F.);
#32106=ORIENTED_EDGE('',*,*,#25850,.F.);
#32107=ORIENTED_EDGE('',*,*,#25852,.T.);
#32108=ORIENTED_EDGE('',*,*,#25853,.T.);
#32109=ORIENTED_EDGE('',*,*,#25854,.F.);
#32110=ORIENTED_EDGE('',*,*,#25853,.F.);
#32111=ORIENTED_EDGE('',*,*,#25855,.T.);
#32112=ORIENTED_EDGE('',*,*,#25856,.T.);
#32113=ORIENTED_EDGE('',*,*,#25857,.F.);
#32114=ORIENTED_EDGE('',*,*,#25856,.F.);
#32115=ORIENTED_EDGE('',*,*,#25858,.T.);
#32116=ORIENTED_EDGE('',*,*,#25859,.T.);
#32117=ORIENTED_EDGE('',*,*,#25860,.F.);
#32118=ORIENTED_EDGE('',*,*,#25859,.F.);
#32119=ORIENTED_EDGE('',*,*,#25861,.T.);
#32120=ORIENTED_EDGE('',*,*,#25862,.T.);
#32121=ORIENTED_EDGE('',*,*,#25863,.F.);
#32122=ORIENTED_EDGE('',*,*,#25862,.F.);
#32123=ORIENTED_EDGE('',*,*,#25864,.T.);
#32124=ORIENTED_EDGE('',*,*,#25865,.T.);
#32125=ORIENTED_EDGE('',*,*,#25866,.F.);
#32126=ORIENTED_EDGE('',*,*,#25865,.F.);
#32127=ORIENTED_EDGE('',*,*,#25867,.T.);
#32128=ORIENTED_EDGE('',*,*,#25868,.T.);
#32129=ORIENTED_EDGE('',*,*,#25869,.F.);
#32130=ORIENTED_EDGE('',*,*,#25868,.F.);
#32131=ORIENTED_EDGE('',*,*,#25870,.T.);
#32132=ORIENTED_EDGE('',*,*,#25871,.T.);
#32133=ORIENTED_EDGE('',*,*,#25872,.F.);
#32134=ORIENTED_EDGE('',*,*,#25871,.F.);
#32135=ORIENTED_EDGE('',*,*,#25873,.T.);
#32136=ORIENTED_EDGE('',*,*,#25874,.T.);
#32137=ORIENTED_EDGE('',*,*,#25875,.F.);
#32138=ORIENTED_EDGE('',*,*,#25874,.F.);
#32139=ORIENTED_EDGE('',*,*,#25876,.T.);
#32140=ORIENTED_EDGE('',*,*,#25877,.T.);
#32141=ORIENTED_EDGE('',*,*,#25878,.F.);
#32142=ORIENTED_EDGE('',*,*,#25877,.F.);
#32143=ORIENTED_EDGE('',*,*,#25879,.T.);
#32144=ORIENTED_EDGE('',*,*,#25880,.T.);
#32145=ORIENTED_EDGE('',*,*,#25881,.F.);
#32146=ORIENTED_EDGE('',*,*,#25880,.F.);
#32147=ORIENTED_EDGE('',*,*,#25882,.T.);
#32148=ORIENTED_EDGE('',*,*,#25883,.T.);
#32149=ORIENTED_EDGE('',*,*,#25884,.F.);
#32150=ORIENTED_EDGE('',*,*,#25883,.F.);
#32151=ORIENTED_EDGE('',*,*,#25885,.T.);
#32152=ORIENTED_EDGE('',*,*,#25886,.T.);
#32153=ORIENTED_EDGE('',*,*,#25887,.F.);
#32154=ORIENTED_EDGE('',*,*,#25886,.F.);
#32155=ORIENTED_EDGE('',*,*,#25888,.T.);
#32156=ORIENTED_EDGE('',*,*,#25889,.T.);
#32157=ORIENTED_EDGE('',*,*,#25890,.F.);
#32158=ORIENTED_EDGE('',*,*,#25891,.T.);
#32159=ORIENTED_EDGE('',*,*,#25892,.F.);
#32160=ORIENTED_EDGE('',*,*,#25889,.F.);
#32161=ORIENTED_EDGE('',*,*,#25893,.T.);
#32162=ORIENTED_EDGE('',*,*,#25894,.T.);
#32163=ORIENTED_EDGE('',*,*,#25895,.F.);
#32164=ORIENTED_EDGE('',*,*,#25894,.F.);
#32165=ORIENTED_EDGE('',*,*,#25896,.T.);
#32166=ORIENTED_EDGE('',*,*,#25897,.T.);
#32167=ORIENTED_EDGE('',*,*,#25898,.F.);
#32168=ORIENTED_EDGE('',*,*,#25897,.F.);
#32169=ORIENTED_EDGE('',*,*,#25899,.T.);
#32170=ORIENTED_EDGE('',*,*,#25900,.T.);
#32171=ORIENTED_EDGE('',*,*,#25901,.F.);
#32172=ORIENTED_EDGE('',*,*,#25900,.F.);
#32173=ORIENTED_EDGE('',*,*,#25902,.T.);
#32174=ORIENTED_EDGE('',*,*,#25903,.T.);
#32175=ORIENTED_EDGE('',*,*,#25904,.F.);
#32176=ORIENTED_EDGE('',*,*,#25903,.F.);
#32177=ORIENTED_EDGE('',*,*,#25905,.T.);
#32178=ORIENTED_EDGE('',*,*,#25906,.T.);
#32179=ORIENTED_EDGE('',*,*,#25907,.F.);
#32180=ORIENTED_EDGE('',*,*,#25906,.F.);
#32181=ORIENTED_EDGE('',*,*,#25908,.T.);
#32182=ORIENTED_EDGE('',*,*,#25909,.T.);
#32183=ORIENTED_EDGE('',*,*,#25910,.F.);
#32184=ORIENTED_EDGE('',*,*,#25909,.F.);
#32185=ORIENTED_EDGE('',*,*,#25911,.T.);
#32186=ORIENTED_EDGE('',*,*,#25912,.T.);
#32187=ORIENTED_EDGE('',*,*,#25913,.F.);
#32188=ORIENTED_EDGE('',*,*,#25912,.F.);
#32189=ORIENTED_EDGE('',*,*,#25914,.T.);
#32190=ORIENTED_EDGE('',*,*,#25915,.T.);
#32191=ORIENTED_EDGE('',*,*,#25916,.F.);
#32192=ORIENTED_EDGE('',*,*,#25915,.F.);
#32193=ORIENTED_EDGE('',*,*,#25917,.T.);
#32194=ORIENTED_EDGE('',*,*,#25918,.T.);
#32195=ORIENTED_EDGE('',*,*,#25919,.F.);
#32196=ORIENTED_EDGE('',*,*,#25918,.F.);
#32197=ORIENTED_EDGE('',*,*,#25920,.T.);
#32198=ORIENTED_EDGE('',*,*,#25921,.T.);
#32199=ORIENTED_EDGE('',*,*,#25922,.F.);
#32200=ORIENTED_EDGE('',*,*,#25921,.F.);
#32201=ORIENTED_EDGE('',*,*,#25923,.T.);
#32202=ORIENTED_EDGE('',*,*,#25924,.T.);
#32203=ORIENTED_EDGE('',*,*,#25925,.F.);
#32204=ORIENTED_EDGE('',*,*,#25924,.F.);
#32205=ORIENTED_EDGE('',*,*,#25926,.T.);
#32206=ORIENTED_EDGE('',*,*,#25927,.T.);
#32207=ORIENTED_EDGE('',*,*,#25928,.F.);
#32208=ORIENTED_EDGE('',*,*,#25927,.F.);
#32209=ORIENTED_EDGE('',*,*,#25929,.T.);
#32210=ORIENTED_EDGE('',*,*,#25930,.T.);
#32211=ORIENTED_EDGE('',*,*,#25931,.F.);
#32212=ORIENTED_EDGE('',*,*,#25930,.F.);
#32213=ORIENTED_EDGE('',*,*,#25932,.T.);
#32214=ORIENTED_EDGE('',*,*,#25933,.T.);
#32215=ORIENTED_EDGE('',*,*,#25934,.F.);
#32216=ORIENTED_EDGE('',*,*,#25933,.F.);
#32217=ORIENTED_EDGE('',*,*,#25935,.T.);
#32218=ORIENTED_EDGE('',*,*,#25936,.T.);
#32219=ORIENTED_EDGE('',*,*,#25937,.F.);
#32220=ORIENTED_EDGE('',*,*,#25936,.F.);
#32221=ORIENTED_EDGE('',*,*,#25938,.T.);
#32222=ORIENTED_EDGE('',*,*,#25939,.T.);
#32223=ORIENTED_EDGE('',*,*,#25940,.F.);
#32224=ORIENTED_EDGE('',*,*,#25939,.F.);
#32225=ORIENTED_EDGE('',*,*,#25941,.T.);
#32226=ORIENTED_EDGE('',*,*,#25942,.T.);
#32227=ORIENTED_EDGE('',*,*,#25943,.F.);
#32228=ORIENTED_EDGE('',*,*,#25942,.F.);
#32229=ORIENTED_EDGE('',*,*,#25944,.T.);
#32230=ORIENTED_EDGE('',*,*,#25945,.T.);
#32231=ORIENTED_EDGE('',*,*,#25946,.F.);
#32232=ORIENTED_EDGE('',*,*,#25947,.T.);
#32233=ORIENTED_EDGE('',*,*,#25948,.F.);
#32234=ORIENTED_EDGE('',*,*,#25945,.F.);
#32235=ORIENTED_EDGE('',*,*,#25949,.T.);
#32236=ORIENTED_EDGE('',*,*,#25950,.T.);
#32237=ORIENTED_EDGE('',*,*,#25951,.F.);
#32238=ORIENTED_EDGE('',*,*,#25950,.F.);
#32239=ORIENTED_EDGE('',*,*,#25952,.T.);
#32240=ORIENTED_EDGE('',*,*,#25953,.T.);
#32241=ORIENTED_EDGE('',*,*,#25954,.F.);
#32242=ORIENTED_EDGE('',*,*,#25953,.F.);
#32243=ORIENTED_EDGE('',*,*,#25955,.T.);
#32244=ORIENTED_EDGE('',*,*,#25956,.T.);
#32245=ORIENTED_EDGE('',*,*,#25957,.F.);
#32246=ORIENTED_EDGE('',*,*,#25956,.F.);
#32247=ORIENTED_EDGE('',*,*,#25958,.T.);
#32248=ORIENTED_EDGE('',*,*,#25959,.T.);
#32249=ORIENTED_EDGE('',*,*,#25960,.F.);
#32250=ORIENTED_EDGE('',*,*,#25959,.F.);
#32251=ORIENTED_EDGE('',*,*,#25961,.T.);
#32252=ORIENTED_EDGE('',*,*,#25962,.T.);
#32253=ORIENTED_EDGE('',*,*,#25963,.F.);
#32254=ORIENTED_EDGE('',*,*,#25962,.F.);
#32255=ORIENTED_EDGE('',*,*,#25964,.T.);
#32256=ORIENTED_EDGE('',*,*,#25965,.T.);
#32257=ORIENTED_EDGE('',*,*,#25966,.F.);
#32258=ORIENTED_EDGE('',*,*,#25965,.F.);
#32259=ORIENTED_EDGE('',*,*,#25967,.T.);
#32260=ORIENTED_EDGE('',*,*,#25968,.T.);
#32261=ORIENTED_EDGE('',*,*,#25969,.F.);
#32262=ORIENTED_EDGE('',*,*,#25968,.F.);
#32263=ORIENTED_EDGE('',*,*,#25970,.T.);
#32264=ORIENTED_EDGE('',*,*,#25971,.T.);
#32265=ORIENTED_EDGE('',*,*,#25972,.F.);
#32266=ORIENTED_EDGE('',*,*,#25971,.F.);
#32267=ORIENTED_EDGE('',*,*,#25973,.T.);
#32268=ORIENTED_EDGE('',*,*,#25974,.T.);
#32269=ORIENTED_EDGE('',*,*,#25975,.F.);
#32270=ORIENTED_EDGE('',*,*,#25974,.F.);
#32271=ORIENTED_EDGE('',*,*,#25976,.T.);
#32272=ORIENTED_EDGE('',*,*,#25977,.T.);
#32273=ORIENTED_EDGE('',*,*,#25978,.F.);
#32274=ORIENTED_EDGE('',*,*,#25977,.F.);
#32275=ORIENTED_EDGE('',*,*,#25979,.T.);
#32276=ORIENTED_EDGE('',*,*,#25980,.T.);
#32277=ORIENTED_EDGE('',*,*,#25981,.F.);
#32278=ORIENTED_EDGE('',*,*,#25980,.F.);
#32279=ORIENTED_EDGE('',*,*,#25982,.T.);
#32280=ORIENTED_EDGE('',*,*,#25983,.T.);
#32281=ORIENTED_EDGE('',*,*,#25984,.F.);
#32282=ORIENTED_EDGE('',*,*,#25983,.F.);
#32283=ORIENTED_EDGE('',*,*,#25985,.T.);
#32284=ORIENTED_EDGE('',*,*,#25986,.T.);
#32285=ORIENTED_EDGE('',*,*,#25987,.F.);
#32286=ORIENTED_EDGE('',*,*,#25986,.F.);
#32287=ORIENTED_EDGE('',*,*,#25988,.T.);
#32288=ORIENTED_EDGE('',*,*,#25989,.T.);
#32289=ORIENTED_EDGE('',*,*,#25990,.F.);
#32290=ORIENTED_EDGE('',*,*,#25989,.F.);
#32291=ORIENTED_EDGE('',*,*,#25991,.T.);
#32292=ORIENTED_EDGE('',*,*,#25992,.T.);
#32293=ORIENTED_EDGE('',*,*,#25993,.F.);
#32294=ORIENTED_EDGE('',*,*,#25992,.F.);
#32295=ORIENTED_EDGE('',*,*,#25994,.T.);
#32296=ORIENTED_EDGE('',*,*,#25995,.T.);
#32297=ORIENTED_EDGE('',*,*,#25996,.F.);
#32298=ORIENTED_EDGE('',*,*,#25997,.T.);
#32299=ORIENTED_EDGE('',*,*,#25998,.F.);
#32300=ORIENTED_EDGE('',*,*,#25995,.F.);
#32301=ORIENTED_EDGE('',*,*,#25999,.T.);
#32302=ORIENTED_EDGE('',*,*,#26000,.T.);
#32303=ORIENTED_EDGE('',*,*,#26001,.F.);
#32304=ORIENTED_EDGE('',*,*,#26000,.F.);
#32305=ORIENTED_EDGE('',*,*,#26002,.T.);
#32306=ORIENTED_EDGE('',*,*,#26003,.T.);
#32307=ORIENTED_EDGE('',*,*,#26004,.F.);
#32308=ORIENTED_EDGE('',*,*,#26003,.F.);
#32309=ORIENTED_EDGE('',*,*,#26005,.T.);
#32310=ORIENTED_EDGE('',*,*,#26006,.T.);
#32311=ORIENTED_EDGE('',*,*,#26007,.F.);
#32312=ORIENTED_EDGE('',*,*,#26006,.F.);
#32313=ORIENTED_EDGE('',*,*,#26008,.T.);
#32314=ORIENTED_EDGE('',*,*,#26009,.T.);
#32315=ORIENTED_EDGE('',*,*,#26010,.F.);
#32316=ORIENTED_EDGE('',*,*,#26009,.F.);
#32317=ORIENTED_EDGE('',*,*,#26011,.T.);
#32318=ORIENTED_EDGE('',*,*,#26012,.T.);
#32319=ORIENTED_EDGE('',*,*,#26013,.F.);
#32320=ORIENTED_EDGE('',*,*,#26012,.F.);
#32321=ORIENTED_EDGE('',*,*,#26014,.T.);
#32322=ORIENTED_EDGE('',*,*,#26015,.T.);
#32323=ORIENTED_EDGE('',*,*,#26016,.F.);
#32324=ORIENTED_EDGE('',*,*,#26015,.F.);
#32325=ORIENTED_EDGE('',*,*,#26017,.T.);
#32326=ORIENTED_EDGE('',*,*,#26018,.T.);
#32327=ORIENTED_EDGE('',*,*,#26019,.F.);
#32328=ORIENTED_EDGE('',*,*,#26018,.F.);
#32329=ORIENTED_EDGE('',*,*,#26020,.T.);
#32330=ORIENTED_EDGE('',*,*,#26021,.T.);
#32331=ORIENTED_EDGE('',*,*,#26022,.F.);
#32332=ORIENTED_EDGE('',*,*,#26021,.F.);
#32333=ORIENTED_EDGE('',*,*,#26023,.T.);
#32334=ORIENTED_EDGE('',*,*,#26024,.T.);
#32335=ORIENTED_EDGE('',*,*,#26025,.F.);
#32336=ORIENTED_EDGE('',*,*,#26024,.F.);
#32337=ORIENTED_EDGE('',*,*,#26026,.T.);
#32338=ORIENTED_EDGE('',*,*,#26027,.T.);
#32339=ORIENTED_EDGE('',*,*,#26028,.F.);
#32340=ORIENTED_EDGE('',*,*,#26027,.F.);
#32341=ORIENTED_EDGE('',*,*,#26029,.T.);
#32342=ORIENTED_EDGE('',*,*,#26030,.T.);
#32343=ORIENTED_EDGE('',*,*,#26031,.F.);
#32344=ORIENTED_EDGE('',*,*,#26030,.F.);
#32345=ORIENTED_EDGE('',*,*,#26032,.T.);
#32346=ORIENTED_EDGE('',*,*,#26033,.T.);
#32347=ORIENTED_EDGE('',*,*,#26034,.F.);
#32348=ORIENTED_EDGE('',*,*,#26033,.F.);
#32349=ORIENTED_EDGE('',*,*,#26035,.T.);
#32350=ORIENTED_EDGE('',*,*,#26036,.T.);
#32351=ORIENTED_EDGE('',*,*,#26037,.F.);
#32352=ORIENTED_EDGE('',*,*,#26036,.F.);
#32353=ORIENTED_EDGE('',*,*,#26038,.T.);
#32354=ORIENTED_EDGE('',*,*,#26039,.T.);
#32355=ORIENTED_EDGE('',*,*,#26040,.F.);
#32356=ORIENTED_EDGE('',*,*,#26039,.F.);
#32357=ORIENTED_EDGE('',*,*,#26041,.T.);
#32358=ORIENTED_EDGE('',*,*,#26042,.T.);
#32359=ORIENTED_EDGE('',*,*,#26043,.F.);
#32360=ORIENTED_EDGE('',*,*,#26042,.F.);
#32361=ORIENTED_EDGE('',*,*,#26044,.T.);
#32362=ORIENTED_EDGE('',*,*,#26045,.T.);
#32363=ORIENTED_EDGE('',*,*,#26046,.F.);
#32364=ORIENTED_EDGE('',*,*,#26045,.F.);
#32365=ORIENTED_EDGE('',*,*,#26047,.T.);
#32366=ORIENTED_EDGE('',*,*,#26048,.T.);
#32367=ORIENTED_EDGE('',*,*,#26049,.F.);
#32368=ORIENTED_EDGE('',*,*,#26048,.F.);
#32369=ORIENTED_EDGE('',*,*,#26050,.T.);
#32370=ORIENTED_EDGE('',*,*,#26051,.T.);
#32371=ORIENTED_EDGE('',*,*,#26052,.T.);
#32372=ORIENTED_EDGE('',*,*,#26053,.F.);
#32373=ORIENTED_EDGE('',*,*,#26054,.T.);
#32374=ORIENTED_EDGE('',*,*,#26051,.F.);
#32375=ORIENTED_EDGE('',*,*,#26055,.T.);
#32376=ORIENTED_EDGE('',*,*,#26056,.T.);
#32377=ORIENTED_EDGE('',*,*,#26057,.F.);
#32378=ORIENTED_EDGE('',*,*,#26056,.F.);
#32379=ORIENTED_EDGE('',*,*,#26058,.T.);
#32380=ORIENTED_EDGE('',*,*,#26059,.T.);
#32381=ORIENTED_EDGE('',*,*,#26060,.F.);
#32382=ORIENTED_EDGE('',*,*,#26059,.F.);
#32383=ORIENTED_EDGE('',*,*,#26061,.T.);
#32384=ORIENTED_EDGE('',*,*,#26062,.T.);
#32385=ORIENTED_EDGE('',*,*,#26063,.F.);
#32386=ORIENTED_EDGE('',*,*,#26062,.F.);
#32387=ORIENTED_EDGE('',*,*,#26064,.T.);
#32388=ORIENTED_EDGE('',*,*,#26065,.T.);
#32389=ORIENTED_EDGE('',*,*,#26066,.F.);
#32390=ORIENTED_EDGE('',*,*,#26065,.F.);
#32391=ORIENTED_EDGE('',*,*,#26067,.T.);
#32392=ORIENTED_EDGE('',*,*,#26068,.T.);
#32393=ORIENTED_EDGE('',*,*,#26069,.F.);
#32394=ORIENTED_EDGE('',*,*,#26068,.F.);
#32395=ORIENTED_EDGE('',*,*,#26070,.T.);
#32396=ORIENTED_EDGE('',*,*,#26071,.T.);
#32397=ORIENTED_EDGE('',*,*,#26072,.F.);
#32398=ORIENTED_EDGE('',*,*,#26071,.F.);
#32399=ORIENTED_EDGE('',*,*,#26073,.T.);
#32400=ORIENTED_EDGE('',*,*,#26074,.T.);
#32401=ORIENTED_EDGE('',*,*,#26075,.F.);
#32402=ORIENTED_EDGE('',*,*,#26074,.F.);
#32403=ORIENTED_EDGE('',*,*,#26076,.T.);
#32404=ORIENTED_EDGE('',*,*,#26077,.T.);
#32405=ORIENTED_EDGE('',*,*,#26078,.F.);
#32406=ORIENTED_EDGE('',*,*,#26077,.F.);
#32407=ORIENTED_EDGE('',*,*,#26079,.T.);
#32408=ORIENTED_EDGE('',*,*,#26080,.T.);
#32409=ORIENTED_EDGE('',*,*,#26081,.F.);
#32410=ORIENTED_EDGE('',*,*,#26080,.F.);
#32411=ORIENTED_EDGE('',*,*,#26082,.T.);
#32412=ORIENTED_EDGE('',*,*,#26083,.T.);
#32413=ORIENTED_EDGE('',*,*,#26084,.F.);
#32414=ORIENTED_EDGE('',*,*,#26083,.F.);
#32415=ORIENTED_EDGE('',*,*,#26085,.T.);
#32416=ORIENTED_EDGE('',*,*,#26086,.T.);
#32417=ORIENTED_EDGE('',*,*,#26087,.F.);
#32418=ORIENTED_EDGE('',*,*,#26086,.F.);
#32419=ORIENTED_EDGE('',*,*,#26088,.T.);
#32420=ORIENTED_EDGE('',*,*,#26089,.T.);
#32421=ORIENTED_EDGE('',*,*,#26090,.F.);
#32422=ORIENTED_EDGE('',*,*,#26089,.F.);
#32423=ORIENTED_EDGE('',*,*,#26091,.T.);
#32424=ORIENTED_EDGE('',*,*,#26092,.T.);
#32425=ORIENTED_EDGE('',*,*,#26093,.F.);
#32426=ORIENTED_EDGE('',*,*,#26092,.F.);
#32427=ORIENTED_EDGE('',*,*,#26094,.T.);
#32428=ORIENTED_EDGE('',*,*,#26095,.T.);
#32429=ORIENTED_EDGE('',*,*,#26096,.F.);
#32430=ORIENTED_EDGE('',*,*,#26095,.F.);
#32431=ORIENTED_EDGE('',*,*,#26097,.T.);
#32432=ORIENTED_EDGE('',*,*,#26098,.T.);
#32433=ORIENTED_EDGE('',*,*,#26099,.F.);
#32434=ORIENTED_EDGE('',*,*,#26098,.F.);
#32435=ORIENTED_EDGE('',*,*,#26100,.T.);
#32436=ORIENTED_EDGE('',*,*,#26101,.T.);
#32437=ORIENTED_EDGE('',*,*,#26102,.T.);
#32438=ORIENTED_EDGE('',*,*,#26103,.F.);
#32439=ORIENTED_EDGE('',*,*,#26104,.T.);
#32440=ORIENTED_EDGE('',*,*,#26101,.F.);
#32441=ORIENTED_EDGE('',*,*,#26105,.T.);
#32442=ORIENTED_EDGE('',*,*,#26106,.T.);
#32443=ORIENTED_EDGE('',*,*,#26107,.F.);
#32444=ORIENTED_EDGE('',*,*,#26106,.F.);
#32445=ORIENTED_EDGE('',*,*,#26108,.T.);
#32446=ORIENTED_EDGE('',*,*,#26109,.T.);
#32447=ORIENTED_EDGE('',*,*,#26110,.T.);
#32448=ORIENTED_EDGE('',*,*,#26111,.F.);
#32449=ORIENTED_EDGE('',*,*,#26112,.T.);
#32450=ORIENTED_EDGE('',*,*,#26109,.F.);
#32451=ORIENTED_EDGE('',*,*,#26113,.T.);
#32452=ORIENTED_EDGE('',*,*,#26114,.T.);
#32453=ORIENTED_EDGE('',*,*,#26115,.F.);
#32454=ORIENTED_EDGE('',*,*,#26114,.F.);
#32455=ORIENTED_EDGE('',*,*,#26116,.T.);
#32456=ORIENTED_EDGE('',*,*,#26117,.T.);
#32457=ORIENTED_EDGE('',*,*,#26118,.F.);
#32458=ORIENTED_EDGE('',*,*,#26117,.F.);
#32459=ORIENTED_EDGE('',*,*,#26119,.T.);
#32460=ORIENTED_EDGE('',*,*,#26120,.T.);
#32461=ORIENTED_EDGE('',*,*,#26121,.F.);
#32462=ORIENTED_EDGE('',*,*,#26120,.F.);
#32463=ORIENTED_EDGE('',*,*,#26122,.T.);
#32464=ORIENTED_EDGE('',*,*,#26123,.T.);
#32465=ORIENTED_EDGE('',*,*,#26124,.F.);
#32466=ORIENTED_EDGE('',*,*,#26123,.F.);
#32467=ORIENTED_EDGE('',*,*,#26125,.T.);
#32468=ORIENTED_EDGE('',*,*,#26126,.T.);
#32469=ORIENTED_EDGE('',*,*,#26127,.F.);
#32470=ORIENTED_EDGE('',*,*,#26126,.F.);
#32471=ORIENTED_EDGE('',*,*,#26128,.T.);
#32472=ORIENTED_EDGE('',*,*,#26129,.T.);
#32473=ORIENTED_EDGE('',*,*,#26130,.F.);
#32474=ORIENTED_EDGE('',*,*,#26129,.F.);
#32475=ORIENTED_EDGE('',*,*,#26131,.T.);
#32476=ORIENTED_EDGE('',*,*,#26132,.T.);
#32477=ORIENTED_EDGE('',*,*,#26133,.F.);
#32478=ORIENTED_EDGE('',*,*,#26132,.F.);
#32479=ORIENTED_EDGE('',*,*,#26134,.T.);
#32480=ORIENTED_EDGE('',*,*,#26135,.T.);
#32481=ORIENTED_EDGE('',*,*,#26136,.F.);
#32482=ORIENTED_EDGE('',*,*,#26135,.F.);
#32483=ORIENTED_EDGE('',*,*,#26137,.T.);
#32484=ORIENTED_EDGE('',*,*,#26138,.T.);
#32485=ORIENTED_EDGE('',*,*,#26139,.F.);
#32486=ORIENTED_EDGE('',*,*,#26138,.F.);
#32487=ORIENTED_EDGE('',*,*,#26140,.T.);
#32488=ORIENTED_EDGE('',*,*,#26141,.T.);
#32489=ORIENTED_EDGE('',*,*,#26142,.F.);
#32490=ORIENTED_EDGE('',*,*,#26141,.F.);
#32491=ORIENTED_EDGE('',*,*,#26143,.T.);
#32492=ORIENTED_EDGE('',*,*,#26144,.T.);
#32493=ORIENTED_EDGE('',*,*,#26145,.F.);
#32494=ORIENTED_EDGE('',*,*,#26144,.F.);
#32495=ORIENTED_EDGE('',*,*,#26146,.T.);
#32496=ORIENTED_EDGE('',*,*,#26147,.T.);
#32497=ORIENTED_EDGE('',*,*,#26148,.F.);
#32498=ORIENTED_EDGE('',*,*,#26147,.F.);
#32499=ORIENTED_EDGE('',*,*,#26149,.T.);
#32500=ORIENTED_EDGE('',*,*,#26150,.T.);
#32501=ORIENTED_EDGE('',*,*,#26151,.F.);
#32502=ORIENTED_EDGE('',*,*,#26150,.F.);
#32503=ORIENTED_EDGE('',*,*,#26152,.T.);
#32504=ORIENTED_EDGE('',*,*,#26153,.T.);
#32505=ORIENTED_EDGE('',*,*,#26154,.T.);
#32506=ORIENTED_EDGE('',*,*,#26155,.F.);
#32507=ORIENTED_EDGE('',*,*,#26156,.T.);
#32508=ORIENTED_EDGE('',*,*,#26153,.F.);
#32509=ORIENTED_EDGE('',*,*,#26157,.T.);
#32510=ORIENTED_EDGE('',*,*,#26158,.T.);
#32511=ORIENTED_EDGE('',*,*,#26159,.F.);
#32512=ORIENTED_EDGE('',*,*,#26158,.F.);
#32513=ORIENTED_EDGE('',*,*,#26160,.T.);
#32514=ORIENTED_EDGE('',*,*,#26161,.T.);
#32515=ORIENTED_EDGE('',*,*,#26162,.F.);
#32516=ORIENTED_EDGE('',*,*,#26161,.F.);
#32517=ORIENTED_EDGE('',*,*,#26163,.T.);
#32518=ORIENTED_EDGE('',*,*,#26164,.T.);
#32519=ORIENTED_EDGE('',*,*,#26165,.F.);
#32520=ORIENTED_EDGE('',*,*,#26164,.F.);
#32521=ORIENTED_EDGE('',*,*,#26166,.T.);
#32522=ORIENTED_EDGE('',*,*,#26167,.T.);
#32523=ORIENTED_EDGE('',*,*,#26168,.F.);
#32524=ORIENTED_EDGE('',*,*,#26167,.F.);
#32525=ORIENTED_EDGE('',*,*,#26169,.T.);
#32526=ORIENTED_EDGE('',*,*,#26170,.T.);
#32527=ORIENTED_EDGE('',*,*,#26171,.F.);
#32528=ORIENTED_EDGE('',*,*,#26170,.F.);
#32529=ORIENTED_EDGE('',*,*,#26172,.T.);
#32530=ORIENTED_EDGE('',*,*,#26173,.T.);
#32531=ORIENTED_EDGE('',*,*,#26174,.F.);
#32532=ORIENTED_EDGE('',*,*,#26173,.F.);
#32533=ORIENTED_EDGE('',*,*,#26175,.T.);
#32534=ORIENTED_EDGE('',*,*,#26176,.T.);
#32535=ORIENTED_EDGE('',*,*,#26177,.F.);
#32536=ORIENTED_EDGE('',*,*,#26176,.F.);
#32537=ORIENTED_EDGE('',*,*,#26178,.T.);
#32538=ORIENTED_EDGE('',*,*,#26179,.T.);
#32539=ORIENTED_EDGE('',*,*,#26180,.F.);
#32540=ORIENTED_EDGE('',*,*,#26179,.F.);
#32541=ORIENTED_EDGE('',*,*,#26181,.T.);
#32542=ORIENTED_EDGE('',*,*,#26182,.T.);
#32543=ORIENTED_EDGE('',*,*,#26183,.F.);
#32544=ORIENTED_EDGE('',*,*,#26182,.F.);
#32545=ORIENTED_EDGE('',*,*,#26184,.T.);
#32546=ORIENTED_EDGE('',*,*,#26185,.T.);
#32547=ORIENTED_EDGE('',*,*,#26186,.F.);
#32548=ORIENTED_EDGE('',*,*,#26185,.F.);
#32549=ORIENTED_EDGE('',*,*,#26187,.T.);
#32550=ORIENTED_EDGE('',*,*,#26188,.T.);
#32551=ORIENTED_EDGE('',*,*,#26189,.F.);
#32552=ORIENTED_EDGE('',*,*,#26188,.F.);
#32553=ORIENTED_EDGE('',*,*,#26190,.T.);
#32554=ORIENTED_EDGE('',*,*,#26191,.T.);
#32555=ORIENTED_EDGE('',*,*,#26192,.F.);
#32556=ORIENTED_EDGE('',*,*,#26191,.F.);
#32557=ORIENTED_EDGE('',*,*,#26193,.T.);
#32558=ORIENTED_EDGE('',*,*,#26194,.T.);
#32559=ORIENTED_EDGE('',*,*,#26195,.F.);
#32560=ORIENTED_EDGE('',*,*,#26194,.F.);
#32561=ORIENTED_EDGE('',*,*,#26196,.T.);
#32562=ORIENTED_EDGE('',*,*,#26197,.T.);
#32563=ORIENTED_EDGE('',*,*,#26198,.F.);
#32564=ORIENTED_EDGE('',*,*,#26197,.F.);
#32565=ORIENTED_EDGE('',*,*,#26199,.T.);
#32566=ORIENTED_EDGE('',*,*,#26200,.T.);
#32567=ORIENTED_EDGE('',*,*,#26201,.F.);
#32568=ORIENTED_EDGE('',*,*,#26200,.F.);
#32569=ORIENTED_EDGE('',*,*,#26202,.T.);
#32570=ORIENTED_EDGE('',*,*,#26203,.T.);
#32571=ORIENTED_EDGE('',*,*,#26204,.F.);
#32572=ORIENTED_EDGE('',*,*,#26203,.F.);
#32573=ORIENTED_EDGE('',*,*,#26205,.T.);
#32574=ORIENTED_EDGE('',*,*,#26206,.T.);
#32575=ORIENTED_EDGE('',*,*,#26207,.F.);
#32576=ORIENTED_EDGE('',*,*,#26206,.F.);
#32577=ORIENTED_EDGE('',*,*,#26208,.T.);
#32578=ORIENTED_EDGE('',*,*,#26209,.T.);
#32579=ORIENTED_EDGE('',*,*,#26210,.F.);
#32580=ORIENTED_EDGE('',*,*,#26209,.F.);
#32581=ORIENTED_EDGE('',*,*,#26211,.T.);
#32582=ORIENTED_EDGE('',*,*,#26212,.T.);
#32583=ORIENTED_EDGE('',*,*,#26213,.F.);
#32584=ORIENTED_EDGE('',*,*,#26212,.F.);
#32585=ORIENTED_EDGE('',*,*,#26214,.T.);
#32586=ORIENTED_EDGE('',*,*,#26215,.T.);
#32587=ORIENTED_EDGE('',*,*,#26216,.F.);
#32588=ORIENTED_EDGE('',*,*,#26215,.F.);
#32589=ORIENTED_EDGE('',*,*,#26217,.T.);
#32590=ORIENTED_EDGE('',*,*,#26218,.T.);
#32591=ORIENTED_EDGE('',*,*,#26219,.F.);
#32592=ORIENTED_EDGE('',*,*,#26218,.F.);
#32593=ORIENTED_EDGE('',*,*,#26220,.T.);
#32594=ORIENTED_EDGE('',*,*,#26221,.T.);
#32595=ORIENTED_EDGE('',*,*,#26222,.F.);
#32596=ORIENTED_EDGE('',*,*,#26221,.F.);
#32597=ORIENTED_EDGE('',*,*,#26223,.T.);
#32598=ORIENTED_EDGE('',*,*,#26224,.T.);
#32599=ORIENTED_EDGE('',*,*,#26225,.F.);
#32600=ORIENTED_EDGE('',*,*,#26224,.F.);
#32601=ORIENTED_EDGE('',*,*,#26226,.T.);
#32602=ORIENTED_EDGE('',*,*,#26227,.T.);
#32603=ORIENTED_EDGE('',*,*,#26228,.F.);
#32604=ORIENTED_EDGE('',*,*,#26227,.F.);
#32605=ORIENTED_EDGE('',*,*,#26229,.T.);
#32606=ORIENTED_EDGE('',*,*,#26230,.T.);
#32607=ORIENTED_EDGE('',*,*,#26231,.F.);
#32608=ORIENTED_EDGE('',*,*,#26230,.F.);
#32609=ORIENTED_EDGE('',*,*,#26232,.T.);
#32610=ORIENTED_EDGE('',*,*,#26233,.T.);
#32611=ORIENTED_EDGE('',*,*,#26234,.F.);
#32612=ORIENTED_EDGE('',*,*,#26233,.F.);
#32613=ORIENTED_EDGE('',*,*,#26235,.T.);
#32614=ORIENTED_EDGE('',*,*,#26236,.T.);
#32615=ORIENTED_EDGE('',*,*,#26237,.F.);
#32616=ORIENTED_EDGE('',*,*,#26236,.F.);
#32617=ORIENTED_EDGE('',*,*,#26238,.T.);
#32618=ORIENTED_EDGE('',*,*,#26239,.T.);
#32619=ORIENTED_EDGE('',*,*,#26240,.T.);
#32620=ORIENTED_EDGE('',*,*,#26241,.F.);
#32621=ORIENTED_EDGE('',*,*,#26242,.T.);
#32622=ORIENTED_EDGE('',*,*,#26239,.F.);
#32623=ORIENTED_EDGE('',*,*,#26243,.T.);
#32624=ORIENTED_EDGE('',*,*,#26244,.T.);
#32625=ORIENTED_EDGE('',*,*,#26245,.F.);
#32626=ORIENTED_EDGE('',*,*,#26244,.F.);
#32627=ORIENTED_EDGE('',*,*,#26246,.T.);
#32628=ORIENTED_EDGE('',*,*,#26247,.T.);
#32629=ORIENTED_EDGE('',*,*,#26248,.F.);
#32630=ORIENTED_EDGE('',*,*,#26247,.F.);
#32631=ORIENTED_EDGE('',*,*,#26249,.T.);
#32632=ORIENTED_EDGE('',*,*,#26250,.T.);
#32633=ORIENTED_EDGE('',*,*,#26251,.F.);
#32634=ORIENTED_EDGE('',*,*,#26250,.F.);
#32635=ORIENTED_EDGE('',*,*,#26252,.T.);
#32636=ORIENTED_EDGE('',*,*,#26253,.T.);
#32637=ORIENTED_EDGE('',*,*,#26254,.F.);
#32638=ORIENTED_EDGE('',*,*,#26253,.F.);
#32639=ORIENTED_EDGE('',*,*,#26255,.T.);
#32640=ORIENTED_EDGE('',*,*,#26256,.T.);
#32641=ORIENTED_EDGE('',*,*,#26257,.F.);
#32642=ORIENTED_EDGE('',*,*,#26256,.F.);
#32643=ORIENTED_EDGE('',*,*,#26258,.T.);
#32644=ORIENTED_EDGE('',*,*,#26259,.T.);
#32645=ORIENTED_EDGE('',*,*,#26260,.F.);
#32646=ORIENTED_EDGE('',*,*,#26259,.F.);
#32647=ORIENTED_EDGE('',*,*,#26261,.T.);
#32648=ORIENTED_EDGE('',*,*,#26262,.T.);
#32649=ORIENTED_EDGE('',*,*,#26263,.F.);
#32650=ORIENTED_EDGE('',*,*,#26262,.F.);
#32651=ORIENTED_EDGE('',*,*,#26264,.T.);
#32652=ORIENTED_EDGE('',*,*,#26265,.T.);
#32653=ORIENTED_EDGE('',*,*,#26266,.F.);
#32654=ORIENTED_EDGE('',*,*,#26265,.F.);
#32655=ORIENTED_EDGE('',*,*,#26267,.T.);
#32656=ORIENTED_EDGE('',*,*,#26268,.T.);
#32657=ORIENTED_EDGE('',*,*,#26269,.F.);
#32658=ORIENTED_EDGE('',*,*,#26268,.F.);
#32659=ORIENTED_EDGE('',*,*,#26270,.T.);
#32660=ORIENTED_EDGE('',*,*,#26271,.T.);
#32661=ORIENTED_EDGE('',*,*,#26272,.F.);
#32662=ORIENTED_EDGE('',*,*,#26271,.F.);
#32663=ORIENTED_EDGE('',*,*,#26273,.T.);
#32664=ORIENTED_EDGE('',*,*,#26274,.T.);
#32665=ORIENTED_EDGE('',*,*,#26275,.F.);
#32666=ORIENTED_EDGE('',*,*,#26274,.F.);
#32667=ORIENTED_EDGE('',*,*,#26276,.T.);
#32668=ORIENTED_EDGE('',*,*,#26277,.T.);
#32669=ORIENTED_EDGE('',*,*,#26278,.F.);
#32670=ORIENTED_EDGE('',*,*,#26277,.F.);
#32671=ORIENTED_EDGE('',*,*,#26279,.T.);
#32672=ORIENTED_EDGE('',*,*,#26280,.T.);
#32673=ORIENTED_EDGE('',*,*,#26281,.F.);
#32674=ORIENTED_EDGE('',*,*,#26280,.F.);
#32675=ORIENTED_EDGE('',*,*,#26282,.T.);
#32676=ORIENTED_EDGE('',*,*,#26283,.T.);
#32677=ORIENTED_EDGE('',*,*,#26284,.F.);
#32678=ORIENTED_EDGE('',*,*,#26283,.F.);
#32679=ORIENTED_EDGE('',*,*,#26285,.T.);
#32680=ORIENTED_EDGE('',*,*,#26286,.T.);
#32681=ORIENTED_EDGE('',*,*,#26287,.F.);
#32682=ORIENTED_EDGE('',*,*,#26286,.F.);
#32683=ORIENTED_EDGE('',*,*,#26288,.T.);
#32684=ORIENTED_EDGE('',*,*,#26289,.T.);
#32685=ORIENTED_EDGE('',*,*,#26290,.F.);
#32686=ORIENTED_EDGE('',*,*,#26289,.F.);
#32687=ORIENTED_EDGE('',*,*,#26291,.T.);
#32688=ORIENTED_EDGE('',*,*,#26292,.T.);
#32689=ORIENTED_EDGE('',*,*,#26293,.F.);
#32690=ORIENTED_EDGE('',*,*,#26292,.F.);
#32691=ORIENTED_EDGE('',*,*,#26294,.T.);
#32692=ORIENTED_EDGE('',*,*,#26295,.T.);
#32693=ORIENTED_EDGE('',*,*,#26296,.F.);
#32694=ORIENTED_EDGE('',*,*,#26295,.F.);
#32695=ORIENTED_EDGE('',*,*,#26297,.T.);
#32696=ORIENTED_EDGE('',*,*,#26298,.T.);
#32697=ORIENTED_EDGE('',*,*,#26299,.F.);
#32698=ORIENTED_EDGE('',*,*,#26298,.F.);
#32699=ORIENTED_EDGE('',*,*,#26300,.T.);
#32700=ORIENTED_EDGE('',*,*,#26301,.T.);
#32701=ORIENTED_EDGE('',*,*,#26302,.F.);
#32702=ORIENTED_EDGE('',*,*,#26301,.F.);
#32703=ORIENTED_EDGE('',*,*,#26303,.T.);
#32704=ORIENTED_EDGE('',*,*,#26304,.T.);
#32705=ORIENTED_EDGE('',*,*,#26305,.F.);
#32706=ORIENTED_EDGE('',*,*,#26304,.F.);
#32707=ORIENTED_EDGE('',*,*,#26306,.T.);
#32708=ORIENTED_EDGE('',*,*,#26307,.T.);
#32709=ORIENTED_EDGE('',*,*,#26308,.F.);
#32710=ORIENTED_EDGE('',*,*,#26307,.F.);
#32711=ORIENTED_EDGE('',*,*,#26309,.T.);
#32712=ORIENTED_EDGE('',*,*,#26310,.T.);
#32713=ORIENTED_EDGE('',*,*,#26311,.F.);
#32714=ORIENTED_EDGE('',*,*,#26310,.F.);
#32715=ORIENTED_EDGE('',*,*,#26312,.T.);
#32716=ORIENTED_EDGE('',*,*,#26313,.T.);
#32717=ORIENTED_EDGE('',*,*,#26314,.F.);
#32718=ORIENTED_EDGE('',*,*,#26313,.F.);
#32719=ORIENTED_EDGE('',*,*,#26315,.T.);
#32720=ORIENTED_EDGE('',*,*,#26316,.T.);
#32721=ORIENTED_EDGE('',*,*,#26317,.F.);
#32722=ORIENTED_EDGE('',*,*,#26316,.F.);
#32723=ORIENTED_EDGE('',*,*,#26318,.T.);
#32724=ORIENTED_EDGE('',*,*,#26319,.T.);
#32725=ORIENTED_EDGE('',*,*,#26320,.F.);
#32726=ORIENTED_EDGE('',*,*,#26319,.F.);
#32727=ORIENTED_EDGE('',*,*,#26321,.T.);
#32728=ORIENTED_EDGE('',*,*,#26322,.T.);
#32729=ORIENTED_EDGE('',*,*,#26323,.F.);
#32730=ORIENTED_EDGE('',*,*,#26322,.F.);
#32731=ORIENTED_EDGE('',*,*,#26324,.T.);
#32732=ORIENTED_EDGE('',*,*,#26325,.T.);
#32733=ORIENTED_EDGE('',*,*,#26326,.F.);
#32734=ORIENTED_EDGE('',*,*,#26325,.F.);
#32735=ORIENTED_EDGE('',*,*,#26327,.T.);
#32736=ORIENTED_EDGE('',*,*,#26328,.T.);
#32737=ORIENTED_EDGE('',*,*,#26329,.F.);
#32738=ORIENTED_EDGE('',*,*,#26328,.F.);
#32739=ORIENTED_EDGE('',*,*,#26330,.T.);
#32740=ORIENTED_EDGE('',*,*,#26331,.T.);
#32741=ORIENTED_EDGE('',*,*,#26332,.F.);
#32742=ORIENTED_EDGE('',*,*,#26331,.F.);
#32743=ORIENTED_EDGE('',*,*,#26333,.T.);
#32744=ORIENTED_EDGE('',*,*,#26334,.T.);
#32745=ORIENTED_EDGE('',*,*,#26335,.F.);
#32746=ORIENTED_EDGE('',*,*,#26334,.F.);
#32747=ORIENTED_EDGE('',*,*,#26336,.T.);
#32748=ORIENTED_EDGE('',*,*,#26337,.T.);
#32749=ORIENTED_EDGE('',*,*,#26338,.F.);
#32750=ORIENTED_EDGE('',*,*,#26337,.F.);
#32751=ORIENTED_EDGE('',*,*,#26339,.T.);
#32752=ORIENTED_EDGE('',*,*,#26340,.T.);
#32753=ORIENTED_EDGE('',*,*,#26341,.F.);
#32754=ORIENTED_EDGE('',*,*,#26340,.F.);
#32755=ORIENTED_EDGE('',*,*,#26342,.T.);
#32756=ORIENTED_EDGE('',*,*,#26343,.T.);
#32757=ORIENTED_EDGE('',*,*,#26344,.T.);
#32758=ORIENTED_EDGE('',*,*,#26345,.F.);
#32759=ORIENTED_EDGE('',*,*,#26346,.F.);
#32760=ORIENTED_EDGE('',*,*,#26347,.T.);
#32761=ORIENTED_EDGE('',*,*,#26343,.F.);
#32762=ORIENTED_EDGE('',*,*,#26348,.T.);
#32763=ORIENTED_EDGE('',*,*,#26349,.T.);
#32764=ORIENTED_EDGE('',*,*,#26350,.F.);
#32765=ORIENTED_EDGE('',*,*,#26349,.F.);
#32766=ORIENTED_EDGE('',*,*,#26351,.T.);
#32767=ORIENTED_EDGE('',*,*,#26352,.T.);
#32768=ORIENTED_EDGE('',*,*,#26353,.F.);
#32769=ORIENTED_EDGE('',*,*,#26352,.F.);
#32770=ORIENTED_EDGE('',*,*,#26354,.T.);
#32771=ORIENTED_EDGE('',*,*,#26355,.T.);
#32772=ORIENTED_EDGE('',*,*,#26356,.F.);
#32773=ORIENTED_EDGE('',*,*,#26355,.F.);
#32774=ORIENTED_EDGE('',*,*,#26357,.T.);
#32775=ORIENTED_EDGE('',*,*,#26358,.T.);
#32776=ORIENTED_EDGE('',*,*,#26359,.F.);
#32777=ORIENTED_EDGE('',*,*,#26358,.F.);
#32778=ORIENTED_EDGE('',*,*,#26360,.T.);
#32779=ORIENTED_EDGE('',*,*,#26361,.T.);
#32780=ORIENTED_EDGE('',*,*,#26362,.F.);
#32781=ORIENTED_EDGE('',*,*,#26361,.F.);
#32782=ORIENTED_EDGE('',*,*,#26363,.T.);
#32783=ORIENTED_EDGE('',*,*,#26364,.T.);
#32784=ORIENTED_EDGE('',*,*,#26365,.F.);
#32785=ORIENTED_EDGE('',*,*,#26364,.F.);
#32786=ORIENTED_EDGE('',*,*,#26366,.T.);
#32787=ORIENTED_EDGE('',*,*,#26367,.T.);
#32788=ORIENTED_EDGE('',*,*,#26368,.F.);
#32789=ORIENTED_EDGE('',*,*,#26367,.F.);
#32790=ORIENTED_EDGE('',*,*,#26369,.T.);
#32791=ORIENTED_EDGE('',*,*,#26370,.T.);
#32792=ORIENTED_EDGE('',*,*,#26371,.F.);
#32793=ORIENTED_EDGE('',*,*,#26370,.F.);
#32794=ORIENTED_EDGE('',*,*,#26372,.T.);
#32795=ORIENTED_EDGE('',*,*,#26373,.T.);
#32796=ORIENTED_EDGE('',*,*,#26374,.F.);
#32797=ORIENTED_EDGE('',*,*,#26373,.F.);
#32798=ORIENTED_EDGE('',*,*,#26375,.T.);
#32799=ORIENTED_EDGE('',*,*,#26376,.T.);
#32800=ORIENTED_EDGE('',*,*,#26377,.F.);
#32801=ORIENTED_EDGE('',*,*,#26376,.F.);
#32802=ORIENTED_EDGE('',*,*,#26378,.T.);
#32803=ORIENTED_EDGE('',*,*,#26379,.T.);
#32804=ORIENTED_EDGE('',*,*,#26380,.F.);
#32805=ORIENTED_EDGE('',*,*,#26379,.F.);
#32806=ORIENTED_EDGE('',*,*,#26381,.T.);
#32807=ORIENTED_EDGE('',*,*,#26382,.T.);
#32808=ORIENTED_EDGE('',*,*,#26383,.F.);
#32809=ORIENTED_EDGE('',*,*,#26382,.F.);
#32810=ORIENTED_EDGE('',*,*,#26384,.T.);
#32811=ORIENTED_EDGE('',*,*,#26385,.T.);
#32812=ORIENTED_EDGE('',*,*,#26386,.F.);
#32813=ORIENTED_EDGE('',*,*,#26385,.F.);
#32814=ORIENTED_EDGE('',*,*,#26387,.T.);
#32815=ORIENTED_EDGE('',*,*,#26388,.T.);
#32816=ORIENTED_EDGE('',*,*,#26389,.F.);
#32817=ORIENTED_EDGE('',*,*,#26388,.F.);
#32818=ORIENTED_EDGE('',*,*,#26390,.T.);
#32819=ORIENTED_EDGE('',*,*,#26391,.T.);
#32820=ORIENTED_EDGE('',*,*,#26392,.F.);
#32821=ORIENTED_EDGE('',*,*,#26391,.F.);
#32822=ORIENTED_EDGE('',*,*,#26393,.T.);
#32823=ORIENTED_EDGE('',*,*,#26394,.T.);
#32824=ORIENTED_EDGE('',*,*,#26395,.F.);
#32825=ORIENTED_EDGE('',*,*,#26394,.F.);
#32826=ORIENTED_EDGE('',*,*,#26396,.T.);
#32827=ORIENTED_EDGE('',*,*,#26397,.T.);
#32828=ORIENTED_EDGE('',*,*,#26398,.F.);
#32829=ORIENTED_EDGE('',*,*,#26397,.F.);
#32830=ORIENTED_EDGE('',*,*,#26399,.T.);
#32831=ORIENTED_EDGE('',*,*,#26400,.T.);
#32832=ORIENTED_EDGE('',*,*,#26401,.T.);
#32833=ORIENTED_EDGE('',*,*,#26402,.F.);
#32834=ORIENTED_EDGE('',*,*,#26403,.T.);
#32835=ORIENTED_EDGE('',*,*,#26400,.F.);
#32836=ORIENTED_EDGE('',*,*,#26404,.T.);
#32837=ORIENTED_EDGE('',*,*,#26405,.T.);
#32838=ORIENTED_EDGE('',*,*,#26406,.F.);
#32839=ORIENTED_EDGE('',*,*,#26405,.F.);
#32840=ORIENTED_EDGE('',*,*,#26407,.T.);
#32841=ORIENTED_EDGE('',*,*,#26408,.T.);
#32842=ORIENTED_EDGE('',*,*,#26409,.F.);
#32843=ORIENTED_EDGE('',*,*,#26408,.F.);
#32844=ORIENTED_EDGE('',*,*,#26410,.T.);
#32845=ORIENTED_EDGE('',*,*,#26411,.T.);
#32846=ORIENTED_EDGE('',*,*,#26412,.F.);
#32847=ORIENTED_EDGE('',*,*,#26411,.F.);
#32848=ORIENTED_EDGE('',*,*,#26413,.T.);
#32849=ORIENTED_EDGE('',*,*,#26414,.T.);
#32850=ORIENTED_EDGE('',*,*,#26415,.F.);
#32851=ORIENTED_EDGE('',*,*,#26414,.F.);
#32852=ORIENTED_EDGE('',*,*,#26416,.T.);
#32853=ORIENTED_EDGE('',*,*,#26417,.T.);
#32854=ORIENTED_EDGE('',*,*,#26418,.F.);
#32855=ORIENTED_EDGE('',*,*,#26417,.F.);
#32856=ORIENTED_EDGE('',*,*,#26419,.T.);
#32857=ORIENTED_EDGE('',*,*,#26420,.T.);
#32858=ORIENTED_EDGE('',*,*,#26421,.F.);
#32859=ORIENTED_EDGE('',*,*,#26420,.F.);
#32860=ORIENTED_EDGE('',*,*,#26422,.T.);
#32861=ORIENTED_EDGE('',*,*,#26423,.T.);
#32862=ORIENTED_EDGE('',*,*,#26424,.F.);
#32863=ORIENTED_EDGE('',*,*,#26423,.F.);
#32864=ORIENTED_EDGE('',*,*,#26425,.T.);
#32865=ORIENTED_EDGE('',*,*,#26426,.T.);
#32866=ORIENTED_EDGE('',*,*,#26427,.F.);
#32867=ORIENTED_EDGE('',*,*,#26426,.F.);
#32868=ORIENTED_EDGE('',*,*,#26428,.T.);
#32869=ORIENTED_EDGE('',*,*,#26429,.T.);
#32870=ORIENTED_EDGE('',*,*,#26430,.F.);
#32871=ORIENTED_EDGE('',*,*,#26429,.F.);
#32872=ORIENTED_EDGE('',*,*,#26431,.T.);
#32873=ORIENTED_EDGE('',*,*,#26432,.T.);
#32874=ORIENTED_EDGE('',*,*,#26433,.F.);
#32875=ORIENTED_EDGE('',*,*,#26432,.F.);
#32876=ORIENTED_EDGE('',*,*,#26434,.T.);
#32877=ORIENTED_EDGE('',*,*,#26435,.T.);
#32878=ORIENTED_EDGE('',*,*,#26436,.F.);
#32879=ORIENTED_EDGE('',*,*,#26435,.F.);
#32880=ORIENTED_EDGE('',*,*,#26437,.T.);
#32881=ORIENTED_EDGE('',*,*,#26438,.T.);
#32882=ORIENTED_EDGE('',*,*,#26439,.F.);
#32883=ORIENTED_EDGE('',*,*,#26438,.F.);
#32884=ORIENTED_EDGE('',*,*,#26440,.T.);
#32885=ORIENTED_EDGE('',*,*,#26441,.T.);
#32886=ORIENTED_EDGE('',*,*,#26442,.F.);
#32887=ORIENTED_EDGE('',*,*,#26441,.F.);
#32888=ORIENTED_EDGE('',*,*,#26443,.T.);
#32889=ORIENTED_EDGE('',*,*,#26444,.T.);
#32890=ORIENTED_EDGE('',*,*,#26445,.F.);
#32891=ORIENTED_EDGE('',*,*,#26444,.F.);
#32892=ORIENTED_EDGE('',*,*,#26446,.T.);
#32893=ORIENTED_EDGE('',*,*,#26447,.T.);
#32894=ORIENTED_EDGE('',*,*,#26448,.F.);
#32895=ORIENTED_EDGE('',*,*,#26447,.F.);
#32896=ORIENTED_EDGE('',*,*,#26449,.T.);
#32897=ORIENTED_EDGE('',*,*,#26450,.T.);
#32898=ORIENTED_EDGE('',*,*,#26451,.F.);
#32899=ORIENTED_EDGE('',*,*,#26450,.F.);
#32900=ORIENTED_EDGE('',*,*,#26452,.T.);
#32901=ORIENTED_EDGE('',*,*,#26453,.T.);
#32902=ORIENTED_EDGE('',*,*,#26454,.F.);
#32903=ORIENTED_EDGE('',*,*,#26453,.F.);
#32904=ORIENTED_EDGE('',*,*,#26455,.T.);
#32905=ORIENTED_EDGE('',*,*,#26456,.T.);
#32906=ORIENTED_EDGE('',*,*,#26457,.F.);
#32907=ORIENTED_EDGE('',*,*,#26458,.T.);
#32908=ORIENTED_EDGE('',*,*,#26459,.F.);
#32909=ORIENTED_EDGE('',*,*,#26456,.F.);
#32910=ORIENTED_EDGE('',*,*,#26460,.T.);
#32911=ORIENTED_EDGE('',*,*,#26461,.T.);
#32912=ORIENTED_EDGE('',*,*,#26462,.F.);
#32913=ORIENTED_EDGE('',*,*,#26461,.F.);
#32914=ORIENTED_EDGE('',*,*,#26463,.T.);
#32915=ORIENTED_EDGE('',*,*,#26464,.T.);
#32916=ORIENTED_EDGE('',*,*,#26465,.F.);
#32917=ORIENTED_EDGE('',*,*,#26464,.F.);
#32918=ORIENTED_EDGE('',*,*,#26466,.T.);
#32919=ORIENTED_EDGE('',*,*,#26467,.T.);
#32920=ORIENTED_EDGE('',*,*,#26468,.F.);
#32921=ORIENTED_EDGE('',*,*,#26467,.F.);
#32922=ORIENTED_EDGE('',*,*,#26469,.T.);
#32923=ORIENTED_EDGE('',*,*,#26470,.T.);
#32924=ORIENTED_EDGE('',*,*,#26471,.F.);
#32925=ORIENTED_EDGE('',*,*,#26470,.F.);
#32926=ORIENTED_EDGE('',*,*,#26472,.T.);
#32927=ORIENTED_EDGE('',*,*,#26473,.T.);
#32928=ORIENTED_EDGE('',*,*,#26474,.F.);
#32929=ORIENTED_EDGE('',*,*,#26473,.F.);
#32930=ORIENTED_EDGE('',*,*,#26475,.T.);
#32931=ORIENTED_EDGE('',*,*,#26476,.T.);
#32932=ORIENTED_EDGE('',*,*,#26477,.F.);
#32933=ORIENTED_EDGE('',*,*,#26476,.F.);
#32934=ORIENTED_EDGE('',*,*,#26478,.T.);
#32935=ORIENTED_EDGE('',*,*,#26479,.T.);
#32936=ORIENTED_EDGE('',*,*,#26480,.F.);
#32937=ORIENTED_EDGE('',*,*,#26479,.F.);
#32938=ORIENTED_EDGE('',*,*,#26481,.T.);
#32939=ORIENTED_EDGE('',*,*,#26482,.T.);
#32940=ORIENTED_EDGE('',*,*,#26483,.F.);
#32941=ORIENTED_EDGE('',*,*,#26482,.F.);
#32942=ORIENTED_EDGE('',*,*,#26484,.T.);
#32943=ORIENTED_EDGE('',*,*,#26485,.T.);
#32944=ORIENTED_EDGE('',*,*,#26486,.F.);
#32945=ORIENTED_EDGE('',*,*,#26485,.F.);
#32946=ORIENTED_EDGE('',*,*,#26487,.T.);
#32947=ORIENTED_EDGE('',*,*,#26488,.T.);
#32948=ORIENTED_EDGE('',*,*,#26489,.F.);
#32949=ORIENTED_EDGE('',*,*,#26488,.F.);
#32950=ORIENTED_EDGE('',*,*,#26490,.T.);
#32951=ORIENTED_EDGE('',*,*,#26491,.T.);
#32952=ORIENTED_EDGE('',*,*,#26492,.F.);
#32953=ORIENTED_EDGE('',*,*,#26491,.F.);
#32954=ORIENTED_EDGE('',*,*,#26493,.T.);
#32955=ORIENTED_EDGE('',*,*,#26494,.T.);
#32956=ORIENTED_EDGE('',*,*,#26495,.F.);
#32957=ORIENTED_EDGE('',*,*,#26494,.F.);
#32958=ORIENTED_EDGE('',*,*,#26496,.T.);
#32959=ORIENTED_EDGE('',*,*,#26497,.T.);
#32960=ORIENTED_EDGE('',*,*,#26498,.F.);
#32961=ORIENTED_EDGE('',*,*,#26497,.F.);
#32962=ORIENTED_EDGE('',*,*,#26499,.T.);
#32963=ORIENTED_EDGE('',*,*,#26500,.T.);
#32964=ORIENTED_EDGE('',*,*,#26501,.F.);
#32965=ORIENTED_EDGE('',*,*,#26500,.F.);
#32966=ORIENTED_EDGE('',*,*,#26502,.T.);
#32967=ORIENTED_EDGE('',*,*,#26503,.T.);
#32968=ORIENTED_EDGE('',*,*,#26504,.F.);
#32969=ORIENTED_EDGE('',*,*,#26503,.F.);
#32970=ORIENTED_EDGE('',*,*,#26505,.T.);
#32971=ORIENTED_EDGE('',*,*,#26506,.T.);
#32972=ORIENTED_EDGE('',*,*,#26507,.F.);
#32973=ORIENTED_EDGE('',*,*,#26508,.T.);
#32974=ORIENTED_EDGE('',*,*,#26509,.F.);
#32975=ORIENTED_EDGE('',*,*,#26506,.F.);
#32976=ORIENTED_EDGE('',*,*,#26510,.T.);
#32977=ORIENTED_EDGE('',*,*,#26511,.T.);
#32978=ORIENTED_EDGE('',*,*,#26512,.F.);
#32979=ORIENTED_EDGE('',*,*,#26511,.F.);
#32980=ORIENTED_EDGE('',*,*,#26513,.T.);
#32981=ORIENTED_EDGE('',*,*,#26514,.T.);
#32982=ORIENTED_EDGE('',*,*,#26515,.F.);
#32983=ORIENTED_EDGE('',*,*,#26514,.F.);
#32984=ORIENTED_EDGE('',*,*,#26516,.T.);
#32985=ORIENTED_EDGE('',*,*,#26517,.T.);
#32986=ORIENTED_EDGE('',*,*,#26518,.F.);
#32987=ORIENTED_EDGE('',*,*,#26517,.F.);
#32988=ORIENTED_EDGE('',*,*,#26519,.T.);
#32989=ORIENTED_EDGE('',*,*,#26520,.T.);
#32990=ORIENTED_EDGE('',*,*,#26521,.F.);
#32991=ORIENTED_EDGE('',*,*,#26520,.F.);
#32992=ORIENTED_EDGE('',*,*,#26522,.T.);
#32993=ORIENTED_EDGE('',*,*,#26523,.T.);
#32994=ORIENTED_EDGE('',*,*,#26524,.F.);
#32995=ORIENTED_EDGE('',*,*,#26523,.F.);
#32996=ORIENTED_EDGE('',*,*,#26525,.T.);
#32997=ORIENTED_EDGE('',*,*,#26526,.T.);
#32998=ORIENTED_EDGE('',*,*,#26527,.F.);
#32999=ORIENTED_EDGE('',*,*,#26526,.F.);
#33000=ORIENTED_EDGE('',*,*,#26528,.T.);
#33001=ORIENTED_EDGE('',*,*,#26529,.T.);
#33002=ORIENTED_EDGE('',*,*,#26530,.F.);
#33003=ORIENTED_EDGE('',*,*,#26529,.F.);
#33004=ORIENTED_EDGE('',*,*,#26531,.T.);
#33005=ORIENTED_EDGE('',*,*,#26532,.T.);
#33006=ORIENTED_EDGE('',*,*,#26533,.F.);
#33007=ORIENTED_EDGE('',*,*,#26532,.F.);
#33008=ORIENTED_EDGE('',*,*,#26534,.T.);
#33009=ORIENTED_EDGE('',*,*,#26535,.T.);
#33010=ORIENTED_EDGE('',*,*,#26536,.F.);
#33011=ORIENTED_EDGE('',*,*,#26535,.F.);
#33012=ORIENTED_EDGE('',*,*,#26537,.T.);
#33013=ORIENTED_EDGE('',*,*,#26538,.T.);
#33014=ORIENTED_EDGE('',*,*,#26539,.F.);
#33015=ORIENTED_EDGE('',*,*,#26538,.F.);
#33016=ORIENTED_EDGE('',*,*,#26540,.T.);
#33017=ORIENTED_EDGE('',*,*,#26541,.T.);
#33018=ORIENTED_EDGE('',*,*,#26542,.F.);
#33019=ORIENTED_EDGE('',*,*,#26541,.F.);
#33020=ORIENTED_EDGE('',*,*,#26543,.T.);
#33021=ORIENTED_EDGE('',*,*,#26544,.T.);
#33022=ORIENTED_EDGE('',*,*,#26545,.F.);
#33023=ORIENTED_EDGE('',*,*,#26544,.F.);
#33024=ORIENTED_EDGE('',*,*,#26546,.T.);
#33025=ORIENTED_EDGE('',*,*,#26547,.T.);
#33026=ORIENTED_EDGE('',*,*,#26548,.F.);
#33027=ORIENTED_EDGE('',*,*,#26547,.F.);
#33028=ORIENTED_EDGE('',*,*,#26549,.T.);
#33029=ORIENTED_EDGE('',*,*,#26550,.T.);
#33030=ORIENTED_EDGE('',*,*,#26551,.F.);
#33031=ORIENTED_EDGE('',*,*,#26550,.F.);
#33032=ORIENTED_EDGE('',*,*,#26552,.T.);
#33033=ORIENTED_EDGE('',*,*,#26553,.T.);
#33034=ORIENTED_EDGE('',*,*,#26554,.F.);
#33035=ORIENTED_EDGE('',*,*,#26553,.F.);
#33036=ORIENTED_EDGE('',*,*,#26555,.T.);
#33037=ORIENTED_EDGE('',*,*,#26556,.T.);
#33038=ORIENTED_EDGE('',*,*,#26557,.F.);
#33039=ORIENTED_EDGE('',*,*,#26556,.F.);
#33040=ORIENTED_EDGE('',*,*,#26558,.T.);
#33041=ORIENTED_EDGE('',*,*,#26559,.T.);
#33042=ORIENTED_EDGE('',*,*,#26560,.F.);
#33043=ORIENTED_EDGE('',*,*,#26559,.F.);
#33044=ORIENTED_EDGE('',*,*,#26561,.T.);
#33045=ORIENTED_EDGE('',*,*,#26562,.T.);
#33046=ORIENTED_EDGE('',*,*,#26563,.F.);
#33047=ORIENTED_EDGE('',*,*,#26564,.T.);
#33048=ORIENTED_EDGE('',*,*,#26565,.F.);
#33049=ORIENTED_EDGE('',*,*,#26562,.F.);
#33050=ORIENTED_EDGE('',*,*,#26566,.T.);
#33051=ORIENTED_EDGE('',*,*,#26567,.T.);
#33052=ORIENTED_EDGE('',*,*,#26568,.F.);
#33053=ORIENTED_EDGE('',*,*,#26567,.F.);
#33054=ORIENTED_EDGE('',*,*,#26569,.T.);
#33055=ORIENTED_EDGE('',*,*,#26570,.T.);
#33056=ORIENTED_EDGE('',*,*,#26571,.F.);
#33057=ORIENTED_EDGE('',*,*,#26570,.F.);
#33058=ORIENTED_EDGE('',*,*,#26572,.T.);
#33059=ORIENTED_EDGE('',*,*,#26573,.T.);
#33060=ORIENTED_EDGE('',*,*,#26574,.F.);
#33061=ORIENTED_EDGE('',*,*,#26573,.F.);
#33062=ORIENTED_EDGE('',*,*,#26575,.T.);
#33063=ORIENTED_EDGE('',*,*,#26576,.T.);
#33064=ORIENTED_EDGE('',*,*,#26577,.F.);
#33065=ORIENTED_EDGE('',*,*,#26576,.F.);
#33066=ORIENTED_EDGE('',*,*,#26578,.T.);
#33067=ORIENTED_EDGE('',*,*,#26579,.T.);
#33068=ORIENTED_EDGE('',*,*,#26580,.F.);
#33069=ORIENTED_EDGE('',*,*,#26579,.F.);
#33070=ORIENTED_EDGE('',*,*,#26581,.T.);
#33071=ORIENTED_EDGE('',*,*,#26582,.T.);
#33072=ORIENTED_EDGE('',*,*,#26583,.F.);
#33073=ORIENTED_EDGE('',*,*,#26582,.F.);
#33074=ORIENTED_EDGE('',*,*,#26584,.T.);
#33075=ORIENTED_EDGE('',*,*,#26585,.T.);
#33076=ORIENTED_EDGE('',*,*,#26586,.F.);
#33077=ORIENTED_EDGE('',*,*,#26585,.F.);
#33078=ORIENTED_EDGE('',*,*,#26587,.T.);
#33079=ORIENTED_EDGE('',*,*,#26588,.T.);
#33080=ORIENTED_EDGE('',*,*,#26589,.F.);
#33081=ORIENTED_EDGE('',*,*,#26588,.F.);
#33082=ORIENTED_EDGE('',*,*,#26590,.T.);
#33083=ORIENTED_EDGE('',*,*,#26591,.T.);
#33084=ORIENTED_EDGE('',*,*,#26592,.F.);
#33085=ORIENTED_EDGE('',*,*,#26591,.F.);
#33086=ORIENTED_EDGE('',*,*,#26593,.T.);
#33087=ORIENTED_EDGE('',*,*,#26594,.T.);
#33088=ORIENTED_EDGE('',*,*,#26595,.F.);
#33089=ORIENTED_EDGE('',*,*,#26594,.F.);
#33090=ORIENTED_EDGE('',*,*,#26596,.T.);
#33091=ORIENTED_EDGE('',*,*,#26597,.T.);
#33092=ORIENTED_EDGE('',*,*,#26598,.F.);
#33093=ORIENTED_EDGE('',*,*,#26597,.F.);
#33094=ORIENTED_EDGE('',*,*,#26599,.T.);
#33095=ORIENTED_EDGE('',*,*,#26600,.T.);
#33096=ORIENTED_EDGE('',*,*,#26601,.F.);
#33097=ORIENTED_EDGE('',*,*,#26600,.F.);
#33098=ORIENTED_EDGE('',*,*,#26602,.T.);
#33099=ORIENTED_EDGE('',*,*,#26603,.T.);
#33100=ORIENTED_EDGE('',*,*,#26604,.F.);
#33101=ORIENTED_EDGE('',*,*,#26603,.F.);
#33102=ORIENTED_EDGE('',*,*,#26605,.T.);
#33103=ORIENTED_EDGE('',*,*,#26606,.T.);
#33104=ORIENTED_EDGE('',*,*,#26607,.F.);
#33105=ORIENTED_EDGE('',*,*,#26606,.F.);
#33106=ORIENTED_EDGE('',*,*,#26608,.T.);
#33107=ORIENTED_EDGE('',*,*,#26609,.T.);
#33108=ORIENTED_EDGE('',*,*,#26610,.F.);
#33109=ORIENTED_EDGE('',*,*,#26609,.F.);
#33110=ORIENTED_EDGE('',*,*,#26611,.T.);
#33111=ORIENTED_EDGE('',*,*,#26612,.T.);
#33112=ORIENTED_EDGE('',*,*,#26613,.F.);
#33113=ORIENTED_EDGE('',*,*,#26612,.F.);
#33114=ORIENTED_EDGE('',*,*,#26614,.T.);
#33115=ORIENTED_EDGE('',*,*,#26615,.T.);
#33116=ORIENTED_EDGE('',*,*,#26616,.F.);
#33117=ORIENTED_EDGE('',*,*,#26615,.F.);
#33118=ORIENTED_EDGE('',*,*,#26617,.T.);
#33119=ORIENTED_EDGE('',*,*,#26618,.T.);
#33120=ORIENTED_EDGE('',*,*,#26619,.F.);
#33121=ORIENTED_EDGE('',*,*,#26620,.T.);
#33122=ORIENTED_EDGE('',*,*,#26621,.F.);
#33123=ORIENTED_EDGE('',*,*,#26618,.F.);
#33124=ORIENTED_EDGE('',*,*,#26622,.T.);
#33125=ORIENTED_EDGE('',*,*,#26623,.T.);
#33126=ORIENTED_EDGE('',*,*,#26624,.F.);
#33127=ORIENTED_EDGE('',*,*,#26623,.F.);
#33128=ORIENTED_EDGE('',*,*,#26625,.F.);
#33129=ORIENTED_EDGE('',*,*,#26626,.F.);
#33130=ORIENTED_EDGE('',*,*,#26345,.T.);
#33131=ORIENTED_EDGE('',*,*,#26627,.F.);
#33132=ORIENTED_EDGE('',*,*,#26402,.T.);
#33133=ORIENTED_EDGE('',*,*,#26628,.F.);
#33134=ORIENTED_EDGE('',*,*,#26457,.T.);
#33135=ORIENTED_EDGE('',*,*,#26459,.T.);
#33136=ORIENTED_EDGE('',*,*,#26629,.F.);
#33137=ORIENTED_EDGE('',*,*,#26507,.T.);
#33138=ORIENTED_EDGE('',*,*,#26509,.T.);
#33139=ORIENTED_EDGE('',*,*,#26630,.F.);
#33140=ORIENTED_EDGE('',*,*,#26563,.T.);
#33141=ORIENTED_EDGE('',*,*,#26565,.T.);
#33142=ORIENTED_EDGE('',*,*,#26631,.F.);
#33143=ORIENTED_EDGE('',*,*,#26619,.T.);
#33144=ORIENTED_EDGE('',*,*,#26621,.T.);
#33145=ORIENTED_EDGE('',*,*,#26632,.F.);
#33146=ORIENTED_EDGE('',*,*,#25068,.T.);
#33147=ORIENTED_EDGE('',*,*,#25070,.T.);
#33148=ORIENTED_EDGE('',*,*,#26633,.F.);
#33149=ORIENTED_EDGE('',*,*,#25124,.T.);
#33150=ORIENTED_EDGE('',*,*,#25126,.T.);
#33151=ORIENTED_EDGE('',*,*,#26634,.F.);
#33152=ORIENTED_EDGE('',*,*,#25174,.T.);
#33153=ORIENTED_EDGE('',*,*,#25176,.T.);
#33154=ORIENTED_EDGE('',*,*,#26635,.F.);
#33155=ORIENTED_EDGE('',*,*,#25230,.T.);
#33156=ORIENTED_EDGE('',*,*,#25232,.T.);
#33157=ORIENTED_EDGE('',*,*,#26636,.F.);
#33158=ORIENTED_EDGE('',*,*,#25286,.T.);
#33159=ORIENTED_EDGE('',*,*,#25288,.T.);
#33160=ORIENTED_EDGE('',*,*,#26637,.F.);
#33161=ORIENTED_EDGE('',*,*,#25342,.T.);
#33162=ORIENTED_EDGE('',*,*,#25344,.T.);
#33163=ORIENTED_EDGE('',*,*,#26638,.F.);
#33164=ORIENTED_EDGE('',*,*,#25398,.T.);
#33165=ORIENTED_EDGE('',*,*,#25400,.T.);
#33166=ORIENTED_EDGE('',*,*,#26639,.F.);
#33167=ORIENTED_EDGE('',*,*,#25448,.T.);
#33168=ORIENTED_EDGE('',*,*,#25450,.T.);
#33169=ORIENTED_EDGE('',*,*,#26640,.F.);
#33170=ORIENTED_EDGE('',*,*,#25504,.T.);
#33171=ORIENTED_EDGE('',*,*,#25506,.T.);
#33172=ORIENTED_EDGE('',*,*,#26641,.F.);
#33173=ORIENTED_EDGE('',*,*,#25560,.T.);
#33174=ORIENTED_EDGE('',*,*,#25562,.T.);
#33175=ORIENTED_EDGE('',*,*,#26642,.F.);
#33176=ORIENTED_EDGE('',*,*,#25616,.T.);
#33177=ORIENTED_EDGE('',*,*,#25618,.T.);
#33178=ORIENTED_EDGE('',*,*,#26643,.F.);
#33179=ORIENTED_EDGE('',*,*,#25672,.T.);
#33180=ORIENTED_EDGE('',*,*,#25674,.T.);
#33181=ORIENTED_EDGE('',*,*,#26644,.F.);
#33182=ORIENTED_EDGE('',*,*,#25722,.T.);
#33183=ORIENTED_EDGE('',*,*,#25724,.T.);
#33184=ORIENTED_EDGE('',*,*,#26645,.F.);
#33185=ORIENTED_EDGE('',*,*,#25778,.T.);
#33186=ORIENTED_EDGE('',*,*,#25780,.T.);
#33187=ORIENTED_EDGE('',*,*,#26646,.F.);
#33188=ORIENTED_EDGE('',*,*,#25834,.T.);
#33189=ORIENTED_EDGE('',*,*,#25836,.T.);
#33190=ORIENTED_EDGE('',*,*,#26647,.F.);
#33191=ORIENTED_EDGE('',*,*,#25890,.T.);
#33192=ORIENTED_EDGE('',*,*,#25892,.T.);
#33193=ORIENTED_EDGE('',*,*,#26648,.F.);
#33194=ORIENTED_EDGE('',*,*,#25946,.T.);
#33195=ORIENTED_EDGE('',*,*,#25948,.T.);
#33196=ORIENTED_EDGE('',*,*,#26649,.F.);
#33197=ORIENTED_EDGE('',*,*,#25996,.T.);
#33198=ORIENTED_EDGE('',*,*,#25998,.T.);
#33199=ORIENTED_EDGE('',*,*,#26650,.F.);
#33200=ORIENTED_EDGE('',*,*,#26053,.T.);
#33201=ORIENTED_EDGE('',*,*,#26651,.F.);
#33202=ORIENTED_EDGE('',*,*,#26652,.F.);
#33203=ORIENTED_EDGE('',*,*,#24992,.T.);
#33204=ORIENTED_EDGE('',*,*,#24999,.T.);
#33205=ORIENTED_EDGE('',*,*,#24971,.T.);
#33206=ORIENTED_EDGE('',*,*,#24985,.T.);
#33207=ORIENTED_EDGE('',*,*,#24978,.T.);
#33208=ORIENTED_EDGE('',*,*,#24578,.T.);
#33209=ORIENTED_EDGE('',*,*,#24585,.T.);
#33210=ORIENTED_EDGE('',*,*,#25013,.T.);
#33211=ORIENTED_EDGE('',*,*,#25006,.T.);
#33212=ORIENTED_EDGE('',*,*,#26653,.T.);
#33213=ORIENTED_EDGE('',*,*,#26654,.T.);
#33214=ORIENTED_EDGE('',*,*,#24571,.T.);
#33215=ORIENTED_EDGE('',*,*,#24950,.T.);
#33216=ORIENTED_EDGE('',*,*,#24964,.T.);
#33217=ORIENTED_EDGE('',*,*,#24592,.T.);
#33218=ORIENTED_EDGE('',*,*,#24599,.T.);
#33219=ORIENTED_EDGE('',*,*,#24606,.T.);
#33220=ORIENTED_EDGE('',*,*,#24613,.T.);
#33221=ORIENTED_EDGE('',*,*,#24620,.T.);
#33222=ORIENTED_EDGE('',*,*,#24669,.T.);
#33223=ORIENTED_EDGE('',*,*,#24634,.T.);
#33224=ORIENTED_EDGE('',*,*,#24641,.T.);
#33225=ORIENTED_EDGE('',*,*,#24627,.T.);
#33226=ORIENTED_EDGE('',*,*,#24655,.T.);
#33227=ORIENTED_EDGE('',*,*,#24648,.T.);
#33228=ORIENTED_EDGE('',*,*,#24753,.T.);
#33229=ORIENTED_EDGE('',*,*,#24746,.T.);
#33230=ORIENTED_EDGE('',*,*,#24774,.T.);
#33231=ORIENTED_EDGE('',*,*,#24760,.T.);
#33232=ORIENTED_EDGE('',*,*,#24767,.T.);
#33233=ORIENTED_EDGE('',*,*,#24704,.T.);
#33234=ORIENTED_EDGE('',*,*,#24711,.T.);
#33235=ORIENTED_EDGE('',*,*,#24732,.T.);
#33236=ORIENTED_EDGE('',*,*,#24739,.T.);
#33237=ORIENTED_EDGE('',*,*,#24718,.T.);
#33238=ORIENTED_EDGE('',*,*,#24725,.T.);
#33239=ORIENTED_EDGE('',*,*,#24837,.T.);
#33240=ORIENTED_EDGE('',*,*,#24823,.T.);
#33241=ORIENTED_EDGE('',*,*,#24816,.T.);
#33242=ORIENTED_EDGE('',*,*,#24788,.T.);
#33243=ORIENTED_EDGE('',*,*,#24795,.T.);
#33244=ORIENTED_EDGE('',*,*,#24781,.T.);
#33245=ORIENTED_EDGE('',*,*,#24809,.T.);
#33246=ORIENTED_EDGE('',*,*,#24802,.T.);
#33247=ORIENTED_EDGE('',*,*,#24683,.T.);
#33248=ORIENTED_EDGE('',*,*,#24676,.T.);
#33249=ORIENTED_EDGE('',*,*,#24662,.T.);
#33250=ORIENTED_EDGE('',*,*,#24697,.T.);
#33251=ORIENTED_EDGE('',*,*,#24690,.T.);
#33252=ORIENTED_EDGE('',*,*,#26655,.F.);
#33253=ORIENTED_EDGE('',*,*,#26656,.F.);
#33254=ORIENTED_EDGE('',*,*,#26657,.T.);
#33255=ORIENTED_EDGE('',*,*,#26658,.T.);
#33256=ORIENTED_EDGE('',*,*,#26659,.T.);
#33257=ORIENTED_EDGE('',*,*,#26660,.T.);
#33258=ORIENTED_EDGE('',*,*,#26661,.T.);
#33259=ORIENTED_EDGE('',*,*,#26662,.T.);
#33260=ORIENTED_EDGE('',*,*,#26663,.F.);
#33261=ORIENTED_EDGE('',*,*,#26664,.T.);
#33262=ORIENTED_EDGE('',*,*,#26665,.T.);
#33263=ORIENTED_EDGE('',*,*,#26666,.T.);
#33264=ORIENTED_EDGE('',*,*,#26665,.F.);
#33265=ORIENTED_EDGE('',*,*,#26667,.T.);
#33266=ORIENTED_EDGE('',*,*,#26666,.F.);
#33267=ORIENTED_EDGE('',*,*,#26668,.T.);
#33268=ORIENTED_EDGE('',*,*,#26669,.F.);
#33269=ORIENTED_EDGE('',*,*,#26668,.F.);
#33270=ORIENTED_EDGE('',*,*,#26664,.F.);
#33271=ORIENTED_EDGE('',*,*,#26670,.T.);
#33272=ORIENTED_EDGE('',*,*,#26671,.F.);
#33273=ORIENTED_EDGE('',*,*,#26672,.F.);
#33274=ORIENTED_EDGE('',*,*,#26670,.F.);
#33275=ORIENTED_EDGE('',*,*,#26667,.F.);
#33276=ORIENTED_EDGE('',*,*,#26673,.T.);
#33277=ORIENTED_EDGE('',*,*,#26674,.F.);
#33278=ORIENTED_EDGE('',*,*,#26675,.F.);
#33279=ORIENTED_EDGE('',*,*,#26676,.T.);
#33280=ORIENTED_EDGE('',*,*,#26677,.F.);
#33281=ORIENTED_EDGE('',*,*,#26678,.F.);
#33282=ORIENTED_EDGE('',*,*,#26679,.F.);
#33283=ORIENTED_EDGE('',*,*,#26680,.T.);
#33284=ORIENTED_EDGE('',*,*,#26681,.T.);
#33285=ORIENTED_EDGE('',*,*,#26682,.T.);
#33286=ORIENTED_EDGE('',*,*,#26683,.F.);
#33287=ORIENTED_EDGE('',*,*,#26684,.F.);
#33288=ORIENTED_EDGE('',*,*,#26685,.F.);
#33289=ORIENTED_EDGE('',*,*,#26660,.F.);
#33290=ORIENTED_EDGE('',*,*,#26659,.F.);
#33291=ORIENTED_EDGE('',*,*,#26686,.T.);
#33292=ORIENTED_EDGE('',*,*,#26673,.F.);
#33293=ORIENTED_EDGE('',*,*,#26687,.F.);
#33294=ORIENTED_EDGE('',*,*,#26688,.T.);
#33295=ORIENTED_EDGE('',*,*,#26689,.T.);
#33296=ORIENTED_EDGE('',*,*,#26671,.T.);
#33297=ORIENTED_EDGE('',*,*,#26672,.T.);
#33298=ORIENTED_EDGE('',*,*,#26689,.F.);
#33299=ORIENTED_EDGE('',*,*,#26690,.T.);
#33300=ORIENTED_EDGE('',*,*,#26688,.F.);
#33301=ORIENTED_EDGE('',*,*,#26691,.T.);
#33302=ORIENTED_EDGE('',*,*,#26692,.F.);
#33303=ORIENTED_EDGE('',*,*,#26691,.F.);
#33304=ORIENTED_EDGE('',*,*,#26690,.F.);
#33305=ORIENTED_EDGE('',*,*,#26693,.T.);
#33306=ORIENTED_EDGE('',*,*,#26694,.T.);
#33307=ORIENTED_EDGE('',*,*,#26695,.F.);
#33308=ORIENTED_EDGE('',*,*,#26694,.F.);
#33309=ORIENTED_EDGE('',*,*,#26696,.T.);
#33310=ORIENTED_EDGE('',*,*,#26697,.T.);
#33311=ORIENTED_EDGE('',*,*,#26653,.F.);
#33312=ORIENTED_EDGE('',*,*,#26654,.F.);
#33313=ORIENTED_EDGE('',*,*,#26697,.F.);
#33314=ORIENTED_EDGE('',*,*,#26698,.T.);
#33315=ORIENTED_EDGE('',*,*,#26696,.F.);
#33316=ORIENTED_EDGE('',*,*,#26698,.F.);
#33317=ORIENTED_EDGE('',*,*,#26695,.T.);
#33318=ORIENTED_EDGE('',*,*,#26693,.F.);
#33319=ORIENTED_EDGE('',*,*,#26692,.T.);
#33320=ORIENTED_EDGE('',*,*,#26699,.T.);
#33321=ORIENTED_EDGE('',*,*,#26700,.T.);
#33322=ORIENTED_EDGE('',*,*,#26701,.T.);
#33323=ORIENTED_EDGE('',*,*,#26702,.T.);
#33324=ORIENTED_EDGE('',*,*,#26703,.F.);
#33325=ORIENTED_EDGE('',*,*,#26704,.T.);
#33326=ORIENTED_EDGE('',*,*,#26705,.T.);
#33327=ORIENTED_EDGE('',*,*,#26706,.T.);
#33328=ORIENTED_EDGE('',*,*,#26707,.F.);
#33329=ORIENTED_EDGE('',*,*,#26708,.F.);
#33330=ORIENTED_EDGE('',*,*,#26705,.F.);
#33331=ORIENTED_EDGE('',*,*,#26709,.F.);
#33332=ORIENTED_EDGE('',*,*,#26710,.F.);
#33333=ORIENTED_EDGE('',*,*,#26711,.T.);
#33334=ORIENTED_EDGE('',*,*,#26712,.T.);
#33335=ORIENTED_EDGE('',*,*,#26713,.F.);
#33336=ORIENTED_EDGE('',*,*,#26699,.F.);
#33337=ORIENTED_EDGE('',*,*,#26714,.T.);
#33338=ORIENTED_EDGE('',*,*,#26715,.T.);
#33339=ORIENTED_EDGE('',*,*,#26703,.T.);
#33340=ORIENTED_EDGE('',*,*,#26716,.T.);
#33341=ORIENTED_EDGE('',*,*,#26717,.T.);
#33342=ORIENTED_EDGE('',*,*,#26718,.T.);
#33343=ORIENTED_EDGE('',*,*,#26719,.T.);
#33344=ORIENTED_EDGE('',*,*,#26715,.F.);
#33345=ORIENTED_EDGE('',*,*,#26720,.T.);
#33346=ORIENTED_EDGE('',*,*,#26707,.T.);
#33347=ORIENTED_EDGE('',*,*,#26721,.T.);
#33348=ORIENTED_EDGE('',*,*,#26722,.T.);
#33349=ORIENTED_EDGE('',*,*,#26723,.T.);
#33350=ORIENTED_EDGE('',*,*,#26724,.T.);
#33351=ORIENTED_EDGE('',*,*,#26725,.T.);
#33352=ORIENTED_EDGE('',*,*,#26726,.F.);
#33353=ORIENTED_EDGE('',*,*,#26727,.T.);
#33354=ORIENTED_EDGE('',*,*,#26728,.F.);
#33355=ORIENTED_EDGE('',*,*,#26729,.T.);
#33356=ORIENTED_EDGE('',*,*,#26730,.F.);
#33357=ORIENTED_EDGE('',*,*,#26731,.T.);
#33358=ORIENTED_EDGE('',*,*,#26726,.T.);
#33359=ORIENTED_EDGE('',*,*,#26732,.T.);
#33360=ORIENTED_EDGE('',*,*,#26733,.F.);
#33361=ORIENTED_EDGE('',*,*,#26710,.T.);
#33362=ORIENTED_EDGE('',*,*,#26728,.T.);
#33363=ORIENTED_EDGE('',*,*,#26734,.T.);
#33364=ORIENTED_EDGE('',*,*,#26735,.F.);
#33365=ORIENTED_EDGE('',*,*,#26736,.T.);
#33366=ORIENTED_EDGE('',*,*,#26737,.F.);
#33367=ORIENTED_EDGE('',*,*,#26738,.F.);
#33368=ORIENTED_EDGE('',*,*,#26735,.T.);
#33369=ORIENTED_EDGE('',*,*,#26739,.T.);
#33370=ORIENTED_EDGE('',*,*,#26730,.T.);
#33371=ORIENTED_EDGE('',*,*,#26740,.T.);
#33372=ORIENTED_EDGE('',*,*,#26741,.F.);
#33373=ORIENTED_EDGE('',*,*,#26731,.F.);
#33374=ORIENTED_EDGE('',*,*,#26742,.F.);
#33375=ORIENTED_EDGE('',*,*,#26725,.F.);
#33376=ORIENTED_EDGE('',*,*,#26742,.T.);
#33377=ORIENTED_EDGE('',*,*,#26739,.F.);
#33378=ORIENTED_EDGE('',*,*,#26743,.F.);
#33379=ORIENTED_EDGE('',*,*,#26722,.F.);
#33380=ORIENTED_EDGE('',*,*,#26741,.T.);
#33381=ORIENTED_EDGE('',*,*,#26724,.F.);
#33382=ORIENTED_EDGE('',*,*,#26744,.F.);
#33383=ORIENTED_EDGE('',*,*,#26727,.F.);
#33384=ORIENTED_EDGE('',*,*,#26743,.T.);
#33385=ORIENTED_EDGE('',*,*,#26734,.F.);
#33386=ORIENTED_EDGE('',*,*,#26744,.T.);
#33387=ORIENTED_EDGE('',*,*,#26723,.F.);
#33388=ORIENTED_EDGE('',*,*,#26745,.F.);
#33389=ORIENTED_EDGE('',*,*,#26736,.F.);
#33390=ORIENTED_EDGE('',*,*,#26746,.F.);
#33391=ORIENTED_EDGE('',*,*,#26717,.F.);
#33392=ORIENTED_EDGE('',*,*,#26746,.T.);
#33393=ORIENTED_EDGE('',*,*,#26740,.F.);
#33394=ORIENTED_EDGE('',*,*,#26747,.F.);
#33395=ORIENTED_EDGE('',*,*,#26704,.F.);
#33396=ORIENTED_EDGE('',*,*,#26709,.T.);
#33397=ORIENTED_EDGE('',*,*,#26720,.F.);
#33398=ORIENTED_EDGE('',*,*,#26748,.F.);
#33399=ORIENTED_EDGE('',*,*,#26729,.F.);
#33400=ORIENTED_EDGE('',*,*,#26747,.T.);
#33401=ORIENTED_EDGE('',*,*,#26732,.F.);
#33402=ORIENTED_EDGE('',*,*,#26748,.T.);
#33403=ORIENTED_EDGE('',*,*,#26714,.F.);
#33404=ORIENTED_EDGE('',*,*,#26749,.T.);
#33405=ORIENTED_EDGE('',*,*,#26700,.F.);
#33406=ORIENTED_EDGE('',*,*,#26750,.F.);
#33407=ORIENTED_EDGE('',*,*,#26751,.T.);
#33408=ORIENTED_EDGE('',*,*,#26752,.F.);
#33409=ORIENTED_EDGE('',*,*,#26753,.T.);
#33410=ORIENTED_EDGE('',*,*,#26754,.F.);
#33411=ORIENTED_EDGE('',*,*,#26751,.F.);
#33412=ORIENTED_EDGE('',*,*,#26755,.F.);
#33413=ORIENTED_EDGE('',*,*,#26756,.T.);
#33414=ORIENTED_EDGE('',*,*,#26701,.F.);
#33415=ORIENTED_EDGE('',*,*,#26749,.F.);
#33416=ORIENTED_EDGE('',*,*,#26757,.F.);
#33417=ORIENTED_EDGE('',*,*,#26758,.T.);
#33418=ORIENTED_EDGE('',*,*,#26759,.F.);
#33419=ORIENTED_EDGE('',*,*,#26753,.F.);
#33420=ORIENTED_EDGE('',*,*,#26760,.F.);
#33421=ORIENTED_EDGE('',*,*,#26719,.F.);
#33422=ORIENTED_EDGE('',*,*,#26758,.F.);
#33423=ORIENTED_EDGE('',*,*,#26718,.F.);
#33424=ORIENTED_EDGE('',*,*,#26761,.F.);
#33425=ORIENTED_EDGE('',*,*,#26762,.F.);
#33426=ORIENTED_EDGE('',*,*,#26763,.T.);
#33427=ORIENTED_EDGE('',*,*,#26738,.T.);
#33428=ORIENTED_EDGE('',*,*,#26764,.T.);
#33429=ORIENTED_EDGE('',*,*,#26765,.F.);
#33430=ORIENTED_EDGE('',*,*,#26766,.T.);
#33431=ORIENTED_EDGE('',*,*,#26767,.T.);
#33432=ORIENTED_EDGE('',*,*,#26662,.F.);
#33433=ORIENTED_EDGE('',*,*,#26768,.T.);
#33434=ORIENTED_EDGE('',*,*,#26769,.F.);
#33435=ORIENTED_EDGE('',*,*,#26770,.F.);
#33436=ORIENTED_EDGE('',*,*,#26771,.F.);
#33437=ORIENTED_EDGE('',*,*,#26766,.F.);
#33438=ORIENTED_EDGE('',*,*,#26772,.F.);
#33439=ORIENTED_EDGE('',*,*,#26687,.T.);
#33440=ORIENTED_EDGE('',*,*,#26773,.F.);
#33441=ORIENTED_EDGE('',*,*,#26764,.F.);
#33442=ORIENTED_EDGE('',*,*,#26661,.F.);
#33443=ORIENTED_EDGE('',*,*,#26774,.T.);
#33444=ORIENTED_EDGE('',*,*,#26657,.F.);
#33445=ORIENTED_EDGE('',*,*,#26775,.T.);
#33446=ORIENTED_EDGE('',*,*,#26768,.F.);
#33447=ORIENTED_EDGE('',*,*,#26776,.F.);
#33448=ORIENTED_EDGE('',*,*,#26774,.F.);
#33449=ORIENTED_EDGE('',*,*,#26777,.F.);
#33450=ORIENTED_EDGE('',*,*,#26686,.F.);
#33451=ORIENTED_EDGE('',*,*,#26658,.F.);
#33452=ORIENTED_EDGE('',*,*,#26684,.T.);
#33453=ORIENTED_EDGE('',*,*,#26778,.F.);
#33454=ORIENTED_EDGE('',*,*,#26779,.T.);
#33455=ORIENTED_EDGE('',*,*,#26780,.F.);
#33456=ORIENTED_EDGE('',*,*,#26781,.T.);
#33457=ORIENTED_EDGE('',*,*,#26782,.F.);
#33458=ORIENTED_EDGE('',*,*,#26779,.F.);
#33459=ORIENTED_EDGE('',*,*,#26783,.F.);
#33460=ORIENTED_EDGE('',*,*,#26784,.T.);
#33461=ORIENTED_EDGE('',*,*,#26785,.F.);
#33462=ORIENTED_EDGE('',*,*,#26781,.F.);
#33463=ORIENTED_EDGE('',*,*,#26786,.F.);
#33464=ORIENTED_EDGE('',*,*,#26678,.T.);
#33465=ORIENTED_EDGE('',*,*,#26787,.F.);
#33466=ORIENTED_EDGE('',*,*,#26682,.F.);
#33467=ORIENTED_EDGE('',*,*,#26681,.F.);
#33468=ORIENTED_EDGE('',*,*,#26788,.F.);
#33469=ORIENTED_EDGE('',*,*,#26789,.T.);
#33470=ORIENTED_EDGE('',*,*,#26790,.F.);
#33471=ORIENTED_EDGE('',*,*,#26784,.F.);
#33472=ORIENTED_EDGE('',*,*,#26791,.F.);
#33473=ORIENTED_EDGE('',*,*,#26789,.F.);
#33474=ORIENTED_EDGE('',*,*,#26792,.F.);
#33475=ORIENTED_EDGE('',*,*,#26680,.F.);
#33476=ORIENTED_EDGE('',*,*,#26793,.F.);
#33477=ORIENTED_EDGE('',*,*,#26794,.T.);
#33478=ORIENTED_EDGE('',*,*,#26773,.T.);
#33479=ORIENTED_EDGE('',*,*,#26676,.F.);
#33480=ORIENTED_EDGE('',*,*,#26795,.F.);
#33481=ORIENTED_EDGE('',*,*,#26674,.T.);
#33482=ORIENTED_EDGE('',*,*,#26777,.T.);
#33483=ORIENTED_EDGE('',*,*,#26796,.F.);
#33484=ORIENTED_EDGE('',*,*,#26797,.F.);
#33485=ORIENTED_EDGE('',*,*,#26798,.T.);
#33486=ORIENTED_EDGE('',*,*,#26799,.T.);
#33487=ORIENTED_EDGE('',*,*,#26800,.T.);
#33488=ORIENTED_EDGE('',*,*,#26801,.T.);
#33489=ORIENTED_EDGE('',*,*,#26802,.T.);
#33490=ORIENTED_EDGE('',*,*,#26675,.T.);
#33491=ORIENTED_EDGE('',*,*,#26803,.F.);
#33492=ORIENTED_EDGE('',*,*,#26765,.T.);
#33493=ORIENTED_EDGE('',*,*,#26794,.F.);
#33494=ORIENTED_EDGE('',*,*,#26804,.F.);
#33495=ORIENTED_EDGE('',*,*,#26805,.T.);
#33496=ORIENTED_EDGE('',*,*,#26796,.T.);
#33497=ORIENTED_EDGE('',*,*,#26776,.T.);
#33498=ORIENTED_EDGE('',*,*,#26806,.F.);
#33499=ORIENTED_EDGE('',*,*,#26807,.F.);
#33500=ORIENTED_EDGE('',*,*,#26808,.F.);
#33501=ORIENTED_EDGE('',*,*,#26802,.F.);
#33502=ORIENTED_EDGE('',*,*,#26809,.T.);
#33503=ORIENTED_EDGE('',*,*,#26810,.T.);
#33504=ORIENTED_EDGE('',*,*,#26804,.T.);
#33505=ORIENTED_EDGE('',*,*,#26795,.T.);
#33506=ORIENTED_EDGE('',*,*,#26811,.F.);
#33507=ORIENTED_EDGE('',*,*,#26812,.T.);
#33508=ORIENTED_EDGE('',*,*,#26798,.F.);
#33509=ORIENTED_EDGE('',*,*,#26797,.T.);
#33510=ORIENTED_EDGE('',*,*,#26808,.T.);
#33511=ORIENTED_EDGE('',*,*,#26813,.T.);
#33512=ORIENTED_EDGE('',*,*,#26814,.T.);
#33513=ORIENTED_EDGE('',*,*,#26815,.T.);
#33514=ORIENTED_EDGE('',*,*,#26813,.F.);
#33515=ORIENTED_EDGE('',*,*,#26816,.T.);
#33516=ORIENTED_EDGE('',*,*,#26817,.T.);
#33517=ORIENTED_EDGE('',*,*,#26818,.T.);
#33518=ORIENTED_EDGE('',*,*,#26819,.T.);
#33519=ORIENTED_EDGE('',*,*,#26820,.T.);
#33520=ORIENTED_EDGE('',*,*,#26800,.F.);
#33521=ORIENTED_EDGE('',*,*,#26821,.F.);
#33522=ORIENTED_EDGE('',*,*,#26814,.F.);
#33523=ORIENTED_EDGE('',*,*,#26821,.T.);
#33524=ORIENTED_EDGE('',*,*,#26799,.F.);
#33525=ORIENTED_EDGE('',*,*,#26822,.F.);
#33526=ORIENTED_EDGE('',*,*,#26816,.F.);
#33527=ORIENTED_EDGE('',*,*,#26822,.T.);
#33528=ORIENTED_EDGE('',*,*,#26812,.F.);
#33529=ORIENTED_EDGE('',*,*,#26823,.F.);
#33530=ORIENTED_EDGE('',*,*,#26817,.F.);
#33531=ORIENTED_EDGE('',*,*,#26824,.T.);
#33532=ORIENTED_EDGE('',*,*,#26677,.T.);
#33533=ORIENTED_EDGE('',*,*,#26825,.T.);
#33534=ORIENTED_EDGE('',*,*,#26818,.F.);
#33535=ORIENTED_EDGE('',*,*,#26826,.T.);
#33536=ORIENTED_EDGE('',*,*,#26809,.F.);
#33537=ORIENTED_EDGE('',*,*,#26827,.F.);
#33538=ORIENTED_EDGE('',*,*,#26819,.F.);
#33539=ORIENTED_EDGE('',*,*,#26827,.T.);
#33540=ORIENTED_EDGE('',*,*,#26801,.F.);
#33541=ORIENTED_EDGE('',*,*,#26820,.F.);
#33542=ORIENTED_EDGE('',*,*,#26815,.F.);
#33543=ORIENTED_EDGE('',*,*,#26828,.F.);
#33544=ORIENTED_EDGE('',*,*,#26786,.T.);
#33545=ORIENTED_EDGE('',*,*,#26829,.F.);
#33546=ORIENTED_EDGE('',*,*,#26805,.F.);
#33547=ORIENTED_EDGE('',*,*,#26685,.T.);
#33548=ORIENTED_EDGE('',*,*,#26780,.T.);
#33549=ORIENTED_EDGE('',*,*,#26782,.T.);
#33550=ORIENTED_EDGE('',*,*,#26785,.T.);
#33551=ORIENTED_EDGE('',*,*,#26790,.T.);
#33552=ORIENTED_EDGE('',*,*,#26793,.T.);
#33553=ORIENTED_EDGE('',*,*,#26679,.T.);
#33554=ORIENTED_EDGE('',*,*,#26788,.T.);
#33555=ORIENTED_EDGE('',*,*,#26830,.F.);
#33556=ORIENTED_EDGE('',*,*,#26778,.T.);
#33557=ORIENTED_EDGE('',*,*,#26831,.F.);
#33558=ORIENTED_EDGE('',*,*,#26807,.T.);
#33559=ORIENTED_EDGE('',*,*,#26832,.F.);
#33560=ORIENTED_EDGE('',*,*,#26787,.T.);
#33561=ORIENTED_EDGE('',*,*,#26824,.F.);
#33562=ORIENTED_EDGE('',*,*,#26823,.T.);
#33563=ORIENTED_EDGE('',*,*,#26825,.F.);
#33564=ORIENTED_EDGE('',*,*,#26792,.T.);
#33565=ORIENTED_EDGE('',*,*,#26833,.F.);
#33566=ORIENTED_EDGE('',*,*,#26826,.F.);
#33567=ORIENTED_EDGE('',*,*,#26833,.T.);
#33568=ORIENTED_EDGE('',*,*,#26791,.T.);
#33569=ORIENTED_EDGE('',*,*,#26828,.T.);
#33570=ORIENTED_EDGE('',*,*,#26810,.F.);
#33571=ORIENTED_EDGE('',*,*,#26831,.T.);
#33572=ORIENTED_EDGE('',*,*,#26683,.T.);
#33573=ORIENTED_EDGE('',*,*,#26832,.T.);
#33574=ORIENTED_EDGE('',*,*,#26811,.T.);
#33575=ORIENTED_EDGE('',*,*,#26834,.F.);
#33576=ORIENTED_EDGE('',*,*,#26752,.T.);
#33577=ORIENTED_EDGE('',*,*,#26754,.T.);
#33578=ORIENTED_EDGE('',*,*,#26759,.T.);
#33579=ORIENTED_EDGE('',*,*,#26835,.F.);
#33580=ORIENTED_EDGE('',*,*,#26806,.T.);
#33581=ORIENTED_EDGE('',*,*,#26772,.T.);
#33582=ORIENTED_EDGE('',*,*,#26803,.T.);
#33583=ORIENTED_EDGE('',*,*,#26836,.T.);
#33584=ORIENTED_EDGE('',*,*,#26757,.T.);
#33585=ORIENTED_EDGE('',*,*,#26834,.T.);
#33586=ORIENTED_EDGE('',*,*,#26829,.T.);
#33587=ORIENTED_EDGE('',*,*,#26783,.T.);
#33588=ORIENTED_EDGE('',*,*,#26830,.T.);
#33589=ORIENTED_EDGE('',*,*,#26835,.T.);
#33590=ORIENTED_EDGE('',*,*,#26762,.T.);
#33591=ORIENTED_EDGE('',*,*,#26663,.T.);
#33592=ORIENTED_EDGE('',*,*,#26767,.F.);
#33593=ORIENTED_EDGE('',*,*,#26771,.T.);
#33594=ORIENTED_EDGE('',*,*,#26770,.T.);
#33595=ORIENTED_EDGE('',*,*,#26769,.T.);
#33596=ORIENTED_EDGE('',*,*,#26775,.F.);
#33597=ORIENTED_EDGE('',*,*,#26656,.T.);
#33598=ORIENTED_EDGE('',*,*,#26837,.F.);
#33599=ORIENTED_EDGE('',*,*,#26838,.F.);
#33600=ORIENTED_EDGE('',*,*,#26155,.T.);
#33601=ORIENTED_EDGE('',*,*,#26839,.F.);
#33602=ORIENTED_EDGE('',*,*,#26241,.T.);
#33603=ORIENTED_EDGE('',*,*,#26840,.F.);
#33604=ORIENTED_EDGE('',*,*,#26346,.T.);
#33605=ORIENTED_EDGE('',*,*,#26626,.T.);
#33606=ORIENTED_EDGE('',*,*,#26841,.T.);
#33607=ORIENTED_EDGE('',*,*,#26652,.T.);
#33608=ORIENTED_EDGE('',*,*,#26842,.F.);
#33609=ORIENTED_EDGE('',*,*,#26111,.T.);
#33610=ORIENTED_EDGE('',*,*,#26843,.F.);
#33611=ORIENTED_EDGE('',*,*,#26103,.T.);
#33612=ORIENTED_EDGE('',*,*,#24844,.T.);
#33613=ORIENTED_EDGE('',*,*,#24850,.T.);
#33614=ORIENTED_EDGE('',*,*,#24856,.T.);
#33615=ORIENTED_EDGE('',*,*,#24863,.T.);
#33616=ORIENTED_EDGE('',*,*,#24830,.T.);
#33617=ORIENTED_EDGE('',*,*,#24943,.T.);
#33618=ORIENTED_EDGE('',*,*,#24936,.T.);
#33619=ORIENTED_EDGE('',*,*,#24957,.T.);
#33620=ORIENTED_EDGE('',*,*,#24902,.T.);
#33621=ORIENTED_EDGE('',*,*,#24896,.T.);
#33622=ORIENTED_EDGE('',*,*,#24889,.T.);
#33623=ORIENTED_EDGE('',*,*,#24882,.T.);
#33624=ORIENTED_EDGE('',*,*,#24876,.T.);
#33625=ORIENTED_EDGE('',*,*,#24870,.T.);
#33626=ORIENTED_EDGE('',*,*,#24916,.T.);
#33627=ORIENTED_EDGE('',*,*,#24922,.T.);
#33628=ORIENTED_EDGE('',*,*,#24929,.T.);
#33629=ORIENTED_EDGE('',*,*,#24909,.T.);
#33630=ORIENTED_EDGE('',*,*,#25399,.F.);
#33631=ORIENTED_EDGE('',*,*,#26638,.T.);
#33632=ORIENTED_EDGE('',*,*,#25343,.F.);
#33633=ORIENTED_EDGE('',*,*,#26637,.T.);
#33634=ORIENTED_EDGE('',*,*,#25287,.F.);
#33635=ORIENTED_EDGE('',*,*,#26636,.T.);
#33636=ORIENTED_EDGE('',*,*,#25231,.F.);
#33637=ORIENTED_EDGE('',*,*,#26635,.T.);
#33638=ORIENTED_EDGE('',*,*,#25175,.F.);
#33639=ORIENTED_EDGE('',*,*,#26634,.T.);
#33640=ORIENTED_EDGE('',*,*,#25125,.F.);
#33641=ORIENTED_EDGE('',*,*,#26633,.T.);
#33642=ORIENTED_EDGE('',*,*,#25069,.F.);
#33643=ORIENTED_EDGE('',*,*,#26632,.T.);
#33644=ORIENTED_EDGE('',*,*,#26620,.F.);
#33645=ORIENTED_EDGE('',*,*,#26631,.T.);
#33646=ORIENTED_EDGE('',*,*,#26564,.F.);
#33647=ORIENTED_EDGE('',*,*,#26630,.T.);
#33648=ORIENTED_EDGE('',*,*,#26508,.F.);
#33649=ORIENTED_EDGE('',*,*,#26629,.T.);
#33650=ORIENTED_EDGE('',*,*,#26458,.F.);
#33651=ORIENTED_EDGE('',*,*,#26628,.T.);
#33652=ORIENTED_EDGE('',*,*,#26401,.F.);
#33653=ORIENTED_EDGE('',*,*,#26403,.F.);
#33654=ORIENTED_EDGE('',*,*,#26627,.T.);
#33655=ORIENTED_EDGE('',*,*,#26344,.F.);
#33656=ORIENTED_EDGE('',*,*,#26347,.F.);
#33657=ORIENTED_EDGE('',*,*,#26840,.T.);
#33658=ORIENTED_EDGE('',*,*,#26240,.F.);
#33659=ORIENTED_EDGE('',*,*,#26242,.F.);
#33660=ORIENTED_EDGE('',*,*,#26839,.T.);
#33661=ORIENTED_EDGE('',*,*,#26154,.F.);
#33662=ORIENTED_EDGE('',*,*,#26156,.F.);
#33663=ORIENTED_EDGE('',*,*,#26838,.T.);
#33664=ORIENTED_EDGE('',*,*,#26102,.F.);
#33665=ORIENTED_EDGE('',*,*,#26104,.F.);
#33666=ORIENTED_EDGE('',*,*,#26843,.T.);
#33667=ORIENTED_EDGE('',*,*,#26110,.F.);
#33668=ORIENTED_EDGE('',*,*,#26112,.F.);
#33669=ORIENTED_EDGE('',*,*,#26842,.T.);
#33670=ORIENTED_EDGE('',*,*,#26651,.T.);
#33671=ORIENTED_EDGE('',*,*,#26052,.F.);
#33672=ORIENTED_EDGE('',*,*,#26054,.F.);
#33673=ORIENTED_EDGE('',*,*,#26650,.T.);
#33674=ORIENTED_EDGE('',*,*,#25997,.F.);
#33675=ORIENTED_EDGE('',*,*,#26649,.T.);
#33676=ORIENTED_EDGE('',*,*,#25947,.F.);
#33677=ORIENTED_EDGE('',*,*,#26648,.T.);
#33678=ORIENTED_EDGE('',*,*,#25891,.F.);
#33679=ORIENTED_EDGE('',*,*,#26647,.T.);
#33680=ORIENTED_EDGE('',*,*,#25835,.F.);
#33681=ORIENTED_EDGE('',*,*,#26646,.T.);
#33682=ORIENTED_EDGE('',*,*,#25779,.F.);
#33683=ORIENTED_EDGE('',*,*,#26645,.T.);
#33684=ORIENTED_EDGE('',*,*,#25723,.F.);
#33685=ORIENTED_EDGE('',*,*,#26644,.T.);
#33686=ORIENTED_EDGE('',*,*,#25673,.F.);
#33687=ORIENTED_EDGE('',*,*,#26643,.T.);
#33688=ORIENTED_EDGE('',*,*,#25617,.F.);
#33689=ORIENTED_EDGE('',*,*,#26642,.T.);
#33690=ORIENTED_EDGE('',*,*,#25561,.F.);
#33691=ORIENTED_EDGE('',*,*,#26641,.T.);
#33692=ORIENTED_EDGE('',*,*,#25505,.F.);
#33693=ORIENTED_EDGE('',*,*,#26640,.T.);
#33694=ORIENTED_EDGE('',*,*,#25449,.F.);
#33695=ORIENTED_EDGE('',*,*,#26639,.T.);
#33696=ORIENTED_EDGE('',*,*,#25442,.T.);
#33697=ORIENTED_EDGE('',*,*,#25436,.T.);
#33698=ORIENTED_EDGE('',*,*,#25336,.T.);
#33699=ORIENTED_EDGE('',*,*,#25330,.T.);
#33700=ORIENTED_EDGE('',*,*,#25324,.T.);
#33701=ORIENTED_EDGE('',*,*,#25380,.T.);
#33702=ORIENTED_EDGE('',*,*,#25554,.T.);
#33703=ORIENTED_EDGE('',*,*,#25542,.T.);
#33704=ORIENTED_EDGE('',*,*,#25548,.T.);
#33705=ORIENTED_EDGE('',*,*,#25604,.T.);
#33706=ORIENTED_EDGE('',*,*,#25598,.T.);
#33707=ORIENTED_EDGE('',*,*,#25492,.T.);
#33708=ORIENTED_EDGE('',*,*,#25486,.T.);
#33709=ORIENTED_EDGE('',*,*,#25498,.T.);
#33710=ORIENTED_EDGE('',*,*,#26433,.T.);
#33711=ORIENTED_EDGE('',*,*,#26427,.T.);
#33712=ORIENTED_EDGE('',*,*,#26421,.T.);
#33713=ORIENTED_EDGE('',*,*,#26377,.T.);
#33714=ORIENTED_EDGE('',*,*,#26527,.T.);
#33715=ORIENTED_EDGE('',*,*,#26489,.T.);
#33716=ORIENTED_EDGE('',*,*,#26483,.T.);
#33717=ORIENTED_EDGE('',*,*,#26477,.T.);
#33718=ORIENTED_EDGE('',*,*,#26308,.T.);
#33719=ORIENTED_EDGE('',*,*,#26272,.T.);
#33720=ORIENTED_EDGE('',*,*,#26260,.T.);
#33721=ORIENTED_EDGE('',*,*,#26266,.T.);
#33722=ORIENTED_EDGE('',*,*,#26365,.T.);
#33723=ORIENTED_EDGE('',*,*,#26371,.T.);
#33724=ORIENTED_EDGE('',*,*,#26314,.T.);
#33725=ORIENTED_EDGE('',*,*,#26320,.T.);
#33726=ORIENTED_EDGE('',*,*,#25268,.T.);
#33727=ORIENTED_EDGE('',*,*,#25100,.T.);
#33728=ORIENTED_EDGE('',*,*,#25094,.T.);
#33729=ORIENTED_EDGE('',*,*,#25088,.T.);
#33730=ORIENTED_EDGE('',*,*,#25274,.T.);
#33731=ORIENTED_EDGE('',*,*,#25280,.T.);
#33732=ORIENTED_EDGE('',*,*,#26589,.T.);
#33733=ORIENTED_EDGE('',*,*,#26583,.T.);
#33734=ORIENTED_EDGE('',*,*,#26539,.T.);
#33735=ORIENTED_EDGE('',*,*,#26533,.T.);
#33736=ORIENTED_EDGE('',*,*,#25044,.T.);
#33737=ORIENTED_EDGE('',*,*,#25038,.T.);
#33738=ORIENTED_EDGE('',*,*,#25032,.T.);
#33739=ORIENTED_EDGE('',*,*,#26595,.T.);
#33740=ORIENTED_EDGE('',*,*,#25990,.T.);
#33741=ORIENTED_EDGE('',*,*,#26034,.T.);
#33742=ORIENTED_EDGE('',*,*,#26040,.T.);
#33743=ORIENTED_EDGE('',*,*,#26046,.T.);
#33744=ORIENTED_EDGE('',*,*,#25940,.T.);
#33745=ORIENTED_EDGE('',*,*,#25934,.T.);
#33746=ORIENTED_EDGE('',*,*,#25928,.T.);
#33747=ORIENTED_EDGE('',*,*,#25984,.T.);
#33748=ORIENTED_EDGE('',*,*,#26148,.T.);
#33749=ORIENTED_EDGE('',*,*,#26198,.T.);
#33750=ORIENTED_EDGE('',*,*,#26192,.T.);
#33751=ORIENTED_EDGE('',*,*,#26090,.T.);
#33752=ORIENTED_EDGE('',*,*,#26096,.T.);
#33753=ORIENTED_EDGE('',*,*,#25716,.T.);
#33754=ORIENTED_EDGE('',*,*,#25710,.T.);
#33755=ORIENTED_EDGE('',*,*,#25760,.T.);
#33756=ORIENTED_EDGE('',*,*,#25610,.T.);
#33757=ORIENTED_EDGE('',*,*,#25666,.T.);
#33758=ORIENTED_EDGE('',*,*,#25654,.T.);
#33759=ORIENTED_EDGE('',*,*,#25660,.T.);
#33760=ORIENTED_EDGE('',*,*,#25872,.T.);
#33761=ORIENTED_EDGE('',*,*,#25878,.T.);
#33762=ORIENTED_EDGE('',*,*,#25884,.T.);
#33763=ORIENTED_EDGE('',*,*,#25766,.T.);
#33764=ORIENTED_EDGE('',*,*,#25772,.T.);
#33765=ORIENTED_EDGE('',*,*,#25828,.T.);
#33766=ORIENTED_EDGE('',*,*,#25822,.T.);
#33767=ORIENTED_EDGE('',*,*,#25816,.T.);
#33768=ORIENTED_EDGE('',*,*,#25188,.T.);
#33769=ORIENTED_EDGE('',*,*,#25076,.T.);
#33770=ORIENTED_EDGE('',*,*,#25020,.T.);
#33771=ORIENTED_EDGE('',*,*,#26571,.T.);
#33772=ORIENTED_EDGE('',*,*,#26409,.T.);
#33773=ORIENTED_EDGE('',*,*,#26353,.T.);
#33774=ORIENTED_EDGE('',*,*,#26515,.T.);
#33775=ORIENTED_EDGE('',*,*,#26465,.T.);
#33776=ORIENTED_EDGE('',*,*,#25518,.T.);
#33777=ORIENTED_EDGE('',*,*,#25462,.T.);
#33778=ORIENTED_EDGE('',*,*,#25630,.T.);
#33779=ORIENTED_EDGE('',*,*,#25574,.T.);
#33780=ORIENTED_EDGE('',*,*,#25412,.T.);
#33781=ORIENTED_EDGE('',*,*,#25356,.T.);
#33782=ORIENTED_EDGE('',*,*,#25300,.T.);
#33783=ORIENTED_EDGE('',*,*,#25244,.T.);
#33784=ORIENTED_EDGE('',*,*,#25848,.T.);
#33785=ORIENTED_EDGE('',*,*,#25792,.T.);
#33786=ORIENTED_EDGE('',*,*,#25686,.T.);
#33787=ORIENTED_EDGE('',*,*,#25736,.T.);
#33788=ORIENTED_EDGE('',*,*,#25904,.T.);
#33789=ORIENTED_EDGE('',*,*,#25960,.T.);
#33790=ORIENTED_EDGE('',*,*,#26010,.T.);
#33791=ORIENTED_EDGE('',*,*,#26066,.T.);
#33792=ORIENTED_EDGE('',*,*,#26359,.T.);
#33793=ORIENTED_EDGE('',*,*,#26302,.T.);
#33794=ORIENTED_EDGE('',*,*,#26471,.T.);
#33795=ORIENTED_EDGE('',*,*,#26415,.T.);
#33796=ORIENTED_EDGE('',*,*,#26210,.T.);
#33797=ORIENTED_EDGE('',*,*,#26254,.T.);
#33798=ORIENTED_EDGE('',*,*,#26168,.T.);
#33799=ORIENTED_EDGE('',*,*,#26124,.T.);
#33800=ORIENTED_EDGE('',*,*,#25294,.T.);
#33801=ORIENTED_EDGE('',*,*,#25350,.T.);
#33802=ORIENTED_EDGE('',*,*,#25456,.T.);
#33803=ORIENTED_EDGE('',*,*,#25406,.T.);
#33804=ORIENTED_EDGE('',*,*,#25238,.T.);
#33805=ORIENTED_EDGE('',*,*,#25182,.T.);
#33806=ORIENTED_EDGE('',*,*,#25144,.T.);
#33807=ORIENTED_EDGE('',*,*,#25138,.T.);
#33808=ORIENTED_EDGE('',*,*,#25150,.T.);
#33809=ORIENTED_EDGE('',*,*,#25156,.T.);
#33810=ORIENTED_EDGE('',*,*,#25212,.T.);
#33811=ORIENTED_EDGE('',*,*,#25218,.T.);
#33812=ORIENTED_EDGE('',*,*,#25224,.T.);
#33813=ORIENTED_EDGE('',*,*,#25898,.T.);
#33814=ORIENTED_EDGE('',*,*,#25842,.T.);
#33815=ORIENTED_EDGE('',*,*,#25730,.T.);
#33816=ORIENTED_EDGE('',*,*,#25786,.T.);
#33817=ORIENTED_EDGE('',*,*,#25568,.T.);
#33818=ORIENTED_EDGE('',*,*,#25512,.T.);
#33819=ORIENTED_EDGE('',*,*,#25680,.T.);
#33820=ORIENTED_EDGE('',*,*,#25624,.T.);
#33821=ORIENTED_EDGE('',*,*,#25954,.T.);
#33822=ORIENTED_EDGE('',*,*,#26004,.T.);
#33823=ORIENTED_EDGE('',*,*,#26060,.T.);
#33824=ORIENTED_EDGE('',*,*,#26118,.T.);
#33825=ORIENTED_EDGE('',*,*,#26248,.T.);
#33826=ORIENTED_EDGE('',*,*,#26296,.T.);
#33827=ORIENTED_EDGE('',*,*,#26162,.T.);
#33828=ORIENTED_EDGE('',*,*,#26204,.T.);
#33829=ORIENTED_EDGE('',*,*,#25910,.T.);
#33830=ORIENTED_EDGE('',*,*,#25866,.T.);
#33831=ORIENTED_EDGE('',*,*,#25860,.T.);
#33832=ORIENTED_EDGE('',*,*,#25854,.T.);
#33833=ORIENTED_EDGE('',*,*,#25916,.T.);
#33834=ORIENTED_EDGE('',*,*,#25922,.T.);
#33835=ORIENTED_EDGE('',*,*,#25966,.T.);
#33836=ORIENTED_EDGE('',*,*,#25972,.T.);
#33837=ORIENTED_EDGE('',*,*,#25748,.T.);
#33838=ORIENTED_EDGE('',*,*,#25742,.T.);
#33839=ORIENTED_EDGE('',*,*,#25704,.T.);
#33840=ORIENTED_EDGE('',*,*,#25698,.T.);
#33841=ORIENTED_EDGE('',*,*,#25810,.T.);
#33842=ORIENTED_EDGE('',*,*,#25804,.T.);
#33843=ORIENTED_EDGE('',*,*,#25798,.T.);
#33844=ORIENTED_EDGE('',*,*,#25754,.T.);
#33845=ORIENTED_EDGE('',*,*,#26142,.T.);
#33846=ORIENTED_EDGE('',*,*,#26136,.T.);
#33847=ORIENTED_EDGE('',*,*,#26180,.T.);
#33848=ORIENTED_EDGE('',*,*,#26174,.T.);
#33849=ORIENTED_EDGE('',*,*,#26222,.T.);
#33850=ORIENTED_EDGE('',*,*,#26228,.T.);
#33851=ORIENTED_EDGE('',*,*,#26216,.T.);
#33852=ORIENTED_EDGE('',*,*,#26186,.T.);
#33853=ORIENTED_EDGE('',*,*,#26022,.T.);
#33854=ORIENTED_EDGE('',*,*,#26028,.T.);
#33855=ORIENTED_EDGE('',*,*,#26016,.T.);
#33856=ORIENTED_EDGE('',*,*,#25978,.T.);
#33857=ORIENTED_EDGE('',*,*,#26130,.T.);
#33858=ORIENTED_EDGE('',*,*,#26084,.T.);
#33859=ORIENTED_EDGE('',*,*,#26072,.T.);
#33860=ORIENTED_EDGE('',*,*,#26078,.T.);
#33861=ORIENTED_EDGE('',*,*,#25480,.T.);
#33862=ORIENTED_EDGE('',*,*,#25474,.T.);
#33863=ORIENTED_EDGE('',*,*,#25530,.T.);
#33864=ORIENTED_EDGE('',*,*,#25524,.T.);
#33865=ORIENTED_EDGE('',*,*,#25424,.T.);
#33866=ORIENTED_EDGE('',*,*,#25418,.T.);
#33867=ORIENTED_EDGE('',*,*,#25430,.T.);
#33868=ORIENTED_EDGE('',*,*,#25468,.T.);
#33869=ORIENTED_EDGE('',*,*,#25636,.T.);
#33870=ORIENTED_EDGE('',*,*,#25642,.T.);
#33871=ORIENTED_EDGE('',*,*,#25648,.T.);
#33872=ORIENTED_EDGE('',*,*,#25692,.T.);
#33873=ORIENTED_EDGE('',*,*,#25536,.T.);
#33874=ORIENTED_EDGE('',*,*,#25580,.T.);
#33875=ORIENTED_EDGE('',*,*,#25592,.T.);
#33876=ORIENTED_EDGE('',*,*,#25586,.T.);
#33877=ORIENTED_EDGE('',*,*,#25200,.T.);
#33878=ORIENTED_EDGE('',*,*,#25194,.T.);
#33879=ORIENTED_EDGE('',*,*,#25206,.T.);
#33880=ORIENTED_EDGE('',*,*,#25250,.T.);
#33881=ORIENTED_EDGE('',*,*,#25082,.T.);
#33882=ORIENTED_EDGE('',*,*,#25026,.T.);
#33883=ORIENTED_EDGE('',*,*,#26521,.T.);
#33884=ORIENTED_EDGE('',*,*,#26577,.T.);
#33885=ORIENTED_EDGE('',*,*,#25318,.T.);
#33886=ORIENTED_EDGE('',*,*,#25362,.T.);
#33887=ORIENTED_EDGE('',*,*,#25374,.T.);
#33888=ORIENTED_EDGE('',*,*,#25368,.T.);
#33889=ORIENTED_EDGE('',*,*,#25306,.T.);
#33890=ORIENTED_EDGE('',*,*,#25312,.T.);
#33891=ORIENTED_EDGE('',*,*,#25256,.T.);
#33892=ORIENTED_EDGE('',*,*,#25262,.T.);
#33893=ORIENTED_EDGE('',*,*,#26383,.T.);
#33894=ORIENTED_EDGE('',*,*,#26395,.T.);
#33895=ORIENTED_EDGE('',*,*,#26389,.T.);
#33896=ORIENTED_EDGE('',*,*,#26338,.T.);
#33897=ORIENTED_EDGE('',*,*,#26332,.T.);
#33898=ORIENTED_EDGE('',*,*,#26451,.T.);
#33899=ORIENTED_EDGE('',*,*,#26445,.T.);
#33900=ORIENTED_EDGE('',*,*,#26439,.T.);
#33901=ORIENTED_EDGE('',*,*,#26234,.T.);
#33902=ORIENTED_EDGE('',*,*,#26326,.T.);
#33903=ORIENTED_EDGE('',*,*,#26278,.T.);
#33904=ORIENTED_EDGE('',*,*,#26290,.T.);
#33905=ORIENTED_EDGE('',*,*,#26284,.T.);
#33906=ORIENTED_EDGE('',*,*,#25062,.T.);
#33907=ORIENTED_EDGE('',*,*,#25056,.T.);
#33908=ORIENTED_EDGE('',*,*,#25050,.T.);
#33909=ORIENTED_EDGE('',*,*,#25168,.T.);
#33910=ORIENTED_EDGE('',*,*,#25162,.T.);
#33911=ORIENTED_EDGE('',*,*,#25118,.T.);
#33912=ORIENTED_EDGE('',*,*,#25112,.T.);
#33913=ORIENTED_EDGE('',*,*,#25106,.T.);
#33914=ORIENTED_EDGE('',*,*,#26551,.T.);
#33915=ORIENTED_EDGE('',*,*,#26545,.T.);
#33916=ORIENTED_EDGE('',*,*,#26495,.T.);
#33917=ORIENTED_EDGE('',*,*,#26501,.T.);
#33918=ORIENTED_EDGE('',*,*,#26613,.T.);
#33919=ORIENTED_EDGE('',*,*,#26607,.T.);
#33920=ORIENTED_EDGE('',*,*,#26601,.T.);
#33921=ORIENTED_EDGE('',*,*,#26557,.T.);
#33922=ORIENTED_EDGE('',*,*,#25132,.T.);
#33923=ORIENTED_EDGE('',*,*,#24568,.T.);
#33924=ORIENTED_EDGE('',*,*,#24562,.T.);
#33925=ORIENTED_EDGE('',*,*,#24556,.T.);
#33926=ORIENTED_EDGE('',*,*,#24550,.T.);
#33927=ORIENTED_EDGE('',*,*,#24544,.T.);
#33928=ORIENTED_EDGE('',*,*,#24538,.T.);
#33929=ORIENTED_EDGE('',*,*,#26669,.T.);
#33930=ORIENTED_EDGE('',*,*,#25386,.T.);
#33931=ORIENTED_EDGE('',*,*,#25392,.T.);
#33932=ORIENTED_EDGE('',*,*,#26844,.T.);
#33933=ORIENTED_EDGE('',*,*,#26655,.T.);
#33934=ORIENTED_EDGE('',*,*,#26845,.T.);
#33935=ORIENTED_EDGE('',*,*,#26625,.T.);
#33936=ORIENTED_EDGE('',*,*,#26845,.F.);
#33937=ORIENTED_EDGE('',*,*,#26837,.T.);
#33938=ORIENTED_EDGE('',*,*,#26844,.F.);
#33939=ORIENTED_EDGE('',*,*,#26841,.F.);
#33940=ORIENTED_EDGE('',*,*,#26721,.F.);
#33941=ORIENTED_EDGE('',*,*,#26706,.F.);
#33942=ORIENTED_EDGE('',*,*,#26708,.T.);
#33943=ORIENTED_EDGE('',*,*,#26733,.T.);
#33944=ORIENTED_EDGE('',*,*,#26763,.F.);
#33945=ORIENTED_EDGE('',*,*,#26737,.T.);
#33946=ORIENTED_EDGE('',*,*,#26745,.T.);
#33947=ORIENTED_EDGE('',*,*,#26716,.F.);
#33948=ORIENTED_EDGE('',*,*,#26702,.F.);
#33949=ORIENTED_EDGE('',*,*,#26756,.F.);
#33950=ORIENTED_EDGE('',*,*,#26836,.F.);
#33951=ORIENTED_EDGE('',*,*,#26761,.T.);
#33952=ORIENTED_EDGE('',*,*,#26711,.F.);
#33953=ORIENTED_EDGE('',*,*,#26760,.T.);
#33954=ORIENTED_EDGE('',*,*,#26846,.T.);
#33955=ORIENTED_EDGE('',*,*,#26750,.T.);
#33956=ORIENTED_EDGE('',*,*,#26713,.T.);
#33957=ORIENTED_EDGE('',*,*,#26847,.F.);
#33958=ORIENTED_EDGE('',*,*,#26712,.F.);
#33959=ORIENTED_EDGE('',*,*,#26846,.F.);
#33960=ORIENTED_EDGE('',*,*,#26755,.T.);
#33961=ORIENTED_EDGE('',*,*,#26847,.T.);
#33962=ORIENTED_EDGE('',*,*,#26622,.F.);
#33963=ORIENTED_EDGE('',*,*,#26617,.F.);
#33964=ORIENTED_EDGE('',*,*,#26624,.T.);
#33965=ORIENTED_EDGE('',*,*,#26614,.F.);
#33966=ORIENTED_EDGE('',*,*,#26611,.F.);
#33967=ORIENTED_EDGE('',*,*,#26616,.T.);
#33968=ORIENTED_EDGE('',*,*,#26608,.F.);
#33969=ORIENTED_EDGE('',*,*,#26605,.F.);
#33970=ORIENTED_EDGE('',*,*,#26610,.T.);
#33971=ORIENTED_EDGE('',*,*,#26602,.F.);
#33972=ORIENTED_EDGE('',*,*,#26599,.F.);
#33973=ORIENTED_EDGE('',*,*,#26604,.T.);
#33974=ORIENTED_EDGE('',*,*,#26596,.F.);
#33975=ORIENTED_EDGE('',*,*,#26593,.F.);
#33976=ORIENTED_EDGE('',*,*,#26598,.T.);
#33977=ORIENTED_EDGE('',*,*,#26590,.F.);
#33978=ORIENTED_EDGE('',*,*,#26587,.F.);
#33979=ORIENTED_EDGE('',*,*,#26592,.T.);
#33980=ORIENTED_EDGE('',*,*,#26584,.F.);
#33981=ORIENTED_EDGE('',*,*,#26581,.F.);
#33982=ORIENTED_EDGE('',*,*,#26586,.T.);
#33983=ORIENTED_EDGE('',*,*,#26578,.F.);
#33984=ORIENTED_EDGE('',*,*,#26575,.F.);
#33985=ORIENTED_EDGE('',*,*,#26580,.T.);
#33986=ORIENTED_EDGE('',*,*,#26572,.F.);
#33987=ORIENTED_EDGE('',*,*,#26569,.F.);
#33988=ORIENTED_EDGE('',*,*,#26574,.T.);
#33989=ORIENTED_EDGE('',*,*,#26566,.F.);
#33990=ORIENTED_EDGE('',*,*,#26561,.F.);
#33991=ORIENTED_EDGE('',*,*,#26568,.T.);
#33992=ORIENTED_EDGE('',*,*,#26558,.F.);
#33993=ORIENTED_EDGE('',*,*,#26555,.F.);
#33994=ORIENTED_EDGE('',*,*,#26560,.T.);
#33995=ORIENTED_EDGE('',*,*,#26552,.F.);
#33996=ORIENTED_EDGE('',*,*,#26549,.F.);
#33997=ORIENTED_EDGE('',*,*,#26554,.T.);
#33998=ORIENTED_EDGE('',*,*,#26546,.F.);
#33999=ORIENTED_EDGE('',*,*,#26543,.F.);
#34000=ORIENTED_EDGE('',*,*,#26548,.T.);
#34001=ORIENTED_EDGE('',*,*,#26540,.F.);
#34002=ORIENTED_EDGE('',*,*,#26537,.F.);
#34003=ORIENTED_EDGE('',*,*,#26542,.T.);
#34004=ORIENTED_EDGE('',*,*,#26534,.F.);
#34005=ORIENTED_EDGE('',*,*,#26531,.F.);
#34006=ORIENTED_EDGE('',*,*,#26536,.T.);
#34007=ORIENTED_EDGE('',*,*,#26528,.F.);
#34008=ORIENTED_EDGE('',*,*,#26525,.F.);
#34009=ORIENTED_EDGE('',*,*,#26530,.T.);
#34010=ORIENTED_EDGE('',*,*,#26522,.F.);
#34011=ORIENTED_EDGE('',*,*,#26519,.F.);
#34012=ORIENTED_EDGE('',*,*,#26524,.T.);
#34013=ORIENTED_EDGE('',*,*,#26516,.F.);
#34014=ORIENTED_EDGE('',*,*,#26513,.F.);
#34015=ORIENTED_EDGE('',*,*,#26518,.T.);
#34016=ORIENTED_EDGE('',*,*,#26510,.F.);
#34017=ORIENTED_EDGE('',*,*,#26505,.F.);
#34018=ORIENTED_EDGE('',*,*,#26512,.T.);
#34019=ORIENTED_EDGE('',*,*,#26502,.F.);
#34020=ORIENTED_EDGE('',*,*,#26499,.F.);
#34021=ORIENTED_EDGE('',*,*,#26504,.T.);
#34022=ORIENTED_EDGE('',*,*,#26496,.F.);
#34023=ORIENTED_EDGE('',*,*,#26493,.F.);
#34024=ORIENTED_EDGE('',*,*,#26498,.T.);
#34025=ORIENTED_EDGE('',*,*,#26490,.F.);
#34026=ORIENTED_EDGE('',*,*,#26487,.F.);
#34027=ORIENTED_EDGE('',*,*,#26492,.T.);
#34028=ORIENTED_EDGE('',*,*,#26484,.F.);
#34029=ORIENTED_EDGE('',*,*,#26481,.F.);
#34030=ORIENTED_EDGE('',*,*,#26486,.T.);
#34031=ORIENTED_EDGE('',*,*,#26478,.F.);
#34032=ORIENTED_EDGE('',*,*,#26475,.F.);
#34033=ORIENTED_EDGE('',*,*,#26480,.T.);
#34034=ORIENTED_EDGE('',*,*,#26472,.F.);
#34035=ORIENTED_EDGE('',*,*,#26469,.F.);
#34036=ORIENTED_EDGE('',*,*,#26474,.T.);
#34037=ORIENTED_EDGE('',*,*,#26466,.F.);
#34038=ORIENTED_EDGE('',*,*,#26463,.F.);
#34039=ORIENTED_EDGE('',*,*,#26468,.T.);
#34040=ORIENTED_EDGE('',*,*,#26460,.F.);
#34041=ORIENTED_EDGE('',*,*,#26455,.F.);
#34042=ORIENTED_EDGE('',*,*,#26462,.T.);
#34043=ORIENTED_EDGE('',*,*,#26452,.F.);
#34044=ORIENTED_EDGE('',*,*,#26449,.F.);
#34045=ORIENTED_EDGE('',*,*,#26454,.T.);
#34046=ORIENTED_EDGE('',*,*,#26446,.F.);
#34047=ORIENTED_EDGE('',*,*,#26443,.F.);
#34048=ORIENTED_EDGE('',*,*,#26448,.T.);
#34049=ORIENTED_EDGE('',*,*,#26440,.F.);
#34050=ORIENTED_EDGE('',*,*,#26437,.F.);
#34051=ORIENTED_EDGE('',*,*,#26442,.T.);
#34052=ORIENTED_EDGE('',*,*,#26434,.F.);
#34053=ORIENTED_EDGE('',*,*,#26431,.F.);
#34054=ORIENTED_EDGE('',*,*,#26436,.T.);
#34055=ORIENTED_EDGE('',*,*,#26428,.F.);
#34056=ORIENTED_EDGE('',*,*,#26425,.F.);
#34057=ORIENTED_EDGE('',*,*,#26430,.T.);
#34058=ORIENTED_EDGE('',*,*,#26422,.F.);
#34059=ORIENTED_EDGE('',*,*,#26419,.F.);
#34060=ORIENTED_EDGE('',*,*,#26424,.T.);
#34061=ORIENTED_EDGE('',*,*,#26416,.F.);
#34062=ORIENTED_EDGE('',*,*,#26413,.F.);
#34063=ORIENTED_EDGE('',*,*,#26418,.T.);
#34064=ORIENTED_EDGE('',*,*,#26410,.F.);
#34065=ORIENTED_EDGE('',*,*,#26407,.F.);
#34066=ORIENTED_EDGE('',*,*,#26412,.T.);
#34067=ORIENTED_EDGE('',*,*,#26404,.F.);
#34068=ORIENTED_EDGE('',*,*,#26399,.F.);
#34069=ORIENTED_EDGE('',*,*,#26406,.T.);
#34070=ORIENTED_EDGE('',*,*,#26396,.F.);
#34071=ORIENTED_EDGE('',*,*,#26393,.F.);
#34072=ORIENTED_EDGE('',*,*,#26398,.T.);
#34073=ORIENTED_EDGE('',*,*,#26390,.F.);
#34074=ORIENTED_EDGE('',*,*,#26387,.F.);
#34075=ORIENTED_EDGE('',*,*,#26392,.T.);
#34076=ORIENTED_EDGE('',*,*,#26384,.F.);
#34077=ORIENTED_EDGE('',*,*,#26381,.F.);
#34078=ORIENTED_EDGE('',*,*,#26386,.T.);
#34079=ORIENTED_EDGE('',*,*,#26378,.F.);
#34080=ORIENTED_EDGE('',*,*,#26375,.F.);
#34081=ORIENTED_EDGE('',*,*,#26380,.T.);
#34082=ORIENTED_EDGE('',*,*,#26372,.F.);
#34083=ORIENTED_EDGE('',*,*,#26369,.F.);
#34084=ORIENTED_EDGE('',*,*,#26374,.T.);
#34085=ORIENTED_EDGE('',*,*,#26366,.F.);
#34086=ORIENTED_EDGE('',*,*,#26363,.F.);
#34087=ORIENTED_EDGE('',*,*,#26368,.T.);
#34088=ORIENTED_EDGE('',*,*,#26360,.F.);
#34089=ORIENTED_EDGE('',*,*,#26357,.F.);
#34090=ORIENTED_EDGE('',*,*,#26362,.T.);
#34091=ORIENTED_EDGE('',*,*,#26354,.F.);
#34092=ORIENTED_EDGE('',*,*,#26351,.F.);
#34093=ORIENTED_EDGE('',*,*,#26356,.T.);
#34094=ORIENTED_EDGE('',*,*,#26348,.F.);
#34095=ORIENTED_EDGE('',*,*,#26342,.F.);
#34096=ORIENTED_EDGE('',*,*,#26350,.T.);
#34097=ORIENTED_EDGE('',*,*,#26339,.F.);
#34098=ORIENTED_EDGE('',*,*,#26336,.F.);
#34099=ORIENTED_EDGE('',*,*,#26341,.T.);
#34100=ORIENTED_EDGE('',*,*,#26333,.F.);
#34101=ORIENTED_EDGE('',*,*,#26330,.F.);
#34102=ORIENTED_EDGE('',*,*,#26335,.T.);
#34103=ORIENTED_EDGE('',*,*,#26327,.F.);
#34104=ORIENTED_EDGE('',*,*,#26324,.F.);
#34105=ORIENTED_EDGE('',*,*,#26329,.T.);
#34106=ORIENTED_EDGE('',*,*,#26321,.F.);
#34107=ORIENTED_EDGE('',*,*,#26318,.F.);
#34108=ORIENTED_EDGE('',*,*,#26323,.T.);
#34109=ORIENTED_EDGE('',*,*,#26315,.F.);
#34110=ORIENTED_EDGE('',*,*,#26312,.F.);
#34111=ORIENTED_EDGE('',*,*,#26317,.T.);
#34112=ORIENTED_EDGE('',*,*,#26309,.F.);
#34113=ORIENTED_EDGE('',*,*,#26306,.F.);
#34114=ORIENTED_EDGE('',*,*,#26311,.T.);
#34115=ORIENTED_EDGE('',*,*,#26303,.F.);
#34116=ORIENTED_EDGE('',*,*,#26300,.F.);
#34117=ORIENTED_EDGE('',*,*,#26305,.T.);
#34118=ORIENTED_EDGE('',*,*,#26297,.F.);
#34119=ORIENTED_EDGE('',*,*,#26294,.F.);
#34120=ORIENTED_EDGE('',*,*,#26299,.T.);
#34121=ORIENTED_EDGE('',*,*,#26291,.F.);
#34122=ORIENTED_EDGE('',*,*,#26288,.F.);
#34123=ORIENTED_EDGE('',*,*,#26293,.T.);
#34124=ORIENTED_EDGE('',*,*,#26285,.F.);
#34125=ORIENTED_EDGE('',*,*,#26282,.F.);
#34126=ORIENTED_EDGE('',*,*,#26287,.T.);
#34127=ORIENTED_EDGE('',*,*,#26279,.F.);
#34128=ORIENTED_EDGE('',*,*,#26276,.F.);
#34129=ORIENTED_EDGE('',*,*,#26281,.T.);
#34130=ORIENTED_EDGE('',*,*,#26273,.F.);
#34131=ORIENTED_EDGE('',*,*,#26270,.F.);
#34132=ORIENTED_EDGE('',*,*,#26275,.T.);
#34133=ORIENTED_EDGE('',*,*,#26267,.F.);
#34134=ORIENTED_EDGE('',*,*,#26264,.F.);
#34135=ORIENTED_EDGE('',*,*,#26269,.T.);
#34136=ORIENTED_EDGE('',*,*,#26261,.F.);
#34137=ORIENTED_EDGE('',*,*,#26258,.F.);
#34138=ORIENTED_EDGE('',*,*,#26263,.T.);
#34139=ORIENTED_EDGE('',*,*,#26255,.F.);
#34140=ORIENTED_EDGE('',*,*,#26252,.F.);
#34141=ORIENTED_EDGE('',*,*,#26257,.T.);
#34142=ORIENTED_EDGE('',*,*,#26249,.F.);
#34143=ORIENTED_EDGE('',*,*,#26246,.F.);
#34144=ORIENTED_EDGE('',*,*,#26251,.T.);
#34145=ORIENTED_EDGE('',*,*,#26243,.F.);
#34146=ORIENTED_EDGE('',*,*,#26238,.F.);
#34147=ORIENTED_EDGE('',*,*,#26245,.T.);
#34148=ORIENTED_EDGE('',*,*,#26235,.F.);
#34149=ORIENTED_EDGE('',*,*,#26232,.F.);
#34150=ORIENTED_EDGE('',*,*,#26237,.T.);
#34151=ORIENTED_EDGE('',*,*,#26229,.F.);
#34152=ORIENTED_EDGE('',*,*,#26226,.F.);
#34153=ORIENTED_EDGE('',*,*,#26231,.T.);
#34154=ORIENTED_EDGE('',*,*,#26223,.F.);
#34155=ORIENTED_EDGE('',*,*,#26220,.F.);
#34156=ORIENTED_EDGE('',*,*,#26225,.T.);
#34157=ORIENTED_EDGE('',*,*,#26217,.F.);
#34158=ORIENTED_EDGE('',*,*,#26214,.F.);
#34159=ORIENTED_EDGE('',*,*,#26219,.T.);
#34160=ORIENTED_EDGE('',*,*,#26211,.F.);
#34161=ORIENTED_EDGE('',*,*,#26208,.F.);
#34162=ORIENTED_EDGE('',*,*,#26213,.T.);
#34163=ORIENTED_EDGE('',*,*,#26205,.F.);
#34164=ORIENTED_EDGE('',*,*,#26202,.F.);
#34165=ORIENTED_EDGE('',*,*,#26207,.T.);
#34166=ORIENTED_EDGE('',*,*,#26199,.F.);
#34167=ORIENTED_EDGE('',*,*,#26196,.F.);
#34168=ORIENTED_EDGE('',*,*,#26201,.T.);
#34169=ORIENTED_EDGE('',*,*,#26193,.F.);
#34170=ORIENTED_EDGE('',*,*,#26190,.F.);
#34171=ORIENTED_EDGE('',*,*,#26195,.T.);
#34172=ORIENTED_EDGE('',*,*,#26187,.F.);
#34173=ORIENTED_EDGE('',*,*,#26184,.F.);
#34174=ORIENTED_EDGE('',*,*,#26189,.T.);
#34175=ORIENTED_EDGE('',*,*,#26181,.F.);
#34176=ORIENTED_EDGE('',*,*,#26178,.F.);
#34177=ORIENTED_EDGE('',*,*,#26183,.T.);
#34178=ORIENTED_EDGE('',*,*,#26175,.F.);
#34179=ORIENTED_EDGE('',*,*,#26172,.F.);
#34180=ORIENTED_EDGE('',*,*,#26177,.T.);
#34181=ORIENTED_EDGE('',*,*,#26169,.F.);
#34182=ORIENTED_EDGE('',*,*,#26166,.F.);
#34183=ORIENTED_EDGE('',*,*,#26171,.T.);
#34184=ORIENTED_EDGE('',*,*,#26163,.F.);
#34185=ORIENTED_EDGE('',*,*,#26160,.F.);
#34186=ORIENTED_EDGE('',*,*,#26165,.T.);
#34187=ORIENTED_EDGE('',*,*,#26157,.F.);
#34188=ORIENTED_EDGE('',*,*,#26152,.F.);
#34189=ORIENTED_EDGE('',*,*,#26159,.T.);
#34190=ORIENTED_EDGE('',*,*,#26149,.F.);
#34191=ORIENTED_EDGE('',*,*,#26146,.F.);
#34192=ORIENTED_EDGE('',*,*,#26151,.T.);
#34193=ORIENTED_EDGE('',*,*,#26143,.F.);
#34194=ORIENTED_EDGE('',*,*,#26140,.F.);
#34195=ORIENTED_EDGE('',*,*,#26145,.T.);
#34196=ORIENTED_EDGE('',*,*,#26137,.F.);
#34197=ORIENTED_EDGE('',*,*,#26134,.F.);
#34198=ORIENTED_EDGE('',*,*,#26139,.T.);
#34199=ORIENTED_EDGE('',*,*,#26131,.F.);
#34200=ORIENTED_EDGE('',*,*,#26128,.F.);
#34201=ORIENTED_EDGE('',*,*,#26133,.T.);
#34202=ORIENTED_EDGE('',*,*,#26125,.F.);
#34203=ORIENTED_EDGE('',*,*,#26122,.F.);
#34204=ORIENTED_EDGE('',*,*,#26127,.T.);
#34205=ORIENTED_EDGE('',*,*,#26119,.F.);
#34206=ORIENTED_EDGE('',*,*,#26116,.F.);
#34207=ORIENTED_EDGE('',*,*,#26121,.T.);
#34208=ORIENTED_EDGE('',*,*,#26113,.F.);
#34209=ORIENTED_EDGE('',*,*,#26108,.F.);
#34210=ORIENTED_EDGE('',*,*,#26115,.T.);
#34211=ORIENTED_EDGE('',*,*,#26105,.F.);
#34212=ORIENTED_EDGE('',*,*,#26100,.F.);
#34213=ORIENTED_EDGE('',*,*,#26107,.T.);
#34214=ORIENTED_EDGE('',*,*,#26097,.F.);
#34215=ORIENTED_EDGE('',*,*,#26094,.F.);
#34216=ORIENTED_EDGE('',*,*,#26099,.T.);
#34217=ORIENTED_EDGE('',*,*,#26091,.F.);
#34218=ORIENTED_EDGE('',*,*,#26088,.F.);
#34219=ORIENTED_EDGE('',*,*,#26093,.T.);
#34220=ORIENTED_EDGE('',*,*,#26085,.F.);
#34221=ORIENTED_EDGE('',*,*,#26082,.F.);
#34222=ORIENTED_EDGE('',*,*,#26087,.T.);
#34223=ORIENTED_EDGE('',*,*,#26079,.F.);
#34224=ORIENTED_EDGE('',*,*,#26076,.F.);
#34225=ORIENTED_EDGE('',*,*,#26081,.T.);
#34226=ORIENTED_EDGE('',*,*,#26073,.F.);
#34227=ORIENTED_EDGE('',*,*,#26070,.F.);
#34228=ORIENTED_EDGE('',*,*,#26075,.T.);
#34229=ORIENTED_EDGE('',*,*,#26067,.F.);
#34230=ORIENTED_EDGE('',*,*,#26064,.F.);
#34231=ORIENTED_EDGE('',*,*,#26069,.T.);
#34232=ORIENTED_EDGE('',*,*,#26061,.F.);
#34233=ORIENTED_EDGE('',*,*,#26058,.F.);
#34234=ORIENTED_EDGE('',*,*,#26063,.T.);
#34235=ORIENTED_EDGE('',*,*,#26055,.F.);
#34236=ORIENTED_EDGE('',*,*,#26050,.F.);
#34237=ORIENTED_EDGE('',*,*,#26057,.T.);
#34238=ORIENTED_EDGE('',*,*,#26047,.F.);
#34239=ORIENTED_EDGE('',*,*,#26044,.F.);
#34240=ORIENTED_EDGE('',*,*,#26049,.T.);
#34241=ORIENTED_EDGE('',*,*,#26041,.F.);
#34242=ORIENTED_EDGE('',*,*,#26038,.F.);
#34243=ORIENTED_EDGE('',*,*,#26043,.T.);
#34244=ORIENTED_EDGE('',*,*,#26035,.F.);
#34245=ORIENTED_EDGE('',*,*,#26032,.F.);
#34246=ORIENTED_EDGE('',*,*,#26037,.T.);
#34247=ORIENTED_EDGE('',*,*,#26029,.F.);
#34248=ORIENTED_EDGE('',*,*,#26026,.F.);
#34249=ORIENTED_EDGE('',*,*,#26031,.T.);
#34250=ORIENTED_EDGE('',*,*,#26023,.F.);
#34251=ORIENTED_EDGE('',*,*,#26020,.F.);
#34252=ORIENTED_EDGE('',*,*,#26025,.T.);
#34253=ORIENTED_EDGE('',*,*,#26017,.F.);
#34254=ORIENTED_EDGE('',*,*,#26014,.F.);
#34255=ORIENTED_EDGE('',*,*,#26019,.T.);
#34256=ORIENTED_EDGE('',*,*,#26011,.F.);
#34257=ORIENTED_EDGE('',*,*,#26008,.F.);
#34258=ORIENTED_EDGE('',*,*,#26013,.T.);
#34259=ORIENTED_EDGE('',*,*,#26005,.F.);
#34260=ORIENTED_EDGE('',*,*,#26002,.F.);
#34261=ORIENTED_EDGE('',*,*,#26007,.T.);
#34262=ORIENTED_EDGE('',*,*,#25999,.F.);
#34263=ORIENTED_EDGE('',*,*,#25994,.F.);
#34264=ORIENTED_EDGE('',*,*,#26001,.T.);
#34265=ORIENTED_EDGE('',*,*,#25991,.F.);
#34266=ORIENTED_EDGE('',*,*,#25988,.F.);
#34267=ORIENTED_EDGE('',*,*,#25993,.T.);
#34268=ORIENTED_EDGE('',*,*,#25985,.F.);
#34269=ORIENTED_EDGE('',*,*,#25982,.F.);
#34270=ORIENTED_EDGE('',*,*,#25987,.T.);
#34271=ORIENTED_EDGE('',*,*,#25979,.F.);
#34272=ORIENTED_EDGE('',*,*,#25976,.F.);
#34273=ORIENTED_EDGE('',*,*,#25981,.T.);
#34274=ORIENTED_EDGE('',*,*,#25973,.F.);
#34275=ORIENTED_EDGE('',*,*,#25970,.F.);
#34276=ORIENTED_EDGE('',*,*,#25975,.T.);
#34277=ORIENTED_EDGE('',*,*,#25967,.F.);
#34278=ORIENTED_EDGE('',*,*,#25964,.F.);
#34279=ORIENTED_EDGE('',*,*,#25969,.T.);
#34280=ORIENTED_EDGE('',*,*,#25961,.F.);
#34281=ORIENTED_EDGE('',*,*,#25958,.F.);
#34282=ORIENTED_EDGE('',*,*,#25963,.T.);
#34283=ORIENTED_EDGE('',*,*,#25955,.F.);
#34284=ORIENTED_EDGE('',*,*,#25952,.F.);
#34285=ORIENTED_EDGE('',*,*,#25957,.T.);
#34286=ORIENTED_EDGE('',*,*,#25949,.F.);
#34287=ORIENTED_EDGE('',*,*,#25944,.F.);
#34288=ORIENTED_EDGE('',*,*,#25951,.T.);
#34289=ORIENTED_EDGE('',*,*,#25941,.F.);
#34290=ORIENTED_EDGE('',*,*,#25938,.F.);
#34291=ORIENTED_EDGE('',*,*,#25943,.T.);
#34292=ORIENTED_EDGE('',*,*,#25935,.F.);
#34293=ORIENTED_EDGE('',*,*,#25932,.F.);
#34294=ORIENTED_EDGE('',*,*,#25937,.T.);
#34295=ORIENTED_EDGE('',*,*,#25929,.F.);
#34296=ORIENTED_EDGE('',*,*,#25926,.F.);
#34297=ORIENTED_EDGE('',*,*,#25931,.T.);
#34298=ORIENTED_EDGE('',*,*,#25923,.F.);
#34299=ORIENTED_EDGE('',*,*,#25920,.F.);
#34300=ORIENTED_EDGE('',*,*,#25925,.T.);
#34301=ORIENTED_EDGE('',*,*,#25917,.F.);
#34302=ORIENTED_EDGE('',*,*,#25914,.F.);
#34303=ORIENTED_EDGE('',*,*,#25919,.T.);
#34304=ORIENTED_EDGE('',*,*,#25911,.F.);
#34305=ORIENTED_EDGE('',*,*,#25908,.F.);
#34306=ORIENTED_EDGE('',*,*,#25913,.T.);
#34307=ORIENTED_EDGE('',*,*,#25905,.F.);
#34308=ORIENTED_EDGE('',*,*,#25902,.F.);
#34309=ORIENTED_EDGE('',*,*,#25907,.T.);
#34310=ORIENTED_EDGE('',*,*,#25899,.F.);
#34311=ORIENTED_EDGE('',*,*,#25896,.F.);
#34312=ORIENTED_EDGE('',*,*,#25901,.T.);
#34313=ORIENTED_EDGE('',*,*,#25893,.F.);
#34314=ORIENTED_EDGE('',*,*,#25888,.F.);
#34315=ORIENTED_EDGE('',*,*,#25895,.T.);
#34316=ORIENTED_EDGE('',*,*,#25885,.F.);
#34317=ORIENTED_EDGE('',*,*,#25882,.F.);
#34318=ORIENTED_EDGE('',*,*,#25887,.T.);
#34319=ORIENTED_EDGE('',*,*,#25879,.F.);
#34320=ORIENTED_EDGE('',*,*,#25876,.F.);
#34321=ORIENTED_EDGE('',*,*,#25881,.T.);
#34322=ORIENTED_EDGE('',*,*,#25873,.F.);
#34323=ORIENTED_EDGE('',*,*,#25870,.F.);
#34324=ORIENTED_EDGE('',*,*,#25875,.T.);
#34325=ORIENTED_EDGE('',*,*,#25867,.F.);
#34326=ORIENTED_EDGE('',*,*,#25864,.F.);
#34327=ORIENTED_EDGE('',*,*,#25869,.T.);
#34328=ORIENTED_EDGE('',*,*,#25861,.F.);
#34329=ORIENTED_EDGE('',*,*,#25858,.F.);
#34330=ORIENTED_EDGE('',*,*,#25863,.T.);
#34331=ORIENTED_EDGE('',*,*,#25855,.F.);
#34332=ORIENTED_EDGE('',*,*,#25852,.F.);
#34333=ORIENTED_EDGE('',*,*,#25857,.T.);
#34334=ORIENTED_EDGE('',*,*,#25849,.F.);
#34335=ORIENTED_EDGE('',*,*,#25846,.F.);
#34336=ORIENTED_EDGE('',*,*,#25851,.T.);
#34337=ORIENTED_EDGE('',*,*,#25843,.F.);
#34338=ORIENTED_EDGE('',*,*,#25840,.F.);
#34339=ORIENTED_EDGE('',*,*,#25845,.T.);
#34340=ORIENTED_EDGE('',*,*,#25837,.F.);
#34341=ORIENTED_EDGE('',*,*,#25832,.F.);
#34342=ORIENTED_EDGE('',*,*,#25839,.T.);
#34343=ORIENTED_EDGE('',*,*,#25829,.F.);
#34344=ORIENTED_EDGE('',*,*,#25826,.F.);
#34345=ORIENTED_EDGE('',*,*,#25831,.T.);
#34346=ORIENTED_EDGE('',*,*,#25823,.F.);
#34347=ORIENTED_EDGE('',*,*,#25820,.F.);
#34348=ORIENTED_EDGE('',*,*,#25825,.T.);
#34349=ORIENTED_EDGE('',*,*,#25817,.F.);
#34350=ORIENTED_EDGE('',*,*,#25814,.F.);
#34351=ORIENTED_EDGE('',*,*,#25819,.T.);
#34352=ORIENTED_EDGE('',*,*,#25811,.F.);
#34353=ORIENTED_EDGE('',*,*,#25808,.F.);
#34354=ORIENTED_EDGE('',*,*,#25813,.T.);
#34355=ORIENTED_EDGE('',*,*,#25805,.F.);
#34356=ORIENTED_EDGE('',*,*,#25802,.F.);
#34357=ORIENTED_EDGE('',*,*,#25807,.T.);
#34358=ORIENTED_EDGE('',*,*,#25799,.F.);
#34359=ORIENTED_EDGE('',*,*,#25796,.F.);
#34360=ORIENTED_EDGE('',*,*,#25801,.T.);
#34361=ORIENTED_EDGE('',*,*,#25793,.F.);
#34362=ORIENTED_EDGE('',*,*,#25790,.F.);
#34363=ORIENTED_EDGE('',*,*,#25795,.T.);
#34364=ORIENTED_EDGE('',*,*,#25787,.F.);
#34365=ORIENTED_EDGE('',*,*,#25784,.F.);
#34366=ORIENTED_EDGE('',*,*,#25789,.T.);
#34367=ORIENTED_EDGE('',*,*,#25781,.F.);
#34368=ORIENTED_EDGE('',*,*,#25776,.F.);
#34369=ORIENTED_EDGE('',*,*,#25783,.T.);
#34370=ORIENTED_EDGE('',*,*,#25773,.F.);
#34371=ORIENTED_EDGE('',*,*,#25770,.F.);
#34372=ORIENTED_EDGE('',*,*,#25775,.T.);
#34373=ORIENTED_EDGE('',*,*,#25767,.F.);
#34374=ORIENTED_EDGE('',*,*,#25764,.F.);
#34375=ORIENTED_EDGE('',*,*,#25769,.T.);
#34376=ORIENTED_EDGE('',*,*,#25761,.F.);
#34377=ORIENTED_EDGE('',*,*,#25758,.F.);
#34378=ORIENTED_EDGE('',*,*,#25763,.T.);
#34379=ORIENTED_EDGE('',*,*,#25755,.F.);
#34380=ORIENTED_EDGE('',*,*,#25752,.F.);
#34381=ORIENTED_EDGE('',*,*,#25757,.T.);
#34382=ORIENTED_EDGE('',*,*,#25749,.F.);
#34383=ORIENTED_EDGE('',*,*,#25746,.F.);
#34384=ORIENTED_EDGE('',*,*,#25751,.T.);
#34385=ORIENTED_EDGE('',*,*,#25743,.F.);
#34386=ORIENTED_EDGE('',*,*,#25740,.F.);
#34387=ORIENTED_EDGE('',*,*,#25745,.T.);
#34388=ORIENTED_EDGE('',*,*,#25737,.F.);
#34389=ORIENTED_EDGE('',*,*,#25734,.F.);
#34390=ORIENTED_EDGE('',*,*,#25739,.T.);
#34391=ORIENTED_EDGE('',*,*,#25731,.F.);
#34392=ORIENTED_EDGE('',*,*,#25728,.F.);
#34393=ORIENTED_EDGE('',*,*,#25733,.T.);
#34394=ORIENTED_EDGE('',*,*,#25725,.F.);
#34395=ORIENTED_EDGE('',*,*,#25720,.F.);
#34396=ORIENTED_EDGE('',*,*,#25727,.T.);
#34397=ORIENTED_EDGE('',*,*,#25717,.F.);
#34398=ORIENTED_EDGE('',*,*,#25714,.F.);
#34399=ORIENTED_EDGE('',*,*,#25719,.T.);
#34400=ORIENTED_EDGE('',*,*,#25711,.F.);
#34401=ORIENTED_EDGE('',*,*,#25708,.F.);
#34402=ORIENTED_EDGE('',*,*,#25713,.T.);
#34403=ORIENTED_EDGE('',*,*,#25705,.F.);
#34404=ORIENTED_EDGE('',*,*,#25702,.F.);
#34405=ORIENTED_EDGE('',*,*,#25707,.T.);
#34406=ORIENTED_EDGE('',*,*,#25699,.F.);
#34407=ORIENTED_EDGE('',*,*,#25696,.F.);
#34408=ORIENTED_EDGE('',*,*,#25701,.T.);
#34409=ORIENTED_EDGE('',*,*,#25693,.F.);
#34410=ORIENTED_EDGE('',*,*,#25690,.F.);
#34411=ORIENTED_EDGE('',*,*,#25695,.T.);
#34412=ORIENTED_EDGE('',*,*,#25687,.F.);
#34413=ORIENTED_EDGE('',*,*,#25684,.F.);
#34414=ORIENTED_EDGE('',*,*,#25689,.T.);
#34415=ORIENTED_EDGE('',*,*,#25681,.F.);
#34416=ORIENTED_EDGE('',*,*,#25678,.F.);
#34417=ORIENTED_EDGE('',*,*,#25683,.T.);
#34418=ORIENTED_EDGE('',*,*,#25675,.F.);
#34419=ORIENTED_EDGE('',*,*,#25670,.F.);
#34420=ORIENTED_EDGE('',*,*,#25677,.T.);
#34421=ORIENTED_EDGE('',*,*,#25667,.F.);
#34422=ORIENTED_EDGE('',*,*,#25664,.F.);
#34423=ORIENTED_EDGE('',*,*,#25669,.T.);
#34424=ORIENTED_EDGE('',*,*,#25661,.F.);
#34425=ORIENTED_EDGE('',*,*,#25658,.F.);
#34426=ORIENTED_EDGE('',*,*,#25663,.T.);
#34427=ORIENTED_EDGE('',*,*,#25655,.F.);
#34428=ORIENTED_EDGE('',*,*,#25652,.F.);
#34429=ORIENTED_EDGE('',*,*,#25657,.T.);
#34430=ORIENTED_EDGE('',*,*,#25649,.F.);
#34431=ORIENTED_EDGE('',*,*,#25646,.F.);
#34432=ORIENTED_EDGE('',*,*,#25651,.T.);
#34433=ORIENTED_EDGE('',*,*,#25643,.F.);
#34434=ORIENTED_EDGE('',*,*,#25640,.F.);
#34435=ORIENTED_EDGE('',*,*,#25645,.T.);
#34436=ORIENTED_EDGE('',*,*,#25637,.F.);
#34437=ORIENTED_EDGE('',*,*,#25634,.F.);
#34438=ORIENTED_EDGE('',*,*,#25639,.T.);
#34439=ORIENTED_EDGE('',*,*,#25631,.F.);
#34440=ORIENTED_EDGE('',*,*,#25628,.F.);
#34441=ORIENTED_EDGE('',*,*,#25633,.T.);
#34442=ORIENTED_EDGE('',*,*,#25625,.F.);
#34443=ORIENTED_EDGE('',*,*,#25622,.F.);
#34444=ORIENTED_EDGE('',*,*,#25627,.T.);
#34445=ORIENTED_EDGE('',*,*,#25619,.F.);
#34446=ORIENTED_EDGE('',*,*,#25614,.F.);
#34447=ORIENTED_EDGE('',*,*,#25621,.T.);
#34448=ORIENTED_EDGE('',*,*,#25611,.F.);
#34449=ORIENTED_EDGE('',*,*,#25608,.F.);
#34450=ORIENTED_EDGE('',*,*,#25613,.T.);
#34451=ORIENTED_EDGE('',*,*,#25605,.F.);
#34452=ORIENTED_EDGE('',*,*,#25602,.F.);
#34453=ORIENTED_EDGE('',*,*,#25607,.T.);
#34454=ORIENTED_EDGE('',*,*,#25599,.F.);
#34455=ORIENTED_EDGE('',*,*,#25596,.F.);
#34456=ORIENTED_EDGE('',*,*,#25601,.T.);
#34457=ORIENTED_EDGE('',*,*,#25593,.F.);
#34458=ORIENTED_EDGE('',*,*,#25590,.F.);
#34459=ORIENTED_EDGE('',*,*,#25595,.T.);
#34460=ORIENTED_EDGE('',*,*,#25587,.F.);
#34461=ORIENTED_EDGE('',*,*,#25584,.F.);
#34462=ORIENTED_EDGE('',*,*,#25589,.T.);
#34463=ORIENTED_EDGE('',*,*,#25581,.F.);
#34464=ORIENTED_EDGE('',*,*,#25578,.F.);
#34465=ORIENTED_EDGE('',*,*,#25583,.T.);
#34466=ORIENTED_EDGE('',*,*,#25575,.F.);
#34467=ORIENTED_EDGE('',*,*,#25572,.F.);
#34468=ORIENTED_EDGE('',*,*,#25577,.T.);
#34469=ORIENTED_EDGE('',*,*,#25569,.F.);
#34470=ORIENTED_EDGE('',*,*,#25566,.F.);
#34471=ORIENTED_EDGE('',*,*,#25571,.T.);
#34472=ORIENTED_EDGE('',*,*,#25563,.F.);
#34473=ORIENTED_EDGE('',*,*,#25558,.F.);
#34474=ORIENTED_EDGE('',*,*,#25565,.T.);
#34475=ORIENTED_EDGE('',*,*,#25555,.F.);
#34476=ORIENTED_EDGE('',*,*,#25552,.F.);
#34477=ORIENTED_EDGE('',*,*,#25557,.T.);
#34478=ORIENTED_EDGE('',*,*,#25549,.F.);
#34479=ORIENTED_EDGE('',*,*,#25546,.F.);
#34480=ORIENTED_EDGE('',*,*,#25551,.T.);
#34481=ORIENTED_EDGE('',*,*,#25543,.F.);
#34482=ORIENTED_EDGE('',*,*,#25540,.F.);
#34483=ORIENTED_EDGE('',*,*,#25545,.T.);
#34484=ORIENTED_EDGE('',*,*,#25537,.F.);
#34485=ORIENTED_EDGE('',*,*,#25534,.F.);
#34486=ORIENTED_EDGE('',*,*,#25539,.T.);
#34487=ORIENTED_EDGE('',*,*,#25531,.F.);
#34488=ORIENTED_EDGE('',*,*,#25528,.F.);
#34489=ORIENTED_EDGE('',*,*,#25533,.T.);
#34490=ORIENTED_EDGE('',*,*,#25525,.F.);
#34491=ORIENTED_EDGE('',*,*,#25522,.F.);
#34492=ORIENTED_EDGE('',*,*,#25527,.T.);
#34493=ORIENTED_EDGE('',*,*,#25519,.F.);
#34494=ORIENTED_EDGE('',*,*,#25516,.F.);
#34495=ORIENTED_EDGE('',*,*,#25521,.T.);
#34496=ORIENTED_EDGE('',*,*,#25513,.F.);
#34497=ORIENTED_EDGE('',*,*,#25510,.F.);
#34498=ORIENTED_EDGE('',*,*,#25515,.T.);
#34499=ORIENTED_EDGE('',*,*,#25507,.F.);
#34500=ORIENTED_EDGE('',*,*,#25502,.F.);
#34501=ORIENTED_EDGE('',*,*,#25509,.T.);
#34502=ORIENTED_EDGE('',*,*,#25499,.F.);
#34503=ORIENTED_EDGE('',*,*,#25496,.F.);
#34504=ORIENTED_EDGE('',*,*,#25501,.T.);
#34505=ORIENTED_EDGE('',*,*,#25493,.F.);
#34506=ORIENTED_EDGE('',*,*,#25490,.F.);
#34507=ORIENTED_EDGE('',*,*,#25495,.T.);
#34508=ORIENTED_EDGE('',*,*,#25487,.F.);
#34509=ORIENTED_EDGE('',*,*,#25484,.F.);
#34510=ORIENTED_EDGE('',*,*,#25489,.T.);
#34511=ORIENTED_EDGE('',*,*,#25481,.F.);
#34512=ORIENTED_EDGE('',*,*,#25478,.F.);
#34513=ORIENTED_EDGE('',*,*,#25483,.T.);
#34514=ORIENTED_EDGE('',*,*,#25475,.F.);
#34515=ORIENTED_EDGE('',*,*,#25472,.F.);
#34516=ORIENTED_EDGE('',*,*,#25477,.T.);
#34517=ORIENTED_EDGE('',*,*,#25469,.F.);
#34518=ORIENTED_EDGE('',*,*,#25466,.F.);
#34519=ORIENTED_EDGE('',*,*,#25471,.T.);
#34520=ORIENTED_EDGE('',*,*,#25463,.F.);
#34521=ORIENTED_EDGE('',*,*,#25460,.F.);
#34522=ORIENTED_EDGE('',*,*,#25465,.T.);
#34523=ORIENTED_EDGE('',*,*,#25457,.F.);
#34524=ORIENTED_EDGE('',*,*,#25454,.F.);
#34525=ORIENTED_EDGE('',*,*,#25459,.T.);
#34526=ORIENTED_EDGE('',*,*,#25451,.F.);
#34527=ORIENTED_EDGE('',*,*,#25446,.F.);
#34528=ORIENTED_EDGE('',*,*,#25453,.T.);
#34529=ORIENTED_EDGE('',*,*,#25443,.F.);
#34530=ORIENTED_EDGE('',*,*,#25440,.F.);
#34531=ORIENTED_EDGE('',*,*,#25445,.T.);
#34532=ORIENTED_EDGE('',*,*,#25437,.F.);
#34533=ORIENTED_EDGE('',*,*,#25434,.F.);
#34534=ORIENTED_EDGE('',*,*,#25439,.T.);
#34535=ORIENTED_EDGE('',*,*,#25431,.F.);
#34536=ORIENTED_EDGE('',*,*,#25428,.F.);
#34537=ORIENTED_EDGE('',*,*,#25433,.T.);
#34538=ORIENTED_EDGE('',*,*,#25425,.F.);
#34539=ORIENTED_EDGE('',*,*,#25422,.F.);
#34540=ORIENTED_EDGE('',*,*,#25427,.T.);
#34541=ORIENTED_EDGE('',*,*,#25419,.F.);
#34542=ORIENTED_EDGE('',*,*,#25416,.F.);
#34543=ORIENTED_EDGE('',*,*,#25421,.T.);
#34544=ORIENTED_EDGE('',*,*,#25413,.F.);
#34545=ORIENTED_EDGE('',*,*,#25410,.F.);
#34546=ORIENTED_EDGE('',*,*,#25415,.T.);
#34547=ORIENTED_EDGE('',*,*,#25407,.F.);
#34548=ORIENTED_EDGE('',*,*,#25404,.F.);
#34549=ORIENTED_EDGE('',*,*,#25409,.T.);
#34550=ORIENTED_EDGE('',*,*,#25401,.F.);
#34551=ORIENTED_EDGE('',*,*,#25396,.F.);
#34552=ORIENTED_EDGE('',*,*,#25403,.T.);
#34553=ORIENTED_EDGE('',*,*,#25393,.F.);
#34554=ORIENTED_EDGE('',*,*,#25390,.F.);
#34555=ORIENTED_EDGE('',*,*,#25395,.T.);
#34556=ORIENTED_EDGE('',*,*,#25387,.F.);
#34557=ORIENTED_EDGE('',*,*,#25384,.F.);
#34558=ORIENTED_EDGE('',*,*,#25389,.T.);
#34559=ORIENTED_EDGE('',*,*,#25381,.F.);
#34560=ORIENTED_EDGE('',*,*,#25378,.F.);
#34561=ORIENTED_EDGE('',*,*,#25383,.T.);
#34562=ORIENTED_EDGE('',*,*,#25375,.F.);
#34563=ORIENTED_EDGE('',*,*,#25372,.F.);
#34564=ORIENTED_EDGE('',*,*,#25377,.T.);
#34565=ORIENTED_EDGE('',*,*,#25369,.F.);
#34566=ORIENTED_EDGE('',*,*,#25366,.F.);
#34567=ORIENTED_EDGE('',*,*,#25371,.T.);
#34568=ORIENTED_EDGE('',*,*,#25363,.F.);
#34569=ORIENTED_EDGE('',*,*,#25360,.F.);
#34570=ORIENTED_EDGE('',*,*,#25365,.T.);
#34571=ORIENTED_EDGE('',*,*,#25357,.F.);
#34572=ORIENTED_EDGE('',*,*,#25354,.F.);
#34573=ORIENTED_EDGE('',*,*,#25359,.T.);
#34574=ORIENTED_EDGE('',*,*,#25351,.F.);
#34575=ORIENTED_EDGE('',*,*,#25348,.F.);
#34576=ORIENTED_EDGE('',*,*,#25353,.T.);
#34577=ORIENTED_EDGE('',*,*,#25345,.F.);
#34578=ORIENTED_EDGE('',*,*,#25340,.F.);
#34579=ORIENTED_EDGE('',*,*,#25347,.T.);
#34580=ORIENTED_EDGE('',*,*,#25337,.F.);
#34581=ORIENTED_EDGE('',*,*,#25334,.F.);
#34582=ORIENTED_EDGE('',*,*,#25339,.T.);
#34583=ORIENTED_EDGE('',*,*,#25331,.F.);
#34584=ORIENTED_EDGE('',*,*,#25328,.F.);
#34585=ORIENTED_EDGE('',*,*,#25333,.T.);
#34586=ORIENTED_EDGE('',*,*,#25325,.F.);
#34587=ORIENTED_EDGE('',*,*,#25322,.F.);
#34588=ORIENTED_EDGE('',*,*,#25327,.T.);
#34589=ORIENTED_EDGE('',*,*,#25319,.F.);
#34590=ORIENTED_EDGE('',*,*,#25316,.F.);
#34591=ORIENTED_EDGE('',*,*,#25321,.T.);
#34592=ORIENTED_EDGE('',*,*,#25313,.F.);
#34593=ORIENTED_EDGE('',*,*,#25310,.F.);
#34594=ORIENTED_EDGE('',*,*,#25315,.T.);
#34595=ORIENTED_EDGE('',*,*,#25307,.F.);
#34596=ORIENTED_EDGE('',*,*,#25304,.F.);
#34597=ORIENTED_EDGE('',*,*,#25309,.T.);
#34598=ORIENTED_EDGE('',*,*,#25301,.F.);
#34599=ORIENTED_EDGE('',*,*,#25298,.F.);
#34600=ORIENTED_EDGE('',*,*,#25303,.T.);
#34601=ORIENTED_EDGE('',*,*,#25295,.F.);
#34602=ORIENTED_EDGE('',*,*,#25292,.F.);
#34603=ORIENTED_EDGE('',*,*,#25297,.T.);
#34604=ORIENTED_EDGE('',*,*,#25289,.F.);
#34605=ORIENTED_EDGE('',*,*,#25284,.F.);
#34606=ORIENTED_EDGE('',*,*,#25291,.T.);
#34607=ORIENTED_EDGE('',*,*,#25281,.F.);
#34608=ORIENTED_EDGE('',*,*,#25278,.F.);
#34609=ORIENTED_EDGE('',*,*,#25283,.T.);
#34610=ORIENTED_EDGE('',*,*,#25275,.F.);
#34611=ORIENTED_EDGE('',*,*,#25272,.F.);
#34612=ORIENTED_EDGE('',*,*,#25277,.T.);
#34613=ORIENTED_EDGE('',*,*,#25269,.F.);
#34614=ORIENTED_EDGE('',*,*,#25266,.F.);
#34615=ORIENTED_EDGE('',*,*,#25271,.T.);
#34616=ORIENTED_EDGE('',*,*,#25263,.F.);
#34617=ORIENTED_EDGE('',*,*,#25260,.F.);
#34618=ORIENTED_EDGE('',*,*,#25265,.T.);
#34619=ORIENTED_EDGE('',*,*,#25257,.F.);
#34620=ORIENTED_EDGE('',*,*,#25254,.F.);
#34621=ORIENTED_EDGE('',*,*,#25259,.T.);
#34622=ORIENTED_EDGE('',*,*,#25251,.F.);
#34623=ORIENTED_EDGE('',*,*,#25248,.F.);
#34624=ORIENTED_EDGE('',*,*,#25253,.T.);
#34625=ORIENTED_EDGE('',*,*,#25245,.F.);
#34626=ORIENTED_EDGE('',*,*,#25242,.F.);
#34627=ORIENTED_EDGE('',*,*,#25247,.T.);
#34628=ORIENTED_EDGE('',*,*,#25239,.F.);
#34629=ORIENTED_EDGE('',*,*,#25236,.F.);
#34630=ORIENTED_EDGE('',*,*,#25241,.T.);
#34631=ORIENTED_EDGE('',*,*,#25233,.F.);
#34632=ORIENTED_EDGE('',*,*,#25228,.F.);
#34633=ORIENTED_EDGE('',*,*,#25235,.T.);
#34634=ORIENTED_EDGE('',*,*,#25225,.F.);
#34635=ORIENTED_EDGE('',*,*,#25222,.F.);
#34636=ORIENTED_EDGE('',*,*,#25227,.T.);
#34637=ORIENTED_EDGE('',*,*,#25219,.F.);
#34638=ORIENTED_EDGE('',*,*,#25216,.F.);
#34639=ORIENTED_EDGE('',*,*,#25221,.T.);
#34640=ORIENTED_EDGE('',*,*,#25213,.F.);
#34641=ORIENTED_EDGE('',*,*,#25210,.F.);
#34642=ORIENTED_EDGE('',*,*,#25215,.T.);
#34643=ORIENTED_EDGE('',*,*,#25207,.F.);
#34644=ORIENTED_EDGE('',*,*,#25204,.F.);
#34645=ORIENTED_EDGE('',*,*,#25209,.T.);
#34646=ORIENTED_EDGE('',*,*,#25201,.F.);
#34647=ORIENTED_EDGE('',*,*,#25198,.F.);
#34648=ORIENTED_EDGE('',*,*,#25203,.T.);
#34649=ORIENTED_EDGE('',*,*,#25195,.F.);
#34650=ORIENTED_EDGE('',*,*,#25192,.F.);
#34651=ORIENTED_EDGE('',*,*,#25197,.T.);
#34652=ORIENTED_EDGE('',*,*,#25189,.F.);
#34653=ORIENTED_EDGE('',*,*,#25186,.F.);
#34654=ORIENTED_EDGE('',*,*,#25191,.T.);
#34655=ORIENTED_EDGE('',*,*,#25183,.F.);
#34656=ORIENTED_EDGE('',*,*,#25180,.F.);
#34657=ORIENTED_EDGE('',*,*,#25185,.T.);
#34658=ORIENTED_EDGE('',*,*,#25177,.F.);
#34659=ORIENTED_EDGE('',*,*,#25172,.F.);
#34660=ORIENTED_EDGE('',*,*,#25179,.T.);
#34661=ORIENTED_EDGE('',*,*,#25169,.F.);
#34662=ORIENTED_EDGE('',*,*,#25166,.F.);
#34663=ORIENTED_EDGE('',*,*,#25171,.T.);
#34664=ORIENTED_EDGE('',*,*,#25163,.F.);
#34665=ORIENTED_EDGE('',*,*,#25160,.F.);
#34666=ORIENTED_EDGE('',*,*,#25165,.T.);
#34667=ORIENTED_EDGE('',*,*,#25157,.F.);
#34668=ORIENTED_EDGE('',*,*,#25154,.F.);
#34669=ORIENTED_EDGE('',*,*,#25159,.T.);
#34670=ORIENTED_EDGE('',*,*,#25151,.F.);
#34671=ORIENTED_EDGE('',*,*,#25148,.F.);
#34672=ORIENTED_EDGE('',*,*,#25153,.T.);
#34673=ORIENTED_EDGE('',*,*,#25145,.F.);
#34674=ORIENTED_EDGE('',*,*,#25142,.F.);
#34675=ORIENTED_EDGE('',*,*,#25147,.T.);
#34676=ORIENTED_EDGE('',*,*,#25139,.F.);
#34677=ORIENTED_EDGE('',*,*,#25136,.F.);
#34678=ORIENTED_EDGE('',*,*,#25141,.T.);
#34679=ORIENTED_EDGE('',*,*,#25133,.F.);
#34680=ORIENTED_EDGE('',*,*,#25130,.F.);
#34681=ORIENTED_EDGE('',*,*,#25135,.T.);
#34682=ORIENTED_EDGE('',*,*,#25127,.F.);
#34683=ORIENTED_EDGE('',*,*,#25122,.F.);
#34684=ORIENTED_EDGE('',*,*,#25129,.T.);
#34685=ORIENTED_EDGE('',*,*,#25119,.F.);
#34686=ORIENTED_EDGE('',*,*,#25116,.F.);
#34687=ORIENTED_EDGE('',*,*,#25121,.T.);
#34688=ORIENTED_EDGE('',*,*,#25113,.F.);
#34689=ORIENTED_EDGE('',*,*,#25110,.F.);
#34690=ORIENTED_EDGE('',*,*,#25115,.T.);
#34691=ORIENTED_EDGE('',*,*,#25107,.F.);
#34692=ORIENTED_EDGE('',*,*,#25104,.F.);
#34693=ORIENTED_EDGE('',*,*,#25109,.T.);
#34694=ORIENTED_EDGE('',*,*,#25101,.F.);
#34695=ORIENTED_EDGE('',*,*,#25098,.F.);
#34696=ORIENTED_EDGE('',*,*,#25103,.T.);
#34697=ORIENTED_EDGE('',*,*,#25095,.F.);
#34698=ORIENTED_EDGE('',*,*,#25092,.F.);
#34699=ORIENTED_EDGE('',*,*,#25097,.T.);
#34700=ORIENTED_EDGE('',*,*,#25089,.F.);
#34701=ORIENTED_EDGE('',*,*,#25086,.F.);
#34702=ORIENTED_EDGE('',*,*,#25091,.T.);
#34703=ORIENTED_EDGE('',*,*,#25083,.F.);
#34704=ORIENTED_EDGE('',*,*,#25080,.F.);
#34705=ORIENTED_EDGE('',*,*,#25085,.T.);
#34706=ORIENTED_EDGE('',*,*,#25077,.F.);
#34707=ORIENTED_EDGE('',*,*,#25074,.F.);
#34708=ORIENTED_EDGE('',*,*,#25079,.T.);
#34709=ORIENTED_EDGE('',*,*,#25071,.F.);
#34710=ORIENTED_EDGE('',*,*,#25066,.F.);
#34711=ORIENTED_EDGE('',*,*,#25073,.T.);
#34712=ORIENTED_EDGE('',*,*,#25063,.F.);
#34713=ORIENTED_EDGE('',*,*,#25060,.F.);
#34714=ORIENTED_EDGE('',*,*,#25065,.T.);
#34715=ORIENTED_EDGE('',*,*,#25057,.F.);
#34716=ORIENTED_EDGE('',*,*,#25054,.F.);
#34717=ORIENTED_EDGE('',*,*,#25059,.T.);
#34718=ORIENTED_EDGE('',*,*,#25051,.F.);
#34719=ORIENTED_EDGE('',*,*,#25048,.F.);
#34720=ORIENTED_EDGE('',*,*,#25053,.T.);
#34721=ORIENTED_EDGE('',*,*,#25045,.F.);
#34722=ORIENTED_EDGE('',*,*,#25042,.F.);
#34723=ORIENTED_EDGE('',*,*,#25047,.T.);
#34724=ORIENTED_EDGE('',*,*,#25039,.F.);
#34725=ORIENTED_EDGE('',*,*,#25036,.F.);
#34726=ORIENTED_EDGE('',*,*,#25041,.T.);
#34727=ORIENTED_EDGE('',*,*,#25033,.F.);
#34728=ORIENTED_EDGE('',*,*,#25030,.F.);
#34729=ORIENTED_EDGE('',*,*,#25035,.T.);
#34730=ORIENTED_EDGE('',*,*,#25027,.F.);
#34731=ORIENTED_EDGE('',*,*,#25024,.F.);
#34732=ORIENTED_EDGE('',*,*,#25029,.T.);
#34733=ORIENTED_EDGE('',*,*,#25021,.F.);
#34734=ORIENTED_EDGE('',*,*,#25018,.F.);
#34735=ORIENTED_EDGE('',*,*,#25023,.T.);
#34736=ORIENTED_EDGE('',*,*,#25015,.F.);
#34737=ORIENTED_EDGE('',*,*,#25011,.F.);
#34738=ORIENTED_EDGE('',*,*,#25014,.F.);
#34739=ORIENTED_EDGE('',*,*,#25017,.T.);
#34740=ORIENTED_EDGE('',*,*,#25008,.F.);
#34741=ORIENTED_EDGE('',*,*,#25004,.F.);
#34742=ORIENTED_EDGE('',*,*,#25007,.F.);
#34743=ORIENTED_EDGE('',*,*,#25010,.T.);
#34744=ORIENTED_EDGE('',*,*,#25001,.F.);
#34745=ORIENTED_EDGE('',*,*,#24997,.F.);
#34746=ORIENTED_EDGE('',*,*,#25000,.F.);
#34747=ORIENTED_EDGE('',*,*,#25003,.T.);
#34748=ORIENTED_EDGE('',*,*,#24994,.F.);
#34749=ORIENTED_EDGE('',*,*,#24990,.F.);
#34750=ORIENTED_EDGE('',*,*,#24993,.F.);
#34751=ORIENTED_EDGE('',*,*,#24996,.T.);
#34752=ORIENTED_EDGE('',*,*,#24987,.F.);
#34753=ORIENTED_EDGE('',*,*,#24983,.F.);
#34754=ORIENTED_EDGE('',*,*,#24986,.F.);
#34755=ORIENTED_EDGE('',*,*,#24989,.T.);
#34756=ORIENTED_EDGE('',*,*,#24980,.F.);
#34757=ORIENTED_EDGE('',*,*,#24976,.F.);
#34758=ORIENTED_EDGE('',*,*,#24979,.F.);
#34759=ORIENTED_EDGE('',*,*,#24982,.T.);
#34760=ORIENTED_EDGE('',*,*,#24973,.F.);
#34761=ORIENTED_EDGE('',*,*,#24969,.F.);
#34762=ORIENTED_EDGE('',*,*,#24972,.F.);
#34763=ORIENTED_EDGE('',*,*,#24975,.T.);
#34764=ORIENTED_EDGE('',*,*,#24966,.F.);
#34765=ORIENTED_EDGE('',*,*,#24962,.F.);
#34766=ORIENTED_EDGE('',*,*,#24965,.F.);
#34767=ORIENTED_EDGE('',*,*,#24968,.T.);
#34768=ORIENTED_EDGE('',*,*,#24959,.F.);
#34769=ORIENTED_EDGE('',*,*,#24955,.F.);
#34770=ORIENTED_EDGE('',*,*,#24958,.F.);
#34771=ORIENTED_EDGE('',*,*,#24961,.T.);
#34772=ORIENTED_EDGE('',*,*,#24952,.F.);
#34773=ORIENTED_EDGE('',*,*,#24948,.F.);
#34774=ORIENTED_EDGE('',*,*,#24951,.F.);
#34775=ORIENTED_EDGE('',*,*,#24954,.T.);
#34776=ORIENTED_EDGE('',*,*,#24945,.F.);
#34777=ORIENTED_EDGE('',*,*,#24941,.F.);
#34778=ORIENTED_EDGE('',*,*,#24944,.F.);
#34779=ORIENTED_EDGE('',*,*,#24947,.T.);
#34780=ORIENTED_EDGE('',*,*,#24938,.F.);
#34781=ORIENTED_EDGE('',*,*,#24934,.F.);
#34782=ORIENTED_EDGE('',*,*,#24937,.F.);
#34783=ORIENTED_EDGE('',*,*,#24940,.T.);
#34784=ORIENTED_EDGE('',*,*,#24931,.F.);
#34785=ORIENTED_EDGE('',*,*,#24927,.F.);
#34786=ORIENTED_EDGE('',*,*,#24930,.F.);
#34787=ORIENTED_EDGE('',*,*,#24933,.T.);
#34788=ORIENTED_EDGE('',*,*,#24924,.F.);
#34789=ORIENTED_EDGE('',*,*,#24920,.F.);
#34790=ORIENTED_EDGE('',*,*,#24923,.F.);
#34791=ORIENTED_EDGE('',*,*,#24926,.T.);
#34792=ORIENTED_EDGE('',*,*,#24917,.F.);
#34793=ORIENTED_EDGE('',*,*,#24914,.F.);
#34794=ORIENTED_EDGE('',*,*,#24919,.T.);
#34795=ORIENTED_EDGE('',*,*,#24911,.F.);
#34796=ORIENTED_EDGE('',*,*,#24907,.F.);
#34797=ORIENTED_EDGE('',*,*,#24910,.F.);
#34798=ORIENTED_EDGE('',*,*,#24913,.T.);
#34799=ORIENTED_EDGE('',*,*,#24904,.F.);
#34800=ORIENTED_EDGE('',*,*,#24900,.F.);
#34801=ORIENTED_EDGE('',*,*,#24903,.F.);
#34802=ORIENTED_EDGE('',*,*,#24906,.T.);
#34803=ORIENTED_EDGE('',*,*,#24897,.F.);
#34804=ORIENTED_EDGE('',*,*,#24894,.F.);
#34805=ORIENTED_EDGE('',*,*,#24899,.T.);
#34806=ORIENTED_EDGE('',*,*,#24891,.F.);
#34807=ORIENTED_EDGE('',*,*,#24887,.F.);
#34808=ORIENTED_EDGE('',*,*,#24890,.F.);
#34809=ORIENTED_EDGE('',*,*,#24893,.T.);
#34810=ORIENTED_EDGE('',*,*,#24884,.F.);
#34811=ORIENTED_EDGE('',*,*,#24880,.F.);
#34812=ORIENTED_EDGE('',*,*,#24883,.F.);
#34813=ORIENTED_EDGE('',*,*,#24886,.T.);
#34814=ORIENTED_EDGE('',*,*,#24877,.F.);
#34815=ORIENTED_EDGE('',*,*,#24874,.F.);
#34816=ORIENTED_EDGE('',*,*,#24879,.T.);
#34817=ORIENTED_EDGE('',*,*,#24871,.F.);
#34818=ORIENTED_EDGE('',*,*,#24868,.F.);
#34819=ORIENTED_EDGE('',*,*,#24873,.T.);
#34820=ORIENTED_EDGE('',*,*,#24865,.F.);
#34821=ORIENTED_EDGE('',*,*,#24861,.F.);
#34822=ORIENTED_EDGE('',*,*,#24864,.F.);
#34823=ORIENTED_EDGE('',*,*,#24867,.T.);
#34824=ORIENTED_EDGE('',*,*,#24858,.F.);
#34825=ORIENTED_EDGE('',*,*,#24854,.F.);
#34826=ORIENTED_EDGE('',*,*,#24857,.F.);
#34827=ORIENTED_EDGE('',*,*,#24860,.T.);
#34828=ORIENTED_EDGE('',*,*,#24851,.F.);
#34829=ORIENTED_EDGE('',*,*,#24848,.F.);
#34830=ORIENTED_EDGE('',*,*,#24853,.T.);
#34831=ORIENTED_EDGE('',*,*,#24845,.F.);
#34832=ORIENTED_EDGE('',*,*,#24842,.F.);
#34833=ORIENTED_EDGE('',*,*,#24847,.T.);
#34834=ORIENTED_EDGE('',*,*,#24839,.F.);
#34835=ORIENTED_EDGE('',*,*,#24835,.F.);
#34836=ORIENTED_EDGE('',*,*,#24838,.F.);
#34837=ORIENTED_EDGE('',*,*,#24841,.T.);
#34838=ORIENTED_EDGE('',*,*,#24832,.F.);
#34839=ORIENTED_EDGE('',*,*,#24828,.F.);
#34840=ORIENTED_EDGE('',*,*,#24831,.F.);
#34841=ORIENTED_EDGE('',*,*,#24834,.T.);
#34842=ORIENTED_EDGE('',*,*,#24825,.F.);
#34843=ORIENTED_EDGE('',*,*,#24821,.F.);
#34844=ORIENTED_EDGE('',*,*,#24824,.F.);
#34845=ORIENTED_EDGE('',*,*,#24827,.T.);
#34846=ORIENTED_EDGE('',*,*,#24818,.F.);
#34847=ORIENTED_EDGE('',*,*,#24814,.F.);
#34848=ORIENTED_EDGE('',*,*,#24817,.F.);
#34849=ORIENTED_EDGE('',*,*,#24820,.T.);
#34850=ORIENTED_EDGE('',*,*,#24811,.F.);
#34851=ORIENTED_EDGE('',*,*,#24807,.F.);
#34852=ORIENTED_EDGE('',*,*,#24810,.F.);
#34853=ORIENTED_EDGE('',*,*,#24813,.T.);
#34854=ORIENTED_EDGE('',*,*,#24804,.F.);
#34855=ORIENTED_EDGE('',*,*,#24800,.F.);
#34856=ORIENTED_EDGE('',*,*,#24803,.F.);
#34857=ORIENTED_EDGE('',*,*,#24806,.T.);
#34858=ORIENTED_EDGE('',*,*,#24797,.F.);
#34859=ORIENTED_EDGE('',*,*,#24793,.F.);
#34860=ORIENTED_EDGE('',*,*,#24796,.F.);
#34861=ORIENTED_EDGE('',*,*,#24799,.T.);
#34862=ORIENTED_EDGE('',*,*,#24790,.F.);
#34863=ORIENTED_EDGE('',*,*,#24786,.F.);
#34864=ORIENTED_EDGE('',*,*,#24789,.F.);
#34865=ORIENTED_EDGE('',*,*,#24792,.T.);
#34866=ORIENTED_EDGE('',*,*,#24783,.F.);
#34867=ORIENTED_EDGE('',*,*,#24779,.F.);
#34868=ORIENTED_EDGE('',*,*,#24782,.F.);
#34869=ORIENTED_EDGE('',*,*,#24785,.T.);
#34870=ORIENTED_EDGE('',*,*,#24776,.F.);
#34871=ORIENTED_EDGE('',*,*,#24772,.F.);
#34872=ORIENTED_EDGE('',*,*,#24775,.F.);
#34873=ORIENTED_EDGE('',*,*,#24778,.T.);
#34874=ORIENTED_EDGE('',*,*,#24769,.F.);
#34875=ORIENTED_EDGE('',*,*,#24765,.F.);
#34876=ORIENTED_EDGE('',*,*,#24768,.F.);
#34877=ORIENTED_EDGE('',*,*,#24771,.T.);
#34878=ORIENTED_EDGE('',*,*,#24762,.F.);
#34879=ORIENTED_EDGE('',*,*,#24758,.F.);
#34880=ORIENTED_EDGE('',*,*,#24761,.F.);
#34881=ORIENTED_EDGE('',*,*,#24764,.T.);
#34882=ORIENTED_EDGE('',*,*,#24755,.F.);
#34883=ORIENTED_EDGE('',*,*,#24751,.F.);
#34884=ORIENTED_EDGE('',*,*,#24754,.F.);
#34885=ORIENTED_EDGE('',*,*,#24757,.T.);
#34886=ORIENTED_EDGE('',*,*,#24748,.F.);
#34887=ORIENTED_EDGE('',*,*,#24744,.F.);
#34888=ORIENTED_EDGE('',*,*,#24747,.F.);
#34889=ORIENTED_EDGE('',*,*,#24750,.T.);
#34890=ORIENTED_EDGE('',*,*,#24741,.F.);
#34891=ORIENTED_EDGE('',*,*,#24737,.F.);
#34892=ORIENTED_EDGE('',*,*,#24740,.F.);
#34893=ORIENTED_EDGE('',*,*,#24743,.T.);
#34894=ORIENTED_EDGE('',*,*,#24734,.F.);
#34895=ORIENTED_EDGE('',*,*,#24730,.F.);
#34896=ORIENTED_EDGE('',*,*,#24733,.F.);
#34897=ORIENTED_EDGE('',*,*,#24736,.T.);
#34898=ORIENTED_EDGE('',*,*,#24727,.F.);
#34899=ORIENTED_EDGE('',*,*,#24723,.F.);
#34900=ORIENTED_EDGE('',*,*,#24726,.F.);
#34901=ORIENTED_EDGE('',*,*,#24729,.T.);
#34902=ORIENTED_EDGE('',*,*,#24720,.F.);
#34903=ORIENTED_EDGE('',*,*,#24716,.F.);
#34904=ORIENTED_EDGE('',*,*,#24719,.F.);
#34905=ORIENTED_EDGE('',*,*,#24722,.T.);
#34906=ORIENTED_EDGE('',*,*,#24713,.F.);
#34907=ORIENTED_EDGE('',*,*,#24709,.F.);
#34908=ORIENTED_EDGE('',*,*,#24712,.F.);
#34909=ORIENTED_EDGE('',*,*,#24715,.T.);
#34910=ORIENTED_EDGE('',*,*,#24706,.F.);
#34911=ORIENTED_EDGE('',*,*,#24702,.F.);
#34912=ORIENTED_EDGE('',*,*,#24705,.F.);
#34913=ORIENTED_EDGE('',*,*,#24708,.T.);
#34914=ORIENTED_EDGE('',*,*,#24699,.F.);
#34915=ORIENTED_EDGE('',*,*,#24695,.F.);
#34916=ORIENTED_EDGE('',*,*,#24698,.F.);
#34917=ORIENTED_EDGE('',*,*,#24701,.T.);
#34918=ORIENTED_EDGE('',*,*,#24692,.F.);
#34919=ORIENTED_EDGE('',*,*,#24688,.F.);
#34920=ORIENTED_EDGE('',*,*,#24691,.F.);
#34921=ORIENTED_EDGE('',*,*,#24694,.T.);
#34922=ORIENTED_EDGE('',*,*,#24685,.F.);
#34923=ORIENTED_EDGE('',*,*,#24681,.F.);
#34924=ORIENTED_EDGE('',*,*,#24684,.F.);
#34925=ORIENTED_EDGE('',*,*,#24687,.T.);
#34926=ORIENTED_EDGE('',*,*,#24678,.F.);
#34927=ORIENTED_EDGE('',*,*,#24674,.F.);
#34928=ORIENTED_EDGE('',*,*,#24677,.F.);
#34929=ORIENTED_EDGE('',*,*,#24680,.T.);
#34930=ORIENTED_EDGE('',*,*,#24671,.F.);
#34931=ORIENTED_EDGE('',*,*,#24667,.F.);
#34932=ORIENTED_EDGE('',*,*,#24670,.F.);
#34933=ORIENTED_EDGE('',*,*,#24673,.T.);
#34934=ORIENTED_EDGE('',*,*,#24664,.F.);
#34935=ORIENTED_EDGE('',*,*,#24660,.F.);
#34936=ORIENTED_EDGE('',*,*,#24663,.F.);
#34937=ORIENTED_EDGE('',*,*,#24666,.T.);
#34938=ORIENTED_EDGE('',*,*,#24657,.F.);
#34939=ORIENTED_EDGE('',*,*,#24653,.F.);
#34940=ORIENTED_EDGE('',*,*,#24656,.F.);
#34941=ORIENTED_EDGE('',*,*,#24659,.T.);
#34942=ORIENTED_EDGE('',*,*,#24650,.F.);
#34943=ORIENTED_EDGE('',*,*,#24646,.F.);
#34944=ORIENTED_EDGE('',*,*,#24649,.F.);
#34945=ORIENTED_EDGE('',*,*,#24652,.T.);
#34946=ORIENTED_EDGE('',*,*,#24643,.F.);
#34947=ORIENTED_EDGE('',*,*,#24639,.F.);
#34948=ORIENTED_EDGE('',*,*,#24642,.F.);
#34949=ORIENTED_EDGE('',*,*,#24645,.T.);
#34950=ORIENTED_EDGE('',*,*,#24636,.F.);
#34951=ORIENTED_EDGE('',*,*,#24632,.F.);
#34952=ORIENTED_EDGE('',*,*,#24635,.F.);
#34953=ORIENTED_EDGE('',*,*,#24638,.T.);
#34954=ORIENTED_EDGE('',*,*,#24629,.F.);
#34955=ORIENTED_EDGE('',*,*,#24625,.F.);
#34956=ORIENTED_EDGE('',*,*,#24628,.F.);
#34957=ORIENTED_EDGE('',*,*,#24631,.T.);
#34958=ORIENTED_EDGE('',*,*,#24622,.F.);
#34959=ORIENTED_EDGE('',*,*,#24618,.F.);
#34960=ORIENTED_EDGE('',*,*,#24621,.F.);
#34961=ORIENTED_EDGE('',*,*,#24624,.T.);
#34962=ORIENTED_EDGE('',*,*,#24615,.F.);
#34963=ORIENTED_EDGE('',*,*,#24611,.F.);
#34964=ORIENTED_EDGE('',*,*,#24614,.F.);
#34965=ORIENTED_EDGE('',*,*,#24617,.T.);
#34966=ORIENTED_EDGE('',*,*,#24608,.F.);
#34967=ORIENTED_EDGE('',*,*,#24604,.F.);
#34968=ORIENTED_EDGE('',*,*,#24607,.F.);
#34969=ORIENTED_EDGE('',*,*,#24610,.T.);
#34970=ORIENTED_EDGE('',*,*,#24601,.F.);
#34971=ORIENTED_EDGE('',*,*,#24597,.F.);
#34972=ORIENTED_EDGE('',*,*,#24600,.F.);
#34973=ORIENTED_EDGE('',*,*,#24603,.T.);
#34974=ORIENTED_EDGE('',*,*,#24594,.F.);
#34975=ORIENTED_EDGE('',*,*,#24590,.F.);
#34976=ORIENTED_EDGE('',*,*,#24593,.F.);
#34977=ORIENTED_EDGE('',*,*,#24596,.T.);
#34978=ORIENTED_EDGE('',*,*,#24587,.F.);
#34979=ORIENTED_EDGE('',*,*,#24583,.F.);
#34980=ORIENTED_EDGE('',*,*,#24586,.F.);
#34981=ORIENTED_EDGE('',*,*,#24589,.T.);
#34982=ORIENTED_EDGE('',*,*,#24580,.F.);
#34983=ORIENTED_EDGE('',*,*,#24576,.F.);
#34984=ORIENTED_EDGE('',*,*,#24579,.F.);
#34985=ORIENTED_EDGE('',*,*,#24582,.T.);
#34986=ORIENTED_EDGE('',*,*,#24573,.F.);
#34987=ORIENTED_EDGE('',*,*,#24569,.F.);
#34988=ORIENTED_EDGE('',*,*,#24572,.F.);
#34989=ORIENTED_EDGE('',*,*,#24575,.T.);
#34990=ORIENTED_EDGE('',*,*,#24566,.F.);
#34991=ORIENTED_EDGE('',*,*,#24565,.T.);
#34992=ORIENTED_EDGE('',*,*,#24563,.F.);
#34993=ORIENTED_EDGE('',*,*,#24560,.F.);
#34994=ORIENTED_EDGE('',*,*,#24559,.T.);
#34995=ORIENTED_EDGE('',*,*,#24557,.F.);
#34996=ORIENTED_EDGE('',*,*,#24554,.F.);
#34997=ORIENTED_EDGE('',*,*,#24553,.T.);
#34998=ORIENTED_EDGE('',*,*,#24551,.F.);
#34999=ORIENTED_EDGE('',*,*,#24548,.F.);
#35000=ORIENTED_EDGE('',*,*,#24547,.T.);
#35001=ORIENTED_EDGE('',*,*,#24545,.F.);
#35002=ORIENTED_EDGE('',*,*,#24542,.F.);
#35003=ORIENTED_EDGE('',*,*,#24541,.T.);
#35004=ORIENTED_EDGE('',*,*,#24539,.F.);
#35005=ORIENTED_EDGE('',*,*,#24536,.F.);
#35006=ORIENTED_EDGE('',*,*,#24535,.T.);
#35007=ORIENTED_EDGE('',*,*,#24533,.F.);
#41946=TOROIDAL_SURFACE('',#47410,62.7000000000001,0.3);
#41947=TOROIDAL_SURFACE('',#47418,10.9885950377664,1.);
#41948=TOROIDAL_SURFACE('',#47421,9.19091713639506,0.2);
#41949=TOROIDAL_SURFACE('',#47425,63.,2.);
#41950=TOROIDAL_SURFACE('',#47428,22.4734498738832,0.5);
#41951=TOROIDAL_SURFACE('',#47437,63.2999999999999,0.3);
#41952=TOROIDAL_SURFACE('',#47442,8.79091713639511,0.2);
#41953=TOROIDAL_SURFACE('',#47453,7.3031389659941,1.);
#41954=TOROIDAL_SURFACE('',#47473,5.888925403621,1.);
#41955=TOROIDAL_SURFACE('',#47480,5.888925403621,1.);
#41956=TOROIDAL_SURFACE('',#47481,7.3031389659941,1.);
#41957=TOROIDAL_SURFACE('',#47487,7.3031389659941,1.);
#41958=TOROIDAL_SURFACE('',#47503,22.4734498738832,0.5);
#41959=TOROIDAL_SURFACE('',#47520,63.,2.);
#42054=ADVANCED_FACE('',(#9474),#2952,.F.);
#42055=ADVANCED_FACE('',(#9475),#2953,.T.);
#42056=ADVANCED_FACE('',(#9476),#7863,.F.);
#42057=ADVANCED_FACE('',(#9477),#2954,.T.);
#42058=ADVANCED_FACE('',(#9478),#2955,.T.);
#42059=ADVANCED_FACE('',(#9479),#7864,.T.);
#42060=ADVANCED_FACE('',(#9480),#2956,.T.);
#42061=ADVANCED_FACE('',(#9481),#2957,.T.);
#42062=ADVANCED_FACE('',(#9482),#2958,.T.);
#42063=ADVANCED_FACE('',(#9483),#7865,.F.);
#42064=ADVANCED_FACE('',(#9484),#7866,.F.);
#42065=ADVANCED_FACE('',(#9485),#7867,.T.);
#42066=ADVANCED_FACE('',(#9486),#7868,.F.);
#42067=ADVANCED_FACE('',(#9487),#7869,.T.);
#42068=ADVANCED_FACE('',(#9488),#7870,.F.);
#42069=ADVANCED_FACE('',(#9489),#7871,.T.);
#42070=ADVANCED_FACE('',(#9490),#7872,.F.);
#42071=ADVANCED_FACE('',(#9491),#7873,.T.);
#42072=ADVANCED_FACE('',(#9492),#7874,.F.);
#42073=ADVANCED_FACE('',(#9493),#7875,.T.);
#42074=ADVANCED_FACE('',(#9494),#7876,.F.);
#42075=ADVANCED_FACE('',(#9495),#7877,.T.);
#42076=ADVANCED_FACE('',(#9496),#7878,.T.);
#42077=ADVANCED_FACE('',(#9497),#7879,.F.);
#42078=ADVANCED_FACE('',(#9498),#7880,.T.);
#42079=ADVANCED_FACE('',(#9499),#7881,.F.);
#42080=ADVANCED_FACE('',(#9500),#7882,.T.);
#42081=ADVANCED_FACE('',(#9501),#7883,.F.);
#42082=ADVANCED_FACE('',(#9502),#7884,.T.);
#42083=ADVANCED_FACE('',(#9503),#7885,.F.);
#42084=ADVANCED_FACE('',(#9504),#7886,.T.);
#42085=ADVANCED_FACE('',(#9505),#7887,.F.);
#42086=ADVANCED_FACE('',(#9506),#7888,.T.);
#42087=ADVANCED_FACE('',(#9507),#7889,.F.);
#42088=ADVANCED_FACE('',(#9508),#7890,.T.);
#42089=ADVANCED_FACE('',(#9509),#7891,.F.);
#42090=ADVANCED_FACE('',(#9510),#7892,.T.);
#42091=ADVANCED_FACE('',(#9511),#7893,.F.);
#42092=ADVANCED_FACE('',(#9512),#7894,.T.);
#42093=ADVANCED_FACE('',(#9513),#7895,.F.);
#42094=ADVANCED_FACE('',(#9514),#7896,.T.);
#42095=ADVANCED_FACE('',(#9515),#7897,.F.);
#42096=ADVANCED_FACE('',(#9516),#7898,.T.);
#42097=ADVANCED_FACE('',(#9517),#7899,.F.);
#42098=ADVANCED_FACE('',(#9518),#7900,.T.);
#42099=ADVANCED_FACE('',(#9519),#7901,.F.);
#42100=ADVANCED_FACE('',(#9520),#7902,.T.);
#42101=ADVANCED_FACE('',(#9521),#7903,.F.);
#42102=ADVANCED_FACE('',(#9522),#7904,.T.);
#42103=ADVANCED_FACE('',(#9523),#7905,.F.);
#42104=ADVANCED_FACE('',(#9524),#7906,.T.);
#42105=ADVANCED_FACE('',(#9525),#7907,.F.);
#42106=ADVANCED_FACE('',(#9526),#7908,.T.);
#42107=ADVANCED_FACE('',(#9527),#7909,.F.);
#42108=ADVANCED_FACE('',(#9528),#7910,.T.);
#42109=ADVANCED_FACE('',(#9529),#7911,.F.);
#42110=ADVANCED_FACE('',(#9530),#7912,.T.);
#42111=ADVANCED_FACE('',(#9531),#7913,.F.);
#42112=ADVANCED_FACE('',(#9532),#7914,.T.);
#42113=ADVANCED_FACE('',(#9533),#7915,.F.);
#42114=ADVANCED_FACE('',(#9534),#7916,.T.);
#42115=ADVANCED_FACE('',(#9535),#7917,.F.);
#42116=ADVANCED_FACE('',(#9536),#7918,.T.);
#42117=ADVANCED_FACE('',(#9537),#7919,.F.);
#42118=ADVANCED_FACE('',(#9538),#7920,.T.);
#42119=ADVANCED_FACE('',(#9539),#7921,.F.);
#42120=ADVANCED_FACE('',(#9540),#7922,.T.);
#42121=ADVANCED_FACE('',(#9541),#7923,.F.);
#42122=ADVANCED_FACE('',(#9542),#7924,.T.);
#42123=ADVANCED_FACE('',(#9543),#7925,.F.);
#42124=ADVANCED_FACE('',(#9544),#7926,.T.);
#42125=ADVANCED_FACE('',(#9545),#7927,.F.);
#42126=ADVANCED_FACE('',(#9546),#7928,.T.);
#42127=ADVANCED_FACE('',(#9547),#7929,.F.);
#42128=ADVANCED_FACE('',(#9548),#7930,.T.);
#42129=ADVANCED_FACE('',(#9549),#7931,.F.);
#42130=ADVANCED_FACE('',(#9550),#7932,.T.);
#42131=ADVANCED_FACE('',(#9551),#7933,.F.);
#42132=ADVANCED_FACE('',(#9552),#7934,.T.);
#42133=ADVANCED_FACE('',(#9553),#7935,.F.);
#42134=ADVANCED_FACE('',(#9554),#7936,.T.);
#42135=ADVANCED_FACE('',(#9555),#7937,.F.);
#42136=ADVANCED_FACE('',(#9556),#7938,.T.);
#42137=ADVANCED_FACE('',(#9557),#7939,.F.);
#42138=ADVANCED_FACE('',(#9558),#7940,.T.);
#42139=ADVANCED_FACE('',(#9559),#7941,.F.);
#42140=ADVANCED_FACE('',(#9560),#7942,.T.);
#42141=ADVANCED_FACE('',(#9561),#7943,.F.);
#42142=ADVANCED_FACE('',(#9562),#7944,.T.);
#42143=ADVANCED_FACE('',(#9563),#7945,.F.);
#42144=ADVANCED_FACE('',(#9564),#7946,.T.);
#42145=ADVANCED_FACE('',(#9565),#7947,.F.);
#42146=ADVANCED_FACE('',(#9566),#7948,.T.);
#42147=ADVANCED_FACE('',(#9567),#7949,.F.);
#42148=ADVANCED_FACE('',(#9568),#7950,.T.);
#42149=ADVANCED_FACE('',(#9569),#7951,.F.);
#42150=ADVANCED_FACE('',(#9570),#7952,.T.);
#42151=ADVANCED_FACE('',(#9571),#7953,.F.);
#42152=ADVANCED_FACE('',(#9572),#7954,.T.);
#42153=ADVANCED_FACE('',(#9573),#7955,.F.);
#42154=ADVANCED_FACE('',(#9574),#7956,.T.);
#42155=ADVANCED_FACE('',(#9575),#7957,.F.);
#42156=ADVANCED_FACE('',(#9576),#7958,.T.);
#42157=ADVANCED_FACE('',(#9577),#7959,.F.);
#42158=ADVANCED_FACE('',(#9578),#7960,.T.);
#42159=ADVANCED_FACE('',(#9579),#7961,.F.);
#42160=ADVANCED_FACE('',(#9580),#7962,.T.);
#42161=ADVANCED_FACE('',(#9581),#7963,.F.);
#42162=ADVANCED_FACE('',(#9582),#7964,.T.);
#42163=ADVANCED_FACE('',(#9583),#7965,.F.);
#42164=ADVANCED_FACE('',(#9584),#7966,.T.);
#42165=ADVANCED_FACE('',(#9585),#7967,.F.);
#42166=ADVANCED_FACE('',(#9586),#7968,.T.);
#42167=ADVANCED_FACE('',(#9587),#7969,.F.);
#42168=ADVANCED_FACE('',(#9588),#7970,.T.);
#42169=ADVANCED_FACE('',(#9589),#7971,.F.);
#42170=ADVANCED_FACE('',(#9590),#7972,.T.);
#42171=ADVANCED_FACE('',(#9591),#7973,.F.);
#42172=ADVANCED_FACE('',(#9592),#7974,.T.);
#42173=ADVANCED_FACE('',(#9593),#7975,.F.);
#42174=ADVANCED_FACE('',(#9594),#7976,.T.);
#42175=ADVANCED_FACE('',(#9595),#7977,.F.);
#42176=ADVANCED_FACE('',(#9596),#7978,.T.);
#42177=ADVANCED_FACE('',(#9597),#7979,.F.);
#42178=ADVANCED_FACE('',(#9598),#7980,.T.);
#42179=ADVANCED_FACE('',(#9599),#7981,.F.);
#42180=ADVANCED_FACE('',(#9600),#7982,.T.);
#42181=ADVANCED_FACE('',(#9601),#7983,.F.);
#42182=ADVANCED_FACE('',(#9602),#7984,.T.);
#42183=ADVANCED_FACE('',(#9603),#7985,.F.);
#42184=ADVANCED_FACE('',(#9604),#7986,.T.);
#42185=ADVANCED_FACE('',(#9605),#7987,.F.);
#42186=ADVANCED_FACE('',(#9606),#7988,.T.);
#42187=ADVANCED_FACE('',(#9607),#7989,.F.);
#42188=ADVANCED_FACE('',(#9608),#7990,.T.);
#42189=ADVANCED_FACE('',(#9609),#7991,.F.);
#42190=ADVANCED_FACE('',(#9610),#7992,.T.);
#42191=ADVANCED_FACE('',(#9611),#7993,.F.);
#42192=ADVANCED_FACE('',(#9612),#7994,.T.);
#42193=ADVANCED_FACE('',(#9613),#7995,.F.);
#42194=ADVANCED_FACE('',(#9614),#7996,.T.);
#42195=ADVANCED_FACE('',(#9615),#7997,.F.);
#42196=ADVANCED_FACE('',(#9616),#7998,.T.);
#42197=ADVANCED_FACE('',(#9617),#7999,.F.);
#42198=ADVANCED_FACE('',(#9618),#8000,.T.);
#42199=ADVANCED_FACE('',(#9619),#8001,.F.);
#42200=ADVANCED_FACE('',(#9620),#8002,.T.);
#42201=ADVANCED_FACE('',(#9621),#8003,.F.);
#42202=ADVANCED_FACE('',(#9622),#8004,.T.);
#42203=ADVANCED_FACE('',(#9623),#8005,.F.);
#42204=ADVANCED_FACE('',(#9624),#8006,.T.);
#42205=ADVANCED_FACE('',(#9625),#8007,.F.);
#42206=ADVANCED_FACE('',(#9626),#8008,.T.);
#42207=ADVANCED_FACE('',(#9627),#8009,.F.);
#42208=ADVANCED_FACE('',(#9628),#8010,.T.);
#42209=ADVANCED_FACE('',(#9629),#8011,.F.);
#42210=ADVANCED_FACE('',(#9630),#8012,.T.);
#42211=ADVANCED_FACE('',(#9631),#8013,.F.);
#42212=ADVANCED_FACE('',(#9632),#8014,.T.);
#42213=ADVANCED_FACE('',(#9633),#8015,.F.);
#42214=ADVANCED_FACE('',(#9634),#8016,.T.);
#42215=ADVANCED_FACE('',(#9635),#8017,.F.);
#42216=ADVANCED_FACE('',(#9636),#8018,.T.);
#42217=ADVANCED_FACE('',(#9637),#8019,.F.);
#42218=ADVANCED_FACE('',(#9638),#8020,.T.);
#42219=ADVANCED_FACE('',(#9639),#8021,.F.);
#42220=ADVANCED_FACE('',(#9640),#8022,.T.);
#42221=ADVANCED_FACE('',(#9641),#8023,.F.);
#42222=ADVANCED_FACE('',(#9642),#8024,.T.);
#42223=ADVANCED_FACE('',(#9643),#8025,.F.);
#42224=ADVANCED_FACE('',(#9644),#8026,.T.);
#42225=ADVANCED_FACE('',(#9645),#8027,.F.);
#42226=ADVANCED_FACE('',(#9646),#8028,.T.);
#42227=ADVANCED_FACE('',(#9647),#8029,.F.);
#42228=ADVANCED_FACE('',(#9648),#8030,.T.);
#42229=ADVANCED_FACE('',(#9649),#8031,.F.);
#42230=ADVANCED_FACE('',(#9650),#8032,.T.);
#42231=ADVANCED_FACE('',(#9651),#8033,.F.);
#42232=ADVANCED_FACE('',(#9652),#8034,.T.);
#42233=ADVANCED_FACE('',(#9653),#8035,.F.);
#42234=ADVANCED_FACE('',(#9654),#8036,.T.);
#42235=ADVANCED_FACE('',(#9655),#8037,.F.);
#42236=ADVANCED_FACE('',(#9656),#8038,.T.);
#42237=ADVANCED_FACE('',(#9657),#8039,.F.);
#42238=ADVANCED_FACE('',(#9658),#8040,.T.);
#42239=ADVANCED_FACE('',(#9659),#8041,.F.);
#42240=ADVANCED_FACE('',(#9660),#8042,.T.);
#42241=ADVANCED_FACE('',(#9661),#8043,.F.);
#42242=ADVANCED_FACE('',(#9662),#8044,.T.);
#42243=ADVANCED_FACE('',(#9663),#8045,.F.);
#42244=ADVANCED_FACE('',(#9664),#8046,.T.);
#42245=ADVANCED_FACE('',(#9665),#8047,.F.);
#42246=ADVANCED_FACE('',(#9666),#8048,.T.);
#42247=ADVANCED_FACE('',(#9667),#8049,.F.);
#42248=ADVANCED_FACE('',(#9668),#8050,.T.);
#42249=ADVANCED_FACE('',(#9669),#8051,.F.);
#42250=ADVANCED_FACE('',(#9670),#8052,.T.);
#42251=ADVANCED_FACE('',(#9671),#8053,.F.);
#42252=ADVANCED_FACE('',(#9672),#8054,.T.);
#42253=ADVANCED_FACE('',(#9673),#8055,.F.);
#42254=ADVANCED_FACE('',(#9674),#8056,.T.);
#42255=ADVANCED_FACE('',(#9675),#8057,.F.);
#42256=ADVANCED_FACE('',(#9676),#8058,.T.);
#42257=ADVANCED_FACE('',(#9677),#8059,.F.);
#42258=ADVANCED_FACE('',(#9678),#8060,.T.);
#42259=ADVANCED_FACE('',(#9679),#8061,.F.);
#42260=ADVANCED_FACE('',(#9680),#8062,.T.);
#42261=ADVANCED_FACE('',(#9681),#8063,.F.);
#42262=ADVANCED_FACE('',(#9682),#8064,.T.);
#42263=ADVANCED_FACE('',(#9683),#8065,.F.);
#42264=ADVANCED_FACE('',(#9684),#8066,.T.);
#42265=ADVANCED_FACE('',(#9685),#8067,.F.);
#42266=ADVANCED_FACE('',(#9686),#8068,.T.);
#42267=ADVANCED_FACE('',(#9687),#8069,.F.);
#42268=ADVANCED_FACE('',(#9688),#8070,.T.);
#42269=ADVANCED_FACE('',(#9689),#8071,.F.);
#42270=ADVANCED_FACE('',(#9690),#8072,.T.);
#42271=ADVANCED_FACE('',(#9691),#8073,.F.);
#42272=ADVANCED_FACE('',(#9692),#8074,.T.);
#42273=ADVANCED_FACE('',(#9693),#8075,.F.);
#42274=ADVANCED_FACE('',(#9694),#8076,.T.);
#42275=ADVANCED_FACE('',(#9695),#8077,.F.);
#42276=ADVANCED_FACE('',(#9696),#8078,.T.);
#42277=ADVANCED_FACE('',(#9697),#8079,.F.);
#42278=ADVANCED_FACE('',(#9698),#8080,.T.);
#42279=ADVANCED_FACE('',(#9699),#8081,.F.);
#42280=ADVANCED_FACE('',(#9700),#8082,.T.);
#42281=ADVANCED_FACE('',(#9701),#8083,.F.);
#42282=ADVANCED_FACE('',(#9702),#8084,.T.);
#42283=ADVANCED_FACE('',(#9703),#8085,.F.);
#42284=ADVANCED_FACE('',(#9704),#8086,.T.);
#42285=ADVANCED_FACE('',(#9705),#8087,.F.);
#42286=ADVANCED_FACE('',(#9706),#8088,.T.);
#42287=ADVANCED_FACE('',(#9707),#8089,.F.);
#42288=ADVANCED_FACE('',(#9708),#8090,.T.);
#42289=ADVANCED_FACE('',(#9709),#8091,.F.);
#42290=ADVANCED_FACE('',(#9710),#8092,.T.);
#42291=ADVANCED_FACE('',(#9711),#8093,.F.);
#42292=ADVANCED_FACE('',(#9712),#8094,.T.);
#42293=ADVANCED_FACE('',(#9713),#8095,.F.);
#42294=ADVANCED_FACE('',(#9714),#8096,.T.);
#42295=ADVANCED_FACE('',(#9715),#8097,.F.);
#42296=ADVANCED_FACE('',(#9716),#8098,.T.);
#42297=ADVANCED_FACE('',(#9717),#8099,.F.);
#42298=ADVANCED_FACE('',(#9718),#8100,.T.);
#42299=ADVANCED_FACE('',(#9719),#8101,.F.);
#42300=ADVANCED_FACE('',(#9720),#8102,.T.);
#42301=ADVANCED_FACE('',(#9721),#8103,.F.);
#42302=ADVANCED_FACE('',(#9722),#8104,.T.);
#42303=ADVANCED_FACE('',(#9723),#8105,.F.);
#42304=ADVANCED_FACE('',(#9724),#8106,.T.);
#42305=ADVANCED_FACE('',(#9725),#8107,.F.);
#42306=ADVANCED_FACE('',(#9726),#8108,.T.);
#42307=ADVANCED_FACE('',(#9727),#8109,.F.);
#42308=ADVANCED_FACE('',(#9728),#8110,.T.);
#42309=ADVANCED_FACE('',(#9729),#8111,.F.);
#42310=ADVANCED_FACE('',(#9730),#8112,.T.);
#42311=ADVANCED_FACE('',(#9731),#8113,.F.);
#42312=ADVANCED_FACE('',(#9732),#8114,.T.);
#42313=ADVANCED_FACE('',(#9733),#8115,.F.);
#42314=ADVANCED_FACE('',(#9734),#8116,.T.);
#42315=ADVANCED_FACE('',(#9735),#8117,.F.);
#42316=ADVANCED_FACE('',(#9736),#8118,.T.);
#42317=ADVANCED_FACE('',(#9737),#8119,.F.);
#42318=ADVANCED_FACE('',(#9738),#8120,.T.);
#42319=ADVANCED_FACE('',(#9739),#8121,.F.);
#42320=ADVANCED_FACE('',(#9740),#8122,.T.);
#42321=ADVANCED_FACE('',(#9741),#8123,.F.);
#42322=ADVANCED_FACE('',(#9742),#8124,.T.);
#42323=ADVANCED_FACE('',(#9743),#8125,.F.);
#42324=ADVANCED_FACE('',(#9744),#8126,.T.);
#42325=ADVANCED_FACE('',(#9745),#8127,.F.);
#42326=ADVANCED_FACE('',(#9746),#8128,.T.);
#42327=ADVANCED_FACE('',(#9747),#8129,.F.);
#42328=ADVANCED_FACE('',(#9748),#8130,.T.);
#42329=ADVANCED_FACE('',(#9749),#8131,.F.);
#42330=ADVANCED_FACE('',(#9750),#8132,.T.);
#42331=ADVANCED_FACE('',(#9751),#8133,.F.);
#42332=ADVANCED_FACE('',(#9752),#8134,.T.);
#42333=ADVANCED_FACE('',(#9753),#8135,.F.);
#42334=ADVANCED_FACE('',(#9754),#8136,.T.);
#42335=ADVANCED_FACE('',(#9755),#8137,.F.);
#42336=ADVANCED_FACE('',(#9756),#8138,.T.);
#42337=ADVANCED_FACE('',(#9757),#8139,.F.);
#42338=ADVANCED_FACE('',(#9758),#8140,.T.);
#42339=ADVANCED_FACE('',(#9759),#8141,.F.);
#42340=ADVANCED_FACE('',(#9760),#8142,.T.);
#42341=ADVANCED_FACE('',(#9761),#8143,.F.);
#42342=ADVANCED_FACE('',(#9762),#8144,.T.);
#42343=ADVANCED_FACE('',(#9763),#8145,.F.);
#42344=ADVANCED_FACE('',(#9764),#8146,.T.);
#42345=ADVANCED_FACE('',(#9765),#8147,.F.);
#42346=ADVANCED_FACE('',(#9766),#8148,.T.);
#42347=ADVANCED_FACE('',(#9767),#8149,.F.);
#42348=ADVANCED_FACE('',(#9768),#8150,.T.);
#42349=ADVANCED_FACE('',(#9769),#8151,.F.);
#42350=ADVANCED_FACE('',(#9770),#8152,.T.);
#42351=ADVANCED_FACE('',(#9771),#8153,.F.);
#42352=ADVANCED_FACE('',(#9772),#8154,.T.);
#42353=ADVANCED_FACE('',(#9773),#8155,.F.);
#42354=ADVANCED_FACE('',(#9774),#8156,.T.);
#42355=ADVANCED_FACE('',(#9775),#8157,.F.);
#42356=ADVANCED_FACE('',(#9776),#8158,.T.);
#42357=ADVANCED_FACE('',(#9777),#8159,.F.);
#42358=ADVANCED_FACE('',(#9778),#8160,.T.);
#42359=ADVANCED_FACE('',(#9779),#8161,.F.);
#42360=ADVANCED_FACE('',(#9780),#8162,.T.);
#42361=ADVANCED_FACE('',(#9781),#8163,.F.);
#42362=ADVANCED_FACE('',(#9782),#8164,.T.);
#42363=ADVANCED_FACE('',(#9783),#8165,.F.);
#42364=ADVANCED_FACE('',(#9784),#8166,.T.);
#42365=ADVANCED_FACE('',(#9785),#8167,.F.);
#42366=ADVANCED_FACE('',(#9786),#8168,.T.);
#42367=ADVANCED_FACE('',(#9787),#8169,.F.);
#42368=ADVANCED_FACE('',(#9788),#8170,.T.);
#42369=ADVANCED_FACE('',(#9789),#8171,.F.);
#42370=ADVANCED_FACE('',(#9790),#8172,.T.);
#42371=ADVANCED_FACE('',(#9791),#8173,.F.);
#42372=ADVANCED_FACE('',(#9792),#8174,.T.);
#42373=ADVANCED_FACE('',(#9793),#8175,.F.);
#42374=ADVANCED_FACE('',(#9794),#8176,.T.);
#42375=ADVANCED_FACE('',(#9795),#8177,.F.);
#42376=ADVANCED_FACE('',(#9796),#8178,.T.);
#42377=ADVANCED_FACE('',(#9797),#8179,.F.);
#42378=ADVANCED_FACE('',(#9798),#8180,.T.);
#42379=ADVANCED_FACE('',(#9799),#8181,.F.);
#42380=ADVANCED_FACE('',(#9800),#8182,.T.);
#42381=ADVANCED_FACE('',(#9801),#8183,.F.);
#42382=ADVANCED_FACE('',(#9802),#8184,.T.);
#42383=ADVANCED_FACE('',(#9803),#8185,.F.);
#42384=ADVANCED_FACE('',(#9804),#8186,.T.);
#42385=ADVANCED_FACE('',(#9805),#8187,.F.);
#42386=ADVANCED_FACE('',(#9806),#8188,.T.);
#42387=ADVANCED_FACE('',(#9807),#8189,.F.);
#42388=ADVANCED_FACE('',(#9808),#8190,.T.);
#42389=ADVANCED_FACE('',(#9809),#8191,.F.);
#42390=ADVANCED_FACE('',(#9810),#8192,.T.);
#42391=ADVANCED_FACE('',(#9811),#8193,.F.);
#42392=ADVANCED_FACE('',(#9812),#8194,.T.);
#42393=ADVANCED_FACE('',(#9813),#8195,.F.);
#42394=ADVANCED_FACE('',(#9814),#8196,.T.);
#42395=ADVANCED_FACE('',(#9815),#8197,.F.);
#42396=ADVANCED_FACE('',(#9816),#8198,.T.);
#42397=ADVANCED_FACE('',(#9817),#8199,.F.);
#42398=ADVANCED_FACE('',(#9818),#8200,.T.);
#42399=ADVANCED_FACE('',(#9819),#8201,.F.);
#42400=ADVANCED_FACE('',(#9820),#8202,.T.);
#42401=ADVANCED_FACE('',(#9821),#8203,.F.);
#42402=ADVANCED_FACE('',(#9822),#8204,.T.);
#42403=ADVANCED_FACE('',(#9823),#8205,.F.);
#42404=ADVANCED_FACE('',(#9824),#8206,.T.);
#42405=ADVANCED_FACE('',(#9825),#8207,.F.);
#42406=ADVANCED_FACE('',(#9826),#8208,.T.);
#42407=ADVANCED_FACE('',(#9827),#8209,.F.);
#42408=ADVANCED_FACE('',(#9828),#8210,.T.);
#42409=ADVANCED_FACE('',(#9829),#8211,.F.);
#42410=ADVANCED_FACE('',(#9830),#8212,.T.);
#42411=ADVANCED_FACE('',(#9831),#8213,.F.);
#42412=ADVANCED_FACE('',(#9832),#8214,.T.);
#42413=ADVANCED_FACE('',(#9833),#8215,.F.);
#42414=ADVANCED_FACE('',(#9834),#8216,.T.);
#42415=ADVANCED_FACE('',(#9835),#8217,.F.);
#42416=ADVANCED_FACE('',(#9836),#8218,.T.);
#42417=ADVANCED_FACE('',(#9837),#8219,.F.);
#42418=ADVANCED_FACE('',(#9838),#8220,.T.);
#42419=ADVANCED_FACE('',(#9839),#8221,.F.);
#42420=ADVANCED_FACE('',(#9840),#8222,.T.);
#42421=ADVANCED_FACE('',(#9841),#8223,.F.);
#42422=ADVANCED_FACE('',(#9842),#8224,.T.);
#42423=ADVANCED_FACE('',(#9843),#8225,.F.);
#42424=ADVANCED_FACE('',(#9844),#8226,.T.);
#42425=ADVANCED_FACE('',(#9845),#8227,.F.);
#42426=ADVANCED_FACE('',(#9846),#8228,.T.);
#42427=ADVANCED_FACE('',(#9847),#8229,.F.);
#42428=ADVANCED_FACE('',(#9848),#8230,.T.);
#42429=ADVANCED_FACE('',(#9849),#8231,.F.);
#42430=ADVANCED_FACE('',(#9850),#8232,.T.);
#42431=ADVANCED_FACE('',(#9851),#8233,.F.);
#42432=ADVANCED_FACE('',(#9852),#8234,.T.);
#42433=ADVANCED_FACE('',(#9853),#8235,.F.);
#42434=ADVANCED_FACE('',(#9854),#8236,.T.);
#42435=ADVANCED_FACE('',(#9855),#8237,.F.);
#42436=ADVANCED_FACE('',(#9856),#8238,.T.);
#42437=ADVANCED_FACE('',(#9857),#8239,.F.);
#42438=ADVANCED_FACE('',(#9858),#8240,.T.);
#42439=ADVANCED_FACE('',(#9859),#8241,.F.);
#42440=ADVANCED_FACE('',(#9860),#8242,.T.);
#42441=ADVANCED_FACE('',(#9861),#8243,.F.);
#42442=ADVANCED_FACE('',(#9862),#8244,.T.);
#42443=ADVANCED_FACE('',(#9863),#8245,.F.);
#42444=ADVANCED_FACE('',(#9864),#8246,.T.);
#42445=ADVANCED_FACE('',(#9865),#8247,.F.);
#42446=ADVANCED_FACE('',(#9866),#8248,.T.);
#42447=ADVANCED_FACE('',(#9867),#8249,.F.);
#42448=ADVANCED_FACE('',(#9868),#8250,.T.);
#42449=ADVANCED_FACE('',(#9869),#8251,.F.);
#42450=ADVANCED_FACE('',(#9870),#8252,.T.);
#42451=ADVANCED_FACE('',(#9871),#8253,.F.);
#42452=ADVANCED_FACE('',(#9872),#8254,.T.);
#42453=ADVANCED_FACE('',(#9873),#8255,.F.);
#42454=ADVANCED_FACE('',(#9874),#8256,.T.);
#42455=ADVANCED_FACE('',(#9875),#8257,.F.);
#42456=ADVANCED_FACE('',(#9876),#8258,.T.);
#42457=ADVANCED_FACE('',(#9877),#8259,.F.);
#42458=ADVANCED_FACE('',(#9878),#8260,.T.);
#42459=ADVANCED_FACE('',(#9879),#8261,.F.);
#42460=ADVANCED_FACE('',(#9880),#8262,.T.);
#42461=ADVANCED_FACE('',(#9881),#8263,.F.);
#42462=ADVANCED_FACE('',(#9882),#8264,.T.);
#42463=ADVANCED_FACE('',(#9883),#8265,.F.);
#42464=ADVANCED_FACE('',(#9884),#8266,.T.);
#42465=ADVANCED_FACE('',(#9885),#8267,.F.);
#42466=ADVANCED_FACE('',(#9886),#8268,.T.);
#42467=ADVANCED_FACE('',(#9887),#8269,.F.);
#42468=ADVANCED_FACE('',(#9888),#8270,.T.);
#42469=ADVANCED_FACE('',(#9889),#8271,.F.);
#42470=ADVANCED_FACE('',(#9890),#8272,.T.);
#42471=ADVANCED_FACE('',(#9891),#8273,.F.);
#42472=ADVANCED_FACE('',(#9892),#8274,.T.);
#42473=ADVANCED_FACE('',(#9893),#8275,.F.);
#42474=ADVANCED_FACE('',(#9894),#8276,.T.);
#42475=ADVANCED_FACE('',(#9895),#8277,.F.);
#42476=ADVANCED_FACE('',(#9896),#8278,.T.);
#42477=ADVANCED_FACE('',(#9897),#8279,.F.);
#42478=ADVANCED_FACE('',(#9898),#8280,.T.);
#42479=ADVANCED_FACE('',(#9899),#8281,.F.);
#42480=ADVANCED_FACE('',(#9900),#8282,.T.);
#42481=ADVANCED_FACE('',(#9901),#8283,.F.);
#42482=ADVANCED_FACE('',(#9902),#8284,.T.);
#42483=ADVANCED_FACE('',(#9903),#8285,.F.);
#42484=ADVANCED_FACE('',(#9904),#8286,.T.);
#42485=ADVANCED_FACE('',(#9905),#8287,.F.);
#42486=ADVANCED_FACE('',(#9906),#8288,.T.);
#42487=ADVANCED_FACE('',(#9907),#8289,.F.);
#42488=ADVANCED_FACE('',(#9908),#8290,.T.);
#42489=ADVANCED_FACE('',(#9909),#8291,.F.);
#42490=ADVANCED_FACE('',(#9910),#8292,.T.);
#42491=ADVANCED_FACE('',(#9911),#8293,.F.);
#42492=ADVANCED_FACE('',(#9912),#8294,.T.);
#42493=ADVANCED_FACE('',(#9913),#8295,.F.);
#42494=ADVANCED_FACE('',(#9914),#8296,.T.);
#42495=ADVANCED_FACE('',(#9915),#8297,.F.);
#42496=ADVANCED_FACE('',(#9916),#8298,.T.);
#42497=ADVANCED_FACE('',(#9917),#8299,.F.);
#42498=ADVANCED_FACE('',(#9918),#8300,.T.);
#42499=ADVANCED_FACE('',(#9919),#8301,.F.);
#42500=ADVANCED_FACE('',(#9920),#8302,.T.);
#42501=ADVANCED_FACE('',(#9921),#8303,.F.);
#42502=ADVANCED_FACE('',(#9922),#8304,.T.);
#42503=ADVANCED_FACE('',(#9923),#8305,.F.);
#42504=ADVANCED_FACE('',(#9924),#8306,.T.);
#42505=ADVANCED_FACE('',(#9925),#8307,.F.);
#42506=ADVANCED_FACE('',(#9926),#8308,.T.);
#42507=ADVANCED_FACE('',(#9927),#8309,.F.);
#42508=ADVANCED_FACE('',(#9928),#8310,.T.);
#42509=ADVANCED_FACE('',(#9929),#8311,.F.);
#42510=ADVANCED_FACE('',(#9930),#8312,.T.);
#42511=ADVANCED_FACE('',(#9931),#8313,.F.);
#42512=ADVANCED_FACE('',(#9932),#8314,.T.);
#42513=ADVANCED_FACE('',(#9933),#8315,.F.);
#42514=ADVANCED_FACE('',(#9934),#8316,.T.);
#42515=ADVANCED_FACE('',(#9935),#8317,.F.);
#42516=ADVANCED_FACE('',(#9936),#8318,.T.);
#42517=ADVANCED_FACE('',(#9937),#8319,.F.);
#42518=ADVANCED_FACE('',(#9938),#8320,.T.);
#42519=ADVANCED_FACE('',(#9939),#8321,.F.);
#42520=ADVANCED_FACE('',(#9940),#8322,.T.);
#42521=ADVANCED_FACE('',(#9941),#8323,.F.);
#42522=ADVANCED_FACE('',(#9942),#8324,.T.);
#42523=ADVANCED_FACE('',(#9943),#8325,.F.);
#42524=ADVANCED_FACE('',(#9944),#8326,.T.);
#42525=ADVANCED_FACE('',(#9945),#8327,.F.);
#42526=ADVANCED_FACE('',(#9946),#8328,.T.);
#42527=ADVANCED_FACE('',(#9947),#8329,.F.);
#42528=ADVANCED_FACE('',(#9948),#8330,.T.);
#42529=ADVANCED_FACE('',(#9949),#8331,.F.);
#42530=ADVANCED_FACE('',(#9950),#8332,.T.);
#42531=ADVANCED_FACE('',(#9951),#8333,.F.);
#42532=ADVANCED_FACE('',(#9952),#8334,.T.);
#42533=ADVANCED_FACE('',(#9953),#8335,.F.);
#42534=ADVANCED_FACE('',(#9954),#8336,.T.);
#42535=ADVANCED_FACE('',(#9955),#8337,.F.);
#42536=ADVANCED_FACE('',(#9956),#8338,.T.);
#42537=ADVANCED_FACE('',(#9957),#8339,.F.);
#42538=ADVANCED_FACE('',(#9958),#8340,.T.);
#42539=ADVANCED_FACE('',(#9959),#8341,.F.);
#42540=ADVANCED_FACE('',(#9960),#8342,.T.);
#42541=ADVANCED_FACE('',(#9961),#8343,.F.);
#42542=ADVANCED_FACE('',(#9962),#8344,.T.);
#42543=ADVANCED_FACE('',(#9963),#8345,.F.);
#42544=ADVANCED_FACE('',(#9964),#8346,.T.);
#42545=ADVANCED_FACE('',(#9965),#8347,.F.);
#42546=ADVANCED_FACE('',(#9966),#8348,.T.);
#42547=ADVANCED_FACE('',(#9967),#8349,.F.);
#42548=ADVANCED_FACE('',(#9968),#8350,.T.);
#42549=ADVANCED_FACE('',(#9969),#8351,.F.);
#42550=ADVANCED_FACE('',(#9970),#8352,.T.);
#42551=ADVANCED_FACE('',(#9971),#8353,.F.);
#42552=ADVANCED_FACE('',(#9972),#8354,.T.);
#42553=ADVANCED_FACE('',(#9973),#8355,.F.);
#42554=ADVANCED_FACE('',(#9974),#8356,.T.);
#42555=ADVANCED_FACE('',(#9975),#8357,.F.);
#42556=ADVANCED_FACE('',(#9976),#8358,.T.);
#42557=ADVANCED_FACE('',(#9977),#8359,.F.);
#42558=ADVANCED_FACE('',(#9978),#8360,.T.);
#42559=ADVANCED_FACE('',(#9979),#8361,.F.);
#42560=ADVANCED_FACE('',(#9980),#8362,.T.);
#42561=ADVANCED_FACE('',(#9981),#8363,.F.);
#42562=ADVANCED_FACE('',(#9982),#8364,.T.);
#42563=ADVANCED_FACE('',(#9983),#8365,.F.);
#42564=ADVANCED_FACE('',(#9984),#8366,.T.);
#42565=ADVANCED_FACE('',(#9985),#8367,.F.);
#42566=ADVANCED_FACE('',(#9986),#8368,.T.);
#42567=ADVANCED_FACE('',(#9987),#8369,.F.);
#42568=ADVANCED_FACE('',(#9988),#8370,.T.);
#42569=ADVANCED_FACE('',(#9989),#8371,.F.);
#42570=ADVANCED_FACE('',(#9990),#8372,.T.);
#42571=ADVANCED_FACE('',(#9991),#8373,.F.);
#42572=ADVANCED_FACE('',(#9992),#8374,.T.);
#42573=ADVANCED_FACE('',(#9993),#8375,.F.);
#42574=ADVANCED_FACE('',(#9994),#8376,.T.);
#42575=ADVANCED_FACE('',(#9995),#8377,.F.);
#42576=ADVANCED_FACE('',(#9996),#8378,.T.);
#42577=ADVANCED_FACE('',(#9997),#8379,.F.);
#42578=ADVANCED_FACE('',(#9998),#8380,.T.);
#42579=ADVANCED_FACE('',(#9999),#8381,.F.);
#42580=ADVANCED_FACE('',(#10000),#8382,.T.);
#42581=ADVANCED_FACE('',(#10001),#8383,.F.);
#42582=ADVANCED_FACE('',(#10002),#8384,.T.);
#42583=ADVANCED_FACE('',(#10003),#8385,.F.);
#42584=ADVANCED_FACE('',(#10004),#8386,.T.);
#42585=ADVANCED_FACE('',(#10005),#8387,.F.);
#42586=ADVANCED_FACE('',(#10006),#8388,.T.);
#42587=ADVANCED_FACE('',(#10007),#8389,.F.);
#42588=ADVANCED_FACE('',(#10008),#8390,.T.);
#42589=ADVANCED_FACE('',(#10009),#8391,.F.);
#42590=ADVANCED_FACE('',(#10010),#8392,.T.);
#42591=ADVANCED_FACE('',(#10011),#8393,.F.);
#42592=ADVANCED_FACE('',(#10012),#8394,.T.);
#42593=ADVANCED_FACE('',(#10013),#8395,.F.);
#42594=ADVANCED_FACE('',(#10014),#8396,.T.);
#42595=ADVANCED_FACE('',(#10015),#8397,.F.);
#42596=ADVANCED_FACE('',(#10016),#8398,.T.);
#42597=ADVANCED_FACE('',(#10017),#8399,.F.);
#42598=ADVANCED_FACE('',(#10018),#8400,.T.);
#42599=ADVANCED_FACE('',(#10019),#8401,.F.);
#42600=ADVANCED_FACE('',(#10020),#8402,.T.);
#42601=ADVANCED_FACE('',(#10021),#8403,.F.);
#42602=ADVANCED_FACE('',(#10022),#8404,.T.);
#42603=ADVANCED_FACE('',(#10023),#8405,.F.);
#42604=ADVANCED_FACE('',(#10024),#8406,.T.);
#42605=ADVANCED_FACE('',(#10025),#8407,.F.);
#42606=ADVANCED_FACE('',(#10026),#8408,.T.);
#42607=ADVANCED_FACE('',(#10027),#8409,.F.);
#42608=ADVANCED_FACE('',(#10028),#8410,.T.);
#42609=ADVANCED_FACE('',(#10029),#8411,.F.);
#42610=ADVANCED_FACE('',(#10030),#8412,.T.);
#42611=ADVANCED_FACE('',(#10031),#8413,.F.);
#42612=ADVANCED_FACE('',(#10032),#8414,.T.);
#42613=ADVANCED_FACE('',(#10033),#8415,.F.);
#42614=ADVANCED_FACE('',(#10034),#8416,.T.);
#42615=ADVANCED_FACE('',(#10035),#8417,.F.);
#42616=ADVANCED_FACE('',(#10036),#8418,.T.);
#42617=ADVANCED_FACE('',(#10037),#8419,.F.);
#42618=ADVANCED_FACE('',(#10038),#8420,.T.);
#42619=ADVANCED_FACE('',(#10039),#8421,.F.);
#42620=ADVANCED_FACE('',(#10040),#8422,.T.);
#42621=ADVANCED_FACE('',(#10041),#8423,.F.);
#42622=ADVANCED_FACE('',(#10042),#8424,.T.);
#42623=ADVANCED_FACE('',(#10043),#8425,.F.);
#42624=ADVANCED_FACE('',(#10044),#8426,.T.);
#42625=ADVANCED_FACE('',(#10045),#8427,.F.);
#42626=ADVANCED_FACE('',(#10046),#8428,.T.);
#42627=ADVANCED_FACE('',(#10047),#8429,.F.);
#42628=ADVANCED_FACE('',(#10048),#8430,.T.);
#42629=ADVANCED_FACE('',(#10049),#8431,.F.);
#42630=ADVANCED_FACE('',(#10050),#8432,.T.);
#42631=ADVANCED_FACE('',(#10051),#8433,.F.);
#42632=ADVANCED_FACE('',(#10052),#8434,.T.);
#42633=ADVANCED_FACE('',(#10053),#8435,.F.);
#42634=ADVANCED_FACE('',(#10054),#8436,.T.);
#42635=ADVANCED_FACE('',(#10055),#8437,.F.);
#42636=ADVANCED_FACE('',(#10056),#8438,.T.);
#42637=ADVANCED_FACE('',(#10057),#8439,.F.);
#42638=ADVANCED_FACE('',(#10058),#8440,.T.);
#42639=ADVANCED_FACE('',(#10059),#8441,.F.);
#42640=ADVANCED_FACE('',(#10060),#8442,.T.);
#42641=ADVANCED_FACE('',(#10061),#8443,.F.);
#42642=ADVANCED_FACE('',(#10062),#8444,.T.);
#42643=ADVANCED_FACE('',(#10063),#8445,.F.);
#42644=ADVANCED_FACE('',(#10064),#8446,.T.);
#42645=ADVANCED_FACE('',(#10065),#8447,.F.);
#42646=ADVANCED_FACE('',(#10066),#8448,.T.);
#42647=ADVANCED_FACE('',(#10067),#8449,.F.);
#42648=ADVANCED_FACE('',(#10068),#8450,.T.);
#42649=ADVANCED_FACE('',(#10069),#8451,.F.);
#42650=ADVANCED_FACE('',(#10070),#8452,.T.);
#42651=ADVANCED_FACE('',(#10071),#8453,.F.);
#42652=ADVANCED_FACE('',(#10072),#8454,.T.);
#42653=ADVANCED_FACE('',(#10073),#8455,.F.);
#42654=ADVANCED_FACE('',(#10074),#8456,.T.);
#42655=ADVANCED_FACE('',(#10075),#8457,.F.);
#42656=ADVANCED_FACE('',(#10076),#8458,.T.);
#42657=ADVANCED_FACE('',(#10077),#8459,.F.);
#42658=ADVANCED_FACE('',(#10078),#8460,.T.);
#42659=ADVANCED_FACE('',(#10079),#8461,.F.);
#42660=ADVANCED_FACE('',(#10080),#8462,.T.);
#42661=ADVANCED_FACE('',(#10081),#8463,.F.);
#42662=ADVANCED_FACE('',(#10082),#8464,.T.);
#42663=ADVANCED_FACE('',(#10083),#8465,.F.);
#42664=ADVANCED_FACE('',(#10084),#8466,.T.);
#42665=ADVANCED_FACE('',(#10085),#8467,.F.);
#42666=ADVANCED_FACE('',(#10086),#8468,.T.);
#42667=ADVANCED_FACE('',(#10087),#8469,.F.);
#42668=ADVANCED_FACE('',(#10088),#8470,.T.);
#42669=ADVANCED_FACE('',(#10089),#8471,.F.);
#42670=ADVANCED_FACE('',(#10090),#8472,.T.);
#42671=ADVANCED_FACE('',(#10091),#8473,.F.);
#42672=ADVANCED_FACE('',(#10092),#8474,.T.);
#42673=ADVANCED_FACE('',(#10093),#8475,.F.);
#42674=ADVANCED_FACE('',(#10094),#8476,.T.);
#42675=ADVANCED_FACE('',(#10095),#8477,.F.);
#42676=ADVANCED_FACE('',(#10096),#8478,.T.);
#42677=ADVANCED_FACE('',(#10097),#8479,.F.);
#42678=ADVANCED_FACE('',(#10098),#8480,.T.);
#42679=ADVANCED_FACE('',(#10099),#8481,.F.);
#42680=ADVANCED_FACE('',(#10100),#8482,.T.);
#42681=ADVANCED_FACE('',(#10101),#8483,.F.);
#42682=ADVANCED_FACE('',(#10102),#8484,.T.);
#42683=ADVANCED_FACE('',(#10103),#8485,.F.);
#42684=ADVANCED_FACE('',(#10104),#8486,.T.);
#42685=ADVANCED_FACE('',(#10105),#8487,.F.);
#42686=ADVANCED_FACE('',(#10106),#8488,.T.);
#42687=ADVANCED_FACE('',(#10107),#8489,.F.);
#42688=ADVANCED_FACE('',(#10108),#8490,.T.);
#42689=ADVANCED_FACE('',(#10109),#8491,.F.);
#42690=ADVANCED_FACE('',(#10110),#8492,.T.);
#42691=ADVANCED_FACE('',(#10111),#8493,.F.);
#42692=ADVANCED_FACE('',(#10112),#8494,.T.);
#42693=ADVANCED_FACE('',(#10113),#8495,.F.);
#42694=ADVANCED_FACE('',(#10114),#8496,.T.);
#42695=ADVANCED_FACE('',(#10115),#8497,.F.);
#42696=ADVANCED_FACE('',(#10116),#8498,.T.);
#42697=ADVANCED_FACE('',(#10117),#8499,.F.);
#42698=ADVANCED_FACE('',(#10118),#8500,.T.);
#42699=ADVANCED_FACE('',(#10119),#8501,.F.);
#42700=ADVANCED_FACE('',(#10120),#8502,.T.);
#42701=ADVANCED_FACE('',(#10121),#8503,.F.);
#42702=ADVANCED_FACE('',(#10122),#8504,.T.);
#42703=ADVANCED_FACE('',(#10123),#8505,.F.);
#42704=ADVANCED_FACE('',(#10124),#8506,.T.);
#42705=ADVANCED_FACE('',(#10125),#8507,.F.);
#42706=ADVANCED_FACE('',(#10126),#8508,.T.);
#42707=ADVANCED_FACE('',(#10127),#8509,.F.);
#42708=ADVANCED_FACE('',(#10128),#8510,.T.);
#42709=ADVANCED_FACE('',(#10129),#8511,.F.);
#42710=ADVANCED_FACE('',(#10130),#8512,.T.);
#42711=ADVANCED_FACE('',(#10131),#8513,.F.);
#42712=ADVANCED_FACE('',(#10132),#8514,.T.);
#42713=ADVANCED_FACE('',(#10133),#8515,.F.);
#42714=ADVANCED_FACE('',(#10134),#8516,.T.);
#42715=ADVANCED_FACE('',(#10135),#8517,.F.);
#42716=ADVANCED_FACE('',(#10136),#8518,.T.);
#42717=ADVANCED_FACE('',(#10137),#8519,.F.);
#42718=ADVANCED_FACE('',(#10138),#8520,.T.);
#42719=ADVANCED_FACE('',(#10139),#8521,.F.);
#42720=ADVANCED_FACE('',(#10140),#8522,.T.);
#42721=ADVANCED_FACE('',(#10141),#8523,.F.);
#42722=ADVANCED_FACE('',(#10142,#83,#84,#85,#86,#87,#88,#89,#90,#91,#92,
#93,#94,#95,#96,#97,#98,#99,#100,#101,#102,#103,#104,#105,#106,#107,#108,
#109,#110,#111,#112,#113,#114,#115,#116,#117,#118,#119,#120,#121,#122,#123,
#124,#125,#126,#127,#128,#129,#130),#1517,.T.);
#42723=ADVANCED_FACE('',(#10143),#41946,.T.);
#42724=ADVANCED_FACE('',(#10144),#71,.F.);
#42725=ADVANCED_FACE('',(#10145),#41947,.T.);
#42726=ADVANCED_FACE('',(#10146),#41948,.T.);
#42727=ADVANCED_FACE('',(#10147),#41949,.T.);
#42728=ADVANCED_FACE('',(#10148),#41950,.T.);
#42729=ADVANCED_FACE('',(#10149),#8524,.T.);
#42730=ADVANCED_FACE('',(#10150),#41951,.T.);
#42731=ADVANCED_FACE('',(#10151),#8525,.F.);
#42732=ADVANCED_FACE('',(#10152),#41952,.T.);
#42733=ADVANCED_FACE('',(#10153),#8526,.F.);
#42734=ADVANCED_FACE('',(#10154),#8527,.T.);
#42735=ADVANCED_FACE('',(#10155,#131),#1518,.T.);
#42736=ADVANCED_FACE('',(#10156),#2959,.F.);
#42737=ADVANCED_FACE('',(#10157),#58,.T.);
#42738=ADVANCED_FACE('',(#10158),#2960,.F.);
#42739=ADVANCED_FACE('',(#10159),#8528,.T.);
#42740=ADVANCED_FACE('',(#10160),#41953,.T.);
#42741=ADVANCED_FACE('',(#10161),#8529,.T.);
#42742=ADVANCED_FACE('',(#10162),#8530,.T.);
#42743=ADVANCED_FACE('',(#10163),#2961,.F.);
#42744=ADVANCED_FACE('',(#10164),#2962,.T.);
#42745=ADVANCED_FACE('',(#10165),#2963,.T.);
#42746=ADVANCED_FACE('',(#10166),#72,.T.);
#42747=ADVANCED_FACE('',(#10167),#73,.T.);
#42748=ADVANCED_FACE('',(#10168),#2964,.T.);
#42749=ADVANCED_FACE('',(#10169),#41954,.T.);
#42750=ADVANCED_FACE('',(#10170),#8531,.T.);
#42751=ADVANCED_FACE('',(#10171),#8532,.T.);
#42752=ADVANCED_FACE('',(#10172),#41955,.T.);
#42753=ADVANCED_FACE('',(#10173),#41956,.T.);
#42754=ADVANCED_FACE('',(#10174),#8533,.T.);
#42755=ADVANCED_FACE('',(#10175),#8534,.T.);
#42756=ADVANCED_FACE('',(#10176),#41957,.T.);
#42757=ADVANCED_FACE('',(#10177),#1519,.T.);
#42758=ADVANCED_FACE('',(#10178),#1520,.T.);
#42759=ADVANCED_FACE('',(#10179),#8535,.T.);
#42760=ADVANCED_FACE('',(#10180),#1521,.T.);
#42761=ADVANCED_FACE('',(#10181),#8536,.T.);
#42762=ADVANCED_FACE('',(#10182),#8537,.F.);
#42763=ADVANCED_FACE('',(#10183),#1522,.T.);
#42764=ADVANCED_FACE('',(#10184),#1523,.T.);
#42765=ADVANCED_FACE('',(#10185),#1524,.T.);
#42766=ADVANCED_FACE('',(#10186),#1525,.T.);
#42767=ADVANCED_FACE('',(#10187),#1526,.T.);
#42768=ADVANCED_FACE('',(#10188),#1527,.T.);
#42769=ADVANCED_FACE('',(#10189),#41958,.T.);
#42770=ADVANCED_FACE('',(#10190),#1528,.T.);
#42771=ADVANCED_FACE('',(#10191),#1529,.T.);
#42772=ADVANCED_FACE('',(#10192),#8538,.T.);
#42773=ADVANCED_FACE('',(#10193),#1530,.T.);
#42774=ADVANCED_FACE('',(#10194),#1531,.T.);
#42775=ADVANCED_FACE('',(#10195),#1532,.T.);
#42776=ADVANCED_FACE('',(#10196),#8539,.T.);
#42777=ADVANCED_FACE('',(#10197),#1533,.T.);
#42778=ADVANCED_FACE('',(#10198),#1534,.T.);
#42779=ADVANCED_FACE('',(#10199),#45,.T.);
#42780=ADVANCED_FACE('',(#10200),#46,.T.);
#42781=ADVANCED_FACE('',(#10201),#59,.T.);
#42782=ADVANCED_FACE('',(#10202),#47,.T.);
#42783=ADVANCED_FACE('',(#10203),#41959,.T.);
#42784=ADVANCED_FACE('',(#10204),#1535,.T.);
#42785=ADVANCED_FACE('',(#10205),#1536,.T.);
#42786=ADVANCED_FACE('',(#10206),#74,.T.);
#42787=ADVANCED_FACE('',(#10207),#1537,.T.);
#42788=ADVANCED_FACE('',(#10208),#1538,.T.);
#42789=ADVANCED_FACE('',(#10209),#1539,.T.);
#42790=ADVANCED_FACE('',(#10210),#2965,.T.);
#42791=ADVANCED_FACE('',(#10211),#1540,.T.);
#42792=ADVANCED_FACE('',(#10212),#1541,.T.);
#42793=ADVANCED_FACE('',(#10213),#1542,.T.);
#42794=ADVANCED_FACE('',(#10214),#2966,.T.);
#42795=ADVANCED_FACE('',(#10215),#2967,.T.);
#42796=ADVANCED_FACE('',(#10216),#48,.T.);
#42797=ADVANCED_FACE('',(#10217),#75,.T.);
#42798=ADVANCED_FACE('',(#10218),#1543,.T.);
#42799=ADVANCED_FACE('',(#10219,#132,#133,#134,#135,#136,#137,#138,#139,
#140,#141,#142,#143,#144,#145,#146,#147,#148,#149),#1544,.F.);
#42800=ADVANCED_FACE('',(#10220,#150,#151,#152,#153,#154,#155,#156,#157,
#158,#159,#160,#161,#162,#163,#164,#165,#166,#167,#168,#169,#170,#171,#172,
#173,#174,#175,#176,#177,#178,#179,#180,#181,#182,#183,#184,#185,#186,#187,
#188,#189,#190,#191,#192,#193,#194,#195,#196,#197,#198,#199,#200,#201,#202,
#203,#204,#205,#206,#207,#208,#209,#210,#211,#212,#213,#214,#215,#216,#217,
#218,#219,#220,#221,#222,#223,#224,#225,#226,#227,#228,#229,#230,#231,#232,
#233,#234,#235,#236,#237,#238,#239,#240,#241,#242,#243,#244,#245,#246,#247,
#248,#249,#250,#251,#252,#253,#254,#255,#256,#257,#258,#259,#260,#261,#262,
#263,#264,#265,#266,#267,#268,#269,#270,#271,#272,#273,#274,#275,#276,#277,
#278,#279,#280,#281,#282,#283,#284,#285,#286,#287,#288,#289,#290,#291,#292,
#293,#294,#295,#296,#297,#298,#299,#300,#301,#302,#303,#304,#305,#306,#307,
#308,#309,#310,#311,#312,#313,#314,#315,#316,#317,#318,#319,#320,#321,#322,
#323,#324,#325,#326,#327,#328,#329,#330,#331,#332,#333,#334,#335,#336,#337,
#338,#339,#340,#341,#342,#343,#344,#345,#346,#347,#348,#349,#350,#351,#352,
#353,#354,#355,#356,#357,#358,#359,#360,#361,#362,#363,#364,#365,#366,#367,
#368,#369,#370,#371,#372,#373,#374,#375,#376,#377,#378,#379,#380,#381,#382,
#383,#384,#385),#2968,.T.);
#42801=ADVANCED_FACE('',(#10221),#2969,.F.);
#42802=ADVANCED_FACE('',(#10222),#49,.T.);
#42803=ADVANCED_FACE('',(#10223),#1545,.T.);
#42804=ADVANCED_FACE('',(#10224),#2970,.T.);
#42805=ADVANCED_FACE('',(#10225),#2971,.T.);
#42806=ADVANCED_FACE('',(#10226),#8540,.F.);
#42807=ADVANCED_FACE('',(#10227),#2972,.F.);
#42808=ADVANCED_FACE('',(#10228,#386),#2973,.T.);
#42809=ADVANCED_FACE('',(#10229),#2974,.F.);
#42810=ADVANCED_FACE('',(#10230,#387),#2975,.T.);
#42811=ADVANCED_FACE('',(#10231),#2976,.F.);
#42812=ADVANCED_FACE('',(#10232,#388),#2977,.T.);
#42813=ADVANCED_FACE('',(#10233),#2978,.F.);
#42814=ADVANCED_FACE('',(#10234,#389),#2979,.T.);
#42815=ADVANCED_FACE('',(#10235),#2980,.F.);
#42816=ADVANCED_FACE('',(#10236,#390),#2981,.T.);
#42817=ADVANCED_FACE('',(#10237),#2982,.F.);
#42818=ADVANCED_FACE('',(#10238,#391),#2983,.T.);
#42819=ADVANCED_FACE('',(#10239),#2984,.F.);
#42820=ADVANCED_FACE('',(#10240,#392),#2985,.T.);
#42821=ADVANCED_FACE('',(#10241),#2986,.F.);
#42822=ADVANCED_FACE('',(#10242,#393),#2987,.T.);
#42823=ADVANCED_FACE('',(#10243),#2988,.F.);
#42824=ADVANCED_FACE('',(#10244,#394),#2989,.T.);
#42825=ADVANCED_FACE('',(#10245),#2990,.F.);
#42826=ADVANCED_FACE('',(#10246,#395),#2991,.T.);
#42827=ADVANCED_FACE('',(#10247),#2992,.F.);
#42828=ADVANCED_FACE('',(#10248,#396),#2993,.T.);
#42829=ADVANCED_FACE('',(#10249),#2994,.F.);
#42830=ADVANCED_FACE('',(#10250,#397),#2995,.T.);
#42831=ADVANCED_FACE('',(#10251),#2996,.F.);
#42832=ADVANCED_FACE('',(#10252,#398),#2997,.T.);
#42833=ADVANCED_FACE('',(#10253),#2998,.F.);
#42834=ADVANCED_FACE('',(#10254,#399),#2999,.T.);
#42835=ADVANCED_FACE('',(#10255),#3000,.F.);
#42836=ADVANCED_FACE('',(#10256,#400),#3001,.T.);
#42837=ADVANCED_FACE('',(#10257),#3002,.F.);
#42838=ADVANCED_FACE('',(#10258,#401),#3003,.T.);
#42839=ADVANCED_FACE('',(#10259),#3004,.F.);
#42840=ADVANCED_FACE('',(#10260,#402),#3005,.T.);
#42841=ADVANCED_FACE('',(#10261),#3006,.F.);
#42842=ADVANCED_FACE('',(#10262,#403),#3007,.T.);
#42843=ADVANCED_FACE('',(#10263),#3008,.F.);
#42844=ADVANCED_FACE('',(#10264,#404),#3009,.T.);
#42845=ADVANCED_FACE('',(#10265),#3010,.F.);
#42846=ADVANCED_FACE('',(#10266,#405),#3011,.T.);
#42847=ADVANCED_FACE('',(#10267),#3012,.F.);
#42848=ADVANCED_FACE('',(#10268,#406),#3013,.T.);
#42849=ADVANCED_FACE('',(#10269),#3014,.F.);
#42850=ADVANCED_FACE('',(#10270,#407),#3015,.T.);
#42851=ADVANCED_FACE('',(#10271),#3016,.F.);
#42852=ADVANCED_FACE('',(#10272,#408),#3017,.T.);
#42853=ADVANCED_FACE('',(#10273),#3018,.F.);
#42854=ADVANCED_FACE('',(#10274,#409),#3019,.T.);
#42855=ADVANCED_FACE('',(#10275),#3020,.F.);
#42856=ADVANCED_FACE('',(#10276,#410),#3021,.T.);
#42857=ADVANCED_FACE('',(#10277),#3022,.F.);
#42858=ADVANCED_FACE('',(#10278,#411),#3023,.T.);
#42859=ADVANCED_FACE('',(#10279),#3024,.F.);
#42860=ADVANCED_FACE('',(#10280,#412),#3025,.T.);
#42861=ADVANCED_FACE('',(#10281),#3026,.F.);
#42862=ADVANCED_FACE('',(#10282,#413),#3027,.T.);
#42863=ADVANCED_FACE('',(#10283),#3028,.F.);
#42864=ADVANCED_FACE('',(#10284,#414),#3029,.T.);
#42865=ADVANCED_FACE('',(#10285),#3030,.F.);
#42866=ADVANCED_FACE('',(#10286,#415),#3031,.T.);
#42867=ADVANCED_FACE('',(#10287),#3032,.F.);
#42868=ADVANCED_FACE('',(#10288,#416),#3033,.T.);
#42869=ADVANCED_FACE('',(#10289),#3034,.F.);
#42870=ADVANCED_FACE('',(#10290,#417),#3035,.T.);
#42871=ADVANCED_FACE('',(#10291),#3036,.F.);
#42872=ADVANCED_FACE('',(#10292,#418),#3037,.T.);
#42873=ADVANCED_FACE('',(#10293),#3038,.F.);
#42874=ADVANCED_FACE('',(#10294,#419),#3039,.T.);
#42875=ADVANCED_FACE('',(#10295),#3040,.F.);
#42876=ADVANCED_FACE('',(#10296,#420),#3041,.T.);
#42877=ADVANCED_FACE('',(#10297),#3042,.F.);
#42878=ADVANCED_FACE('',(#10298,#421),#3043,.T.);
#42879=ADVANCED_FACE('',(#10299),#3044,.F.);
#42880=ADVANCED_FACE('',(#10300,#422),#3045,.T.);
#42881=ADVANCED_FACE('',(#10301),#3046,.F.);
#42882=ADVANCED_FACE('',(#10302,#423),#3047,.T.);
#42883=ADVANCED_FACE('',(#10303),#3048,.F.);
#42884=ADVANCED_FACE('',(#10304,#424),#3049,.T.);
#42885=ADVANCED_FACE('',(#10305),#3050,.F.);
#42886=ADVANCED_FACE('',(#10306,#425),#3051,.T.);
#42887=ADVANCED_FACE('',(#10307),#3052,.F.);
#42888=ADVANCED_FACE('',(#10308,#426),#3053,.T.);
#42889=ADVANCED_FACE('',(#10309),#3054,.F.);
#42890=ADVANCED_FACE('',(#10310,#427),#3055,.T.);
#42891=ADVANCED_FACE('',(#10311),#3056,.F.);
#42892=ADVANCED_FACE('',(#10312,#428),#3057,.T.);
#42893=ADVANCED_FACE('',(#10313),#3058,.F.);
#42894=ADVANCED_FACE('',(#10314,#429),#3059,.T.);
#42895=ADVANCED_FACE('',(#10315),#3060,.F.);
#42896=ADVANCED_FACE('',(#10316,#430),#3061,.T.);
#42897=ADVANCED_FACE('',(#10317),#3062,.F.);
#42898=ADVANCED_FACE('',(#10318,#431),#3063,.T.);
#42899=ADVANCED_FACE('',(#10319),#3064,.F.);
#42900=ADVANCED_FACE('',(#10320,#432),#3065,.T.);
#42901=ADVANCED_FACE('',(#10321),#3066,.F.);
#42902=ADVANCED_FACE('',(#10322,#433),#3067,.T.);
#42903=ADVANCED_FACE('',(#10323),#3068,.F.);
#42904=ADVANCED_FACE('',(#10324,#434),#3069,.T.);
#42905=ADVANCED_FACE('',(#10325),#3070,.F.);
#42906=ADVANCED_FACE('',(#10326,#435),#3071,.T.);
#42907=ADVANCED_FACE('',(#10327),#3072,.F.);
#42908=ADVANCED_FACE('',(#10328,#436),#3073,.T.);
#42909=ADVANCED_FACE('',(#10329),#3074,.F.);
#42910=ADVANCED_FACE('',(#10330,#437),#3075,.T.);
#42911=ADVANCED_FACE('',(#10331),#3076,.F.);
#42912=ADVANCED_FACE('',(#10332,#438),#3077,.T.);
#42913=ADVANCED_FACE('',(#10333),#3078,.F.);
#42914=ADVANCED_FACE('',(#10334,#439),#3079,.T.);
#42915=ADVANCED_FACE('',(#10335),#3080,.F.);
#42916=ADVANCED_FACE('',(#10336,#440),#3081,.T.);
#42917=ADVANCED_FACE('',(#10337),#3082,.F.);
#42918=ADVANCED_FACE('',(#10338,#441),#3083,.T.);
#42919=ADVANCED_FACE('',(#10339),#3084,.F.);
#42920=ADVANCED_FACE('',(#10340,#442),#3085,.T.);
#42921=ADVANCED_FACE('',(#10341),#3086,.F.);
#42922=ADVANCED_FACE('',(#10342,#443),#3087,.T.);
#42923=ADVANCED_FACE('',(#10343),#3088,.F.);
#42924=ADVANCED_FACE('',(#10344,#444),#3089,.T.);
#42925=ADVANCED_FACE('',(#10345),#3090,.F.);
#42926=ADVANCED_FACE('',(#10346,#445),#3091,.T.);
#42927=ADVANCED_FACE('',(#10347),#3092,.F.);
#42928=ADVANCED_FACE('',(#10348,#446),#3093,.T.);
#42929=ADVANCED_FACE('',(#10349),#3094,.F.);
#42930=ADVANCED_FACE('',(#10350,#447),#3095,.T.);
#42931=ADVANCED_FACE('',(#10351),#3096,.F.);
#42932=ADVANCED_FACE('',(#10352,#448),#3097,.T.);
#42933=ADVANCED_FACE('',(#10353),#3098,.F.);
#42934=ADVANCED_FACE('',(#10354,#449),#3099,.T.);
#42935=ADVANCED_FACE('',(#10355),#3100,.F.);
#42936=ADVANCED_FACE('',(#10356,#450),#3101,.T.);
#42937=ADVANCED_FACE('',(#10357),#3102,.F.);
#42938=ADVANCED_FACE('',(#10358,#451),#3103,.T.);
#42939=ADVANCED_FACE('',(#10359),#3104,.F.);
#42940=ADVANCED_FACE('',(#10360,#452),#3105,.T.);
#42941=ADVANCED_FACE('',(#10361),#3106,.F.);
#42942=ADVANCED_FACE('',(#10362,#453),#3107,.T.);
#42943=ADVANCED_FACE('',(#10363),#3108,.F.);
#42944=ADVANCED_FACE('',(#10364,#454),#3109,.T.);
#42945=ADVANCED_FACE('',(#10365),#3110,.F.);
#42946=ADVANCED_FACE('',(#10366,#455),#3111,.T.);
#42947=ADVANCED_FACE('',(#10367),#3112,.F.);
#42948=ADVANCED_FACE('',(#10368,#456),#3113,.T.);
#42949=ADVANCED_FACE('',(#10369),#3114,.F.);
#42950=ADVANCED_FACE('',(#10370,#457),#3115,.T.);
#42951=ADVANCED_FACE('',(#10371),#3116,.F.);
#42952=ADVANCED_FACE('',(#10372,#458),#3117,.T.);
#42953=ADVANCED_FACE('',(#10373),#3118,.F.);
#42954=ADVANCED_FACE('',(#10374,#459),#3119,.T.);
#42955=ADVANCED_FACE('',(#10375),#3120,.F.);
#42956=ADVANCED_FACE('',(#10376,#460),#3121,.T.);
#42957=ADVANCED_FACE('',(#10377),#3122,.F.);
#42958=ADVANCED_FACE('',(#10378,#461),#3123,.T.);
#42959=ADVANCED_FACE('',(#10379),#3124,.F.);
#42960=ADVANCED_FACE('',(#10380,#462),#3125,.T.);
#42961=ADVANCED_FACE('',(#10381),#3126,.F.);
#42962=ADVANCED_FACE('',(#10382,#463),#3127,.T.);
#42963=ADVANCED_FACE('',(#10383),#3128,.F.);
#42964=ADVANCED_FACE('',(#10384,#464),#3129,.T.);
#42965=ADVANCED_FACE('',(#10385),#3130,.F.);
#42966=ADVANCED_FACE('',(#10386,#465),#3131,.T.);
#42967=ADVANCED_FACE('',(#10387),#3132,.F.);
#42968=ADVANCED_FACE('',(#10388,#466),#3133,.T.);
#42969=ADVANCED_FACE('',(#10389),#3134,.F.);
#42970=ADVANCED_FACE('',(#10390,#467),#3135,.T.);
#42971=ADVANCED_FACE('',(#10391),#3136,.F.);
#42972=ADVANCED_FACE('',(#10392,#468),#3137,.T.);
#42973=ADVANCED_FACE('',(#10393),#3138,.F.);
#42974=ADVANCED_FACE('',(#10394,#469),#3139,.T.);
#42975=ADVANCED_FACE('',(#10395),#3140,.F.);
#42976=ADVANCED_FACE('',(#10396,#470),#3141,.T.);
#42977=ADVANCED_FACE('',(#10397),#3142,.F.);
#42978=ADVANCED_FACE('',(#10398,#471),#3143,.T.);
#42979=ADVANCED_FACE('',(#10399),#3144,.F.);
#42980=ADVANCED_FACE('',(#10400,#472),#3145,.T.);
#42981=ADVANCED_FACE('',(#10401),#3146,.F.);
#42982=ADVANCED_FACE('',(#10402,#473),#3147,.T.);
#42983=ADVANCED_FACE('',(#10403),#3148,.F.);
#42984=ADVANCED_FACE('',(#10404,#474),#3149,.T.);
#42985=ADVANCED_FACE('',(#10405),#3150,.F.);
#42986=ADVANCED_FACE('',(#10406,#475),#3151,.T.);
#42987=ADVANCED_FACE('',(#10407),#3152,.F.);
#42988=ADVANCED_FACE('',(#10408,#476),#3153,.T.);
#42989=ADVANCED_FACE('',(#10409),#3154,.F.);
#42990=ADVANCED_FACE('',(#10410,#477),#3155,.T.);
#42991=ADVANCED_FACE('',(#10411),#3156,.F.);
#42992=ADVANCED_FACE('',(#10412,#478),#3157,.T.);
#42993=ADVANCED_FACE('',(#10413),#3158,.F.);
#42994=ADVANCED_FACE('',(#10414,#479),#3159,.T.);
#42995=ADVANCED_FACE('',(#10415),#3160,.F.);
#42996=ADVANCED_FACE('',(#10416,#480),#3161,.T.);
#42997=ADVANCED_FACE('',(#10417),#3162,.F.);
#42998=ADVANCED_FACE('',(#10418,#481),#3163,.T.);
#42999=ADVANCED_FACE('',(#10419),#3164,.F.);
#43000=ADVANCED_FACE('',(#10420,#482),#3165,.T.);
#43001=ADVANCED_FACE('',(#10421),#3166,.F.);
#43002=ADVANCED_FACE('',(#10422,#483),#3167,.T.);
#43003=ADVANCED_FACE('',(#10423),#3168,.F.);
#43004=ADVANCED_FACE('',(#10424,#484),#3169,.T.);
#43005=ADVANCED_FACE('',(#10425),#3170,.F.);
#43006=ADVANCED_FACE('',(#10426,#485),#3171,.T.);
#43007=ADVANCED_FACE('',(#10427),#3172,.F.);
#43008=ADVANCED_FACE('',(#10428,#486),#3173,.T.);
#43009=ADVANCED_FACE('',(#10429),#3174,.F.);
#43010=ADVANCED_FACE('',(#10430,#487),#3175,.T.);
#43011=ADVANCED_FACE('',(#10431),#3176,.F.);
#43012=ADVANCED_FACE('',(#10432,#488),#3177,.T.);
#43013=ADVANCED_FACE('',(#10433),#3178,.F.);
#43014=ADVANCED_FACE('',(#10434,#489),#3179,.T.);
#43015=ADVANCED_FACE('',(#10435),#3180,.F.);
#43016=ADVANCED_FACE('',(#10436,#490),#3181,.T.);
#43017=ADVANCED_FACE('',(#10437),#3182,.F.);
#43018=ADVANCED_FACE('',(#10438,#491),#3183,.T.);
#43019=ADVANCED_FACE('',(#10439),#3184,.F.);
#43020=ADVANCED_FACE('',(#10440,#492),#3185,.T.);
#43021=ADVANCED_FACE('',(#10441),#3186,.F.);
#43022=ADVANCED_FACE('',(#10442,#493),#3187,.T.);
#43023=ADVANCED_FACE('',(#10443),#3188,.F.);
#43024=ADVANCED_FACE('',(#10444,#494),#3189,.T.);
#43025=ADVANCED_FACE('',(#10445),#3190,.F.);
#43026=ADVANCED_FACE('',(#10446,#495),#3191,.T.);
#43027=ADVANCED_FACE('',(#10447),#3192,.F.);
#43028=ADVANCED_FACE('',(#10448,#496),#3193,.T.);
#43029=ADVANCED_FACE('',(#10449),#3194,.F.);
#43030=ADVANCED_FACE('',(#10450,#497),#3195,.T.);
#43031=ADVANCED_FACE('',(#10451),#3196,.F.);
#43032=ADVANCED_FACE('',(#10452,#498),#3197,.T.);
#43033=ADVANCED_FACE('',(#10453),#3198,.F.);
#43034=ADVANCED_FACE('',(#10454,#499),#3199,.T.);
#43035=ADVANCED_FACE('',(#10455),#3200,.F.);
#43036=ADVANCED_FACE('',(#10456,#500),#3201,.T.);
#43037=ADVANCED_FACE('',(#10457),#3202,.F.);
#43038=ADVANCED_FACE('',(#10458,#501),#3203,.T.);
#43039=ADVANCED_FACE('',(#10459),#3204,.F.);
#43040=ADVANCED_FACE('',(#10460,#502),#3205,.T.);
#43041=ADVANCED_FACE('',(#10461),#3206,.F.);
#43042=ADVANCED_FACE('',(#10462,#503),#3207,.T.);
#43043=ADVANCED_FACE('',(#10463),#3208,.F.);
#43044=ADVANCED_FACE('',(#10464,#504),#3209,.T.);
#43045=ADVANCED_FACE('',(#10465),#3210,.F.);
#43046=ADVANCED_FACE('',(#10466,#505),#3211,.T.);
#43047=ADVANCED_FACE('',(#10467),#3212,.F.);
#43048=ADVANCED_FACE('',(#10468,#506),#3213,.T.);
#43049=ADVANCED_FACE('',(#10469),#3214,.F.);
#43050=ADVANCED_FACE('',(#10470,#507),#3215,.T.);
#43051=ADVANCED_FACE('',(#10471),#3216,.F.);
#43052=ADVANCED_FACE('',(#10472,#508),#3217,.T.);
#43053=ADVANCED_FACE('',(#10473),#3218,.F.);
#43054=ADVANCED_FACE('',(#10474,#509),#3219,.T.);
#43055=ADVANCED_FACE('',(#10475),#3220,.F.);
#43056=ADVANCED_FACE('',(#10476,#510),#3221,.T.);
#43057=ADVANCED_FACE('',(#10477),#3222,.F.);
#43058=ADVANCED_FACE('',(#10478,#511),#3223,.T.);
#43059=ADVANCED_FACE('',(#10479),#3224,.F.);
#43060=ADVANCED_FACE('',(#10480,#512),#3225,.T.);
#43061=ADVANCED_FACE('',(#10481),#3226,.F.);
#43062=ADVANCED_FACE('',(#10482,#513),#3227,.T.);
#43063=ADVANCED_FACE('',(#10483),#3228,.F.);
#43064=ADVANCED_FACE('',(#10484,#514),#3229,.T.);
#43065=ADVANCED_FACE('',(#10485),#3230,.F.);
#43066=ADVANCED_FACE('',(#10486,#515),#3231,.T.);
#43067=ADVANCED_FACE('',(#10487),#3232,.F.);
#43068=ADVANCED_FACE('',(#10488,#516),#3233,.T.);
#43069=ADVANCED_FACE('',(#10489),#3234,.F.);
#43070=ADVANCED_FACE('',(#10490,#517),#3235,.T.);
#43071=ADVANCED_FACE('',(#10491),#3236,.F.);
#43072=ADVANCED_FACE('',(#10492,#518),#3237,.T.);
#43073=ADVANCED_FACE('',(#10493),#3238,.F.);
#43074=ADVANCED_FACE('',(#10494,#519),#3239,.T.);
#43075=ADVANCED_FACE('',(#10495),#3240,.F.);
#43076=ADVANCED_FACE('',(#10496,#520),#3241,.T.);
#43077=ADVANCED_FACE('',(#10497),#3242,.F.);
#43078=ADVANCED_FACE('',(#10498,#521),#3243,.T.);
#43079=ADVANCED_FACE('',(#10499),#3244,.F.);
#43080=ADVANCED_FACE('',(#10500,#522),#3245,.T.);
#43081=ADVANCED_FACE('',(#10501),#3246,.F.);
#43082=ADVANCED_FACE('',(#10502,#523),#3247,.T.);
#43083=ADVANCED_FACE('',(#10503),#3248,.F.);
#43084=ADVANCED_FACE('',(#10504,#524),#3249,.T.);
#43085=ADVANCED_FACE('',(#10505),#3250,.F.);
#43086=ADVANCED_FACE('',(#10506,#525),#3251,.T.);
#43087=ADVANCED_FACE('',(#10507),#3252,.F.);
#43088=ADVANCED_FACE('',(#10508,#526),#3253,.T.);
#43089=ADVANCED_FACE('',(#10509),#3254,.F.);
#43090=ADVANCED_FACE('',(#10510,#527),#3255,.T.);
#43091=ADVANCED_FACE('',(#10511),#3256,.F.);
#43092=ADVANCED_FACE('',(#10512,#528),#3257,.T.);
#43093=ADVANCED_FACE('',(#10513),#3258,.F.);
#43094=ADVANCED_FACE('',(#10514,#529),#3259,.T.);
#43095=ADVANCED_FACE('',(#10515),#3260,.F.);
#43096=ADVANCED_FACE('',(#10516,#530),#3261,.T.);
#43097=ADVANCED_FACE('',(#10517),#3262,.F.);
#43098=ADVANCED_FACE('',(#10518,#531),#3263,.T.);
#43099=ADVANCED_FACE('',(#10519),#3264,.F.);
#43100=ADVANCED_FACE('',(#10520,#532),#3265,.T.);
#43101=ADVANCED_FACE('',(#10521),#3266,.F.);
#43102=ADVANCED_FACE('',(#10522,#533),#3267,.T.);
#43103=ADVANCED_FACE('',(#10523),#3268,.F.);
#43104=ADVANCED_FACE('',(#10524,#534),#3269,.T.);
#43105=ADVANCED_FACE('',(#10525),#3270,.F.);
#43106=ADVANCED_FACE('',(#10526,#535),#3271,.T.);
#43107=ADVANCED_FACE('',(#10527),#3272,.F.);
#43108=ADVANCED_FACE('',(#10528,#536),#3273,.T.);
#43109=ADVANCED_FACE('',(#10529),#3274,.F.);
#43110=ADVANCED_FACE('',(#10530,#537),#3275,.T.);
#43111=ADVANCED_FACE('',(#10531),#3276,.F.);
#43112=ADVANCED_FACE('',(#10532,#538),#3277,.T.);
#43113=ADVANCED_FACE('',(#10533),#3278,.F.);
#43114=ADVANCED_FACE('',(#10534,#539),#3279,.T.);
#43115=ADVANCED_FACE('',(#10535),#3280,.F.);
#43116=ADVANCED_FACE('',(#10536,#540),#3281,.T.);
#43117=ADVANCED_FACE('',(#10537),#3282,.F.);
#43118=ADVANCED_FACE('',(#10538,#541),#3283,.T.);
#43119=ADVANCED_FACE('',(#10539),#3284,.F.);
#43120=ADVANCED_FACE('',(#10540,#542),#3285,.T.);
#43121=ADVANCED_FACE('',(#10541),#3286,.F.);
#43122=ADVANCED_FACE('',(#10542,#543),#3287,.T.);
#43123=ADVANCED_FACE('',(#10543),#3288,.F.);
#43124=ADVANCED_FACE('',(#10544,#544),#3289,.T.);
#43125=ADVANCED_FACE('',(#10545),#3290,.F.);
#43126=ADVANCED_FACE('',(#10546,#545),#3291,.T.);
#43127=ADVANCED_FACE('',(#10547),#3292,.F.);
#43128=ADVANCED_FACE('',(#10548,#546),#3293,.T.);
#43129=ADVANCED_FACE('',(#10549),#3294,.F.);
#43130=ADVANCED_FACE('',(#10550,#547),#3295,.T.);
#43131=ADVANCED_FACE('',(#10551),#3296,.F.);
#43132=ADVANCED_FACE('',(#10552,#548),#3297,.T.);
#43133=ADVANCED_FACE('',(#10553),#3298,.F.);
#43134=ADVANCED_FACE('',(#10554,#549),#3299,.T.);
#43135=ADVANCED_FACE('',(#10555),#3300,.F.);
#43136=ADVANCED_FACE('',(#10556,#550),#3301,.T.);
#43137=ADVANCED_FACE('',(#10557),#3302,.F.);
#43138=ADVANCED_FACE('',(#10558,#551),#3303,.T.);
#43139=ADVANCED_FACE('',(#10559),#3304,.F.);
#43140=ADVANCED_FACE('',(#10560,#552),#3305,.T.);
#43141=ADVANCED_FACE('',(#10561),#3306,.F.);
#43142=ADVANCED_FACE('',(#10562,#553),#3307,.T.);
#43143=ADVANCED_FACE('',(#10563),#3308,.F.);
#43144=ADVANCED_FACE('',(#10564,#554),#3309,.T.);
#43145=ADVANCED_FACE('',(#10565),#3310,.F.);
#43146=ADVANCED_FACE('',(#10566,#555),#3311,.T.);
#43147=ADVANCED_FACE('',(#10567),#3312,.F.);
#43148=ADVANCED_FACE('',(#10568,#556),#3313,.T.);
#43149=ADVANCED_FACE('',(#10569),#3314,.F.);
#43150=ADVANCED_FACE('',(#10570,#557),#3315,.T.);
#43151=ADVANCED_FACE('',(#10571),#3316,.F.);
#43152=ADVANCED_FACE('',(#10572,#558),#3317,.T.);
#43153=ADVANCED_FACE('',(#10573),#3318,.F.);
#43154=ADVANCED_FACE('',(#10574,#559),#3319,.T.);
#43155=ADVANCED_FACE('',(#10575),#3320,.F.);
#43156=ADVANCED_FACE('',(#10576,#560),#3321,.T.);
#43157=ADVANCED_FACE('',(#10577),#3322,.F.);
#43158=ADVANCED_FACE('',(#10578,#561),#3323,.T.);
#43159=ADVANCED_FACE('',(#10579),#3324,.F.);
#43160=ADVANCED_FACE('',(#10580,#562),#3325,.T.);
#43161=ADVANCED_FACE('',(#10581),#3326,.F.);
#43162=ADVANCED_FACE('',(#10582,#563),#3327,.T.);
#43163=ADVANCED_FACE('',(#10583),#3328,.F.);
#43164=ADVANCED_FACE('',(#10584,#564),#3329,.T.);
#43165=ADVANCED_FACE('',(#10585),#3330,.F.);
#43166=ADVANCED_FACE('',(#10586,#565),#3331,.T.);
#43167=ADVANCED_FACE('',(#10587),#3332,.F.);
#43168=ADVANCED_FACE('',(#10588,#566),#3333,.T.);
#43169=ADVANCED_FACE('',(#10589),#3334,.F.);
#43170=ADVANCED_FACE('',(#10590,#567),#3335,.T.);
#43171=ADVANCED_FACE('',(#10591),#3336,.F.);
#43172=ADVANCED_FACE('',(#10592,#568),#3337,.T.);
#43173=ADVANCED_FACE('',(#10593),#3338,.F.);
#43174=ADVANCED_FACE('',(#10594,#569),#3339,.T.);
#43175=ADVANCED_FACE('',(#10595),#3340,.F.);
#43176=ADVANCED_FACE('',(#10596,#570),#3341,.T.);
#43177=ADVANCED_FACE('',(#10597),#3342,.F.);
#43178=ADVANCED_FACE('',(#10598,#571),#3343,.T.);
#43179=ADVANCED_FACE('',(#10599),#3344,.F.);
#43180=ADVANCED_FACE('',(#10600,#572),#3345,.T.);
#43181=ADVANCED_FACE('',(#10601),#3346,.F.);
#43182=ADVANCED_FACE('',(#10602,#573),#3347,.T.);
#43183=ADVANCED_FACE('',(#10603),#3348,.F.);
#43184=ADVANCED_FACE('',(#10604,#574),#3349,.T.);
#43185=ADVANCED_FACE('',(#10605),#3350,.F.);
#43186=ADVANCED_FACE('',(#10606,#575),#3351,.T.);
#43187=ADVANCED_FACE('',(#10607),#3352,.F.);
#43188=ADVANCED_FACE('',(#10608,#576),#3353,.T.);
#43189=ADVANCED_FACE('',(#10609),#3354,.F.);
#43190=ADVANCED_FACE('',(#10610,#577),#3355,.T.);
#43191=ADVANCED_FACE('',(#10611),#3356,.F.);
#43192=ADVANCED_FACE('',(#10612,#578),#3357,.T.);
#43193=ADVANCED_FACE('',(#10613),#3358,.F.);
#43194=ADVANCED_FACE('',(#10614,#579),#3359,.T.);
#43195=ADVANCED_FACE('',(#10615),#3360,.F.);
#43196=ADVANCED_FACE('',(#10616,#580),#3361,.T.);
#43197=ADVANCED_FACE('',(#10617),#3362,.F.);
#43198=ADVANCED_FACE('',(#10618,#581),#3363,.T.);
#43199=ADVANCED_FACE('',(#10619),#3364,.F.);
#43200=ADVANCED_FACE('',(#10620,#582),#3365,.T.);
#43201=ADVANCED_FACE('',(#10621),#3366,.F.);
#43202=ADVANCED_FACE('',(#10622,#583),#3367,.T.);
#43203=ADVANCED_FACE('',(#10623),#3368,.F.);
#43204=ADVANCED_FACE('',(#10624,#584),#3369,.T.);
#43205=ADVANCED_FACE('',(#10625),#3370,.F.);
#43206=ADVANCED_FACE('',(#10626,#585),#3371,.T.);
#43207=ADVANCED_FACE('',(#10627),#3372,.F.);
#43208=ADVANCED_FACE('',(#10628,#586),#3373,.T.);
#43209=ADVANCED_FACE('',(#10629),#3374,.F.);
#43210=ADVANCED_FACE('',(#10630,#587),#3375,.T.);
#43211=ADVANCED_FACE('',(#10631),#3376,.F.);
#43212=ADVANCED_FACE('',(#10632,#588),#3377,.T.);
#43213=ADVANCED_FACE('',(#10633),#3378,.F.);
#43214=ADVANCED_FACE('',(#10634,#589),#3379,.T.);
#43215=ADVANCED_FACE('',(#10635),#3380,.F.);
#43216=ADVANCED_FACE('',(#10636,#590),#3381,.T.);
#43217=ADVANCED_FACE('',(#10637),#3382,.F.);
#43218=ADVANCED_FACE('',(#10638,#591),#3383,.T.);
#43219=ADVANCED_FACE('',(#10639),#3384,.F.);
#43220=ADVANCED_FACE('',(#10640,#592),#3385,.T.);
#43221=ADVANCED_FACE('',(#10641),#3386,.F.);
#43222=ADVANCED_FACE('',(#10642,#593),#3387,.T.);
#43223=ADVANCED_FACE('',(#10643),#3388,.F.);
#43224=ADVANCED_FACE('',(#10644,#594),#3389,.T.);
#43225=ADVANCED_FACE('',(#10645),#3390,.F.);
#43226=ADVANCED_FACE('',(#10646,#595),#3391,.T.);
#43227=ADVANCED_FACE('',(#10647),#3392,.F.);
#43228=ADVANCED_FACE('',(#10648,#596),#3393,.T.);
#43229=ADVANCED_FACE('',(#10649),#3394,.F.);
#43230=ADVANCED_FACE('',(#10650,#597),#3395,.T.);
#43231=ADVANCED_FACE('',(#10651),#3396,.F.);
#43232=ADVANCED_FACE('',(#10652,#598),#3397,.T.);
#43233=ADVANCED_FACE('',(#10653),#3398,.F.);
#43234=ADVANCED_FACE('',(#10654,#599),#3399,.T.);
#43235=ADVANCED_FACE('',(#10655),#3400,.F.);
#43236=ADVANCED_FACE('',(#10656,#600),#3401,.T.);
#43237=ADVANCED_FACE('',(#10657),#3402,.F.);
#43238=ADVANCED_FACE('',(#10658,#601),#3403,.T.);
#43239=ADVANCED_FACE('',(#10659),#3404,.F.);
#43240=ADVANCED_FACE('',(#10660,#602),#3405,.T.);
#43241=ADVANCED_FACE('',(#10661),#3406,.F.);
#43242=ADVANCED_FACE('',(#10662,#603),#3407,.T.);
#43243=ADVANCED_FACE('',(#10663),#3408,.F.);
#43244=ADVANCED_FACE('',(#10664,#604),#3409,.T.);
#43245=ADVANCED_FACE('',(#10665),#3410,.F.);
#43246=ADVANCED_FACE('',(#10666,#605),#3411,.T.);
#43247=ADVANCED_FACE('',(#10667),#3412,.F.);
#43248=ADVANCED_FACE('',(#10668,#606),#3413,.T.);
#43249=ADVANCED_FACE('',(#10669),#3414,.F.);
#43250=ADVANCED_FACE('',(#10670,#607),#3415,.T.);
#43251=ADVANCED_FACE('',(#10671),#3416,.F.);
#43252=ADVANCED_FACE('',(#10672,#608),#3417,.T.);
#43253=ADVANCED_FACE('',(#10673),#3418,.F.);
#43254=ADVANCED_FACE('',(#10674,#609),#3419,.T.);
#43255=ADVANCED_FACE('',(#10675),#3420,.F.);
#43256=ADVANCED_FACE('',(#10676,#610),#3421,.T.);
#43257=ADVANCED_FACE('',(#10677),#3422,.F.);
#43258=ADVANCED_FACE('',(#10678,#611),#3423,.T.);
#43259=ADVANCED_FACE('',(#10679),#3424,.F.);
#43260=ADVANCED_FACE('',(#10680,#612),#3425,.T.);
#43261=ADVANCED_FACE('',(#10681),#3426,.F.);
#43262=ADVANCED_FACE('',(#10682,#613),#3427,.T.);
#43263=ADVANCED_FACE('',(#10683),#3428,.F.);
#43264=ADVANCED_FACE('',(#10684,#614),#3429,.T.);
#43265=ADVANCED_FACE('',(#10685),#3430,.F.);
#43266=ADVANCED_FACE('',(#10686,#615),#3431,.T.);
#43267=ADVANCED_FACE('',(#10687),#3432,.F.);
#43268=ADVANCED_FACE('',(#10688,#616),#3433,.T.);
#43269=ADVANCED_FACE('',(#10689),#3434,.F.);
#43270=ADVANCED_FACE('',(#10690,#617),#3435,.T.);
#43271=ADVANCED_FACE('',(#10691),#3436,.F.);
#43272=ADVANCED_FACE('',(#10692,#618),#3437,.T.);
#43273=ADVANCED_FACE('',(#10693),#3438,.F.);
#43274=ADVANCED_FACE('',(#10694,#619),#3439,.T.);
#43275=ADVANCED_FACE('',(#10695),#3440,.F.);
#43276=ADVANCED_FACE('',(#10696,#620),#3441,.T.);
#43277=ADVANCED_FACE('',(#10697),#3442,.F.);
#43278=ADVANCED_FACE('',(#10698,#621),#3443,.T.);
#43279=ADVANCED_FACE('',(#10699),#3444,.F.);
#43280=ADVANCED_FACE('',(#10700,#622),#3445,.T.);
#43281=ADVANCED_FACE('',(#10701),#3446,.F.);
#43282=ADVANCED_FACE('',(#10702,#623),#3447,.T.);
#43283=ADVANCED_FACE('',(#10703),#3448,.F.);
#43284=ADVANCED_FACE('',(#10704,#624),#3449,.T.);
#43285=ADVANCED_FACE('',(#10705),#3450,.F.);
#43286=ADVANCED_FACE('',(#10706,#625),#3451,.T.);
#43287=ADVANCED_FACE('',(#10707),#3452,.F.);
#43288=ADVANCED_FACE('',(#10708,#626),#3453,.T.);
#43289=ADVANCED_FACE('',(#10709),#3454,.F.);
#43290=ADVANCED_FACE('',(#10710,#627),#3455,.T.);
#43291=ADVANCED_FACE('',(#10711),#3456,.F.);
#43292=ADVANCED_FACE('',(#10712,#628),#3457,.T.);
#43293=ADVANCED_FACE('',(#10713),#3458,.F.);
#43294=ADVANCED_FACE('',(#10714,#629),#3459,.T.);
#43295=ADVANCED_FACE('',(#10715),#3460,.F.);
#43296=ADVANCED_FACE('',(#10716,#630),#3461,.T.);
#43297=ADVANCED_FACE('',(#10717),#3462,.F.);
#43298=ADVANCED_FACE('',(#10718,#631),#3463,.T.);
#43299=ADVANCED_FACE('',(#10719),#3464,.F.);
#43300=ADVANCED_FACE('',(#10720,#632),#3465,.T.);
#43301=ADVANCED_FACE('',(#10721),#3466,.F.);
#43302=ADVANCED_FACE('',(#10722,#633),#3467,.T.);
#43303=ADVANCED_FACE('',(#10723),#3468,.F.);
#43304=ADVANCED_FACE('',(#10724,#634),#3469,.T.);
#43305=ADVANCED_FACE('',(#10725),#3470,.F.);
#43306=ADVANCED_FACE('',(#10726,#635),#3471,.T.);
#43307=ADVANCED_FACE('',(#10727),#3472,.F.);
#43308=ADVANCED_FACE('',(#10728,#636),#3473,.T.);
#43309=ADVANCED_FACE('',(#10729),#3474,.F.);
#43310=ADVANCED_FACE('',(#10730,#637),#3475,.T.);
#43311=ADVANCED_FACE('',(#10731),#3476,.F.);
#43312=ADVANCED_FACE('',(#10732,#638),#3477,.T.);
#43313=ADVANCED_FACE('',(#10733),#3478,.F.);
#43314=ADVANCED_FACE('',(#10734,#639),#3479,.T.);
#43315=ADVANCED_FACE('',(#10735),#3480,.F.);
#43316=ADVANCED_FACE('',(#10736,#640),#3481,.T.);
#43317=ADVANCED_FACE('',(#10737),#3482,.F.);
#43318=ADVANCED_FACE('',(#10738,#641),#3483,.T.);
#43319=ADVANCED_FACE('',(#10739),#3484,.F.);
#43320=ADVANCED_FACE('',(#10740,#642),#3485,.T.);
#43321=ADVANCED_FACE('',(#10741),#3486,.F.);
#43322=ADVANCED_FACE('',(#10742,#643),#3487,.T.);
#43323=ADVANCED_FACE('',(#10743),#3488,.F.);
#43324=ADVANCED_FACE('',(#10744,#644),#1546,.T.);
#43325=ADVANCED_FACE('',(#10745),#3489,.F.);
#43326=ADVANCED_FACE('',(#10746,#645),#1547,.T.);
#43327=ADVANCED_FACE('',(#10747),#3490,.F.);
#43328=ADVANCED_FACE('',(#10748,#646),#1548,.T.);
#43329=ADVANCED_FACE('',(#10749),#3491,.F.);
#43330=ADVANCED_FACE('',(#10750,#647),#1549,.T.);
#43331=ADVANCED_FACE('',(#10751),#3492,.F.);
#43332=ADVANCED_FACE('',(#10752,#648),#1550,.T.);
#43333=ADVANCED_FACE('',(#10753),#3493,.F.);
#43334=ADVANCED_FACE('',(#10754,#649),#1551,.T.);
#43335=ADVANCED_FACE('',(#10755),#3494,.F.);
#43336=ADVANCED_FACE('',(#10756,#650),#1552,.T.);
#43337=ADVANCED_FACE('',(#10757),#3495,.F.);
#43338=ADVANCED_FACE('',(#10758,#651),#1553,.T.);
#43339=ADVANCED_FACE('',(#10759),#3496,.F.);
#43340=ADVANCED_FACE('',(#10760,#652),#1554,.T.);
#43341=ADVANCED_FACE('',(#10761),#3497,.F.);
#43342=ADVANCED_FACE('',(#10762,#653),#1555,.T.);
#43343=ADVANCED_FACE('',(#10763),#3498,.F.);
#43344=ADVANCED_FACE('',(#10764,#654),#1556,.T.);
#43345=ADVANCED_FACE('',(#10765),#3499,.F.);
#43346=ADVANCED_FACE('',(#10766,#655),#1557,.T.);
#43347=ADVANCED_FACE('',(#10767),#3500,.F.);
#43348=ADVANCED_FACE('',(#10768,#656),#1558,.T.);
#43349=ADVANCED_FACE('',(#10769),#3501,.F.);
#43350=ADVANCED_FACE('',(#10770,#657),#1559,.T.);
#43351=ADVANCED_FACE('',(#10771),#3502,.F.);
#43352=ADVANCED_FACE('',(#10772,#658),#3503,.T.);
#43353=ADVANCED_FACE('',(#10773),#3504,.F.);
#43354=ADVANCED_FACE('',(#10774,#659),#1560,.T.);
#43355=ADVANCED_FACE('',(#10775),#3505,.F.);
#43356=ADVANCED_FACE('',(#10776,#660),#1561,.T.);
#43357=ADVANCED_FACE('',(#10777),#3506,.F.);
#43358=ADVANCED_FACE('',(#10778,#661),#3507,.T.);
#43359=ADVANCED_FACE('',(#10779),#3508,.F.);
#43360=ADVANCED_FACE('',(#10780,#662),#1562,.T.);
#43361=ADVANCED_FACE('',(#10781),#3509,.F.);
#43362=ADVANCED_FACE('',(#10782,#663),#1563,.T.);
#43363=ADVANCED_FACE('',(#10783),#3510,.F.);
#43364=ADVANCED_FACE('',(#10784,#664),#3511,.T.);
#43365=ADVANCED_FACE('',(#10785),#3512,.F.);
#43366=ADVANCED_FACE('',(#10786,#665),#3513,.T.);
#43367=ADVANCED_FACE('',(#10787),#3514,.F.);
#43368=ADVANCED_FACE('',(#10788,#666),#1564,.T.);
#43369=ADVANCED_FACE('',(#10789),#3515,.F.);
#43370=ADVANCED_FACE('',(#10790,#667),#1565,.T.);
#43371=ADVANCED_FACE('',(#10791),#3516,.F.);
#43372=ADVANCED_FACE('',(#10792,#668),#3517,.T.);
#43373=ADVANCED_FACE('',(#10793),#3518,.F.);
#43374=ADVANCED_FACE('',(#10794,#669),#3519,.T.);
#43375=ADVANCED_FACE('',(#10795),#3520,.F.);
#43376=ADVANCED_FACE('',(#10796,#670),#1566,.T.);
#43377=ADVANCED_FACE('',(#10797),#3521,.F.);
#43378=ADVANCED_FACE('',(#10798,#671),#1567,.T.);
#43379=ADVANCED_FACE('',(#10799),#3522,.F.);
#43380=ADVANCED_FACE('',(#10800,#672),#1568,.T.);
#43381=ADVANCED_FACE('',(#10801),#3523,.F.);
#43382=ADVANCED_FACE('',(#10802,#673),#1569,.T.);
#43383=ADVANCED_FACE('',(#10803),#3524,.F.);
#43384=ADVANCED_FACE('',(#10804,#674),#1570,.T.);
#43385=ADVANCED_FACE('',(#10805),#3525,.F.);
#43386=ADVANCED_FACE('',(#10806,#675),#1571,.T.);
#43387=ADVANCED_FACE('',(#10807),#3526,.F.);
#43388=ADVANCED_FACE('',(#10808,#676),#1572,.T.);
#43389=ADVANCED_FACE('',(#10809),#3527,.F.);
#43390=ADVANCED_FACE('',(#10810,#677),#1573,.T.);
#43391=ADVANCED_FACE('',(#10811),#3528,.F.);
#43392=ADVANCED_FACE('',(#10812,#678),#1574,.T.);
#43393=ADVANCED_FACE('',(#10813),#3529,.F.);
#43394=ADVANCED_FACE('',(#10814,#679),#1575,.T.);
#43395=ADVANCED_FACE('',(#10815),#3530,.F.);
#43396=ADVANCED_FACE('',(#10816,#680),#1576,.T.);
#43397=ADVANCED_FACE('',(#10817),#3531,.F.);
#43398=ADVANCED_FACE('',(#10818,#681),#1577,.T.);
#43399=ADVANCED_FACE('',(#10819),#3532,.F.);
#43400=ADVANCED_FACE('',(#10820,#682),#1578,.T.);
#43401=ADVANCED_FACE('',(#10821),#3533,.F.);
#43402=ADVANCED_FACE('',(#10822,#683),#1579,.T.);
#43403=ADVANCED_FACE('',(#10823),#3534,.F.);
#43404=ADVANCED_FACE('',(#10824,#684),#1580,.T.);
#43405=ADVANCED_FACE('',(#10825),#3535,.F.);
#43406=ADVANCED_FACE('',(#10826,#685),#1581,.T.);
#43407=ADVANCED_FACE('',(#10827),#3536,.F.);
#43408=ADVANCED_FACE('',(#10828,#686),#1582,.T.);
#43409=ADVANCED_FACE('',(#10829),#3537,.F.);
#43410=ADVANCED_FACE('',(#10830,#687),#1583,.T.);
#43411=ADVANCED_FACE('',(#10831),#3538,.F.);
#43412=ADVANCED_FACE('',(#10832,#688),#1584,.T.);
#43413=ADVANCED_FACE('',(#10833),#3539,.F.);
#43414=ADVANCED_FACE('',(#10834,#689),#1585,.T.);
#43415=ADVANCED_FACE('',(#10835),#3540,.F.);
#43416=ADVANCED_FACE('',(#10836,#690),#1586,.T.);
#43417=ADVANCED_FACE('',(#10837),#3541,.F.);
#43418=ADVANCED_FACE('',(#10838,#691),#1587,.T.);
#43419=ADVANCED_FACE('',(#10839),#3542,.F.);
#43420=ADVANCED_FACE('',(#10840,#692),#1588,.T.);
#43421=ADVANCED_FACE('',(#10841),#3543,.F.);
#43422=ADVANCED_FACE('',(#10842,#693),#1589,.T.);
#43423=ADVANCED_FACE('',(#10843),#3544,.F.);
#43424=ADVANCED_FACE('',(#10844,#694),#1590,.T.);
#43425=ADVANCED_FACE('',(#10845),#3545,.F.);
#43426=ADVANCED_FACE('',(#10846,#695),#1591,.T.);
#43427=ADVANCED_FACE('',(#10847),#3546,.F.);
#43428=ADVANCED_FACE('',(#10848,#696),#1592,.T.);
#43429=ADVANCED_FACE('',(#10849),#3547,.F.);
#43430=ADVANCED_FACE('',(#10850,#697),#1593,.T.);
#43431=ADVANCED_FACE('',(#10851),#3548,.F.);
#43432=ADVANCED_FACE('',(#10852,#698),#1594,.T.);
#43433=ADVANCED_FACE('',(#10853),#3549,.F.);
#43434=ADVANCED_FACE('',(#10854,#699),#1595,.T.);
#43435=ADVANCED_FACE('',(#10855),#3550,.F.);
#43436=ADVANCED_FACE('',(#10856,#700),#1596,.T.);
#43437=ADVANCED_FACE('',(#10857),#3551,.F.);
#43438=ADVANCED_FACE('',(#10858,#701),#1597,.T.);
#43439=ADVANCED_FACE('',(#10859),#3552,.F.);
#43440=ADVANCED_FACE('',(#10860,#702),#1598,.T.);
#43441=ADVANCED_FACE('',(#10861),#3553,.F.);
#43442=ADVANCED_FACE('',(#10862,#703),#1599,.T.);
#43443=ADVANCED_FACE('',(#10863),#3554,.F.);
#43444=ADVANCED_FACE('',(#10864,#704),#1600,.T.);
#43445=ADVANCED_FACE('',(#10865),#3555,.F.);
#43446=ADVANCED_FACE('',(#10866,#705),#1601,.T.);
#43447=ADVANCED_FACE('',(#10867),#3556,.F.);
#43448=ADVANCED_FACE('',(#10868,#706),#1602,.T.);
#43449=ADVANCED_FACE('',(#10869),#3557,.F.);
#43450=ADVANCED_FACE('',(#10870,#707),#1603,.T.);
#43451=ADVANCED_FACE('',(#10871),#3558,.F.);
#43452=ADVANCED_FACE('',(#10872,#708),#1604,.T.);
#43453=ADVANCED_FACE('',(#10873,#709),#3559,.T.);
#43454=ADVANCED_FACE('',(#10874),#3560,.T.);
#43455=ADVANCED_FACE('',(#10875,#710),#3561,.T.);
#43456=ADVANCED_FACE('',(#10876),#3562,.T.);
#43457=ADVANCED_FACE('',(#10877,#711),#3563,.T.);
#43458=ADVANCED_FACE('',(#10878),#3564,.T.);
#43459=ADVANCED_FACE('',(#10879,#712),#3565,.T.);
#43460=ADVANCED_FACE('',(#10880),#3566,.T.);
#43461=ADVANCED_FACE('',(#10881,#713),#3567,.T.);
#43462=ADVANCED_FACE('',(#10882),#3568,.T.);
#43463=ADVANCED_FACE('',(#10883,#714),#3569,.T.);
#43464=ADVANCED_FACE('',(#10884),#3570,.T.);
#45449=CLOSED_SHELL('',(#42054,#42055,#42056,#42057,#42058));
#45450=CLOSED_SHELL('',(#42059,#42060,#42061,#42062,#42063));
#45451=CLOSED_SHELL('',(#42064,#42065,#42066,#42067,#42068,#42069,#42070,
#42071,#42072,#42073,#42074,#42075,#42076,#42077,#42078,#42079,#42080,#42081,
#42082,#42083,#42084,#42085,#42086,#42087,#42088,#42089,#42090,#42091,#42092,
#42093,#42094,#42095,#42096,#42097,#42098,#42099,#42100,#42101,#42102,#42103,
#42104,#42105,#42106,#42107,#42108,#42109,#42110,#42111,#42112,#42113,#42114,
#42115,#42116,#42117,#42118,#42119,#42120,#42121,#42122,#42123,#42124,#42125,
#42126,#42127,#42128,#42129,#42130,#42131,#42132,#42133,#42134,#42135,#42136,
#42137,#42138,#42139,#42140,#42141,#42142,#42143,#42144,#42145,#42146,#42147,
#42148,#42149,#42150,#42151,#42152,#42153,#42154,#42155,#42156,#42157,#42158,
#42159,#42160,#42161,#42162,#42163,#42164,#42165,#42166,#42167,#42168,#42169,
#42170,#42171,#42172,#42173,#42174,#42175,#42176,#42177,#42178,#42179,#42180,
#42181,#42182,#42183,#42184,#42185,#42186,#42187,#42188,#42189,#42190,#42191,
#42192,#42193,#42194,#42195,#42196,#42197,#42198,#42199,#42200,#42201,#42202,
#42203,#42204,#42205,#42206,#42207,#42208,#42209,#42210,#42211,#42212,#42213,
#42214,#42215,#42216,#42217,#42218,#42219,#42220,#42221,#42222,#42223,#42224,
#42225,#42226,#42227,#42228,#42229,#42230,#42231,#42232,#42233,#42234,#42235,
#42236,#42237,#42238,#42239,#42240,#42241,#42242,#42243,#42244,#42245,#42246,
#42247,#42248,#42249,#42250,#42251,#42252,#42253,#42254,#42255,#42256,#42257,
#42258,#42259,#42260,#42261,#42262,#42263,#42264,#42265,#42266,#42267,#42268,
#42269,#42270,#42271,#42272,#42273,#42274,#42275,#42276,#42277,#42278,#42279,
#42280,#42281,#42282,#42283,#42284,#42285,#42286,#42287,#42288,#42289,#42290,
#42291,#42292,#42293,#42294,#42295,#42296,#42297,#42298,#42299,#42300,#42301,
#42302,#42303,#42304,#42305,#42306,#42307,#42308,#42309,#42310,#42311,#42312,
#42313,#42314,#42315,#42316,#42317,#42318,#42319,#42320,#42321,#42322,#42323,
#42324,#42325,#42326,#42327,#42328,#42329,#42330,#42331,#42332,#42333,#42334,
#42335,#42336,#42337,#42338,#42339,#42340,#42341,#42342,#42343,#42344,#42345,
#42346,#42347,#42348,#42349,#42350,#42351,#42352,#42353,#42354,#42355,#42356,
#42357,#42358,#42359,#42360,#42361,#42362,#42363,#42364,#42365,#42366,#42367,
#42368,#42369,#42370,#42371,#42372,#42373,#42374,#42375,#42376,#42377,#42378,
#42379,#42380,#42381,#42382,#42383,#42384,#42385,#42386,#42387,#42388,#42389,
#42390,#42391,#42392,#42393,#42394,#42395,#42396,#42397,#42398,#42399,#42400,
#42401,#42402,#42403,#42404,#42405,#42406,#42407,#42408,#42409,#42410,#42411,
#42412,#42413,#42414,#42415,#42416,#42417,#42418,#42419,#42420,#42421,#42422,
#42423,#42424,#42425,#42426,#42427,#42428,#42429,#42430,#42431,#42432,#42433,
#42434,#42435,#42436,#42437,#42438,#42439,#42440,#42441,#42442,#42443,#42444,
#42445,#42446,#42447,#42448,#42449,#42450,#42451,#42452,#42453,#42454,#42455,
#42456,#42457,#42458,#42459,#42460,#42461,#42462,#42463,#42464,#42465,#42466,
#42467,#42468,#42469,#42470,#42471,#42472,#42473,#42474,#42475,#42476,#42477,
#42478,#42479,#42480,#42481,#42482,#42483,#42484,#42485,#42486,#42487,#42488,
#42489,#42490,#42491,#42492,#42493,#42494,#42495,#42496,#42497,#42498,#42499,
#42500,#42501,#42502,#42503,#42504,#42505,#42506,#42507,#42508,#42509,#42510,
#42511,#42512,#42513,#42514,#42515,#42516,#42517,#42518,#42519,#42520,#42521,
#42522,#42523,#42524,#42525,#42526,#42527,#42528,#42529,#42530,#42531,#42532,
#42533,#42534,#42535,#42536,#42537,#42538,#42539,#42540,#42541,#42542,#42543,
#42544,#42545,#42546,#42547,#42548,#42549,#42550,#42551,#42552,#42553,#42554,
#42555,#42556,#42557,#42558,#42559,#42560,#42561,#42562,#42563,#42564,#42565,
#42566,#42567,#42568,#42569,#42570,#42571,#42572,#42573,#42574,#42575,#42576,
#42577,#42578,#42579,#42580,#42581,#42582,#42583,#42584,#42585,#42586,#42587,
#42588,#42589,#42590,#42591,#42592,#42593,#42594,#42595,#42596,#42597,#42598,
#42599,#42600,#42601,#42602,#42603,#42604,#42605,#42606,#42607,#42608,#42609,
#42610,#42611,#42612,#42613,#42614,#42615,#42616,#42617,#42618,#42619,#42620,
#42621,#42622,#42623,#42624,#42625,#42626,#42627,#42628,#42629,#42630,#42631,
#42632,#42633,#42634,#42635,#42636,#42637,#42638,#42639,#42640,#42641,#42642,
#42643,#42644,#42645,#42646,#42647,#42648,#42649,#42650,#42651,#42652,#42653,
#42654,#42655,#42656,#42657,#42658,#42659,#42660,#42661,#42662,#42663,#42664,
#42665,#42666,#42667,#42668,#42669,#42670,#42671,#42672,#42673,#42674,#42675,
#42676,#42677,#42678,#42679,#42680,#42681,#42682,#42683,#42684,#42685,#42686,
#42687,#42688,#42689,#42690,#42691,#42692,#42693,#42694,#42695,#42696,#42697,
#42698,#42699,#42700,#42701,#42702,#42703,#42704,#42705,#42706,#42707,#42708,
#42709,#42710,#42711,#42712,#42713,#42714,#42715,#42716,#42717,#42718,#42719,
#42720,#42721,#42722,#42723,#42724,#42725,#42726,#42727,#42728,#42729,#42730,
#42731,#42732,#42733,#42734,#42735,#42736,#42737,#42738,#42739,#42740,#42741,
#42742,#42743,#42744,#42745,#42746,#42747,#42748,#42749,#42750,#42751,#42752,
#42753,#42754,#42755,#42756,#42757,#42758,#42759,#42760,#42761,#42762,#42763,
#42764,#42765,#42766,#42767,#42768,#42769,#42770,#42771,#42772,#42773,#42774,
#42775,#42776,#42777,#42778,#42779,#42780,#42781,#42782,#42783,#42784,#42785,
#42786,#42787,#42788,#42789,#42790,#42791,#42792,#42793,#42794,#42795,#42796,
#42797,#42798,#42799,#42800,#42801,#42802,#42803,#42804,#42805,#42806,#42807,
#42808,#42809,#42810,#42811,#42812,#42813,#42814,#42815,#42816,#42817,#42818,
#42819,#42820,#42821,#42822,#42823,#42824,#42825,#42826,#42827,#42828,#42829,
#42830,#42831,#42832,#42833,#42834,#42835,#42836,#42837,#42838,#42839,#42840,
#42841,#42842,#42843,#42844,#42845,#42846,#42847,#42848,#42849,#42850,#42851,
#42852,#42853,#42854,#42855,#42856,#42857,#42858,#42859,#42860,#42861,#42862,
#42863,#42864,#42865,#42866,#42867,#42868,#42869,#42870,#42871,#42872,#42873,
#42874,#42875,#42876,#42877,#42878,#42879,#42880,#42881,#42882,#42883,#42884,
#42885,#42886,#42887,#42888,#42889,#42890,#42891,#42892,#42893,#42894,#42895,
#42896,#42897,#42898,#42899,#42900,#42901,#42902,#42903,#42904,#42905,#42906,
#42907,#42908,#42909,#42910,#42911,#42912,#42913,#42914,#42915,#42916,#42917,
#42918,#42919,#42920,#42921,#42922,#42923,#42924,#42925,#42926,#42927,#42928,
#42929,#42930,#42931,#42932,#42933,#42934,#42935,#42936,#42937,#42938,#42939,
#42940,#42941,#42942,#42943,#42944,#42945,#42946,#42947,#42948,#42949,#42950,
#42951,#42952,#42953,#42954,#42955,#42956,#42957,#42958,#42959,#42960,#42961,
#42962,#42963,#42964,#42965,#42966,#42967,#42968,#42969,#42970,#42971,#42972,
#42973,#42974,#42975,#42976,#42977,#42978,#42979,#42980,#42981,#42982,#42983,
#42984,#42985,#42986,#42987,#42988,#42989,#42990,#42991,#42992,#42993,#42994,
#42995,#42996,#42997,#42998,#42999,#43000,#43001,#43002,#43003,#43004,#43005,
#43006,#43007,#43008,#43009,#43010,#43011,#43012,#43013,#43014,#43015,#43016,
#43017,#43018,#43019,#43020,#43021,#43022,#43023,#43024,#43025,#43026,#43027,
#43028,#43029,#43030,#43031,#43032,#43033,#43034,#43035,#43036,#43037,#43038,
#43039,#43040,#43041,#43042,#43043,#43044,#43045,#43046,#43047,#43048,#43049,
#43050,#43051,#43052,#43053,#43054,#43055,#43056,#43057,#43058,#43059,#43060,
#43061,#43062,#43063,#43064,#43065,#43066,#43067,#43068,#43069,#43070,#43071,
#43072,#43073,#43074,#43075,#43076,#43077,#43078,#43079,#43080,#43081,#43082,
#43083,#43084,#43085,#43086,#43087,#43088,#43089,#43090,#43091,#43092,#43093,
#43094,#43095,#43096,#43097,#43098,#43099,#43100,#43101,#43102,#43103,#43104,
#43105,#43106,#43107,#43108,#43109,#43110,#43111,#43112,#43113,#43114,#43115,
#43116,#43117,#43118,#43119,#43120,#43121,#43122,#43123,#43124,#43125,#43126,
#43127,#43128,#43129,#43130,#43131,#43132,#43133,#43134,#43135,#43136,#43137,
#43138,#43139,#43140,#43141,#43142,#43143,#43144,#43145,#43146,#43147,#43148,
#43149,#43150,#43151,#43152,#43153,#43154,#43155,#43156,#43157,#43158,#43159,
#43160,#43161,#43162,#43163,#43164,#43165,#43166,#43167,#43168,#43169,#43170,
#43171,#43172,#43173,#43174,#43175,#43176,#43177,#43178,#43179,#43180,#43181,
#43182,#43183,#43184,#43185,#43186,#43187,#43188,#43189,#43190,#43191,#43192,
#43193,#43194,#43195,#43196,#43197,#43198,#43199,#43200,#43201,#43202,#43203,
#43204,#43205,#43206,#43207,#43208,#43209,#43210,#43211,#43212,#43213,#43214,
#43215,#43216,#43217,#43218,#43219,#43220,#43221,#43222,#43223,#43224,#43225,
#43226,#43227,#43228,#43229,#43230,#43231,#43232,#43233,#43234,#43235,#43236,
#43237,#43238,#43239,#43240,#43241,#43242,#43243,#43244,#43245,#43246,#43247,
#43248,#43249,#43250,#43251,#43252,#43253,#43254,#43255,#43256,#43257,#43258,
#43259,#43260,#43261,#43262,#43263,#43264,#43265,#43266,#43267,#43268,#43269,
#43270,#43271,#43272,#43273,#43274,#43275,#43276,#43277,#43278,#43279,#43280,
#43281,#43282,#43283,#43284,#43285,#43286,#43287,#43288,#43289,#43290,#43291,
#43292,#43293,#43294,#43295,#43296,#43297,#43298,#43299,#43300,#43301,#43302,
#43303,#43304,#43305,#43306,#43307,#43308,#43309,#43310,#43311,#43312,#43313,
#43314,#43315,#43316,#43317,#43318,#43319,#43320,#43321,#43322,#43323,#43324,
#43325,#43326,#43327,#43328,#43329,#43330,#43331,#43332,#43333,#43334,#43335,
#43336,#43337,#43338,#43339,#43340,#43341,#43342,#43343,#43344,#43345,#43346,
#43347,#43348,#43349,#43350,#43351,#43352,#43353,#43354,#43355,#43356,#43357,
#43358,#43359,#43360,#43361,#43362,#43363,#43364,#43365,#43366,#43367,#43368,
#43369,#43370,#43371,#43372,#43373,#43374,#43375,#43376,#43377,#43378,#43379,
#43380,#43381,#43382,#43383,#43384,#43385,#43386,#43387,#43388,#43389,#43390,
#43391,#43392,#43393,#43394,#43395,#43396,#43397,#43398,#43399,#43400,#43401,
#43402,#43403,#43404,#43405,#43406,#43407,#43408,#43409,#43410,#43411,#43412,
#43413,#43414,#43415,#43416,#43417,#43418,#43419,#43420,#43421,#43422,#43423,
#43424,#43425,#43426,#43427,#43428,#43429,#43430,#43431,#43432,#43433,#43434,
#43435,#43436,#43437,#43438,#43439,#43440,#43441,#43442,#43443,#43444,#43445,
#43446,#43447,#43448,#43449,#43450,#43451,#43452,#43453,#43454,#43455,#43456,
#43457,#43458,#43459,#43460,#43461,#43462,#43463,#43464));
#45568=AXIS2_PLACEMENT_3D('',#65509,#51642,#51643);
#45569=AXIS2_PLACEMENT_3D('',#65510,#51644,#51645);
#45570=AXIS2_PLACEMENT_3D('',#65515,#51647,#51648);
#45571=AXIS2_PLACEMENT_3D('',#65519,#51651,#51652);
#45572=AXIS2_PLACEMENT_3D('',#65523,#51654,#51655);
#45573=AXIS2_PLACEMENT_3D('',#65525,#51657,#51658);
#45574=AXIS2_PLACEMENT_3D('',#65528,#51661,#51662);
#45575=AXIS2_PLACEMENT_3D('',#65529,#51663,#51664);
#45576=AXIS2_PLACEMENT_3D('',#65530,#51665,#51666);
#45577=AXIS2_PLACEMENT_3D('',#65535,#51668,#51669);
#45578=AXIS2_PLACEMENT_3D('',#65538,#51671,#51672);
#45579=AXIS2_PLACEMENT_3D('',#65539,#51673,#51674);
#45580=AXIS2_PLACEMENT_3D('',#65543,#51677,#51678);
#45581=AXIS2_PLACEMENT_3D('',#65547,#51681,#51682);
#45582=AXIS2_PLACEMENT_3D('',#65548,#51683,#51684);
#45583=AXIS2_PLACEMENT_3D('',#65549,#51685,#51686);
#45584=AXIS2_PLACEMENT_3D('',#65550,#51687,#51688);
#45585=AXIS2_PLACEMENT_3D('',#65552,#51689,#51690);
#45586=AXIS2_PLACEMENT_3D('',#65555,#51692,#51693);
#45587=AXIS2_PLACEMENT_3D('',#65556,#51694,#51695);
#45588=AXIS2_PLACEMENT_3D('',#65558,#51696,#51697);
#45589=AXIS2_PLACEMENT_3D('',#65561,#51699,#51700);
#45590=AXIS2_PLACEMENT_3D('',#65562,#51701,#51702);
#45591=AXIS2_PLACEMENT_3D('',#65564,#51703,#51704);
#45592=AXIS2_PLACEMENT_3D('',#65567,#51706,#51707);
#45593=AXIS2_PLACEMENT_3D('',#65568,#51708,#51709);
#45594=AXIS2_PLACEMENT_3D('',#65570,#51710,#51711);
#45595=AXIS2_PLACEMENT_3D('',#65573,#51713,#51714);
#45596=AXIS2_PLACEMENT_3D('',#65574,#51715,#51716);
#45597=AXIS2_PLACEMENT_3D('',#65576,#51717,#51718);
#45598=AXIS2_PLACEMENT_3D('',#65579,#51720,#51721);
#45599=AXIS2_PLACEMENT_3D('',#65580,#51722,#51723);
#45600=AXIS2_PLACEMENT_3D('',#65582,#51724,#51725);
#45601=AXIS2_PLACEMENT_3D('',#65585,#51727,#51728);
#45602=AXIS2_PLACEMENT_3D('',#65586,#51729,#51730);
#45603=AXIS2_PLACEMENT_3D('',#65588,#51731,#51732);
#45604=AXIS2_PLACEMENT_3D('',#65591,#51734,#51735);
#45605=AXIS2_PLACEMENT_3D('',#65592,#51736,#51737);
#45606=AXIS2_PLACEMENT_3D('',#65594,#51738,#51739);
#45607=AXIS2_PLACEMENT_3D('',#65597,#51741,#51742);
#45608=AXIS2_PLACEMENT_3D('',#65598,#51743,#51744);
#45609=AXIS2_PLACEMENT_3D('',#65600,#51745,#51746);
#45610=AXIS2_PLACEMENT_3D('',#65603,#51748,#51749);
#45611=AXIS2_PLACEMENT_3D('',#65604,#51750,#51751);
#45612=AXIS2_PLACEMENT_3D('',#65606,#51752,#51753);
#45613=AXIS2_PLACEMENT_3D('',#65609,#51755,#51756);
#45614=AXIS2_PLACEMENT_3D('',#65610,#51757,#51758);
#45615=AXIS2_PLACEMENT_3D('',#65612,#51759,#51760);
#45616=AXIS2_PLACEMENT_3D('',#65615,#51762,#51763);
#45617=AXIS2_PLACEMENT_3D('',#65616,#51764,#51765);
#45618=AXIS2_PLACEMENT_3D('',#65618,#51766,#51767);
#45619=AXIS2_PLACEMENT_3D('',#65621,#51769,#51770);
#45620=AXIS2_PLACEMENT_3D('',#65622,#51771,#51772);
#45621=AXIS2_PLACEMENT_3D('',#65704,#51774,#51775);
#45622=AXIS2_PLACEMENT_3D('',#65706,#51776,#51777);
#45623=AXIS2_PLACEMENT_3D('',#65743,#51779,#51780);
#45624=AXIS2_PLACEMENT_3D('',#65825,#51782,#51783);
#45625=AXIS2_PLACEMENT_3D('',#65827,#51784,#51785);
#45626=AXIS2_PLACEMENT_3D('',#65864,#51787,#51788);
#45627=AXIS2_PLACEMENT_3D('',#65946,#51790,#51791);
#45628=AXIS2_PLACEMENT_3D('',#65948,#51792,#51793);
#45629=AXIS2_PLACEMENT_3D('',#65985,#51795,#51796);
#45630=AXIS2_PLACEMENT_3D('',#66067,#51798,#51799);
#45631=AXIS2_PLACEMENT_3D('',#66069,#51800,#51801);
#45632=AXIS2_PLACEMENT_3D('',#66106,#51803,#51804);
#45633=AXIS2_PLACEMENT_3D('',#66188,#51806,#51807);
#45634=AXIS2_PLACEMENT_3D('',#66190,#51808,#51809);
#45635=AXIS2_PLACEMENT_3D('',#66227,#51811,#51812);
#45636=AXIS2_PLACEMENT_3D('',#66309,#51814,#51815);
#45637=AXIS2_PLACEMENT_3D('',#66311,#51816,#51817);
#45638=AXIS2_PLACEMENT_3D('',#66348,#51819,#51820);
#45639=AXIS2_PLACEMENT_3D('',#66430,#51822,#51823);
#45640=AXIS2_PLACEMENT_3D('',#66432,#51824,#51825);
#45641=AXIS2_PLACEMENT_3D('',#66469,#51827,#51828);
#45642=AXIS2_PLACEMENT_3D('',#66551,#51830,#51831);
#45643=AXIS2_PLACEMENT_3D('',#66553,#51832,#51833);
#45644=AXIS2_PLACEMENT_3D('',#66590,#51835,#51836);
#45645=AXIS2_PLACEMENT_3D('',#66672,#51838,#51839);
#45646=AXIS2_PLACEMENT_3D('',#66674,#51840,#51841);
#45647=AXIS2_PLACEMENT_3D('',#66711,#51843,#51844);
#45648=AXIS2_PLACEMENT_3D('',#66793,#51846,#51847);
#45649=AXIS2_PLACEMENT_3D('',#66795,#51848,#51849);
#45650=AXIS2_PLACEMENT_3D('',#66832,#51851,#51852);
#45651=AXIS2_PLACEMENT_3D('',#66914,#51854,#51855);
#45652=AXIS2_PLACEMENT_3D('',#66916,#51856,#51857);
#45653=AXIS2_PLACEMENT_3D('',#66953,#51859,#51860);
#45654=AXIS2_PLACEMENT_3D('',#67035,#51862,#51863);
#45655=AXIS2_PLACEMENT_3D('',#67037,#51864,#51865);
#45656=AXIS2_PLACEMENT_3D('',#67074,#51867,#51868);
#45657=AXIS2_PLACEMENT_3D('',#67156,#51870,#51871);
#45658=AXIS2_PLACEMENT_3D('',#67158,#51872,#51873);
#45659=AXIS2_PLACEMENT_3D('',#67195,#51875,#51876);
#45660=AXIS2_PLACEMENT_3D('',#67277,#51878,#51879);
#45661=AXIS2_PLACEMENT_3D('',#67279,#51880,#51881);
#45662=AXIS2_PLACEMENT_3D('',#67316,#51883,#51884);
#45663=AXIS2_PLACEMENT_3D('',#67398,#51886,#51887);
#45664=AXIS2_PLACEMENT_3D('',#67400,#51888,#51889);
#45665=AXIS2_PLACEMENT_3D('',#67437,#51891,#51892);
#45666=AXIS2_PLACEMENT_3D('',#67519,#51894,#51895);
#45667=AXIS2_PLACEMENT_3D('',#67521,#51896,#51897);
#45668=AXIS2_PLACEMENT_3D('',#67558,#51899,#51900);
#45669=AXIS2_PLACEMENT_3D('',#67640,#51902,#51903);
#45670=AXIS2_PLACEMENT_3D('',#67642,#51904,#51905);
#45671=AXIS2_PLACEMENT_3D('',#67679,#51907,#51908);
#45672=AXIS2_PLACEMENT_3D('',#67761,#51910,#51911);
#45673=AXIS2_PLACEMENT_3D('',#67763,#51912,#51913);
#45674=AXIS2_PLACEMENT_3D('',#67800,#51915,#51916);
#45675=AXIS2_PLACEMENT_3D('',#67882,#51918,#51919);
#45676=AXIS2_PLACEMENT_3D('',#67884,#51920,#51921);
#45677=AXIS2_PLACEMENT_3D('',#67921,#51923,#51924);
#45678=AXIS2_PLACEMENT_3D('',#68003,#51926,#51927);
#45679=AXIS2_PLACEMENT_3D('',#68005,#51928,#51929);
#45680=AXIS2_PLACEMENT_3D('',#68042,#51931,#51932);
#45681=AXIS2_PLACEMENT_3D('',#68124,#51934,#51935);
#45682=AXIS2_PLACEMENT_3D('',#68126,#51936,#51937);
#45683=AXIS2_PLACEMENT_3D('',#68163,#51939,#51940);
#45684=AXIS2_PLACEMENT_3D('',#68245,#51942,#51943);
#45685=AXIS2_PLACEMENT_3D('',#68247,#51944,#51945);
#45686=AXIS2_PLACEMENT_3D('',#68284,#51947,#51948);
#45687=AXIS2_PLACEMENT_3D('',#68366,#51950,#51951);
#45688=AXIS2_PLACEMENT_3D('',#68368,#51952,#51953);
#45689=AXIS2_PLACEMENT_3D('',#68405,#51955,#51956);
#45690=AXIS2_PLACEMENT_3D('',#68487,#51958,#51959);
#45691=AXIS2_PLACEMENT_3D('',#68489,#51960,#51961);
#45692=AXIS2_PLACEMENT_3D('',#68526,#51963,#51964);
#45693=AXIS2_PLACEMENT_3D('',#68608,#51966,#51967);
#45694=AXIS2_PLACEMENT_3D('',#68610,#51968,#51969);
#45695=AXIS2_PLACEMENT_3D('',#68647,#51971,#51972);
#45696=AXIS2_PLACEMENT_3D('',#68729,#51974,#51975);
#45697=AXIS2_PLACEMENT_3D('',#68731,#51976,#51977);
#45698=AXIS2_PLACEMENT_3D('',#68768,#51979,#51980);
#45699=AXIS2_PLACEMENT_3D('',#68850,#51982,#51983);
#45700=AXIS2_PLACEMENT_3D('',#68852,#51984,#51985);
#45701=AXIS2_PLACEMENT_3D('',#68889,#51987,#51988);
#45702=AXIS2_PLACEMENT_3D('',#68971,#51990,#51991);
#45703=AXIS2_PLACEMENT_3D('',#68973,#51992,#51993);
#45704=AXIS2_PLACEMENT_3D('',#69010,#51995,#51996);
#45705=AXIS2_PLACEMENT_3D('',#69092,#51998,#51999);
#45706=AXIS2_PLACEMENT_3D('',#69094,#52000,#52001);
#45707=AXIS2_PLACEMENT_3D('',#69131,#52003,#52004);
#45708=AXIS2_PLACEMENT_3D('',#69213,#52006,#52007);
#45709=AXIS2_PLACEMENT_3D('',#69215,#52008,#52009);
#45710=AXIS2_PLACEMENT_3D('',#69252,#52011,#52012);
#45711=AXIS2_PLACEMENT_3D('',#69334,#52014,#52015);
#45712=AXIS2_PLACEMENT_3D('',#69336,#52016,#52017);
#45713=AXIS2_PLACEMENT_3D('',#69373,#52019,#52020);
#45714=AXIS2_PLACEMENT_3D('',#69455,#52022,#52023);
#45715=AXIS2_PLACEMENT_3D('',#69457,#52024,#52025);
#45716=AXIS2_PLACEMENT_3D('',#69494,#52027,#52028);
#45717=AXIS2_PLACEMENT_3D('',#69578,#52030,#52031);
#45718=AXIS2_PLACEMENT_3D('',#69580,#52032,#52033);
#45719=AXIS2_PLACEMENT_3D('',#69617,#52035,#52036);
#45720=AXIS2_PLACEMENT_3D('',#69699,#52038,#52039);
#45721=AXIS2_PLACEMENT_3D('',#69701,#52040,#52041);
#45722=AXIS2_PLACEMENT_3D('',#69738,#52043,#52044);
#45723=AXIS2_PLACEMENT_3D('',#69820,#52046,#52047);
#45724=AXIS2_PLACEMENT_3D('',#69822,#52048,#52049);
#45725=AXIS2_PLACEMENT_3D('',#69859,#52051,#52052);
#45726=AXIS2_PLACEMENT_3D('',#69941,#52054,#52055);
#45727=AXIS2_PLACEMENT_3D('',#69943,#52056,#52057);
#45728=AXIS2_PLACEMENT_3D('',#69980,#52059,#52060);
#45729=AXIS2_PLACEMENT_3D('',#70062,#52062,#52063);
#45730=AXIS2_PLACEMENT_3D('',#70064,#52064,#52065);
#45731=AXIS2_PLACEMENT_3D('',#70101,#52067,#52068);
#45732=AXIS2_PLACEMENT_3D('',#70195,#52070,#52071);
#45733=AXIS2_PLACEMENT_3D('',#70197,#52072,#52073);
#45734=AXIS2_PLACEMENT_3D('',#70234,#52075,#52076);
#45735=AXIS2_PLACEMENT_3D('',#70316,#52078,#52079);
#45736=AXIS2_PLACEMENT_3D('',#70318,#52080,#52081);
#45737=AXIS2_PLACEMENT_3D('',#70355,#52083,#52084);
#45738=AXIS2_PLACEMENT_3D('',#70357,#52085,#52086);
#45739=AXIS2_PLACEMENT_3D('',#70404,#52088,#52089);
#45740=AXIS2_PLACEMENT_3D('',#70406,#52090,#52091);
#45741=AXIS2_PLACEMENT_3D('',#70409,#52093,#52094);
#45742=AXIS2_PLACEMENT_3D('',#70410,#52095,#52096);
#45743=AXIS2_PLACEMENT_3D('',#70412,#52097,#52098);
#45744=AXIS2_PLACEMENT_3D('',#70461,#52100,#52101);
#45745=AXIS2_PLACEMENT_3D('',#70463,#52102,#52103);
#45746=AXIS2_PLACEMENT_3D('',#70466,#52105,#52106);
#45747=AXIS2_PLACEMENT_3D('',#70467,#52107,#52108);
#45748=AXIS2_PLACEMENT_3D('',#70565,#52110,#52111);
#45749=AXIS2_PLACEMENT_3D('',#70567,#52112,#52113);
#45750=AXIS2_PLACEMENT_3D('',#70604,#52115,#52116);
#45751=AXIS2_PLACEMENT_3D('',#70704,#52118,#52119);
#45752=AXIS2_PLACEMENT_3D('',#70706,#52120,#52121);
#45753=AXIS2_PLACEMENT_3D('',#70743,#52123,#52124);
#45754=AXIS2_PLACEMENT_3D('',#70745,#52125,#52126);
#45755=AXIS2_PLACEMENT_3D('',#70796,#52128,#52129);
#45756=AXIS2_PLACEMENT_3D('',#70798,#52130,#52131);
#45757=AXIS2_PLACEMENT_3D('',#70801,#52133,#52134);
#45758=AXIS2_PLACEMENT_3D('',#70802,#52135,#52136);
#45759=AXIS2_PLACEMENT_3D('',#70804,#52137,#52138);
#45760=AXIS2_PLACEMENT_3D('',#70853,#52140,#52141);
#45761=AXIS2_PLACEMENT_3D('',#70855,#52142,#52143);
#45762=AXIS2_PLACEMENT_3D('',#70858,#52145,#52146);
#45763=AXIS2_PLACEMENT_3D('',#70859,#52147,#52148);
#45764=AXIS2_PLACEMENT_3D('',#70951,#52150,#52151);
#45765=AXIS2_PLACEMENT_3D('',#70953,#52152,#52153);
#45766=AXIS2_PLACEMENT_3D('',#70990,#52155,#52156);
#45767=AXIS2_PLACEMENT_3D('',#71086,#52158,#52159);
#45768=AXIS2_PLACEMENT_3D('',#71088,#52160,#52161);
#45769=AXIS2_PLACEMENT_3D('',#71125,#52163,#52164);
#45770=AXIS2_PLACEMENT_3D('',#71127,#52165,#52166);
#45771=AXIS2_PLACEMENT_3D('',#71178,#52168,#52169);
#45772=AXIS2_PLACEMENT_3D('',#71180,#52170,#52171);
#45773=AXIS2_PLACEMENT_3D('',#71183,#52173,#52174);
#45774=AXIS2_PLACEMENT_3D('',#71184,#52175,#52176);
#45775=AXIS2_PLACEMENT_3D('',#71276,#52178,#52179);
#45776=AXIS2_PLACEMENT_3D('',#71278,#52180,#52181);
#45777=AXIS2_PLACEMENT_3D('',#71315,#52183,#52184);
#45778=AXIS2_PLACEMENT_3D('',#71405,#52186,#52187);
#45779=AXIS2_PLACEMENT_3D('',#71407,#52188,#52189);
#45780=AXIS2_PLACEMENT_3D('',#71444,#52191,#52192);
#45781=AXIS2_PLACEMENT_3D('',#71446,#52193,#52194);
#45782=AXIS2_PLACEMENT_3D('',#71499,#52196,#52197);
#45783=AXIS2_PLACEMENT_3D('',#71501,#52198,#52199);
#45784=AXIS2_PLACEMENT_3D('',#71504,#52201,#52202);
#45785=AXIS2_PLACEMENT_3D('',#71505,#52203,#52204);
#45786=AXIS2_PLACEMENT_3D('',#71599,#52206,#52207);
#45787=AXIS2_PLACEMENT_3D('',#71601,#52208,#52209);
#45788=AXIS2_PLACEMENT_3D('',#71638,#52211,#52212);
#45789=AXIS2_PLACEMENT_3D('',#71730,#52214,#52215);
#45790=AXIS2_PLACEMENT_3D('',#71732,#52216,#52217);
#45791=AXIS2_PLACEMENT_3D('',#71769,#52219,#52220);
#45792=AXIS2_PLACEMENT_3D('',#71867,#52222,#52223);
#45793=AXIS2_PLACEMENT_3D('',#71869,#52224,#52225);
#45794=AXIS2_PLACEMENT_3D('',#71906,#52227,#52228);
#45795=AXIS2_PLACEMENT_3D('',#72008,#52230,#52231);
#45796=AXIS2_PLACEMENT_3D('',#72010,#52232,#52233);
#45797=AXIS2_PLACEMENT_3D('',#72047,#52235,#52236);
#45798=AXIS2_PLACEMENT_3D('',#72129,#52238,#52239);
#45799=AXIS2_PLACEMENT_3D('',#72131,#52240,#52241);
#45800=AXIS2_PLACEMENT_3D('',#72168,#52243,#52244);
#45801=AXIS2_PLACEMENT_3D('',#72264,#52246,#52247);
#45802=AXIS2_PLACEMENT_3D('',#72266,#52248,#52249);
#45803=AXIS2_PLACEMENT_3D('',#72303,#52251,#52252);
#45804=AXIS2_PLACEMENT_3D('',#72385,#52254,#52255);
#45805=AXIS2_PLACEMENT_3D('',#72387,#52256,#52257);
#45806=AXIS2_PLACEMENT_3D('',#72424,#52259,#52260);
#45807=AXIS2_PLACEMENT_3D('',#72506,#52262,#52263);
#45808=AXIS2_PLACEMENT_3D('',#72508,#52264,#52265);
#45809=AXIS2_PLACEMENT_3D('',#72545,#52267,#52268);
#45810=AXIS2_PLACEMENT_3D('',#72627,#52270,#52271);
#45811=AXIS2_PLACEMENT_3D('',#72629,#52272,#52273);
#45812=AXIS2_PLACEMENT_3D('',#72666,#52275,#52276);
#45813=AXIS2_PLACEMENT_3D('',#72748,#52278,#52279);
#45814=AXIS2_PLACEMENT_3D('',#72750,#52280,#52281);
#45815=AXIS2_PLACEMENT_3D('',#72787,#52283,#52284);
#45816=AXIS2_PLACEMENT_3D('',#72869,#52286,#52287);
#45817=AXIS2_PLACEMENT_3D('',#72871,#52288,#52289);
#45818=AXIS2_PLACEMENT_3D('',#72908,#52291,#52292);
#45819=AXIS2_PLACEMENT_3D('',#72990,#52294,#52295);
#45820=AXIS2_PLACEMENT_3D('',#72992,#52296,#52297);
#45821=AXIS2_PLACEMENT_3D('',#73029,#52299,#52300);
#45822=AXIS2_PLACEMENT_3D('',#73113,#52302,#52303);
#45823=AXIS2_PLACEMENT_3D('',#73115,#52304,#52305);
#45824=AXIS2_PLACEMENT_3D('',#73152,#52307,#52308);
#45825=AXIS2_PLACEMENT_3D('',#73234,#52310,#52311);
#45826=AXIS2_PLACEMENT_3D('',#73236,#52312,#52313);
#45827=AXIS2_PLACEMENT_3D('',#73273,#52315,#52316);
#45828=AXIS2_PLACEMENT_3D('',#73275,#52317,#52318);
#45829=AXIS2_PLACEMENT_3D('',#73278,#52320,#52321);
#45830=AXIS2_PLACEMENT_3D('',#73279,#52322,#52323);
#45831=AXIS2_PLACEMENT_3D('',#73281,#52324,#52325);
#45832=AXIS2_PLACEMENT_3D('',#73284,#52327,#52328);
#45833=AXIS2_PLACEMENT_3D('',#73285,#52329,#52330);
#45834=AXIS2_PLACEMENT_3D('',#73287,#52331,#52332);
#45835=AXIS2_PLACEMENT_3D('',#73290,#52334,#52335);
#45836=AXIS2_PLACEMENT_3D('',#73291,#52336,#52337);
#45837=AXIS2_PLACEMENT_3D('',#73293,#52338,#52339);
#45838=AXIS2_PLACEMENT_3D('',#73296,#52341,#52342);
#45839=AXIS2_PLACEMENT_3D('',#73297,#52343,#52344);
#45840=AXIS2_PLACEMENT_3D('',#73299,#52345,#52346);
#45841=AXIS2_PLACEMENT_3D('',#73302,#52348,#52349);
#45842=AXIS2_PLACEMENT_3D('',#73303,#52350,#52351);
#45843=AXIS2_PLACEMENT_3D('',#73305,#52352,#52353);
#45844=AXIS2_PLACEMENT_3D('',#73308,#52355,#52356);
#45845=AXIS2_PLACEMENT_3D('',#73309,#52357,#52358);
#45846=AXIS2_PLACEMENT_3D('',#73311,#52359,#52360);
#45847=AXIS2_PLACEMENT_3D('',#73314,#52362,#52363);
#45848=AXIS2_PLACEMENT_3D('',#73315,#52364,#52365);
#45849=AXIS2_PLACEMENT_3D('',#73317,#52366,#52367);
#45850=AXIS2_PLACEMENT_3D('',#73320,#52369,#52370);
#45851=AXIS2_PLACEMENT_3D('',#73321,#52371,#52372);
#45852=AXIS2_PLACEMENT_3D('',#73323,#52373,#52374);
#45853=AXIS2_PLACEMENT_3D('',#73326,#52376,#52377);
#45854=AXIS2_PLACEMENT_3D('',#73327,#52378,#52379);
#45855=AXIS2_PLACEMENT_3D('',#73329,#52380,#52381);
#45856=AXIS2_PLACEMENT_3D('',#73332,#52383,#52384);
#45857=AXIS2_PLACEMENT_3D('',#73333,#52385,#52386);
#45858=AXIS2_PLACEMENT_3D('',#73335,#52387,#52388);
#45859=AXIS2_PLACEMENT_3D('',#73338,#52390,#52391);
#45860=AXIS2_PLACEMENT_3D('',#73339,#52392,#52393);
#45861=AXIS2_PLACEMENT_3D('',#73341,#52394,#52395);
#45862=AXIS2_PLACEMENT_3D('',#73344,#52397,#52398);
#45863=AXIS2_PLACEMENT_3D('',#73345,#52399,#52400);
#45864=AXIS2_PLACEMENT_3D('',#73347,#52401,#52402);
#45865=AXIS2_PLACEMENT_3D('',#73350,#52404,#52405);
#45866=AXIS2_PLACEMENT_3D('',#73351,#52406,#52407);
#45867=AXIS2_PLACEMENT_3D('',#73353,#52408,#52409);
#45868=AXIS2_PLACEMENT_3D('',#73356,#52411,#52412);
#45869=AXIS2_PLACEMENT_3D('',#73357,#52413,#52414);
#45870=AXIS2_PLACEMENT_3D('',#73359,#52415,#52416);
#45871=AXIS2_PLACEMENT_3D('',#73362,#52418,#52419);
#45872=AXIS2_PLACEMENT_3D('',#73363,#52420,#52421);
#45873=AXIS2_PLACEMENT_3D('',#73365,#52422,#52423);
#45874=AXIS2_PLACEMENT_3D('',#73368,#52425,#52426);
#45875=AXIS2_PLACEMENT_3D('',#73369,#52427,#52428);
#45876=AXIS2_PLACEMENT_3D('',#73371,#52429,#52430);
#45877=AXIS2_PLACEMENT_3D('',#73401,#52432,#52433);
#45878=AXIS2_PLACEMENT_3D('',#73410,#52434,#52435);
#45879=AXIS2_PLACEMENT_3D('',#73412,#52436,#52437);
#45880=AXIS2_PLACEMENT_3D('',#73415,#52439,#52440);
#45881=AXIS2_PLACEMENT_3D('',#73416,#52441,#52442);
#45882=AXIS2_PLACEMENT_3D('',#73418,#52443,#52444);
#45883=AXIS2_PLACEMENT_3D('',#73421,#52446,#52447);
#45884=AXIS2_PLACEMENT_3D('',#73422,#52448,#52449);
#45885=AXIS2_PLACEMENT_3D('',#73424,#52450,#52451);
#45886=AXIS2_PLACEMENT_3D('',#73427,#52453,#52454);
#45887=AXIS2_PLACEMENT_3D('',#73428,#52455,#52456);
#45888=AXIS2_PLACEMENT_3D('',#73430,#52457,#52458);
#45889=AXIS2_PLACEMENT_3D('',#73433,#52460,#52461);
#45890=AXIS2_PLACEMENT_3D('',#73434,#52462,#52463);
#45891=AXIS2_PLACEMENT_3D('',#73436,#52464,#52465);
#45892=AXIS2_PLACEMENT_3D('',#73439,#52467,#52468);
#45893=AXIS2_PLACEMENT_3D('',#73440,#52469,#52470);
#45894=AXIS2_PLACEMENT_3D('',#73442,#52471,#52472);
#45895=AXIS2_PLACEMENT_3D('',#73445,#52474,#52475);
#45896=AXIS2_PLACEMENT_3D('',#73446,#52476,#52477);
#45897=AXIS2_PLACEMENT_3D('',#73448,#52478,#52479);
#45898=AXIS2_PLACEMENT_3D('',#73451,#52481,#52482);
#45899=AXIS2_PLACEMENT_3D('',#73452,#52483,#52484);
#45900=AXIS2_PLACEMENT_3D('',#73454,#52485,#52486);
#45901=AXIS2_PLACEMENT_3D('',#73457,#52488,#52489);
#45902=AXIS2_PLACEMENT_3D('',#73458,#52490,#52491);
#45903=AXIS2_PLACEMENT_3D('',#73460,#52492,#52493);
#45904=AXIS2_PLACEMENT_3D('',#73463,#52495,#52496);
#45905=AXIS2_PLACEMENT_3D('',#73464,#52497,#52498);
#45906=AXIS2_PLACEMENT_3D('',#73466,#52499,#52500);
#45907=AXIS2_PLACEMENT_3D('',#73469,#52502,#52503);
#45908=AXIS2_PLACEMENT_3D('',#73470,#52504,#52505);
#45909=AXIS2_PLACEMENT_3D('',#73472,#52506,#52507);
#45910=AXIS2_PLACEMENT_3D('',#73475,#52509,#52510);
#45911=AXIS2_PLACEMENT_3D('',#73476,#52511,#52512);
#45912=AXIS2_PLACEMENT_3D('',#73478,#52513,#52514);
#45913=AXIS2_PLACEMENT_3D('',#73481,#52516,#52517);
#45914=AXIS2_PLACEMENT_3D('',#73482,#52518,#52519);
#45915=AXIS2_PLACEMENT_3D('',#73484,#52520,#52521);
#45916=AXIS2_PLACEMENT_3D('',#73487,#52523,#52524);
#45917=AXIS2_PLACEMENT_3D('',#73488,#52525,#52526);
#45918=AXIS2_PLACEMENT_3D('',#73490,#52527,#52528);
#45919=AXIS2_PLACEMENT_3D('',#73493,#52530,#52531);
#45920=AXIS2_PLACEMENT_3D('',#73494,#52532,#52533);
#45921=AXIS2_PLACEMENT_3D('',#73496,#52534,#52535);
#45922=AXIS2_PLACEMENT_3D('',#73499,#52537,#52538);
#45923=AXIS2_PLACEMENT_3D('',#73500,#52539,#52540);
#45924=AXIS2_PLACEMENT_3D('',#73502,#52541,#52542);
#45925=AXIS2_PLACEMENT_3D('',#73505,#52544,#52545);
#45926=AXIS2_PLACEMENT_3D('',#73506,#52546,#52547);
#45927=AXIS2_PLACEMENT_3D('',#73508,#52548,#52549);
#45928=AXIS2_PLACEMENT_3D('',#73511,#52551,#52552);
#45929=AXIS2_PLACEMENT_3D('',#73512,#52553,#52554);
#45930=AXIS2_PLACEMENT_3D('',#73514,#52555,#52556);
#45931=AXIS2_PLACEMENT_3D('',#73542,#52558,#52559);
#45932=AXIS2_PLACEMENT_3D('',#73553,#52560,#52561);
#45933=AXIS2_PLACEMENT_3D('',#73555,#52562,#52563);
#45934=AXIS2_PLACEMENT_3D('',#73558,#52565,#52566);
#45935=AXIS2_PLACEMENT_3D('',#73559,#52567,#52568);
#45936=AXIS2_PLACEMENT_3D('',#73561,#52569,#52570);
#45937=AXIS2_PLACEMENT_3D('',#73564,#52572,#52573);
#45938=AXIS2_PLACEMENT_3D('',#73565,#52574,#52575);
#45939=AXIS2_PLACEMENT_3D('',#73567,#52576,#52577);
#45940=AXIS2_PLACEMENT_3D('',#73570,#52579,#52580);
#45941=AXIS2_PLACEMENT_3D('',#73571,#52581,#52582);
#45942=AXIS2_PLACEMENT_3D('',#73573,#52583,#52584);
#45943=AXIS2_PLACEMENT_3D('',#73576,#52586,#52587);
#45944=AXIS2_PLACEMENT_3D('',#73577,#52588,#52589);
#45945=AXIS2_PLACEMENT_3D('',#73579,#52590,#52591);
#45946=AXIS2_PLACEMENT_3D('',#73582,#52593,#52594);
#45947=AXIS2_PLACEMENT_3D('',#73583,#52595,#52596);
#45948=AXIS2_PLACEMENT_3D('',#73585,#52597,#52598);
#45949=AXIS2_PLACEMENT_3D('',#73588,#52600,#52601);
#45950=AXIS2_PLACEMENT_3D('',#73589,#52602,#52603);
#45951=AXIS2_PLACEMENT_3D('',#73591,#52604,#52605);
#45952=AXIS2_PLACEMENT_3D('',#73594,#52607,#52608);
#45953=AXIS2_PLACEMENT_3D('',#73595,#52609,#52610);
#45954=AXIS2_PLACEMENT_3D('',#73597,#52611,#52612);
#45955=AXIS2_PLACEMENT_3D('',#73600,#52614,#52615);
#45956=AXIS2_PLACEMENT_3D('',#73601,#52616,#52617);
#45957=AXIS2_PLACEMENT_3D('',#73603,#52618,#52619);
#45958=AXIS2_PLACEMENT_3D('',#73606,#52621,#52622);
#45959=AXIS2_PLACEMENT_3D('',#73607,#52623,#52624);
#45960=AXIS2_PLACEMENT_3D('',#73609,#52625,#52626);
#45961=AXIS2_PLACEMENT_3D('',#73612,#52628,#52629);
#45962=AXIS2_PLACEMENT_3D('',#73613,#52630,#52631);
#45963=AXIS2_PLACEMENT_3D('',#73615,#52632,#52633);
#45964=AXIS2_PLACEMENT_3D('',#73618,#52635,#52636);
#45965=AXIS2_PLACEMENT_3D('',#73619,#52637,#52638);
#45966=AXIS2_PLACEMENT_3D('',#73621,#52639,#52640);
#45967=AXIS2_PLACEMENT_3D('',#73624,#52642,#52643);
#45968=AXIS2_PLACEMENT_3D('',#73625,#52644,#52645);
#45969=AXIS2_PLACEMENT_3D('',#73627,#52646,#52647);
#45970=AXIS2_PLACEMENT_3D('',#73630,#52649,#52650);
#45971=AXIS2_PLACEMENT_3D('',#73631,#52651,#52652);
#45972=AXIS2_PLACEMENT_3D('',#73633,#52653,#52654);
#45973=AXIS2_PLACEMENT_3D('',#73636,#52656,#52657);
#45974=AXIS2_PLACEMENT_3D('',#73637,#52658,#52659);
#45975=AXIS2_PLACEMENT_3D('',#73639,#52660,#52661);
#45976=AXIS2_PLACEMENT_3D('',#73642,#52663,#52664);
#45977=AXIS2_PLACEMENT_3D('',#73643,#52665,#52666);
#45978=AXIS2_PLACEMENT_3D('',#73645,#52667,#52668);
#45979=AXIS2_PLACEMENT_3D('',#73673,#52670,#52671);
#45980=AXIS2_PLACEMENT_3D('',#73684,#52672,#52673);
#45981=AXIS2_PLACEMENT_3D('',#73686,#52674,#52675);
#45982=AXIS2_PLACEMENT_3D('',#73689,#52677,#52678);
#45983=AXIS2_PLACEMENT_3D('',#73690,#52679,#52680);
#45984=AXIS2_PLACEMENT_3D('',#73692,#52681,#52682);
#45985=AXIS2_PLACEMENT_3D('',#73695,#52684,#52685);
#45986=AXIS2_PLACEMENT_3D('',#73696,#52686,#52687);
#45987=AXIS2_PLACEMENT_3D('',#73698,#52688,#52689);
#45988=AXIS2_PLACEMENT_3D('',#73701,#52691,#52692);
#45989=AXIS2_PLACEMENT_3D('',#73702,#52693,#52694);
#45990=AXIS2_PLACEMENT_3D('',#73704,#52695,#52696);
#45991=AXIS2_PLACEMENT_3D('',#73707,#52698,#52699);
#45992=AXIS2_PLACEMENT_3D('',#73708,#52700,#52701);
#45993=AXIS2_PLACEMENT_3D('',#73710,#52702,#52703);
#45994=AXIS2_PLACEMENT_3D('',#73713,#52705,#52706);
#45995=AXIS2_PLACEMENT_3D('',#73714,#52707,#52708);
#45996=AXIS2_PLACEMENT_3D('',#73716,#52709,#52710);
#45997=AXIS2_PLACEMENT_3D('',#73719,#52712,#52713);
#45998=AXIS2_PLACEMENT_3D('',#73720,#52714,#52715);
#45999=AXIS2_PLACEMENT_3D('',#73722,#52716,#52717);
#46000=AXIS2_PLACEMENT_3D('',#73725,#52719,#52720);
#46001=AXIS2_PLACEMENT_3D('',#73726,#52721,#52722);
#46002=AXIS2_PLACEMENT_3D('',#73728,#52723,#52724);
#46003=AXIS2_PLACEMENT_3D('',#73731,#52726,#52727);
#46004=AXIS2_PLACEMENT_3D('',#73732,#52728,#52729);
#46005=AXIS2_PLACEMENT_3D('',#73734,#52730,#52731);
#46006=AXIS2_PLACEMENT_3D('',#73737,#52733,#52734);
#46007=AXIS2_PLACEMENT_3D('',#73738,#52735,#52736);
#46008=AXIS2_PLACEMENT_3D('',#73740,#52737,#52738);
#46009=AXIS2_PLACEMENT_3D('',#73743,#52740,#52741);
#46010=AXIS2_PLACEMENT_3D('',#73744,#52742,#52743);
#46011=AXIS2_PLACEMENT_3D('',#73746,#52744,#52745);
#46012=AXIS2_PLACEMENT_3D('',#73749,#52747,#52748);
#46013=AXIS2_PLACEMENT_3D('',#73750,#52749,#52750);
#46014=AXIS2_PLACEMENT_3D('',#73752,#52751,#52752);
#46015=AXIS2_PLACEMENT_3D('',#73755,#52754,#52755);
#46016=AXIS2_PLACEMENT_3D('',#73756,#52756,#52757);
#46017=AXIS2_PLACEMENT_3D('',#73758,#52758,#52759);
#46018=AXIS2_PLACEMENT_3D('',#73761,#52761,#52762);
#46019=AXIS2_PLACEMENT_3D('',#73762,#52763,#52764);
#46020=AXIS2_PLACEMENT_3D('',#73764,#52765,#52766);
#46021=AXIS2_PLACEMENT_3D('',#73767,#52768,#52769);
#46022=AXIS2_PLACEMENT_3D('',#73768,#52770,#52771);
#46023=AXIS2_PLACEMENT_3D('',#73770,#52772,#52773);
#46024=AXIS2_PLACEMENT_3D('',#73773,#52775,#52776);
#46025=AXIS2_PLACEMENT_3D('',#73774,#52777,#52778);
#46026=AXIS2_PLACEMENT_3D('',#73776,#52779,#52780);
#46027=AXIS2_PLACEMENT_3D('',#73779,#52782,#52783);
#46028=AXIS2_PLACEMENT_3D('',#73780,#52784,#52785);
#46029=AXIS2_PLACEMENT_3D('',#73782,#52786,#52787);
#46030=AXIS2_PLACEMENT_3D('',#73785,#52789,#52790);
#46031=AXIS2_PLACEMENT_3D('',#73786,#52791,#52792);
#46032=AXIS2_PLACEMENT_3D('',#73788,#52793,#52794);
#46033=AXIS2_PLACEMENT_3D('',#73814,#52796,#52797);
#46034=AXIS2_PLACEMENT_3D('',#73827,#52798,#52799);
#46035=AXIS2_PLACEMENT_3D('',#73829,#52800,#52801);
#46036=AXIS2_PLACEMENT_3D('',#73832,#52803,#52804);
#46037=AXIS2_PLACEMENT_3D('',#73833,#52805,#52806);
#46038=AXIS2_PLACEMENT_3D('',#73835,#52807,#52808);
#46039=AXIS2_PLACEMENT_3D('',#73838,#52810,#52811);
#46040=AXIS2_PLACEMENT_3D('',#73839,#52812,#52813);
#46041=AXIS2_PLACEMENT_3D('',#73841,#52814,#52815);
#46042=AXIS2_PLACEMENT_3D('',#73844,#52817,#52818);
#46043=AXIS2_PLACEMENT_3D('',#73845,#52819,#52820);
#46044=AXIS2_PLACEMENT_3D('',#73847,#52821,#52822);
#46045=AXIS2_PLACEMENT_3D('',#73850,#52824,#52825);
#46046=AXIS2_PLACEMENT_3D('',#73851,#52826,#52827);
#46047=AXIS2_PLACEMENT_3D('',#73853,#52828,#52829);
#46048=AXIS2_PLACEMENT_3D('',#73856,#52831,#52832);
#46049=AXIS2_PLACEMENT_3D('',#73857,#52833,#52834);
#46050=AXIS2_PLACEMENT_3D('',#73859,#52835,#52836);
#46051=AXIS2_PLACEMENT_3D('',#73862,#52838,#52839);
#46052=AXIS2_PLACEMENT_3D('',#73863,#52840,#52841);
#46053=AXIS2_PLACEMENT_3D('',#73865,#52842,#52843);
#46054=AXIS2_PLACEMENT_3D('',#73868,#52845,#52846);
#46055=AXIS2_PLACEMENT_3D('',#73869,#52847,#52848);
#46056=AXIS2_PLACEMENT_3D('',#73871,#52849,#52850);
#46057=AXIS2_PLACEMENT_3D('',#73874,#52852,#52853);
#46058=AXIS2_PLACEMENT_3D('',#73875,#52854,#52855);
#46059=AXIS2_PLACEMENT_3D('',#73877,#52856,#52857);
#46060=AXIS2_PLACEMENT_3D('',#73880,#52859,#52860);
#46061=AXIS2_PLACEMENT_3D('',#73881,#52861,#52862);
#46062=AXIS2_PLACEMENT_3D('',#73883,#52863,#52864);
#46063=AXIS2_PLACEMENT_3D('',#73886,#52866,#52867);
#46064=AXIS2_PLACEMENT_3D('',#73887,#52868,#52869);
#46065=AXIS2_PLACEMENT_3D('',#73889,#52870,#52871);
#46066=AXIS2_PLACEMENT_3D('',#73892,#52873,#52874);
#46067=AXIS2_PLACEMENT_3D('',#73893,#52875,#52876);
#46068=AXIS2_PLACEMENT_3D('',#73895,#52877,#52878);
#46069=AXIS2_PLACEMENT_3D('',#73898,#52880,#52881);
#46070=AXIS2_PLACEMENT_3D('',#73899,#52882,#52883);
#46071=AXIS2_PLACEMENT_3D('',#73901,#52884,#52885);
#46072=AXIS2_PLACEMENT_3D('',#73904,#52887,#52888);
#46073=AXIS2_PLACEMENT_3D('',#73905,#52889,#52890);
#46074=AXIS2_PLACEMENT_3D('',#73907,#52891,#52892);
#46075=AXIS2_PLACEMENT_3D('',#73910,#52894,#52895);
#46076=AXIS2_PLACEMENT_3D('',#73911,#52896,#52897);
#46077=AXIS2_PLACEMENT_3D('',#73913,#52898,#52899);
#46078=AXIS2_PLACEMENT_3D('',#73916,#52901,#52902);
#46079=AXIS2_PLACEMENT_3D('',#73917,#52903,#52904);
#46080=AXIS2_PLACEMENT_3D('',#73919,#52905,#52906);
#46081=AXIS2_PLACEMENT_3D('',#73922,#52908,#52909);
#46082=AXIS2_PLACEMENT_3D('',#73923,#52910,#52911);
#46083=AXIS2_PLACEMENT_3D('',#73925,#52912,#52913);
#46084=AXIS2_PLACEMENT_3D('',#73928,#52915,#52916);
#46085=AXIS2_PLACEMENT_3D('',#73929,#52917,#52918);
#46086=AXIS2_PLACEMENT_3D('',#73931,#52919,#52920);
#46087=AXIS2_PLACEMENT_3D('',#73957,#52922,#52923);
#46088=AXIS2_PLACEMENT_3D('',#73970,#52924,#52925);
#46089=AXIS2_PLACEMENT_3D('',#73972,#52926,#52927);
#46090=AXIS2_PLACEMENT_3D('',#73975,#52929,#52930);
#46091=AXIS2_PLACEMENT_3D('',#73976,#52931,#52932);
#46092=AXIS2_PLACEMENT_3D('',#73978,#52933,#52934);
#46093=AXIS2_PLACEMENT_3D('',#73981,#52936,#52937);
#46094=AXIS2_PLACEMENT_3D('',#73982,#52938,#52939);
#46095=AXIS2_PLACEMENT_3D('',#73984,#52940,#52941);
#46096=AXIS2_PLACEMENT_3D('',#73987,#52943,#52944);
#46097=AXIS2_PLACEMENT_3D('',#73988,#52945,#52946);
#46098=AXIS2_PLACEMENT_3D('',#73990,#52947,#52948);
#46099=AXIS2_PLACEMENT_3D('',#73993,#52950,#52951);
#46100=AXIS2_PLACEMENT_3D('',#73994,#52952,#52953);
#46101=AXIS2_PLACEMENT_3D('',#73996,#52954,#52955);
#46102=AXIS2_PLACEMENT_3D('',#73999,#52957,#52958);
#46103=AXIS2_PLACEMENT_3D('',#74000,#52959,#52960);
#46104=AXIS2_PLACEMENT_3D('',#74002,#52961,#52962);
#46105=AXIS2_PLACEMENT_3D('',#74005,#52964,#52965);
#46106=AXIS2_PLACEMENT_3D('',#74006,#52966,#52967);
#46107=AXIS2_PLACEMENT_3D('',#74008,#52968,#52969);
#46108=AXIS2_PLACEMENT_3D('',#74011,#52971,#52972);
#46109=AXIS2_PLACEMENT_3D('',#74012,#52973,#52974);
#46110=AXIS2_PLACEMENT_3D('',#74014,#52975,#52976);
#46111=AXIS2_PLACEMENT_3D('',#74017,#52978,#52979);
#46112=AXIS2_PLACEMENT_3D('',#74018,#52980,#52981);
#46113=AXIS2_PLACEMENT_3D('',#74020,#52982,#52983);
#46114=AXIS2_PLACEMENT_3D('',#74023,#52985,#52986);
#46115=AXIS2_PLACEMENT_3D('',#74024,#52987,#52988);
#46116=AXIS2_PLACEMENT_3D('',#74026,#52989,#52990);
#46117=AXIS2_PLACEMENT_3D('',#74029,#52992,#52993);
#46118=AXIS2_PLACEMENT_3D('',#74030,#52994,#52995);
#46119=AXIS2_PLACEMENT_3D('',#74032,#52996,#52997);
#46120=AXIS2_PLACEMENT_3D('',#74035,#52999,#53000);
#46121=AXIS2_PLACEMENT_3D('',#74036,#53001,#53002);
#46122=AXIS2_PLACEMENT_3D('',#74038,#53003,#53004);
#46123=AXIS2_PLACEMENT_3D('',#74041,#53006,#53007);
#46124=AXIS2_PLACEMENT_3D('',#74042,#53008,#53009);
#46125=AXIS2_PLACEMENT_3D('',#74044,#53010,#53011);
#46126=AXIS2_PLACEMENT_3D('',#74047,#53013,#53014);
#46127=AXIS2_PLACEMENT_3D('',#74048,#53015,#53016);
#46128=AXIS2_PLACEMENT_3D('',#74050,#53017,#53018);
#46129=AXIS2_PLACEMENT_3D('',#74053,#53020,#53021);
#46130=AXIS2_PLACEMENT_3D('',#74054,#53022,#53023);
#46131=AXIS2_PLACEMENT_3D('',#74056,#53024,#53025);
#46132=AXIS2_PLACEMENT_3D('',#74059,#53027,#53028);
#46133=AXIS2_PLACEMENT_3D('',#74060,#53029,#53030);
#46134=AXIS2_PLACEMENT_3D('',#74062,#53031,#53032);
#46135=AXIS2_PLACEMENT_3D('',#74065,#53034,#53035);
#46136=AXIS2_PLACEMENT_3D('',#74066,#53036,#53037);
#46137=AXIS2_PLACEMENT_3D('',#74068,#53038,#53039);
#46138=AXIS2_PLACEMENT_3D('',#74071,#53041,#53042);
#46139=AXIS2_PLACEMENT_3D('',#74072,#53043,#53044);
#46140=AXIS2_PLACEMENT_3D('',#74074,#53045,#53046);
#46141=AXIS2_PLACEMENT_3D('',#74098,#53048,#53049);
#46142=AXIS2_PLACEMENT_3D('',#74113,#53050,#53051);
#46143=AXIS2_PLACEMENT_3D('',#74115,#53052,#53053);
#46144=AXIS2_PLACEMENT_3D('',#74118,#53055,#53056);
#46145=AXIS2_PLACEMENT_3D('',#74119,#53057,#53058);
#46146=AXIS2_PLACEMENT_3D('',#74121,#53059,#53060);
#46147=AXIS2_PLACEMENT_3D('',#74124,#53062,#53063);
#46148=AXIS2_PLACEMENT_3D('',#74125,#53064,#53065);
#46149=AXIS2_PLACEMENT_3D('',#74127,#53066,#53067);
#46150=AXIS2_PLACEMENT_3D('',#74130,#53069,#53070);
#46151=AXIS2_PLACEMENT_3D('',#74131,#53071,#53072);
#46152=AXIS2_PLACEMENT_3D('',#74133,#53073,#53074);
#46153=AXIS2_PLACEMENT_3D('',#74136,#53076,#53077);
#46154=AXIS2_PLACEMENT_3D('',#74137,#53078,#53079);
#46155=AXIS2_PLACEMENT_3D('',#74139,#53080,#53081);
#46156=AXIS2_PLACEMENT_3D('',#74142,#53083,#53084);
#46157=AXIS2_PLACEMENT_3D('',#74143,#53085,#53086);
#46158=AXIS2_PLACEMENT_3D('',#74145,#53087,#53088);
#46159=AXIS2_PLACEMENT_3D('',#74148,#53090,#53091);
#46160=AXIS2_PLACEMENT_3D('',#74149,#53092,#53093);
#46161=AXIS2_PLACEMENT_3D('',#74151,#53094,#53095);
#46162=AXIS2_PLACEMENT_3D('',#74154,#53097,#53098);
#46163=AXIS2_PLACEMENT_3D('',#74155,#53099,#53100);
#46164=AXIS2_PLACEMENT_3D('',#74157,#53101,#53102);
#46165=AXIS2_PLACEMENT_3D('',#74160,#53104,#53105);
#46166=AXIS2_PLACEMENT_3D('',#74161,#53106,#53107);
#46167=AXIS2_PLACEMENT_3D('',#74163,#53108,#53109);
#46168=AXIS2_PLACEMENT_3D('',#74166,#53111,#53112);
#46169=AXIS2_PLACEMENT_3D('',#74167,#53113,#53114);
#46170=AXIS2_PLACEMENT_3D('',#74169,#53115,#53116);
#46171=AXIS2_PLACEMENT_3D('',#74172,#53118,#53119);
#46172=AXIS2_PLACEMENT_3D('',#74173,#53120,#53121);
#46173=AXIS2_PLACEMENT_3D('',#74175,#53122,#53123);
#46174=AXIS2_PLACEMENT_3D('',#74178,#53125,#53126);
#46175=AXIS2_PLACEMENT_3D('',#74179,#53127,#53128);
#46176=AXIS2_PLACEMENT_3D('',#74181,#53129,#53130);
#46177=AXIS2_PLACEMENT_3D('',#74184,#53132,#53133);
#46178=AXIS2_PLACEMENT_3D('',#74185,#53134,#53135);
#46179=AXIS2_PLACEMENT_3D('',#74187,#53136,#53137);
#46180=AXIS2_PLACEMENT_3D('',#74190,#53139,#53140);
#46181=AXIS2_PLACEMENT_3D('',#74191,#53141,#53142);
#46182=AXIS2_PLACEMENT_3D('',#74193,#53143,#53144);
#46183=AXIS2_PLACEMENT_3D('',#74196,#53146,#53147);
#46184=AXIS2_PLACEMENT_3D('',#74197,#53148,#53149);
#46185=AXIS2_PLACEMENT_3D('',#74199,#53150,#53151);
#46186=AXIS2_PLACEMENT_3D('',#74202,#53153,#53154);
#46187=AXIS2_PLACEMENT_3D('',#74203,#53155,#53156);
#46188=AXIS2_PLACEMENT_3D('',#74205,#53157,#53158);
#46189=AXIS2_PLACEMENT_3D('',#74208,#53160,#53161);
#46190=AXIS2_PLACEMENT_3D('',#74209,#53162,#53163);
#46191=AXIS2_PLACEMENT_3D('',#74211,#53164,#53165);
#46192=AXIS2_PLACEMENT_3D('',#74214,#53167,#53168);
#46193=AXIS2_PLACEMENT_3D('',#74215,#53169,#53170);
#46194=AXIS2_PLACEMENT_3D('',#74217,#53171,#53172);
#46195=AXIS2_PLACEMENT_3D('',#74241,#53174,#53175);
#46196=AXIS2_PLACEMENT_3D('',#74256,#53176,#53177);
#46197=AXIS2_PLACEMENT_3D('',#74258,#53178,#53179);
#46198=AXIS2_PLACEMENT_3D('',#74261,#53181,#53182);
#46199=AXIS2_PLACEMENT_3D('',#74262,#53183,#53184);
#46200=AXIS2_PLACEMENT_3D('',#74264,#53185,#53186);
#46201=AXIS2_PLACEMENT_3D('',#74267,#53188,#53189);
#46202=AXIS2_PLACEMENT_3D('',#74268,#53190,#53191);
#46203=AXIS2_PLACEMENT_3D('',#74270,#53192,#53193);
#46204=AXIS2_PLACEMENT_3D('',#74273,#53195,#53196);
#46205=AXIS2_PLACEMENT_3D('',#74274,#53197,#53198);
#46206=AXIS2_PLACEMENT_3D('',#74276,#53199,#53200);
#46207=AXIS2_PLACEMENT_3D('',#74279,#53202,#53203);
#46208=AXIS2_PLACEMENT_3D('',#74280,#53204,#53205);
#46209=AXIS2_PLACEMENT_3D('',#74282,#53206,#53207);
#46210=AXIS2_PLACEMENT_3D('',#74285,#53209,#53210);
#46211=AXIS2_PLACEMENT_3D('',#74286,#53211,#53212);
#46212=AXIS2_PLACEMENT_3D('',#74288,#53213,#53214);
#46213=AXIS2_PLACEMENT_3D('',#74291,#53216,#53217);
#46214=AXIS2_PLACEMENT_3D('',#74292,#53218,#53219);
#46215=AXIS2_PLACEMENT_3D('',#74294,#53220,#53221);
#46216=AXIS2_PLACEMENT_3D('',#74297,#53223,#53224);
#46217=AXIS2_PLACEMENT_3D('',#74298,#53225,#53226);
#46218=AXIS2_PLACEMENT_3D('',#74300,#53227,#53228);
#46219=AXIS2_PLACEMENT_3D('',#74303,#53230,#53231);
#46220=AXIS2_PLACEMENT_3D('',#74304,#53232,#53233);
#46221=AXIS2_PLACEMENT_3D('',#74306,#53234,#53235);
#46222=AXIS2_PLACEMENT_3D('',#74309,#53237,#53238);
#46223=AXIS2_PLACEMENT_3D('',#74310,#53239,#53240);
#46224=AXIS2_PLACEMENT_3D('',#74312,#53241,#53242);
#46225=AXIS2_PLACEMENT_3D('',#74315,#53244,#53245);
#46226=AXIS2_PLACEMENT_3D('',#74316,#53246,#53247);
#46227=AXIS2_PLACEMENT_3D('',#74318,#53248,#53249);
#46228=AXIS2_PLACEMENT_3D('',#74321,#53251,#53252);
#46229=AXIS2_PLACEMENT_3D('',#74322,#53253,#53254);
#46230=AXIS2_PLACEMENT_3D('',#74324,#53255,#53256);
#46231=AXIS2_PLACEMENT_3D('',#74327,#53258,#53259);
#46232=AXIS2_PLACEMENT_3D('',#74328,#53260,#53261);
#46233=AXIS2_PLACEMENT_3D('',#74330,#53262,#53263);
#46234=AXIS2_PLACEMENT_3D('',#74333,#53265,#53266);
#46235=AXIS2_PLACEMENT_3D('',#74334,#53267,#53268);
#46236=AXIS2_PLACEMENT_3D('',#74336,#53269,#53270);
#46237=AXIS2_PLACEMENT_3D('',#74339,#53272,#53273);
#46238=AXIS2_PLACEMENT_3D('',#74340,#53274,#53275);
#46239=AXIS2_PLACEMENT_3D('',#74342,#53276,#53277);
#46240=AXIS2_PLACEMENT_3D('',#74345,#53279,#53280);
#46241=AXIS2_PLACEMENT_3D('',#74346,#53281,#53282);
#46242=AXIS2_PLACEMENT_3D('',#74348,#53283,#53284);
#46243=AXIS2_PLACEMENT_3D('',#74367,#53286,#53287);
#46244=AXIS2_PLACEMENT_3D('',#74387,#53288,#53289);
#46245=AXIS2_PLACEMENT_3D('',#74389,#53290,#53291);
#46246=AXIS2_PLACEMENT_3D('',#74392,#53293,#53294);
#46247=AXIS2_PLACEMENT_3D('',#74393,#53295,#53296);
#46248=AXIS2_PLACEMENT_3D('',#74395,#53297,#53298);
#46249=AXIS2_PLACEMENT_3D('',#74398,#53300,#53301);
#46250=AXIS2_PLACEMENT_3D('',#74399,#53302,#53303);
#46251=AXIS2_PLACEMENT_3D('',#74401,#53304,#53305);
#46252=AXIS2_PLACEMENT_3D('',#74404,#53307,#53308);
#46253=AXIS2_PLACEMENT_3D('',#74405,#53309,#53310);
#46254=AXIS2_PLACEMENT_3D('',#74407,#53311,#53312);
#46255=AXIS2_PLACEMENT_3D('',#74410,#53314,#53315);
#46256=AXIS2_PLACEMENT_3D('',#74411,#53316,#53317);
#46257=AXIS2_PLACEMENT_3D('',#74413,#53318,#53319);
#46258=AXIS2_PLACEMENT_3D('',#74416,#53321,#53322);
#46259=AXIS2_PLACEMENT_3D('',#74417,#53323,#53324);
#46260=AXIS2_PLACEMENT_3D('',#74419,#53325,#53326);
#46261=AXIS2_PLACEMENT_3D('',#74422,#53328,#53329);
#46262=AXIS2_PLACEMENT_3D('',#74423,#53330,#53331);
#46263=AXIS2_PLACEMENT_3D('',#74425,#53332,#53333);
#46264=AXIS2_PLACEMENT_3D('',#74428,#53335,#53336);
#46265=AXIS2_PLACEMENT_3D('',#74429,#53337,#53338);
#46266=AXIS2_PLACEMENT_3D('',#74431,#53339,#53340);
#46267=AXIS2_PLACEMENT_3D('',#74434,#53342,#53343);
#46268=AXIS2_PLACEMENT_3D('',#74435,#53344,#53345);
#46269=AXIS2_PLACEMENT_3D('',#74437,#53346,#53347);
#46270=AXIS2_PLACEMENT_3D('',#74440,#53349,#53350);
#46271=AXIS2_PLACEMENT_3D('',#74441,#53351,#53352);
#46272=AXIS2_PLACEMENT_3D('',#74443,#53353,#53354);
#46273=AXIS2_PLACEMENT_3D('',#74446,#53356,#53357);
#46274=AXIS2_PLACEMENT_3D('',#74447,#53358,#53359);
#46275=AXIS2_PLACEMENT_3D('',#74449,#53360,#53361);
#46276=AXIS2_PLACEMENT_3D('',#74452,#53363,#53364);
#46277=AXIS2_PLACEMENT_3D('',#74453,#53365,#53366);
#46278=AXIS2_PLACEMENT_3D('',#74455,#53367,#53368);
#46279=AXIS2_PLACEMENT_3D('',#74458,#53370,#53371);
#46280=AXIS2_PLACEMENT_3D('',#74459,#53372,#53373);
#46281=AXIS2_PLACEMENT_3D('',#74461,#53374,#53375);
#46282=AXIS2_PLACEMENT_3D('',#74464,#53377,#53378);
#46283=AXIS2_PLACEMENT_3D('',#74465,#53379,#53380);
#46284=AXIS2_PLACEMENT_3D('',#74467,#53381,#53382);
#46285=AXIS2_PLACEMENT_3D('',#74470,#53384,#53385);
#46286=AXIS2_PLACEMENT_3D('',#74471,#53386,#53387);
#46287=AXIS2_PLACEMENT_3D('',#74473,#53388,#53389);
#46288=AXIS2_PLACEMENT_3D('',#74476,#53391,#53392);
#46289=AXIS2_PLACEMENT_3D('',#74477,#53393,#53394);
#46290=AXIS2_PLACEMENT_3D('',#74479,#53395,#53396);
#46291=AXIS2_PLACEMENT_3D('',#74482,#53398,#53399);
#46292=AXIS2_PLACEMENT_3D('',#74483,#53400,#53401);
#46293=AXIS2_PLACEMENT_3D('',#74485,#53402,#53403);
#46294=AXIS2_PLACEMENT_3D('',#74488,#53405,#53406);
#46295=AXIS2_PLACEMENT_3D('',#74489,#53407,#53408);
#46296=AXIS2_PLACEMENT_3D('',#74491,#53409,#53410);
#46297=AXIS2_PLACEMENT_3D('',#74510,#53412,#53413);
#46298=AXIS2_PLACEMENT_3D('',#74530,#53414,#53415);
#46299=AXIS2_PLACEMENT_3D('',#74532,#53416,#53417);
#46300=AXIS2_PLACEMENT_3D('',#74535,#53419,#53420);
#46301=AXIS2_PLACEMENT_3D('',#74536,#53421,#53422);
#46302=AXIS2_PLACEMENT_3D('',#74538,#53423,#53424);
#46303=AXIS2_PLACEMENT_3D('',#74541,#53426,#53427);
#46304=AXIS2_PLACEMENT_3D('',#74542,#53428,#53429);
#46305=AXIS2_PLACEMENT_3D('',#74544,#53430,#53431);
#46306=AXIS2_PLACEMENT_3D('',#74547,#53433,#53434);
#46307=AXIS2_PLACEMENT_3D('',#74548,#53435,#53436);
#46308=AXIS2_PLACEMENT_3D('',#74550,#53437,#53438);
#46309=AXIS2_PLACEMENT_3D('',#74553,#53440,#53441);
#46310=AXIS2_PLACEMENT_3D('',#74554,#53442,#53443);
#46311=AXIS2_PLACEMENT_3D('',#74556,#53444,#53445);
#46312=AXIS2_PLACEMENT_3D('',#74559,#53447,#53448);
#46313=AXIS2_PLACEMENT_3D('',#74560,#53449,#53450);
#46314=AXIS2_PLACEMENT_3D('',#74562,#53451,#53452);
#46315=AXIS2_PLACEMENT_3D('',#74565,#53454,#53455);
#46316=AXIS2_PLACEMENT_3D('',#74566,#53456,#53457);
#46317=AXIS2_PLACEMENT_3D('',#74568,#53458,#53459);
#46318=AXIS2_PLACEMENT_3D('',#74571,#53461,#53462);
#46319=AXIS2_PLACEMENT_3D('',#74572,#53463,#53464);
#46320=AXIS2_PLACEMENT_3D('',#74574,#53465,#53466);
#46321=AXIS2_PLACEMENT_3D('',#74577,#53468,#53469);
#46322=AXIS2_PLACEMENT_3D('',#74578,#53470,#53471);
#46323=AXIS2_PLACEMENT_3D('',#74580,#53472,#53473);
#46324=AXIS2_PLACEMENT_3D('',#74583,#53475,#53476);
#46325=AXIS2_PLACEMENT_3D('',#74584,#53477,#53478);
#46326=AXIS2_PLACEMENT_3D('',#74586,#53479,#53480);
#46327=AXIS2_PLACEMENT_3D('',#74589,#53482,#53483);
#46328=AXIS2_PLACEMENT_3D('',#74590,#53484,#53485);
#46329=AXIS2_PLACEMENT_3D('',#74592,#53486,#53487);
#46330=AXIS2_PLACEMENT_3D('',#74595,#53489,#53490);
#46331=AXIS2_PLACEMENT_3D('',#74596,#53491,#53492);
#46332=AXIS2_PLACEMENT_3D('',#74598,#53493,#53494);
#46333=AXIS2_PLACEMENT_3D('',#74601,#53496,#53497);
#46334=AXIS2_PLACEMENT_3D('',#74602,#53498,#53499);
#46335=AXIS2_PLACEMENT_3D('',#74604,#53500,#53501);
#46336=AXIS2_PLACEMENT_3D('',#74607,#53503,#53504);
#46337=AXIS2_PLACEMENT_3D('',#74608,#53505,#53506);
#46338=AXIS2_PLACEMENT_3D('',#74610,#53507,#53508);
#46339=AXIS2_PLACEMENT_3D('',#74613,#53510,#53511);
#46340=AXIS2_PLACEMENT_3D('',#74614,#53512,#53513);
#46341=AXIS2_PLACEMENT_3D('',#74616,#53514,#53515);
#46342=AXIS2_PLACEMENT_3D('',#74619,#53517,#53518);
#46343=AXIS2_PLACEMENT_3D('',#74620,#53519,#53520);
#46344=AXIS2_PLACEMENT_3D('',#74622,#53521,#53522);
#46345=AXIS2_PLACEMENT_3D('',#74625,#53524,#53525);
#46346=AXIS2_PLACEMENT_3D('',#74626,#53526,#53527);
#46347=AXIS2_PLACEMENT_3D('',#74628,#53528,#53529);
#46348=AXIS2_PLACEMENT_3D('',#74631,#53531,#53532);
#46349=AXIS2_PLACEMENT_3D('',#74632,#53533,#53534);
#46350=AXIS2_PLACEMENT_3D('',#74634,#53535,#53536);
#46351=AXIS2_PLACEMENT_3D('',#74651,#53538,#53539);
#46352=AXIS2_PLACEMENT_3D('',#74673,#53540,#53541);
#46353=AXIS2_PLACEMENT_3D('',#74675,#53542,#53543);
#46354=AXIS2_PLACEMENT_3D('',#74678,#53545,#53546);
#46355=AXIS2_PLACEMENT_3D('',#74679,#53547,#53548);
#46356=AXIS2_PLACEMENT_3D('',#74681,#53549,#53550);
#46357=AXIS2_PLACEMENT_3D('',#74684,#53552,#53553);
#46358=AXIS2_PLACEMENT_3D('',#74685,#53554,#53555);
#46359=AXIS2_PLACEMENT_3D('',#74687,#53556,#53557);
#46360=AXIS2_PLACEMENT_3D('',#74690,#53559,#53560);
#46361=AXIS2_PLACEMENT_3D('',#74691,#53561,#53562);
#46362=AXIS2_PLACEMENT_3D('',#74693,#53563,#53564);
#46363=AXIS2_PLACEMENT_3D('',#74696,#53566,#53567);
#46364=AXIS2_PLACEMENT_3D('',#74697,#53568,#53569);
#46365=AXIS2_PLACEMENT_3D('',#74699,#53570,#53571);
#46366=AXIS2_PLACEMENT_3D('',#74702,#53573,#53574);
#46367=AXIS2_PLACEMENT_3D('',#74703,#53575,#53576);
#46368=AXIS2_PLACEMENT_3D('',#74705,#53577,#53578);
#46369=AXIS2_PLACEMENT_3D('',#74708,#53580,#53581);
#46370=AXIS2_PLACEMENT_3D('',#74709,#53582,#53583);
#46371=AXIS2_PLACEMENT_3D('',#74711,#53584,#53585);
#46372=AXIS2_PLACEMENT_3D('',#74714,#53587,#53588);
#46373=AXIS2_PLACEMENT_3D('',#74715,#53589,#53590);
#46374=AXIS2_PLACEMENT_3D('',#74717,#53591,#53592);
#46375=AXIS2_PLACEMENT_3D('',#74720,#53594,#53595);
#46376=AXIS2_PLACEMENT_3D('',#74721,#53596,#53597);
#46377=AXIS2_PLACEMENT_3D('',#74723,#53598,#53599);
#46378=AXIS2_PLACEMENT_3D('',#74726,#53601,#53602);
#46379=AXIS2_PLACEMENT_3D('',#74727,#53603,#53604);
#46380=AXIS2_PLACEMENT_3D('',#74729,#53605,#53606);
#46381=AXIS2_PLACEMENT_3D('',#74732,#53608,#53609);
#46382=AXIS2_PLACEMENT_3D('',#74733,#53610,#53611);
#46383=AXIS2_PLACEMENT_3D('',#74735,#53612,#53613);
#46384=AXIS2_PLACEMENT_3D('',#74738,#53615,#53616);
#46385=AXIS2_PLACEMENT_3D('',#74739,#53617,#53618);
#46386=AXIS2_PLACEMENT_3D('',#74741,#53619,#53620);
#46387=AXIS2_PLACEMENT_3D('',#74744,#53622,#53623);
#46388=AXIS2_PLACEMENT_3D('',#74745,#53624,#53625);
#46389=AXIS2_PLACEMENT_3D('',#74747,#53626,#53627);
#46390=AXIS2_PLACEMENT_3D('',#74750,#53629,#53630);
#46391=AXIS2_PLACEMENT_3D('',#74751,#53631,#53632);
#46392=AXIS2_PLACEMENT_3D('',#74753,#53633,#53634);
#46393=AXIS2_PLACEMENT_3D('',#74756,#53636,#53637);
#46394=AXIS2_PLACEMENT_3D('',#74757,#53638,#53639);
#46395=AXIS2_PLACEMENT_3D('',#74759,#53640,#53641);
#46396=AXIS2_PLACEMENT_3D('',#74762,#53643,#53644);
#46397=AXIS2_PLACEMENT_3D('',#74763,#53645,#53646);
#46398=AXIS2_PLACEMENT_3D('',#74765,#53647,#53648);
#46399=AXIS2_PLACEMENT_3D('',#74768,#53650,#53651);
#46400=AXIS2_PLACEMENT_3D('',#74769,#53652,#53653);
#46401=AXIS2_PLACEMENT_3D('',#74771,#53654,#53655);
#46402=AXIS2_PLACEMENT_3D('',#74774,#53657,#53658);
#46403=AXIS2_PLACEMENT_3D('',#74775,#53659,#53660);
#46404=AXIS2_PLACEMENT_3D('',#74777,#53661,#53662);
#46405=AXIS2_PLACEMENT_3D('',#74794,#53664,#53665);
#46406=AXIS2_PLACEMENT_3D('',#74816,#53666,#53667);
#46407=AXIS2_PLACEMENT_3D('',#74818,#53668,#53669);
#46408=AXIS2_PLACEMENT_3D('',#74821,#53671,#53672);
#46409=AXIS2_PLACEMENT_3D('',#74822,#53673,#53674);
#46410=AXIS2_PLACEMENT_3D('',#74824,#53675,#53676);
#46411=AXIS2_PLACEMENT_3D('',#74827,#53678,#53679);
#46412=AXIS2_PLACEMENT_3D('',#74828,#53680,#53681);
#46413=AXIS2_PLACEMENT_3D('',#74830,#53682,#53683);
#46414=AXIS2_PLACEMENT_3D('',#74833,#53685,#53686);
#46415=AXIS2_PLACEMENT_3D('',#74834,#53687,#53688);
#46416=AXIS2_PLACEMENT_3D('',#74836,#53689,#53690);
#46417=AXIS2_PLACEMENT_3D('',#74839,#53692,#53693);
#46418=AXIS2_PLACEMENT_3D('',#74840,#53694,#53695);
#46419=AXIS2_PLACEMENT_3D('',#74842,#53696,#53697);
#46420=AXIS2_PLACEMENT_3D('',#74845,#53699,#53700);
#46421=AXIS2_PLACEMENT_3D('',#74846,#53701,#53702);
#46422=AXIS2_PLACEMENT_3D('',#74848,#53703,#53704);
#46423=AXIS2_PLACEMENT_3D('',#74851,#53706,#53707);
#46424=AXIS2_PLACEMENT_3D('',#74852,#53708,#53709);
#46425=AXIS2_PLACEMENT_3D('',#74854,#53710,#53711);
#46426=AXIS2_PLACEMENT_3D('',#74857,#53713,#53714);
#46427=AXIS2_PLACEMENT_3D('',#74858,#53715,#53716);
#46428=AXIS2_PLACEMENT_3D('',#74860,#53717,#53718);
#46429=AXIS2_PLACEMENT_3D('',#74863,#53720,#53721);
#46430=AXIS2_PLACEMENT_3D('',#74864,#53722,#53723);
#46431=AXIS2_PLACEMENT_3D('',#74866,#53724,#53725);
#46432=AXIS2_PLACEMENT_3D('',#74869,#53727,#53728);
#46433=AXIS2_PLACEMENT_3D('',#74870,#53729,#53730);
#46434=AXIS2_PLACEMENT_3D('',#74872,#53731,#53732);
#46435=AXIS2_PLACEMENT_3D('',#74875,#53734,#53735);
#46436=AXIS2_PLACEMENT_3D('',#74876,#53736,#53737);
#46437=AXIS2_PLACEMENT_3D('',#74878,#53738,#53739);
#46438=AXIS2_PLACEMENT_3D('',#74881,#53741,#53742);
#46439=AXIS2_PLACEMENT_3D('',#74882,#53743,#53744);
#46440=AXIS2_PLACEMENT_3D('',#74884,#53745,#53746);
#46441=AXIS2_PLACEMENT_3D('',#74887,#53748,#53749);
#46442=AXIS2_PLACEMENT_3D('',#74888,#53750,#53751);
#46443=AXIS2_PLACEMENT_3D('',#74890,#53752,#53753);
#46444=AXIS2_PLACEMENT_3D('',#74893,#53755,#53756);
#46445=AXIS2_PLACEMENT_3D('',#74894,#53757,#53758);
#46446=AXIS2_PLACEMENT_3D('',#74896,#53759,#53760);
#46447=AXIS2_PLACEMENT_3D('',#74899,#53762,#53763);
#46448=AXIS2_PLACEMENT_3D('',#74900,#53764,#53765);
#46449=AXIS2_PLACEMENT_3D('',#74902,#53766,#53767);
#46450=AXIS2_PLACEMENT_3D('',#74905,#53769,#53770);
#46451=AXIS2_PLACEMENT_3D('',#74906,#53771,#53772);
#46452=AXIS2_PLACEMENT_3D('',#74908,#53773,#53774);
#46453=AXIS2_PLACEMENT_3D('',#74911,#53776,#53777);
#46454=AXIS2_PLACEMENT_3D('',#74912,#53778,#53779);
#46455=AXIS2_PLACEMENT_3D('',#74914,#53780,#53781);
#46456=AXIS2_PLACEMENT_3D('',#74917,#53783,#53784);
#46457=AXIS2_PLACEMENT_3D('',#74918,#53785,#53786);
#46458=AXIS2_PLACEMENT_3D('',#74920,#53787,#53788);
#46459=AXIS2_PLACEMENT_3D('',#74935,#53790,#53791);
#46460=AXIS2_PLACEMENT_3D('',#74959,#53792,#53793);
#46461=AXIS2_PLACEMENT_3D('',#74961,#53794,#53795);
#46462=AXIS2_PLACEMENT_3D('',#74964,#53797,#53798);
#46463=AXIS2_PLACEMENT_3D('',#74965,#53799,#53800);
#46464=AXIS2_PLACEMENT_3D('',#74967,#53801,#53802);
#46465=AXIS2_PLACEMENT_3D('',#74970,#53804,#53805);
#46466=AXIS2_PLACEMENT_3D('',#74971,#53806,#53807);
#46467=AXIS2_PLACEMENT_3D('',#74973,#53808,#53809);
#46468=AXIS2_PLACEMENT_3D('',#74976,#53811,#53812);
#46469=AXIS2_PLACEMENT_3D('',#74977,#53813,#53814);
#46470=AXIS2_PLACEMENT_3D('',#74979,#53815,#53816);
#46471=AXIS2_PLACEMENT_3D('',#74982,#53818,#53819);
#46472=AXIS2_PLACEMENT_3D('',#74983,#53820,#53821);
#46473=AXIS2_PLACEMENT_3D('',#74985,#53822,#53823);
#46474=AXIS2_PLACEMENT_3D('',#74988,#53825,#53826);
#46475=AXIS2_PLACEMENT_3D('',#74989,#53827,#53828);
#46476=AXIS2_PLACEMENT_3D('',#74991,#53829,#53830);
#46477=AXIS2_PLACEMENT_3D('',#74994,#53832,#53833);
#46478=AXIS2_PLACEMENT_3D('',#74995,#53834,#53835);
#46479=AXIS2_PLACEMENT_3D('',#74997,#53836,#53837);
#46480=AXIS2_PLACEMENT_3D('',#75000,#53839,#53840);
#46481=AXIS2_PLACEMENT_3D('',#75001,#53841,#53842);
#46482=AXIS2_PLACEMENT_3D('',#75003,#53843,#53844);
#46483=AXIS2_PLACEMENT_3D('',#75006,#53846,#53847);
#46484=AXIS2_PLACEMENT_3D('',#75007,#53848,#53849);
#46485=AXIS2_PLACEMENT_3D('',#75009,#53850,#53851);
#46486=AXIS2_PLACEMENT_3D('',#75012,#53853,#53854);
#46487=AXIS2_PLACEMENT_3D('',#75013,#53855,#53856);
#46488=AXIS2_PLACEMENT_3D('',#75015,#53857,#53858);
#46489=AXIS2_PLACEMENT_3D('',#75018,#53860,#53861);
#46490=AXIS2_PLACEMENT_3D('',#75019,#53862,#53863);
#46491=AXIS2_PLACEMENT_3D('',#75021,#53864,#53865);
#46492=AXIS2_PLACEMENT_3D('',#75024,#53867,#53868);
#46493=AXIS2_PLACEMENT_3D('',#75025,#53869,#53870);
#46494=AXIS2_PLACEMENT_3D('',#75027,#53871,#53872);
#46495=AXIS2_PLACEMENT_3D('',#75030,#53874,#53875);
#46496=AXIS2_PLACEMENT_3D('',#75031,#53876,#53877);
#46497=AXIS2_PLACEMENT_3D('',#75033,#53878,#53879);
#46498=AXIS2_PLACEMENT_3D('',#75036,#53881,#53882);
#46499=AXIS2_PLACEMENT_3D('',#75037,#53883,#53884);
#46500=AXIS2_PLACEMENT_3D('',#75039,#53885,#53886);
#46501=AXIS2_PLACEMENT_3D('',#75042,#53888,#53889);
#46502=AXIS2_PLACEMENT_3D('',#75043,#53890,#53891);
#46503=AXIS2_PLACEMENT_3D('',#75045,#53892,#53893);
#46504=AXIS2_PLACEMENT_3D('',#75048,#53895,#53896);
#46505=AXIS2_PLACEMENT_3D('',#75049,#53897,#53898);
#46506=AXIS2_PLACEMENT_3D('',#75051,#53899,#53900);
#46507=AXIS2_PLACEMENT_3D('',#75066,#53902,#53903);
#46508=AXIS2_PLACEMENT_3D('',#75090,#53904,#53905);
#46509=AXIS2_PLACEMENT_3D('',#75092,#53906,#53907);
#46510=AXIS2_PLACEMENT_3D('',#75095,#53909,#53910);
#46511=AXIS2_PLACEMENT_3D('',#75096,#53911,#53912);
#46512=AXIS2_PLACEMENT_3D('',#75098,#53913,#53914);
#46513=AXIS2_PLACEMENT_3D('',#75101,#53916,#53917);
#46514=AXIS2_PLACEMENT_3D('',#75102,#53918,#53919);
#46515=AXIS2_PLACEMENT_3D('',#75104,#53920,#53921);
#46516=AXIS2_PLACEMENT_3D('',#75107,#53923,#53924);
#46517=AXIS2_PLACEMENT_3D('',#75108,#53925,#53926);
#46518=AXIS2_PLACEMENT_3D('',#75110,#53927,#53928);
#46519=AXIS2_PLACEMENT_3D('',#75113,#53930,#53931);
#46520=AXIS2_PLACEMENT_3D('',#75114,#53932,#53933);
#46521=AXIS2_PLACEMENT_3D('',#75116,#53934,#53935);
#46522=AXIS2_PLACEMENT_3D('',#75119,#53937,#53938);
#46523=AXIS2_PLACEMENT_3D('',#75120,#53939,#53940);
#46524=AXIS2_PLACEMENT_3D('',#75122,#53941,#53942);
#46525=AXIS2_PLACEMENT_3D('',#75125,#53944,#53945);
#46526=AXIS2_PLACEMENT_3D('',#75126,#53946,#53947);
#46527=AXIS2_PLACEMENT_3D('',#75128,#53948,#53949);
#46528=AXIS2_PLACEMENT_3D('',#75131,#53951,#53952);
#46529=AXIS2_PLACEMENT_3D('',#75132,#53953,#53954);
#46530=AXIS2_PLACEMENT_3D('',#75134,#53955,#53956);
#46531=AXIS2_PLACEMENT_3D('',#75137,#53958,#53959);
#46532=AXIS2_PLACEMENT_3D('',#75138,#53960,#53961);
#46533=AXIS2_PLACEMENT_3D('',#75140,#53962,#53963);
#46534=AXIS2_PLACEMENT_3D('',#75143,#53965,#53966);
#46535=AXIS2_PLACEMENT_3D('',#75144,#53967,#53968);
#46536=AXIS2_PLACEMENT_3D('',#75146,#53969,#53970);
#46537=AXIS2_PLACEMENT_3D('',#75149,#53972,#53973);
#46538=AXIS2_PLACEMENT_3D('',#75150,#53974,#53975);
#46539=AXIS2_PLACEMENT_3D('',#75152,#53976,#53977);
#46540=AXIS2_PLACEMENT_3D('',#75155,#53979,#53980);
#46541=AXIS2_PLACEMENT_3D('',#75156,#53981,#53982);
#46542=AXIS2_PLACEMENT_3D('',#75158,#53983,#53984);
#46543=AXIS2_PLACEMENT_3D('',#75161,#53986,#53987);
#46544=AXIS2_PLACEMENT_3D('',#75162,#53988,#53989);
#46545=AXIS2_PLACEMENT_3D('',#75164,#53990,#53991);
#46546=AXIS2_PLACEMENT_3D('',#75167,#53993,#53994);
#46547=AXIS2_PLACEMENT_3D('',#75168,#53995,#53996);
#46548=AXIS2_PLACEMENT_3D('',#75170,#53997,#53998);
#46549=AXIS2_PLACEMENT_3D('',#75173,#54000,#54001);
#46550=AXIS2_PLACEMENT_3D('',#75174,#54002,#54003);
#46551=AXIS2_PLACEMENT_3D('',#75176,#54004,#54005);
#46552=AXIS2_PLACEMENT_3D('',#75179,#54007,#54008);
#46553=AXIS2_PLACEMENT_3D('',#75180,#54009,#54010);
#46554=AXIS2_PLACEMENT_3D('',#75182,#54011,#54012);
#46555=AXIS2_PLACEMENT_3D('',#75185,#54014,#54015);
#46556=AXIS2_PLACEMENT_3D('',#75186,#54016,#54017);
#46557=AXIS2_PLACEMENT_3D('',#75188,#54018,#54019);
#46558=AXIS2_PLACEMENT_3D('',#75191,#54021,#54022);
#46559=AXIS2_PLACEMENT_3D('',#75192,#54023,#54024);
#46560=AXIS2_PLACEMENT_3D('',#75194,#54025,#54026);
#46561=AXIS2_PLACEMENT_3D('',#75207,#54028,#54029);
#46562=AXIS2_PLACEMENT_3D('',#75233,#54030,#54031);
#46563=AXIS2_PLACEMENT_3D('',#75235,#54032,#54033);
#46564=AXIS2_PLACEMENT_3D('',#75238,#54035,#54036);
#46565=AXIS2_PLACEMENT_3D('',#75239,#54037,#54038);
#46566=AXIS2_PLACEMENT_3D('',#75241,#54039,#54040);
#46567=AXIS2_PLACEMENT_3D('',#75244,#54042,#54043);
#46568=AXIS2_PLACEMENT_3D('',#75245,#54044,#54045);
#46569=AXIS2_PLACEMENT_3D('',#75247,#54046,#54047);
#46570=AXIS2_PLACEMENT_3D('',#75250,#54049,#54050);
#46571=AXIS2_PLACEMENT_3D('',#75251,#54051,#54052);
#46572=AXIS2_PLACEMENT_3D('',#75253,#54053,#54054);
#46573=AXIS2_PLACEMENT_3D('',#75256,#54056,#54057);
#46574=AXIS2_PLACEMENT_3D('',#75257,#54058,#54059);
#46575=AXIS2_PLACEMENT_3D('',#75259,#54060,#54061);
#46576=AXIS2_PLACEMENT_3D('',#75262,#54063,#54064);
#46577=AXIS2_PLACEMENT_3D('',#75263,#54065,#54066);
#46578=AXIS2_PLACEMENT_3D('',#75265,#54067,#54068);
#46579=AXIS2_PLACEMENT_3D('',#75268,#54070,#54071);
#46580=AXIS2_PLACEMENT_3D('',#75269,#54072,#54073);
#46581=AXIS2_PLACEMENT_3D('',#75271,#54074,#54075);
#46582=AXIS2_PLACEMENT_3D('',#75274,#54077,#54078);
#46583=AXIS2_PLACEMENT_3D('',#75275,#54079,#54080);
#46584=AXIS2_PLACEMENT_3D('',#75277,#54081,#54082);
#46585=AXIS2_PLACEMENT_3D('',#75280,#54084,#54085);
#46586=AXIS2_PLACEMENT_3D('',#75281,#54086,#54087);
#46587=AXIS2_PLACEMENT_3D('',#75283,#54088,#54089);
#46588=AXIS2_PLACEMENT_3D('',#75286,#54091,#54092);
#46589=AXIS2_PLACEMENT_3D('',#75287,#54093,#54094);
#46590=AXIS2_PLACEMENT_3D('',#75289,#54095,#54096);
#46591=AXIS2_PLACEMENT_3D('',#75292,#54098,#54099);
#46592=AXIS2_PLACEMENT_3D('',#75293,#54100,#54101);
#46593=AXIS2_PLACEMENT_3D('',#75295,#54102,#54103);
#46594=AXIS2_PLACEMENT_3D('',#75298,#54105,#54106);
#46595=AXIS2_PLACEMENT_3D('',#75299,#54107,#54108);
#46596=AXIS2_PLACEMENT_3D('',#75301,#54109,#54110);
#46597=AXIS2_PLACEMENT_3D('',#75304,#54112,#54113);
#46598=AXIS2_PLACEMENT_3D('',#75305,#54114,#54115);
#46599=AXIS2_PLACEMENT_3D('',#75307,#54116,#54117);
#46600=AXIS2_PLACEMENT_3D('',#75310,#54119,#54120);
#46601=AXIS2_PLACEMENT_3D('',#75311,#54121,#54122);
#46602=AXIS2_PLACEMENT_3D('',#75313,#54123,#54124);
#46603=AXIS2_PLACEMENT_3D('',#75316,#54126,#54127);
#46604=AXIS2_PLACEMENT_3D('',#75317,#54128,#54129);
#46605=AXIS2_PLACEMENT_3D('',#75319,#54130,#54131);
#46606=AXIS2_PLACEMENT_3D('',#75322,#54133,#54134);
#46607=AXIS2_PLACEMENT_3D('',#75323,#54135,#54136);
#46608=AXIS2_PLACEMENT_3D('',#75325,#54137,#54138);
#46609=AXIS2_PLACEMENT_3D('',#75328,#54140,#54141);
#46610=AXIS2_PLACEMENT_3D('',#75329,#54142,#54143);
#46611=AXIS2_PLACEMENT_3D('',#75331,#54144,#54145);
#46612=AXIS2_PLACEMENT_3D('',#75334,#54147,#54148);
#46613=AXIS2_PLACEMENT_3D('',#75335,#54149,#54150);
#46614=AXIS2_PLACEMENT_3D('',#75337,#54151,#54152);
#46615=AXIS2_PLACEMENT_3D('',#75350,#54154,#54155);
#46616=AXIS2_PLACEMENT_3D('',#75376,#54156,#54157);
#46617=AXIS2_PLACEMENT_3D('',#75378,#54158,#54159);
#46618=AXIS2_PLACEMENT_3D('',#75381,#54161,#54162);
#46619=AXIS2_PLACEMENT_3D('',#75382,#54163,#54164);
#46620=AXIS2_PLACEMENT_3D('',#75384,#54165,#54166);
#46621=AXIS2_PLACEMENT_3D('',#75387,#54168,#54169);
#46622=AXIS2_PLACEMENT_3D('',#75388,#54170,#54171);
#46623=AXIS2_PLACEMENT_3D('',#75390,#54172,#54173);
#46624=AXIS2_PLACEMENT_3D('',#75393,#54175,#54176);
#46625=AXIS2_PLACEMENT_3D('',#75394,#54177,#54178);
#46626=AXIS2_PLACEMENT_3D('',#75396,#54179,#54180);
#46627=AXIS2_PLACEMENT_3D('',#75399,#54182,#54183);
#46628=AXIS2_PLACEMENT_3D('',#75400,#54184,#54185);
#46629=AXIS2_PLACEMENT_3D('',#75402,#54186,#54187);
#46630=AXIS2_PLACEMENT_3D('',#75405,#54189,#54190);
#46631=AXIS2_PLACEMENT_3D('',#75406,#54191,#54192);
#46632=AXIS2_PLACEMENT_3D('',#75408,#54193,#54194);
#46633=AXIS2_PLACEMENT_3D('',#75411,#54196,#54197);
#46634=AXIS2_PLACEMENT_3D('',#75412,#54198,#54199);
#46635=AXIS2_PLACEMENT_3D('',#75414,#54200,#54201);
#46636=AXIS2_PLACEMENT_3D('',#75417,#54203,#54204);
#46637=AXIS2_PLACEMENT_3D('',#75418,#54205,#54206);
#46638=AXIS2_PLACEMENT_3D('',#75420,#54207,#54208);
#46639=AXIS2_PLACEMENT_3D('',#75423,#54210,#54211);
#46640=AXIS2_PLACEMENT_3D('',#75424,#54212,#54213);
#46641=AXIS2_PLACEMENT_3D('',#75426,#54214,#54215);
#46642=AXIS2_PLACEMENT_3D('',#75429,#54217,#54218);
#46643=AXIS2_PLACEMENT_3D('',#75430,#54219,#54220);
#46644=AXIS2_PLACEMENT_3D('',#75432,#54221,#54222);
#46645=AXIS2_PLACEMENT_3D('',#75435,#54224,#54225);
#46646=AXIS2_PLACEMENT_3D('',#75436,#54226,#54227);
#46647=AXIS2_PLACEMENT_3D('',#75438,#54228,#54229);
#46648=AXIS2_PLACEMENT_3D('',#75441,#54231,#54232);
#46649=AXIS2_PLACEMENT_3D('',#75442,#54233,#54234);
#46650=AXIS2_PLACEMENT_3D('',#75444,#54235,#54236);
#46651=AXIS2_PLACEMENT_3D('',#75447,#54238,#54239);
#46652=AXIS2_PLACEMENT_3D('',#75448,#54240,#54241);
#46653=AXIS2_PLACEMENT_3D('',#75450,#54242,#54243);
#46654=AXIS2_PLACEMENT_3D('',#75453,#54245,#54246);
#46655=AXIS2_PLACEMENT_3D('',#75454,#54247,#54248);
#46656=AXIS2_PLACEMENT_3D('',#75456,#54249,#54250);
#46657=AXIS2_PLACEMENT_3D('',#75459,#54252,#54253);
#46658=AXIS2_PLACEMENT_3D('',#75460,#54254,#54255);
#46659=AXIS2_PLACEMENT_3D('',#75462,#54256,#54257);
#46660=AXIS2_PLACEMENT_3D('',#75465,#54259,#54260);
#46661=AXIS2_PLACEMENT_3D('',#75466,#54261,#54262);
#46662=AXIS2_PLACEMENT_3D('',#75468,#54263,#54264);
#46663=AXIS2_PLACEMENT_3D('',#75471,#54266,#54267);
#46664=AXIS2_PLACEMENT_3D('',#75472,#54268,#54269);
#46665=AXIS2_PLACEMENT_3D('',#75474,#54270,#54271);
#46666=AXIS2_PLACEMENT_3D('',#75477,#54273,#54274);
#46667=AXIS2_PLACEMENT_3D('',#75478,#54275,#54276);
#46668=AXIS2_PLACEMENT_3D('',#75480,#54277,#54278);
#46669=AXIS2_PLACEMENT_3D('',#75491,#54280,#54281);
#46670=AXIS2_PLACEMENT_3D('',#75519,#54282,#54283);
#46671=AXIS2_PLACEMENT_3D('',#75521,#54284,#54285);
#46672=AXIS2_PLACEMENT_3D('',#75524,#54287,#54288);
#46673=AXIS2_PLACEMENT_3D('',#75525,#54289,#54290);
#46674=AXIS2_PLACEMENT_3D('',#75527,#54291,#54292);
#46675=AXIS2_PLACEMENT_3D('',#75530,#54294,#54295);
#46676=AXIS2_PLACEMENT_3D('',#75531,#54296,#54297);
#46677=AXIS2_PLACEMENT_3D('',#75533,#54298,#54299);
#46678=AXIS2_PLACEMENT_3D('',#75536,#54301,#54302);
#46679=AXIS2_PLACEMENT_3D('',#75537,#54303,#54304);
#46680=AXIS2_PLACEMENT_3D('',#75539,#54305,#54306);
#46681=AXIS2_PLACEMENT_3D('',#75542,#54308,#54309);
#46682=AXIS2_PLACEMENT_3D('',#75543,#54310,#54311);
#46683=AXIS2_PLACEMENT_3D('',#75545,#54312,#54313);
#46684=AXIS2_PLACEMENT_3D('',#75548,#54315,#54316);
#46685=AXIS2_PLACEMENT_3D('',#75549,#54317,#54318);
#46686=AXIS2_PLACEMENT_3D('',#75551,#54319,#54320);
#46687=AXIS2_PLACEMENT_3D('',#75554,#54322,#54323);
#46688=AXIS2_PLACEMENT_3D('',#75555,#54324,#54325);
#46689=AXIS2_PLACEMENT_3D('',#75557,#54326,#54327);
#46690=AXIS2_PLACEMENT_3D('',#75560,#54329,#54330);
#46691=AXIS2_PLACEMENT_3D('',#75561,#54331,#54332);
#46692=AXIS2_PLACEMENT_3D('',#75563,#54333,#54334);
#46693=AXIS2_PLACEMENT_3D('',#75566,#54336,#54337);
#46694=AXIS2_PLACEMENT_3D('',#75567,#54338,#54339);
#46695=AXIS2_PLACEMENT_3D('',#75569,#54340,#54341);
#46696=AXIS2_PLACEMENT_3D('',#75572,#54343,#54344);
#46697=AXIS2_PLACEMENT_3D('',#75573,#54345,#54346);
#46698=AXIS2_PLACEMENT_3D('',#75575,#54347,#54348);
#46699=AXIS2_PLACEMENT_3D('',#75578,#54350,#54351);
#46700=AXIS2_PLACEMENT_3D('',#75579,#54352,#54353);
#46701=AXIS2_PLACEMENT_3D('',#75581,#54354,#54355);
#46702=AXIS2_PLACEMENT_3D('',#75584,#54357,#54358);
#46703=AXIS2_PLACEMENT_3D('',#75585,#54359,#54360);
#46704=AXIS2_PLACEMENT_3D('',#75587,#54361,#54362);
#46705=AXIS2_PLACEMENT_3D('',#75590,#54364,#54365);
#46706=AXIS2_PLACEMENT_3D('',#75591,#54366,#54367);
#46707=AXIS2_PLACEMENT_3D('',#75593,#54368,#54369);
#46708=AXIS2_PLACEMENT_3D('',#75596,#54371,#54372);
#46709=AXIS2_PLACEMENT_3D('',#75597,#54373,#54374);
#46710=AXIS2_PLACEMENT_3D('',#75599,#54375,#54376);
#46711=AXIS2_PLACEMENT_3D('',#75602,#54378,#54379);
#46712=AXIS2_PLACEMENT_3D('',#75603,#54380,#54381);
#46713=AXIS2_PLACEMENT_3D('',#75605,#54382,#54383);
#46714=AXIS2_PLACEMENT_3D('',#75608,#54385,#54386);
#46715=AXIS2_PLACEMENT_3D('',#75609,#54387,#54388);
#46716=AXIS2_PLACEMENT_3D('',#75611,#54389,#54390);
#46717=AXIS2_PLACEMENT_3D('',#75614,#54392,#54393);
#46718=AXIS2_PLACEMENT_3D('',#75615,#54394,#54395);
#46719=AXIS2_PLACEMENT_3D('',#75617,#54396,#54397);
#46720=AXIS2_PLACEMENT_3D('',#75620,#54399,#54400);
#46721=AXIS2_PLACEMENT_3D('',#75621,#54401,#54402);
#46722=AXIS2_PLACEMENT_3D('',#75623,#54403,#54404);
#46723=AXIS2_PLACEMENT_3D('',#75632,#54406,#54407);
#46724=AXIS2_PLACEMENT_3D('',#75662,#54408,#54409);
#46725=AXIS2_PLACEMENT_3D('',#75664,#54410,#54411);
#46726=AXIS2_PLACEMENT_3D('',#75667,#54413,#54414);
#46727=AXIS2_PLACEMENT_3D('',#75668,#54415,#54416);
#46728=AXIS2_PLACEMENT_3D('',#75670,#54417,#54418);
#46729=AXIS2_PLACEMENT_3D('',#75673,#54420,#54421);
#46730=AXIS2_PLACEMENT_3D('',#75674,#54422,#54423);
#46731=AXIS2_PLACEMENT_3D('',#75676,#54424,#54425);
#46732=AXIS2_PLACEMENT_3D('',#75679,#54427,#54428);
#46733=AXIS2_PLACEMENT_3D('',#75680,#54429,#54430);
#46734=AXIS2_PLACEMENT_3D('',#75682,#54431,#54432);
#46735=AXIS2_PLACEMENT_3D('',#75685,#54434,#54435);
#46736=AXIS2_PLACEMENT_3D('',#75686,#54436,#54437);
#46737=AXIS2_PLACEMENT_3D('',#75688,#54438,#54439);
#46738=AXIS2_PLACEMENT_3D('',#75691,#54441,#54442);
#46739=AXIS2_PLACEMENT_3D('',#75692,#54443,#54444);
#46740=AXIS2_PLACEMENT_3D('',#75694,#54445,#54446);
#46741=AXIS2_PLACEMENT_3D('',#75697,#54448,#54449);
#46742=AXIS2_PLACEMENT_3D('',#75698,#54450,#54451);
#46743=AXIS2_PLACEMENT_3D('',#75700,#54452,#54453);
#46744=AXIS2_PLACEMENT_3D('',#75703,#54455,#54456);
#46745=AXIS2_PLACEMENT_3D('',#75704,#54457,#54458);
#46746=AXIS2_PLACEMENT_3D('',#75706,#54459,#54460);
#46747=AXIS2_PLACEMENT_3D('',#75709,#54462,#54463);
#46748=AXIS2_PLACEMENT_3D('',#75710,#54464,#54465);
#46749=AXIS2_PLACEMENT_3D('',#75712,#54466,#54467);
#46750=AXIS2_PLACEMENT_3D('',#75715,#54469,#54470);
#46751=AXIS2_PLACEMENT_3D('',#75716,#54471,#54472);
#46752=AXIS2_PLACEMENT_3D('',#75718,#54473,#54474);
#46753=AXIS2_PLACEMENT_3D('',#75721,#54476,#54477);
#46754=AXIS2_PLACEMENT_3D('',#75722,#54478,#54479);
#46755=AXIS2_PLACEMENT_3D('',#75724,#54480,#54481);
#46756=AXIS2_PLACEMENT_3D('',#75727,#54483,#54484);
#46757=AXIS2_PLACEMENT_3D('',#75728,#54485,#54486);
#46758=AXIS2_PLACEMENT_3D('',#75730,#54487,#54488);
#46759=AXIS2_PLACEMENT_3D('',#75733,#54490,#54491);
#46760=AXIS2_PLACEMENT_3D('',#75734,#54492,#54493);
#46761=AXIS2_PLACEMENT_3D('',#75736,#54494,#54495);
#46762=AXIS2_PLACEMENT_3D('',#75739,#54497,#54498);
#46763=AXIS2_PLACEMENT_3D('',#75740,#54499,#54500);
#46764=AXIS2_PLACEMENT_3D('',#75742,#54501,#54502);
#46765=AXIS2_PLACEMENT_3D('',#75745,#54504,#54505);
#46766=AXIS2_PLACEMENT_3D('',#75746,#54506,#54507);
#46767=AXIS2_PLACEMENT_3D('',#75748,#54508,#54509);
#46768=AXIS2_PLACEMENT_3D('',#75751,#54511,#54512);
#46769=AXIS2_PLACEMENT_3D('',#75752,#54513,#54514);
#46770=AXIS2_PLACEMENT_3D('',#75754,#54515,#54516);
#46771=AXIS2_PLACEMENT_3D('',#75763,#54518,#54519);
#46772=AXIS2_PLACEMENT_3D('',#75793,#54520,#54521);
#46773=AXIS2_PLACEMENT_3D('',#75795,#54522,#54523);
#46774=AXIS2_PLACEMENT_3D('',#75798,#54525,#54526);
#46775=AXIS2_PLACEMENT_3D('',#75799,#54527,#54528);
#46776=AXIS2_PLACEMENT_3D('',#75801,#54529,#54530);
#46777=AXIS2_PLACEMENT_3D('',#75804,#54532,#54533);
#46778=AXIS2_PLACEMENT_3D('',#75805,#54534,#54535);
#46779=AXIS2_PLACEMENT_3D('',#75807,#54536,#54537);
#46780=AXIS2_PLACEMENT_3D('',#75810,#54539,#54540);
#46781=AXIS2_PLACEMENT_3D('',#75811,#54541,#54542);
#46782=AXIS2_PLACEMENT_3D('',#75813,#54543,#54544);
#46783=AXIS2_PLACEMENT_3D('',#75816,#54546,#54547);
#46784=AXIS2_PLACEMENT_3D('',#75817,#54548,#54549);
#46785=AXIS2_PLACEMENT_3D('',#75819,#54550,#54551);
#46786=AXIS2_PLACEMENT_3D('',#75822,#54553,#54554);
#46787=AXIS2_PLACEMENT_3D('',#75823,#54555,#54556);
#46788=AXIS2_PLACEMENT_3D('',#75825,#54557,#54558);
#46789=AXIS2_PLACEMENT_3D('',#75828,#54560,#54561);
#46790=AXIS2_PLACEMENT_3D('',#75829,#54562,#54563);
#46791=AXIS2_PLACEMENT_3D('',#75831,#54564,#54565);
#46792=AXIS2_PLACEMENT_3D('',#75834,#54567,#54568);
#46793=AXIS2_PLACEMENT_3D('',#75835,#54569,#54570);
#46794=AXIS2_PLACEMENT_3D('',#75837,#54571,#54572);
#46795=AXIS2_PLACEMENT_3D('',#75840,#54574,#54575);
#46796=AXIS2_PLACEMENT_3D('',#75841,#54576,#54577);
#46797=AXIS2_PLACEMENT_3D('',#75843,#54578,#54579);
#46798=AXIS2_PLACEMENT_3D('',#75846,#54581,#54582);
#46799=AXIS2_PLACEMENT_3D('',#75847,#54583,#54584);
#46800=AXIS2_PLACEMENT_3D('',#75849,#54585,#54586);
#46801=AXIS2_PLACEMENT_3D('',#75852,#54588,#54589);
#46802=AXIS2_PLACEMENT_3D('',#75853,#54590,#54591);
#46803=AXIS2_PLACEMENT_3D('',#75855,#54592,#54593);
#46804=AXIS2_PLACEMENT_3D('',#75858,#54595,#54596);
#46805=AXIS2_PLACEMENT_3D('',#75859,#54597,#54598);
#46806=AXIS2_PLACEMENT_3D('',#75861,#54599,#54600);
#46807=AXIS2_PLACEMENT_3D('',#75864,#54602,#54603);
#46808=AXIS2_PLACEMENT_3D('',#75865,#54604,#54605);
#46809=AXIS2_PLACEMENT_3D('',#75867,#54606,#54607);
#46810=AXIS2_PLACEMENT_3D('',#75870,#54609,#54610);
#46811=AXIS2_PLACEMENT_3D('',#75871,#54611,#54612);
#46812=AXIS2_PLACEMENT_3D('',#75873,#54613,#54614);
#46813=AXIS2_PLACEMENT_3D('',#75876,#54616,#54617);
#46814=AXIS2_PLACEMENT_3D('',#75877,#54618,#54619);
#46815=AXIS2_PLACEMENT_3D('',#75879,#54620,#54621);
#46816=AXIS2_PLACEMENT_3D('',#75882,#54623,#54624);
#46817=AXIS2_PLACEMENT_3D('',#75883,#54625,#54626);
#46818=AXIS2_PLACEMENT_3D('',#75885,#54627,#54628);
#46819=AXIS2_PLACEMENT_3D('',#75888,#54630,#54631);
#46820=AXIS2_PLACEMENT_3D('',#75889,#54632,#54633);
#46821=AXIS2_PLACEMENT_3D('',#75891,#54634,#54635);
#46822=AXIS2_PLACEMENT_3D('',#75894,#54637,#54638);
#46823=AXIS2_PLACEMENT_3D('',#75895,#54639,#54640);
#46824=AXIS2_PLACEMENT_3D('',#75897,#54641,#54642);
#46825=AXIS2_PLACEMENT_3D('',#75901,#54644,#54645);
#46826=AXIS2_PLACEMENT_3D('',#75932,#54646,#54647);
#46827=AXIS2_PLACEMENT_3D('',#75933,#54648,#54649);
#46828=AXIS2_PLACEMENT_3D('',#75935,#54650,#54651);
#46829=AXIS2_PLACEMENT_3D('',#75938,#54653,#54654);
#46830=AXIS2_PLACEMENT_3D('',#75939,#54655,#54656);
#46831=AXIS2_PLACEMENT_3D('',#75941,#54657,#54658);
#46832=AXIS2_PLACEMENT_3D('',#75944,#54660,#54661);
#46833=AXIS2_PLACEMENT_3D('',#75945,#54662,#54663);
#46834=AXIS2_PLACEMENT_3D('',#75947,#54664,#54665);
#46835=AXIS2_PLACEMENT_3D('',#75950,#54667,#54668);
#46836=AXIS2_PLACEMENT_3D('',#75951,#54669,#54670);
#46837=AXIS2_PLACEMENT_3D('',#75953,#54671,#54672);
#46838=AXIS2_PLACEMENT_3D('',#75956,#54674,#54675);
#46839=AXIS2_PLACEMENT_3D('',#75957,#54676,#54677);
#46840=AXIS2_PLACEMENT_3D('',#75959,#54678,#54679);
#46841=AXIS2_PLACEMENT_3D('',#75962,#54681,#54682);
#46842=AXIS2_PLACEMENT_3D('',#75963,#54683,#54684);
#46843=AXIS2_PLACEMENT_3D('',#75965,#54685,#54686);
#46844=AXIS2_PLACEMENT_3D('',#75968,#54688,#54689);
#46845=AXIS2_PLACEMENT_3D('',#75969,#54690,#54691);
#46846=AXIS2_PLACEMENT_3D('',#75971,#54692,#54693);
#46847=AXIS2_PLACEMENT_3D('',#75974,#54695,#54696);
#46848=AXIS2_PLACEMENT_3D('',#75975,#54697,#54698);
#46849=AXIS2_PLACEMENT_3D('',#75977,#54699,#54700);
#46850=AXIS2_PLACEMENT_3D('',#75980,#54702,#54703);
#46851=AXIS2_PLACEMENT_3D('',#75981,#54704,#54705);
#46852=AXIS2_PLACEMENT_3D('',#75983,#54706,#54707);
#46853=AXIS2_PLACEMENT_3D('',#75986,#54709,#54710);
#46854=AXIS2_PLACEMENT_3D('',#75987,#54711,#54712);
#46855=AXIS2_PLACEMENT_3D('',#75989,#54713,#54714);
#46856=AXIS2_PLACEMENT_3D('',#75992,#54716,#54717);
#46857=AXIS2_PLACEMENT_3D('',#75993,#54718,#54719);
#46858=AXIS2_PLACEMENT_3D('',#75995,#54720,#54721);
#46859=AXIS2_PLACEMENT_3D('',#75998,#54723,#54724);
#46860=AXIS2_PLACEMENT_3D('',#75999,#54725,#54726);
#46861=AXIS2_PLACEMENT_3D('',#76001,#54727,#54728);
#46862=AXIS2_PLACEMENT_3D('',#76004,#54730,#54731);
#46863=AXIS2_PLACEMENT_3D('',#76005,#54732,#54733);
#46864=AXIS2_PLACEMENT_3D('',#76007,#54734,#54735);
#46865=AXIS2_PLACEMENT_3D('',#76010,#54737,#54738);
#46866=AXIS2_PLACEMENT_3D('',#76011,#54739,#54740);
#46867=AXIS2_PLACEMENT_3D('',#76013,#54741,#54742);
#46868=AXIS2_PLACEMENT_3D('',#76016,#54744,#54745);
#46869=AXIS2_PLACEMENT_3D('',#76017,#54746,#54747);
#46870=AXIS2_PLACEMENT_3D('',#76019,#54748,#54749);
#46871=AXIS2_PLACEMENT_3D('',#76022,#54751,#54752);
#46872=AXIS2_PLACEMENT_3D('',#76023,#54753,#54754);
#46873=AXIS2_PLACEMENT_3D('',#76025,#54755,#54756);
#46874=AXIS2_PLACEMENT_3D('',#76029,#54758,#54759);
#46875=AXIS2_PLACEMENT_3D('',#76043,#54760,#54761);
#46876=AXIS2_PLACEMENT_3D('',#76044,#54762,#54763);
#46877=AXIS2_PLACEMENT_3D('',#76046,#54764,#54765);
#46878=AXIS2_PLACEMENT_3D('',#76049,#54767,#54768);
#46879=AXIS2_PLACEMENT_3D('',#76050,#54769,#54770);
#46880=AXIS2_PLACEMENT_3D('',#76052,#54771,#54772);
#46881=AXIS2_PLACEMENT_3D('',#76056,#54774,#54775);
#46882=AXIS2_PLACEMENT_3D('',#76094,#54776,#54777);
#46883=AXIS2_PLACEMENT_3D('',#76095,#54778,#54779);
#46884=AXIS2_PLACEMENT_3D('',#76097,#54780,#54781);
#46885=AXIS2_PLACEMENT_3D('',#76100,#54783,#54784);
#46886=AXIS2_PLACEMENT_3D('',#76101,#54785,#54786);
#46887=AXIS2_PLACEMENT_3D('',#76103,#54787,#54788);
#46888=AXIS2_PLACEMENT_3D('',#76106,#54790,#54791);
#46889=AXIS2_PLACEMENT_3D('',#76107,#54792,#54793);
#46890=AXIS2_PLACEMENT_3D('',#76109,#54794,#54795);
#46891=AXIS2_PLACEMENT_3D('',#76112,#54797,#54798);
#46892=AXIS2_PLACEMENT_3D('',#76113,#54799,#54800);
#46893=AXIS2_PLACEMENT_3D('',#76115,#54801,#54802);
#46894=AXIS2_PLACEMENT_3D('',#76118,#54804,#54805);
#46895=AXIS2_PLACEMENT_3D('',#76119,#54806,#54807);
#46896=AXIS2_PLACEMENT_3D('',#76121,#54808,#54809);
#46897=AXIS2_PLACEMENT_3D('',#76124,#54811,#54812);
#46898=AXIS2_PLACEMENT_3D('',#76125,#54813,#54814);
#46899=AXIS2_PLACEMENT_3D('',#76127,#54815,#54816);
#46900=AXIS2_PLACEMENT_3D('',#76130,#54818,#54819);
#46901=AXIS2_PLACEMENT_3D('',#76131,#54820,#54821);
#46902=AXIS2_PLACEMENT_3D('',#76133,#54822,#54823);
#46903=AXIS2_PLACEMENT_3D('',#76136,#54825,#54826);
#46904=AXIS2_PLACEMENT_3D('',#76137,#54827,#54828);
#46905=AXIS2_PLACEMENT_3D('',#76139,#54829,#54830);
#46906=AXIS2_PLACEMENT_3D('',#76142,#54832,#54833);
#46907=AXIS2_PLACEMENT_3D('',#76143,#54834,#54835);
#46908=AXIS2_PLACEMENT_3D('',#76145,#54836,#54837);
#46909=AXIS2_PLACEMENT_3D('',#76148,#54839,#54840);
#46910=AXIS2_PLACEMENT_3D('',#76149,#54841,#54842);
#46911=AXIS2_PLACEMENT_3D('',#76151,#54843,#54844);
#46912=AXIS2_PLACEMENT_3D('',#76154,#54846,#54847);
#46913=AXIS2_PLACEMENT_3D('',#76155,#54848,#54849);
#46914=AXIS2_PLACEMENT_3D('',#76157,#54850,#54851);
#46915=AXIS2_PLACEMENT_3D('',#76160,#54853,#54854);
#46916=AXIS2_PLACEMENT_3D('',#76161,#54855,#54856);
#46917=AXIS2_PLACEMENT_3D('',#76163,#54857,#54858);
#46918=AXIS2_PLACEMENT_3D('',#76166,#54860,#54861);
#46919=AXIS2_PLACEMENT_3D('',#76167,#54862,#54863);
#46920=AXIS2_PLACEMENT_3D('',#76169,#54864,#54865);
#46921=AXIS2_PLACEMENT_3D('',#76172,#54867,#54868);
#46922=AXIS2_PLACEMENT_3D('',#76173,#54869,#54870);
#46923=AXIS2_PLACEMENT_3D('',#76175,#54871,#54872);
#46924=AXIS2_PLACEMENT_3D('',#76179,#54874,#54875);
#46925=AXIS2_PLACEMENT_3D('',#76195,#54876,#54877);
#46926=AXIS2_PLACEMENT_3D('',#76196,#54878,#54879);
#46927=AXIS2_PLACEMENT_3D('',#76198,#54880,#54881);
#46928=AXIS2_PLACEMENT_3D('',#76201,#54883,#54884);
#46929=AXIS2_PLACEMENT_3D('',#76202,#54885,#54886);
#46930=AXIS2_PLACEMENT_3D('',#76204,#54887,#54888);
#46931=AXIS2_PLACEMENT_3D('',#76207,#54890,#54891);
#46932=AXIS2_PLACEMENT_3D('',#76208,#54892,#54893);
#46933=AXIS2_PLACEMENT_3D('',#76210,#54894,#54895);
#46934=AXIS2_PLACEMENT_3D('',#76213,#54897,#54898);
#46935=AXIS2_PLACEMENT_3D('',#76214,#54899,#54900);
#46936=AXIS2_PLACEMENT_3D('',#76216,#54901,#54902);
#46937=AXIS2_PLACEMENT_3D('',#76219,#54904,#54905);
#46938=AXIS2_PLACEMENT_3D('',#76220,#54906,#54907);
#46939=AXIS2_PLACEMENT_3D('',#76222,#54908,#54909);
#46940=AXIS2_PLACEMENT_3D('',#76225,#54911,#54912);
#46941=AXIS2_PLACEMENT_3D('',#76226,#54913,#54914);
#46942=AXIS2_PLACEMENT_3D('',#76228,#54915,#54916);
#46943=AXIS2_PLACEMENT_3D('',#76231,#54918,#54919);
#46944=AXIS2_PLACEMENT_3D('',#76232,#54920,#54921);
#46945=AXIS2_PLACEMENT_3D('',#76234,#54922,#54923);
#46946=AXIS2_PLACEMENT_3D('',#76237,#54925,#54926);
#46947=AXIS2_PLACEMENT_3D('',#76238,#54927,#54928);
#46948=AXIS2_PLACEMENT_3D('',#76240,#54929,#54930);
#46949=AXIS2_PLACEMENT_3D('',#76243,#54932,#54933);
#46950=AXIS2_PLACEMENT_3D('',#76244,#54934,#54935);
#46951=AXIS2_PLACEMENT_3D('',#76246,#54936,#54937);
#46952=AXIS2_PLACEMENT_3D('',#76249,#54939,#54940);
#46953=AXIS2_PLACEMENT_3D('',#76250,#54941,#54942);
#46954=AXIS2_PLACEMENT_3D('',#76252,#54943,#54944);
#46955=AXIS2_PLACEMENT_3D('',#76255,#54946,#54947);
#46956=AXIS2_PLACEMENT_3D('',#76256,#54948,#54949);
#46957=AXIS2_PLACEMENT_3D('',#76258,#54950,#54951);
#46958=AXIS2_PLACEMENT_3D('',#76261,#54953,#54954);
#46959=AXIS2_PLACEMENT_3D('',#76262,#54955,#54956);
#46960=AXIS2_PLACEMENT_3D('',#76264,#54957,#54958);
#46961=AXIS2_PLACEMENT_3D('',#76267,#54960,#54961);
#46962=AXIS2_PLACEMENT_3D('',#76268,#54962,#54963);
#46963=AXIS2_PLACEMENT_3D('',#76270,#54964,#54965);
#46964=AXIS2_PLACEMENT_3D('',#76273,#54967,#54968);
#46965=AXIS2_PLACEMENT_3D('',#76274,#54969,#54970);
#46966=AXIS2_PLACEMENT_3D('',#76276,#54971,#54972);
#46967=AXIS2_PLACEMENT_3D('',#76279,#54974,#54975);
#46968=AXIS2_PLACEMENT_3D('',#76280,#54976,#54977);
#46969=AXIS2_PLACEMENT_3D('',#76282,#54978,#54979);
#46970=AXIS2_PLACEMENT_3D('',#76285,#54981,#54982);
#46971=AXIS2_PLACEMENT_3D('',#76286,#54983,#54984);
#46972=AXIS2_PLACEMENT_3D('',#76288,#54985,#54986);
#46973=AXIS2_PLACEMENT_3D('',#76291,#54988,#54989);
#46974=AXIS2_PLACEMENT_3D('',#76292,#54990,#54991);
#46975=AXIS2_PLACEMENT_3D('',#76294,#54992,#54993);
#46976=AXIS2_PLACEMENT_3D('',#76297,#54995,#54996);
#46977=AXIS2_PLACEMENT_3D('',#76298,#54997,#54998);
#46978=AXIS2_PLACEMENT_3D('',#76300,#54999,#55000);
#46979=AXIS2_PLACEMENT_3D('',#76303,#55002,#55003);
#46980=AXIS2_PLACEMENT_3D('',#76304,#55004,#55005);
#46981=AXIS2_PLACEMENT_3D('',#76306,#55006,#55007);
#46982=AXIS2_PLACEMENT_3D('',#76309,#55009,#55010);
#46983=AXIS2_PLACEMENT_3D('',#76310,#55011,#55012);
#46984=AXIS2_PLACEMENT_3D('',#76312,#55013,#55014);
#46985=AXIS2_PLACEMENT_3D('',#76315,#55016,#55017);
#46986=AXIS2_PLACEMENT_3D('',#76316,#55018,#55019);
#46987=AXIS2_PLACEMENT_3D('',#76318,#55020,#55021);
#46988=AXIS2_PLACEMENT_3D('',#76321,#55023,#55024);
#46989=AXIS2_PLACEMENT_3D('',#76322,#55025,#55026);
#46990=AXIS2_PLACEMENT_3D('',#76324,#55027,#55028);
#46991=AXIS2_PLACEMENT_3D('',#76327,#55030,#55031);
#46992=AXIS2_PLACEMENT_3D('',#76328,#55032,#55033);
#46993=AXIS2_PLACEMENT_3D('',#76330,#55034,#55035);
#46994=AXIS2_PLACEMENT_3D('',#76333,#55037,#55038);
#46995=AXIS2_PLACEMENT_3D('',#76334,#55039,#55040);
#46996=AXIS2_PLACEMENT_3D('',#76336,#55041,#55042);
#46997=AXIS2_PLACEMENT_3D('',#76339,#55044,#55045);
#46998=AXIS2_PLACEMENT_3D('',#76340,#55046,#55047);
#46999=AXIS2_PLACEMENT_3D('',#76342,#55048,#55049);
#47000=AXIS2_PLACEMENT_3D('',#76345,#55051,#55052);
#47001=AXIS2_PLACEMENT_3D('',#76346,#55053,#55054);
#47002=AXIS2_PLACEMENT_3D('',#76348,#55055,#55056);
#47003=AXIS2_PLACEMENT_3D('',#76351,#55058,#55059);
#47004=AXIS2_PLACEMENT_3D('',#76352,#55060,#55061);
#47005=AXIS2_PLACEMENT_3D('',#76354,#55062,#55063);
#47006=AXIS2_PLACEMENT_3D('',#76357,#55065,#55066);
#47007=AXIS2_PLACEMENT_3D('',#76358,#55067,#55068);
#47008=AXIS2_PLACEMENT_3D('',#76360,#55069,#55070);
#47009=AXIS2_PLACEMENT_3D('',#76364,#55072,#55073);
#47010=AXIS2_PLACEMENT_3D('',#76390,#55074,#55075);
#47011=AXIS2_PLACEMENT_3D('',#76391,#55076,#55077);
#47012=AXIS2_PLACEMENT_3D('',#76393,#55078,#55079);
#47013=AXIS2_PLACEMENT_3D('',#76396,#55081,#55082);
#47014=AXIS2_PLACEMENT_3D('',#76397,#55083,#55084);
#47015=AXIS2_PLACEMENT_3D('',#76399,#55085,#55086);
#47016=AXIS2_PLACEMENT_3D('',#76402,#55088,#55089);
#47017=AXIS2_PLACEMENT_3D('',#76403,#55090,#55091);
#47018=AXIS2_PLACEMENT_3D('',#76405,#55092,#55093);
#47019=AXIS2_PLACEMENT_3D('',#76408,#55095,#55096);
#47020=AXIS2_PLACEMENT_3D('',#76409,#55097,#55098);
#47021=AXIS2_PLACEMENT_3D('',#76411,#55099,#55100);
#47022=AXIS2_PLACEMENT_3D('',#76414,#55102,#55103);
#47023=AXIS2_PLACEMENT_3D('',#76415,#55104,#55105);
#47024=AXIS2_PLACEMENT_3D('',#76417,#55106,#55107);
#47025=AXIS2_PLACEMENT_3D('',#76420,#55109,#55110);
#47026=AXIS2_PLACEMENT_3D('',#76421,#55111,#55112);
#47027=AXIS2_PLACEMENT_3D('',#76423,#55113,#55114);
#47028=AXIS2_PLACEMENT_3D('',#76426,#55116,#55117);
#47029=AXIS2_PLACEMENT_3D('',#76427,#55118,#55119);
#47030=AXIS2_PLACEMENT_3D('',#76429,#55120,#55121);
#47031=AXIS2_PLACEMENT_3D('',#76432,#55123,#55124);
#47032=AXIS2_PLACEMENT_3D('',#76433,#55125,#55126);
#47033=AXIS2_PLACEMENT_3D('',#76435,#55127,#55128);
#47034=AXIS2_PLACEMENT_3D('',#76438,#55130,#55131);
#47035=AXIS2_PLACEMENT_3D('',#76439,#55132,#55133);
#47036=AXIS2_PLACEMENT_3D('',#76441,#55134,#55135);
#47037=AXIS2_PLACEMENT_3D('',#76444,#55137,#55138);
#47038=AXIS2_PLACEMENT_3D('',#76445,#55139,#55140);
#47039=AXIS2_PLACEMENT_3D('',#76447,#55141,#55142);
#47040=AXIS2_PLACEMENT_3D('',#76450,#55144,#55145);
#47041=AXIS2_PLACEMENT_3D('',#76451,#55146,#55147);
#47042=AXIS2_PLACEMENT_3D('',#76453,#55148,#55149);
#47043=AXIS2_PLACEMENT_3D('',#76456,#55151,#55152);
#47044=AXIS2_PLACEMENT_3D('',#76457,#55153,#55154);
#47045=AXIS2_PLACEMENT_3D('',#76459,#55155,#55156);
#47046=AXIS2_PLACEMENT_3D('',#76462,#55158,#55159);
#47047=AXIS2_PLACEMENT_3D('',#76463,#55160,#55161);
#47048=AXIS2_PLACEMENT_3D('',#76465,#55162,#55163);
#47049=AXIS2_PLACEMENT_3D('',#76468,#55165,#55166);
#47050=AXIS2_PLACEMENT_3D('',#76469,#55167,#55168);
#47051=AXIS2_PLACEMENT_3D('',#76471,#55169,#55170);
#47052=AXIS2_PLACEMENT_3D('',#76474,#55172,#55173);
#47053=AXIS2_PLACEMENT_3D('',#76475,#55174,#55175);
#47054=AXIS2_PLACEMENT_3D('',#76477,#55176,#55177);
#47055=AXIS2_PLACEMENT_3D('',#76480,#55179,#55180);
#47056=AXIS2_PLACEMENT_3D('',#76481,#55181,#55182);
#47057=AXIS2_PLACEMENT_3D('',#76483,#55183,#55184);
#47058=AXIS2_PLACEMENT_3D('',#76486,#55186,#55187);
#47059=AXIS2_PLACEMENT_3D('',#76487,#55188,#55189);
#47060=AXIS2_PLACEMENT_3D('',#76489,#55190,#55191);
#47061=AXIS2_PLACEMENT_3D('',#76492,#55193,#55194);
#47062=AXIS2_PLACEMENT_3D('',#76493,#55195,#55196);
#47063=AXIS2_PLACEMENT_3D('',#76495,#55197,#55198);
#47064=AXIS2_PLACEMENT_3D('',#76498,#55200,#55201);
#47065=AXIS2_PLACEMENT_3D('',#76499,#55202,#55203);
#47066=AXIS2_PLACEMENT_3D('',#76501,#55204,#55205);
#47067=AXIS2_PLACEMENT_3D('',#76504,#55207,#55208);
#47068=AXIS2_PLACEMENT_3D('',#76505,#55209,#55210);
#47069=AXIS2_PLACEMENT_3D('',#76507,#55211,#55212);
#47070=AXIS2_PLACEMENT_3D('',#76510,#55214,#55215);
#47071=AXIS2_PLACEMENT_3D('',#76511,#55216,#55217);
#47072=AXIS2_PLACEMENT_3D('',#76513,#55218,#55219);
#47073=AXIS2_PLACEMENT_3D('',#76516,#55221,#55222);
#47074=AXIS2_PLACEMENT_3D('',#76517,#55223,#55224);
#47075=AXIS2_PLACEMENT_3D('',#76519,#55225,#55226);
#47076=AXIS2_PLACEMENT_3D('',#76522,#55228,#55229);
#47077=AXIS2_PLACEMENT_3D('',#76523,#55230,#55231);
#47078=AXIS2_PLACEMENT_3D('',#76525,#55232,#55233);
#47079=AXIS2_PLACEMENT_3D('',#76528,#55235,#55236);
#47080=AXIS2_PLACEMENT_3D('',#76529,#55237,#55238);
#47081=AXIS2_PLACEMENT_3D('',#76531,#55239,#55240);
#47082=AXIS2_PLACEMENT_3D('',#76534,#55242,#55243);
#47083=AXIS2_PLACEMENT_3D('',#76535,#55244,#55245);
#47084=AXIS2_PLACEMENT_3D('',#76537,#55246,#55247);
#47085=AXIS2_PLACEMENT_3D('',#76540,#55249,#55250);
#47086=AXIS2_PLACEMENT_3D('',#76541,#55251,#55252);
#47087=AXIS2_PLACEMENT_3D('',#76543,#55253,#55254);
#47088=AXIS2_PLACEMENT_3D('',#76546,#55256,#55257);
#47089=AXIS2_PLACEMENT_3D('',#76547,#55258,#55259);
#47090=AXIS2_PLACEMENT_3D('',#76549,#55260,#55261);
#47091=AXIS2_PLACEMENT_3D('',#76552,#55263,#55264);
#47092=AXIS2_PLACEMENT_3D('',#76553,#55265,#55266);
#47093=AXIS2_PLACEMENT_3D('',#76555,#55267,#55268);
#47094=AXIS2_PLACEMENT_3D('',#76558,#55270,#55271);
#47095=AXIS2_PLACEMENT_3D('',#76559,#55272,#55273);
#47096=AXIS2_PLACEMENT_3D('',#76561,#55274,#55275);
#47097=AXIS2_PLACEMENT_3D('',#76564,#55277,#55278);
#47098=AXIS2_PLACEMENT_3D('',#76565,#55279,#55280);
#47099=AXIS2_PLACEMENT_3D('',#76567,#55281,#55282);
#47100=AXIS2_PLACEMENT_3D('',#76570,#55284,#55285);
#47101=AXIS2_PLACEMENT_3D('',#76571,#55286,#55287);
#47102=AXIS2_PLACEMENT_3D('',#76573,#55288,#55289);
#47103=AXIS2_PLACEMENT_3D('',#76576,#55291,#55292);
#47104=AXIS2_PLACEMENT_3D('',#76577,#55293,#55294);
#47105=AXIS2_PLACEMENT_3D('',#76579,#55295,#55296);
#47106=AXIS2_PLACEMENT_3D('',#76582,#55298,#55299);
#47107=AXIS2_PLACEMENT_3D('',#76583,#55300,#55301);
#47108=AXIS2_PLACEMENT_3D('',#76585,#55302,#55303);
#47109=AXIS2_PLACEMENT_3D('',#76588,#55305,#55306);
#47110=AXIS2_PLACEMENT_3D('',#76589,#55307,#55308);
#47111=AXIS2_PLACEMENT_3D('',#76591,#55309,#55310);
#47112=AXIS2_PLACEMENT_3D('',#76595,#55312,#55313);
#47113=AXIS2_PLACEMENT_3D('',#76636,#55314,#55315);
#47114=AXIS2_PLACEMENT_3D('',#76637,#55316,#55317);
#47115=AXIS2_PLACEMENT_3D('',#76639,#55318,#55319);
#47116=AXIS2_PLACEMENT_3D('',#76642,#55321,#55322);
#47117=AXIS2_PLACEMENT_3D('',#76643,#55323,#55324);
#47118=AXIS2_PLACEMENT_3D('',#76645,#55325,#55326);
#47119=AXIS2_PLACEMENT_3D('',#76648,#55328,#55329);
#47120=AXIS2_PLACEMENT_3D('',#76649,#55330,#55331);
#47121=AXIS2_PLACEMENT_3D('',#76651,#55332,#55333);
#47122=AXIS2_PLACEMENT_3D('',#76654,#55335,#55336);
#47123=AXIS2_PLACEMENT_3D('',#76655,#55337,#55338);
#47124=AXIS2_PLACEMENT_3D('',#76657,#55339,#55340);
#47125=AXIS2_PLACEMENT_3D('',#76660,#55342,#55343);
#47126=AXIS2_PLACEMENT_3D('',#76661,#55344,#55345);
#47127=AXIS2_PLACEMENT_3D('',#76663,#55346,#55347);
#47128=AXIS2_PLACEMENT_3D('',#76666,#55349,#55350);
#47129=AXIS2_PLACEMENT_3D('',#76667,#55351,#55352);
#47130=AXIS2_PLACEMENT_3D('',#76669,#55353,#55354);
#47131=AXIS2_PLACEMENT_3D('',#76672,#55356,#55357);
#47132=AXIS2_PLACEMENT_3D('',#76673,#55358,#55359);
#47133=AXIS2_PLACEMENT_3D('',#76675,#55360,#55361);
#47134=AXIS2_PLACEMENT_3D('',#76678,#55363,#55364);
#47135=AXIS2_PLACEMENT_3D('',#76679,#55365,#55366);
#47136=AXIS2_PLACEMENT_3D('',#76681,#55367,#55368);
#47137=AXIS2_PLACEMENT_3D('',#76684,#55370,#55371);
#47138=AXIS2_PLACEMENT_3D('',#76685,#55372,#55373);
#47139=AXIS2_PLACEMENT_3D('',#76687,#55374,#55375);
#47140=AXIS2_PLACEMENT_3D('',#76690,#55377,#55378);
#47141=AXIS2_PLACEMENT_3D('',#76691,#55379,#55380);
#47142=AXIS2_PLACEMENT_3D('',#76693,#55381,#55382);
#47143=AXIS2_PLACEMENT_3D('',#76696,#55384,#55385);
#47144=AXIS2_PLACEMENT_3D('',#76697,#55386,#55387);
#47145=AXIS2_PLACEMENT_3D('',#76699,#55388,#55389);
#47146=AXIS2_PLACEMENT_3D('',#76702,#55391,#55392);
#47147=AXIS2_PLACEMENT_3D('',#76703,#55393,#55394);
#47148=AXIS2_PLACEMENT_3D('',#76705,#55395,#55396);
#47149=AXIS2_PLACEMENT_3D('',#76708,#55398,#55399);
#47150=AXIS2_PLACEMENT_3D('',#76709,#55400,#55401);
#47151=AXIS2_PLACEMENT_3D('',#76711,#55402,#55403);
#47152=AXIS2_PLACEMENT_3D('',#76714,#55405,#55406);
#47153=AXIS2_PLACEMENT_3D('',#76715,#55407,#55408);
#47154=AXIS2_PLACEMENT_3D('',#76717,#55409,#55410);
#47155=AXIS2_PLACEMENT_3D('',#76720,#55412,#55413);
#47156=AXIS2_PLACEMENT_3D('',#76721,#55414,#55415);
#47157=AXIS2_PLACEMENT_3D('',#76723,#55416,#55417);
#47158=AXIS2_PLACEMENT_3D('',#76726,#55419,#55420);
#47159=AXIS2_PLACEMENT_3D('',#76727,#55421,#55422);
#47160=AXIS2_PLACEMENT_3D('',#76729,#55423,#55424);
#47161=AXIS2_PLACEMENT_3D('',#76732,#55426,#55427);
#47162=AXIS2_PLACEMENT_3D('',#76733,#55428,#55429);
#47163=AXIS2_PLACEMENT_3D('',#76735,#55430,#55431);
#47164=AXIS2_PLACEMENT_3D('',#76738,#55433,#55434);
#47165=AXIS2_PLACEMENT_3D('',#76739,#55435,#55436);
#47166=AXIS2_PLACEMENT_3D('',#76741,#55437,#55438);
#47167=AXIS2_PLACEMENT_3D('',#76745,#55440,#55441);
#47168=AXIS2_PLACEMENT_3D('',#76776,#55442,#55443);
#47169=AXIS2_PLACEMENT_3D('',#76777,#55444,#55445);
#47170=AXIS2_PLACEMENT_3D('',#76779,#55446,#55447);
#47171=AXIS2_PLACEMENT_3D('',#76782,#55449,#55450);
#47172=AXIS2_PLACEMENT_3D('',#76783,#55451,#55452);
#47173=AXIS2_PLACEMENT_3D('',#76785,#55453,#55454);
#47174=AXIS2_PLACEMENT_3D('',#76788,#55456,#55457);
#47175=AXIS2_PLACEMENT_3D('',#76789,#55458,#55459);
#47176=AXIS2_PLACEMENT_3D('',#76791,#55460,#55461);
#47177=AXIS2_PLACEMENT_3D('',#76794,#55463,#55464);
#47178=AXIS2_PLACEMENT_3D('',#76795,#55465,#55466);
#47179=AXIS2_PLACEMENT_3D('',#76797,#55467,#55468);
#47180=AXIS2_PLACEMENT_3D('',#76800,#55470,#55471);
#47181=AXIS2_PLACEMENT_3D('',#76801,#55472,#55473);
#47182=AXIS2_PLACEMENT_3D('',#76803,#55474,#55475);
#47183=AXIS2_PLACEMENT_3D('',#76806,#55477,#55478);
#47184=AXIS2_PLACEMENT_3D('',#76807,#55479,#55480);
#47185=AXIS2_PLACEMENT_3D('',#76809,#55481,#55482);
#47186=AXIS2_PLACEMENT_3D('',#76812,#55484,#55485);
#47187=AXIS2_PLACEMENT_3D('',#76813,#55486,#55487);
#47188=AXIS2_PLACEMENT_3D('',#76815,#55488,#55489);
#47189=AXIS2_PLACEMENT_3D('',#76818,#55491,#55492);
#47190=AXIS2_PLACEMENT_3D('',#76819,#55493,#55494);
#47191=AXIS2_PLACEMENT_3D('',#76821,#55495,#55496);
#47192=AXIS2_PLACEMENT_3D('',#76824,#55498,#55499);
#47193=AXIS2_PLACEMENT_3D('',#76825,#55500,#55501);
#47194=AXIS2_PLACEMENT_3D('',#76827,#55502,#55503);
#47195=AXIS2_PLACEMENT_3D('',#76830,#55505,#55506);
#47196=AXIS2_PLACEMENT_3D('',#76831,#55507,#55508);
#47197=AXIS2_PLACEMENT_3D('',#76833,#55509,#55510);
#47198=AXIS2_PLACEMENT_3D('',#76836,#55512,#55513);
#47199=AXIS2_PLACEMENT_3D('',#76837,#55514,#55515);
#47200=AXIS2_PLACEMENT_3D('',#76839,#55516,#55517);
#47201=AXIS2_PLACEMENT_3D('',#76842,#55519,#55520);
#47202=AXIS2_PLACEMENT_3D('',#76843,#55521,#55522);
#47203=AXIS2_PLACEMENT_3D('',#76845,#55523,#55524);
#47204=AXIS2_PLACEMENT_3D('',#76848,#55526,#55527);
#47205=AXIS2_PLACEMENT_3D('',#76849,#55528,#55529);
#47206=AXIS2_PLACEMENT_3D('',#76851,#55530,#55531);
#47207=AXIS2_PLACEMENT_3D('',#76854,#55533,#55534);
#47208=AXIS2_PLACEMENT_3D('',#76855,#55535,#55536);
#47209=AXIS2_PLACEMENT_3D('',#76857,#55537,#55538);
#47210=AXIS2_PLACEMENT_3D('',#76860,#55540,#55541);
#47211=AXIS2_PLACEMENT_3D('',#76861,#55542,#55543);
#47212=AXIS2_PLACEMENT_3D('',#76863,#55544,#55545);
#47213=AXIS2_PLACEMENT_3D('',#76866,#55547,#55548);
#47214=AXIS2_PLACEMENT_3D('',#76867,#55549,#55550);
#47215=AXIS2_PLACEMENT_3D('',#76869,#55551,#55552);
#47216=AXIS2_PLACEMENT_3D('',#76872,#55554,#55555);
#47217=AXIS2_PLACEMENT_3D('',#76873,#55556,#55557);
#47218=AXIS2_PLACEMENT_3D('',#76875,#55558,#55559);
#47219=AXIS2_PLACEMENT_3D('',#76878,#55561,#55562);
#47220=AXIS2_PLACEMENT_3D('',#76879,#55563,#55564);
#47221=AXIS2_PLACEMENT_3D('',#76881,#55565,#55566);
#47222=AXIS2_PLACEMENT_3D('',#76915,#55568,#55569);
#47223=AXIS2_PLACEMENT_3D('',#76920,#55570,#55571);
#47224=AXIS2_PLACEMENT_3D('',#76922,#55572,#55573);
#47225=AXIS2_PLACEMENT_3D('',#76925,#55575,#55576);
#47226=AXIS2_PLACEMENT_3D('',#76926,#55577,#55578);
#47227=AXIS2_PLACEMENT_3D('',#76928,#55579,#55580);
#47228=AXIS2_PLACEMENT_3D('',#76931,#55582,#55583);
#47229=AXIS2_PLACEMENT_3D('',#76932,#55584,#55585);
#47230=AXIS2_PLACEMENT_3D('',#76934,#55586,#55587);
#47231=AXIS2_PLACEMENT_3D('',#76937,#55589,#55590);
#47232=AXIS2_PLACEMENT_3D('',#76938,#55591,#55592);
#47233=AXIS2_PLACEMENT_3D('',#76940,#55593,#55594);
#47234=AXIS2_PLACEMENT_3D('',#76943,#55596,#55597);
#47235=AXIS2_PLACEMENT_3D('',#76944,#55598,#55599);
#47236=AXIS2_PLACEMENT_3D('',#76946,#55600,#55601);
#47237=AXIS2_PLACEMENT_3D('',#76949,#55603,#55604);
#47238=AXIS2_PLACEMENT_3D('',#76950,#55605,#55606);
#47239=AXIS2_PLACEMENT_3D('',#76952,#55607,#55608);
#47240=AXIS2_PLACEMENT_3D('',#76955,#55610,#55611);
#47241=AXIS2_PLACEMENT_3D('',#76956,#55612,#55613);
#47242=AXIS2_PLACEMENT_3D('',#76958,#55614,#55615);
#47243=AXIS2_PLACEMENT_3D('',#76961,#55617,#55618);
#47244=AXIS2_PLACEMENT_3D('',#76962,#55619,#55620);
#47245=AXIS2_PLACEMENT_3D('',#76964,#55621,#55622);
#47246=AXIS2_PLACEMENT_3D('',#76967,#55624,#55625);
#47247=AXIS2_PLACEMENT_3D('',#76968,#55626,#55627);
#47248=AXIS2_PLACEMENT_3D('',#76970,#55628,#55629);
#47249=AXIS2_PLACEMENT_3D('',#76973,#55631,#55632);
#47250=AXIS2_PLACEMENT_3D('',#76974,#55633,#55634);
#47251=AXIS2_PLACEMENT_3D('',#76976,#55635,#55636);
#47252=AXIS2_PLACEMENT_3D('',#76979,#55638,#55639);
#47253=AXIS2_PLACEMENT_3D('',#76980,#55640,#55641);
#47254=AXIS2_PLACEMENT_3D('',#76982,#55642,#55643);
#47255=AXIS2_PLACEMENT_3D('',#76985,#55645,#55646);
#47256=AXIS2_PLACEMENT_3D('',#76986,#55647,#55648);
#47257=AXIS2_PLACEMENT_3D('',#76988,#55649,#55650);
#47258=AXIS2_PLACEMENT_3D('',#76991,#55652,#55653);
#47259=AXIS2_PLACEMENT_3D('',#76992,#55654,#55655);
#47260=AXIS2_PLACEMENT_3D('',#76994,#55656,#55657);
#47261=AXIS2_PLACEMENT_3D('',#76997,#55659,#55660);
#47262=AXIS2_PLACEMENT_3D('',#76998,#55661,#55662);
#47263=AXIS2_PLACEMENT_3D('',#77000,#55663,#55664);
#47264=AXIS2_PLACEMENT_3D('',#77003,#55666,#55667);
#47265=AXIS2_PLACEMENT_3D('',#77004,#55668,#55669);
#47266=AXIS2_PLACEMENT_3D('',#77006,#55670,#55671);
#47267=AXIS2_PLACEMENT_3D('',#77009,#55673,#55674);
#47268=AXIS2_PLACEMENT_3D('',#77010,#55675,#55676);
#47269=AXIS2_PLACEMENT_3D('',#77012,#55677,#55678);
#47270=AXIS2_PLACEMENT_3D('',#77046,#55680,#55681);
#47271=AXIS2_PLACEMENT_3D('',#77051,#55682,#55683);
#47272=AXIS2_PLACEMENT_3D('',#77053,#55684,#55685);
#47273=AXIS2_PLACEMENT_3D('',#77056,#55687,#55688);
#47274=AXIS2_PLACEMENT_3D('',#77057,#55689,#55690);
#47275=AXIS2_PLACEMENT_3D('',#77059,#55691,#55692);
#47276=AXIS2_PLACEMENT_3D('',#77062,#55694,#55695);
#47277=AXIS2_PLACEMENT_3D('',#77063,#55696,#55697);
#47278=AXIS2_PLACEMENT_3D('',#77065,#55698,#55699);
#47279=AXIS2_PLACEMENT_3D('',#77068,#55701,#55702);
#47280=AXIS2_PLACEMENT_3D('',#77069,#55703,#55704);
#47281=AXIS2_PLACEMENT_3D('',#77071,#55705,#55706);
#47282=AXIS2_PLACEMENT_3D('',#77074,#55708,#55709);
#47283=AXIS2_PLACEMENT_3D('',#77075,#55710,#55711);
#47284=AXIS2_PLACEMENT_3D('',#77077,#55712,#55713);
#47285=AXIS2_PLACEMENT_3D('',#77080,#55715,#55716);
#47286=AXIS2_PLACEMENT_3D('',#77081,#55717,#55718);
#47287=AXIS2_PLACEMENT_3D('',#77083,#55719,#55720);
#47288=AXIS2_PLACEMENT_3D('',#77086,#55722,#55723);
#47289=AXIS2_PLACEMENT_3D('',#77087,#55724,#55725);
#47290=AXIS2_PLACEMENT_3D('',#77089,#55726,#55727);
#47291=AXIS2_PLACEMENT_3D('',#77092,#55729,#55730);
#47292=AXIS2_PLACEMENT_3D('',#77093,#55731,#55732);
#47293=AXIS2_PLACEMENT_3D('',#77095,#55733,#55734);
#47294=AXIS2_PLACEMENT_3D('',#77098,#55736,#55737);
#47295=AXIS2_PLACEMENT_3D('',#77099,#55738,#55739);
#47296=AXIS2_PLACEMENT_3D('',#77101,#55740,#55741);
#47297=AXIS2_PLACEMENT_3D('',#77104,#55743,#55744);
#47298=AXIS2_PLACEMENT_3D('',#77105,#55745,#55746);
#47299=AXIS2_PLACEMENT_3D('',#77107,#55747,#55748);
#47300=AXIS2_PLACEMENT_3D('',#77110,#55750,#55751);
#47301=AXIS2_PLACEMENT_3D('',#77111,#55752,#55753);
#47302=AXIS2_PLACEMENT_3D('',#77113,#55754,#55755);
#47303=AXIS2_PLACEMENT_3D('',#77116,#55757,#55758);
#47304=AXIS2_PLACEMENT_3D('',#77117,#55759,#55760);
#47305=AXIS2_PLACEMENT_3D('',#77119,#55761,#55762);
#47306=AXIS2_PLACEMENT_3D('',#77122,#55764,#55765);
#47307=AXIS2_PLACEMENT_3D('',#77123,#55766,#55767);
#47308=AXIS2_PLACEMENT_3D('',#77125,#55768,#55769);
#47309=AXIS2_PLACEMENT_3D('',#77128,#55771,#55772);
#47310=AXIS2_PLACEMENT_3D('',#77129,#55773,#55774);
#47311=AXIS2_PLACEMENT_3D('',#77131,#55775,#55776);
#47312=AXIS2_PLACEMENT_3D('',#77134,#55778,#55779);
#47313=AXIS2_PLACEMENT_3D('',#77135,#55780,#55781);
#47314=AXIS2_PLACEMENT_3D('',#77137,#55782,#55783);
#47315=AXIS2_PLACEMENT_3D('',#77140,#55785,#55786);
#47316=AXIS2_PLACEMENT_3D('',#77141,#55787,#55788);
#47317=AXIS2_PLACEMENT_3D('',#77143,#55789,#55790);
#47318=AXIS2_PLACEMENT_3D('',#77146,#55792,#55793);
#47319=AXIS2_PLACEMENT_3D('',#77147,#55794,#55795);
#47320=AXIS2_PLACEMENT_3D('',#77149,#55796,#55797);
#47321=AXIS2_PLACEMENT_3D('',#77152,#55799,#55800);
#47322=AXIS2_PLACEMENT_3D('',#77153,#55801,#55802);
#47323=AXIS2_PLACEMENT_3D('',#77155,#55803,#55804);
#47324=AXIS2_PLACEMENT_3D('',#77187,#55806,#55807);
#47325=AXIS2_PLACEMENT_3D('',#77194,#55808,#55809);
#47326=AXIS2_PLACEMENT_3D('',#77196,#55810,#55811);
#47327=AXIS2_PLACEMENT_3D('',#77199,#55813,#55814);
#47328=AXIS2_PLACEMENT_3D('',#77200,#55815,#55816);
#47329=AXIS2_PLACEMENT_3D('',#77202,#55817,#55818);
#47330=AXIS2_PLACEMENT_3D('',#77205,#55820,#55821);
#47331=AXIS2_PLACEMENT_3D('',#77206,#55822,#55823);
#47332=AXIS2_PLACEMENT_3D('',#77208,#55824,#55825);
#47333=AXIS2_PLACEMENT_3D('',#77211,#55827,#55828);
#47334=AXIS2_PLACEMENT_3D('',#77212,#55829,#55830);
#47335=AXIS2_PLACEMENT_3D('',#77214,#55831,#55832);
#47336=AXIS2_PLACEMENT_3D('',#77217,#55834,#55835);
#47337=AXIS2_PLACEMENT_3D('',#77218,#55836,#55837);
#47338=AXIS2_PLACEMENT_3D('',#77220,#55838,#55839);
#47339=AXIS2_PLACEMENT_3D('',#77223,#55841,#55842);
#47340=AXIS2_PLACEMENT_3D('',#77224,#55843,#55844);
#47341=AXIS2_PLACEMENT_3D('',#77226,#55845,#55846);
#47342=AXIS2_PLACEMENT_3D('',#77229,#55848,#55849);
#47343=AXIS2_PLACEMENT_3D('',#77230,#55850,#55851);
#47344=AXIS2_PLACEMENT_3D('',#77232,#55852,#55853);
#47345=AXIS2_PLACEMENT_3D('',#77235,#55855,#55856);
#47346=AXIS2_PLACEMENT_3D('',#77236,#55857,#55858);
#47347=AXIS2_PLACEMENT_3D('',#77238,#55859,#55860);
#47348=AXIS2_PLACEMENT_3D('',#77241,#55862,#55863);
#47349=AXIS2_PLACEMENT_3D('',#77242,#55864,#55865);
#47350=AXIS2_PLACEMENT_3D('',#77244,#55866,#55867);
#47351=AXIS2_PLACEMENT_3D('',#77247,#55869,#55870);
#47352=AXIS2_PLACEMENT_3D('',#77248,#55871,#55872);
#47353=AXIS2_PLACEMENT_3D('',#77250,#55873,#55874);
#47354=AXIS2_PLACEMENT_3D('',#77253,#55876,#55877);
#47355=AXIS2_PLACEMENT_3D('',#77254,#55878,#55879);
#47356=AXIS2_PLACEMENT_3D('',#77256,#55880,#55881);
#47357=AXIS2_PLACEMENT_3D('',#77259,#55883,#55884);
#47358=AXIS2_PLACEMENT_3D('',#77260,#55885,#55886);
#47359=AXIS2_PLACEMENT_3D('',#77262,#55887,#55888);
#47360=AXIS2_PLACEMENT_3D('',#77265,#55890,#55891);
#47361=AXIS2_PLACEMENT_3D('',#77266,#55892,#55893);
#47362=AXIS2_PLACEMENT_3D('',#77268,#55894,#55895);
#47363=AXIS2_PLACEMENT_3D('',#77271,#55897,#55898);
#47364=AXIS2_PLACEMENT_3D('',#77272,#55899,#55900);
#47365=AXIS2_PLACEMENT_3D('',#77274,#55901,#55902);
#47366=AXIS2_PLACEMENT_3D('',#77277,#55904,#55905);
#47367=AXIS2_PLACEMENT_3D('',#77278,#55906,#55907);
#47368=AXIS2_PLACEMENT_3D('',#77280,#55908,#55909);
#47369=AXIS2_PLACEMENT_3D('',#77283,#55911,#55912);
#47370=AXIS2_PLACEMENT_3D('',#77284,#55913,#55914);
#47371=AXIS2_PLACEMENT_3D('',#77286,#55915,#55916);
#47372=AXIS2_PLACEMENT_3D('',#77289,#55918,#55919);
#47373=AXIS2_PLACEMENT_3D('',#77290,#55920,#55921);
#47374=AXIS2_PLACEMENT_3D('',#77292,#55922,#55923);
#47375=AXIS2_PLACEMENT_3D('',#77295,#55925,#55926);
#47376=AXIS2_PLACEMENT_3D('',#77296,#55927,#55928);
#47377=AXIS2_PLACEMENT_3D('',#77298,#55929,#55930);
#47378=AXIS2_PLACEMENT_3D('',#77328,#55932,#55933);
#47379=AXIS2_PLACEMENT_3D('',#77337,#55934,#55935);
#47380=AXIS2_PLACEMENT_3D('',#77339,#55936,#55937);
#47381=AXIS2_PLACEMENT_3D('',#77342,#55939,#55940);
#47382=AXIS2_PLACEMENT_3D('',#77372,#55941,#55942);
#47383=AXIS2_PLACEMENT_3D('',#77373,#55943,#55944);
#47384=AXIS2_PLACEMENT_3D('',#77374,#55945,#55946);
#47385=AXIS2_PLACEMENT_3D('',#77375,#55947,#55948);
#47386=AXIS2_PLACEMENT_3D('',#77376,#55949,#55950);
#47387=AXIS2_PLACEMENT_3D('',#77377,#55951,#55952);
#47388=AXIS2_PLACEMENT_3D('',#77378,#55953,#55954);
#47389=AXIS2_PLACEMENT_3D('',#77379,#55955,#55956);
#47390=AXIS2_PLACEMENT_3D('',#77380,#55957,#55958);
#47391=AXIS2_PLACEMENT_3D('',#77381,#55959,#55960);
#47392=AXIS2_PLACEMENT_3D('',#77382,#55961,#55962);
#47393=AXIS2_PLACEMENT_3D('',#77383,#55963,#55964);
#47394=AXIS2_PLACEMENT_3D('',#77384,#55965,#55966);
#47395=AXIS2_PLACEMENT_3D('',#77385,#55967,#55968);
#47396=AXIS2_PLACEMENT_3D('',#77386,#55969,#55970);
#47397=AXIS2_PLACEMENT_3D('',#77387,#55971,#55972);
#47398=AXIS2_PLACEMENT_3D('',#77388,#55973,#55974);
#47399=AXIS2_PLACEMENT_3D('',#77389,#55975,#55976);
#47400=AXIS2_PLACEMENT_3D('',#77390,#55977,#55978);
#47401=AXIS2_PLACEMENT_3D('',#77391,#55979,#55980);
#47402=AXIS2_PLACEMENT_3D('',#77392,#55981,#55982);
#47403=AXIS2_PLACEMENT_3D('',#77393,#55983,#55984);
#47404=AXIS2_PLACEMENT_3D('',#77394,#55985,#55986);
#47405=AXIS2_PLACEMENT_3D('',#77395,#55987,#55988);
#47406=AXIS2_PLACEMENT_3D('',#77396,#55989,#55990);
#47407=AXIS2_PLACEMENT_3D('',#77397,#55991,#55992);
#47408=AXIS2_PLACEMENT_3D('',#77399,#55993,#55994);
#47409=AXIS2_PLACEMENT_3D('',#77400,#55995,#55996);
#47410=AXIS2_PLACEMENT_3D('',#77446,#55997,#55998);
#47411=AXIS2_PLACEMENT_3D('',#77449,#55999,#56000);
#47412=AXIS2_PLACEMENT_3D('',#77451,#56001,#56002);
#47413=AXIS2_PLACEMENT_3D('',#77794,#56003,#56004);
#47414=AXIS2_PLACEMENT_3D('',#77795,#56005,#56006);
#47415=AXIS2_PLACEMENT_3D('',#77798,#56007,#56008);
#47416=AXIS2_PLACEMENT_3D('',#77801,#56010,#56011);
#47417=AXIS2_PLACEMENT_3D('',#77802,#56012,#56013);
#47418=AXIS2_PLACEMENT_3D('',#77803,#56014,#56015);
#47419=AXIS2_PLACEMENT_3D('',#77805,#56016,#56017);
#47420=AXIS2_PLACEMENT_3D('',#77806,#56018,#56019);
#47421=AXIS2_PLACEMENT_3D('',#77807,#56020,#56021);
#47422=AXIS2_PLACEMENT_3D('',#77809,#56022,#56023);
#47423=AXIS2_PLACEMENT_3D('',#77811,#56024,#56025);
#47424=AXIS2_PLACEMENT_3D('',#77812,#56026,#56027);
#47425=AXIS2_PLACEMENT_3D('',#77813,#56028,#56029);
#47426=AXIS2_PLACEMENT_3D('',#77816,#56030,#56031);
#47427=AXIS2_PLACEMENT_3D('',#77829,#56032,#56033);
#47428=AXIS2_PLACEMENT_3D('',#77840,#56034,#56035);
#47429=AXIS2_PLACEMENT_3D('',#77843,#56036,#56037);
#47430=AXIS2_PLACEMENT_3D('',#77845,#56038,#56039);
#47431=AXIS2_PLACEMENT_3D('',#77847,#56040,#56041);
#47432=AXIS2_PLACEMENT_3D('',#77848,#56042,#56043);
#47433=AXIS2_PLACEMENT_3D('',#77849,#56044,#56045);
#47434=AXIS2_PLACEMENT_3D('',#77852,#56046,#56047);
#47435=AXIS2_PLACEMENT_3D('',#77854,#56048,#56049);
#47436=AXIS2_PLACEMENT_3D('',#77858,#56051,#56052);
#47437=AXIS2_PLACEMENT_3D('',#77860,#56054,#56055);
#47438=AXIS2_PLACEMENT_3D('',#77892,#56056,#56057);
#47439=AXIS2_PLACEMENT_3D('',#77893,#56058,#56059);
#47440=AXIS2_PLACEMENT_3D('',#77896,#56060,#56061);
#47441=AXIS2_PLACEMENT_3D('',#77898,#56063,#56064);
#47442=AXIS2_PLACEMENT_3D('',#77899,#56065,#56066);
#47443=AXIS2_PLACEMENT_3D('',#77901,#56067,#56068);
#47444=AXIS2_PLACEMENT_3D('',#77902,#56069,#56070);
#47445=AXIS2_PLACEMENT_3D('',#77903,#56071,#56072);
#47446=AXIS2_PLACEMENT_3D('',#77905,#56073,#56074);
#47447=AXIS2_PLACEMENT_3D('',#77942,#56076,#56077);
#47448=AXIS2_PLACEMENT_3D('',#77999,#56079,#56080);
#47449=AXIS2_PLACEMENT_3D('',#78000,#56081,#56082);
#47450=AXIS2_PLACEMENT_3D('',#78001,#56083,#56084);
#47451=AXIS2_PLACEMENT_3D('',#78042,#56089,#56090);
#47452=AXIS2_PLACEMENT_3D('',#78045,#56091,#56092);
#47453=AXIS2_PLACEMENT_3D('',#78070,#56094,#56095);
#47454=AXIS2_PLACEMENT_3D('',#78091,#56096,#56097);
#47455=AXIS2_PLACEMENT_3D('',#78092,#56098,#56099);
#47456=AXIS2_PLACEMENT_3D('',#78093,#56100,#56101);
#47457=AXIS2_PLACEMENT_3D('',#78098,#56103,#56104);
#47458=AXIS2_PLACEMENT_3D('',#78101,#56106,#56107);
#47459=AXIS2_PLACEMENT_3D('',#78103,#56109,#56110);
#47460=AXIS2_PLACEMENT_3D('',#78111,#56111,#56112);
#47461=AXIS2_PLACEMENT_3D('',#78112,#56113,#56114);
#47462=AXIS2_PLACEMENT_3D('',#78146,#56117,#56118);
#47463=AXIS2_PLACEMENT_3D('',#78151,#56120,#56121);
#47464=AXIS2_PLACEMENT_3D('',#78154,#56123,#56124);
#47465=AXIS2_PLACEMENT_3D('',#78155,#56125,#56126);
#47466=AXIS2_PLACEMENT_3D('',#78163,#56131,#56132);
#47467=AXIS2_PLACEMENT_3D('',#78167,#56134,#56135);
#47468=AXIS2_PLACEMENT_3D('',#78168,#56136,#56137);
#47469=AXIS2_PLACEMENT_3D('',#78169,#56138,#56139);
#47470=AXIS2_PLACEMENT_3D('',#78185,#56140,#56141);
#47471=AXIS2_PLACEMENT_3D('',#78189,#56143,#56144);
#47472=AXIS2_PLACEMENT_3D('',#78294,#56145,#56146);
#47473=AXIS2_PLACEMENT_3D('',#78297,#56149,#56150);
#47474=AXIS2_PLACEMENT_3D('',#78298,#56151,#56152);
#47475=AXIS2_PLACEMENT_3D('',#78299,#56153,#56154);
#47476=AXIS2_PLACEMENT_3D('',#78300,#56155,#56156);
#47477=AXIS2_PLACEMENT_3D('',#78301,#56157,#56158);
#47478=AXIS2_PLACEMENT_3D('',#78302,#56159,#56160);
#47479=AXIS2_PLACEMENT_3D('',#78303,#56161,#56162);
#47480=AXIS2_PLACEMENT_3D('',#78304,#56163,#56164);
#47481=AXIS2_PLACEMENT_3D('',#78305,#56165,#56166);
#47482=AXIS2_PLACEMENT_3D('',#78324,#56167,#56168);
#47483=AXIS2_PLACEMENT_3D('',#78325,#56169,#56170);
#47484=AXIS2_PLACEMENT_3D('',#78326,#56171,#56172);
#47485=AXIS2_PLACEMENT_3D('',#78327,#56173,#56174);
#47486=AXIS2_PLACEMENT_3D('',#78328,#56175,#56176);
#47487=AXIS2_PLACEMENT_3D('',#78329,#56177,#56178);
#47488=AXIS2_PLACEMENT_3D('',#78355,#56179,#56180);
#47489=AXIS2_PLACEMENT_3D('',#78362,#56181,#56182);
#47490=AXIS2_PLACEMENT_3D('',#78561,#56183,#56184);
#47491=AXIS2_PLACEMENT_3D('',#78903,#56185,#56186);
#47492=AXIS2_PLACEMENT_3D('',#78905,#56187,#56188);
#47493=AXIS2_PLACEMENT_3D('',#78932,#56190,#56191);
#47494=AXIS2_PLACEMENT_3D('',#78983,#56192,#56193);
#47495=AXIS2_PLACEMENT_3D('',#78985,#56194,#56195);
#47496=AXIS2_PLACEMENT_3D('',#78987,#56197,#56198);
#47497=AXIS2_PLACEMENT_3D('',#79074,#56199,#56200);
#47498=AXIS2_PLACEMENT_3D('',#79081,#56201,#56202);
#47499=AXIS2_PLACEMENT_3D('',#79202,#56203,#56204);
#47500=AXIS2_PLACEMENT_3D('',#79514,#56205,#56206);
#47501=AXIS2_PLACEMENT_3D('',#79567,#56207,#56208);
#47502=AXIS2_PLACEMENT_3D('',#79569,#56209,#56210);
#47503=AXIS2_PLACEMENT_3D('',#79586,#56211,#56212);
#47504=AXIS2_PLACEMENT_3D('',#79589,#56213,#56214);
#47505=AXIS2_PLACEMENT_3D('',#79590,#56215,#56216);
#47506=AXIS2_PLACEMENT_3D('',#79591,#56217,#56218);
#47507=AXIS2_PLACEMENT_3D('',#79618,#56219,#56220);
#47508=AXIS2_PLACEMENT_3D('',#79635,#56221,#56222);
#47509=AXIS2_PLACEMENT_3D('',#79660,#56223,#56224);
#47510=AXIS2_PLACEMENT_3D('',#79677,#56225,#56226);
#47511=AXIS2_PLACEMENT_3D('',#79680,#56227,#56228);
#47512=AXIS2_PLACEMENT_3D('',#79707,#56231,#56232);
#47513=AXIS2_PLACEMENT_3D('',#79881,#56233,#56234);
#47514=AXIS2_PLACEMENT_3D('',#79907,#56235,#56236);
#47515=AXIS2_PLACEMENT_3D('',#79924,#56237,#56238);
#47516=AXIS2_PLACEMENT_3D('',#80258,#56239,#56240);
#47517=AXIS2_PLACEMENT_3D('',#80451,#56241,#56242);
#47518=AXIS2_PLACEMENT_3D('',#81089,#56245,#56246);
#47519=AXIS2_PLACEMENT_3D('',#81336,#56247,#56248);
#47520=AXIS2_PLACEMENT_3D('',#81961,#56249,#56250);
#47521=AXIS2_PLACEMENT_3D('',#81999,#56251,#56252);
#47522=AXIS2_PLACEMENT_3D('',#82145,#56253,#56254);
#47523=AXIS2_PLACEMENT_3D('',#82146,#56255,#56256);
#47524=AXIS2_PLACEMENT_3D('',#82284,#56257,#56258);
#47525=AXIS2_PLACEMENT_3D('',#82357,#56259,#56260);
#47526=AXIS2_PLACEMENT_3D('',#82410,#56261,#56262);
#47527=AXIS2_PLACEMENT_3D('',#82411,#56263,#56264);
#47528=AXIS2_PLACEMENT_3D('',#82472,#56265,#56266);
#47529=AXIS2_PLACEMENT_3D('',#82473,#56267,#56268);
#47530=AXIS2_PLACEMENT_3D('',#82474,#56269,#56270);
#47531=AXIS2_PLACEMENT_3D('',#83489,#56271,#56272);
#47532=AXIS2_PLACEMENT_3D('',#83490,#56273,#56274);
#47533=AXIS2_PLACEMENT_3D('',#83491,#56275,#56276);
#47534=AXIS2_PLACEMENT_3D('',#83492,#56277,#56278);
#47535=AXIS2_PLACEMENT_3D('',#83691,#56279,#56280);
#47536=AXIS2_PLACEMENT_3D('',#83693,#56282,#56283);
#47537=AXIS2_PLACEMENT_3D('',#83695,#56285,#56286);
#47538=AXIS2_PLACEMENT_3D('',#83696,#56287,#56288);
#47539=AXIS2_PLACEMENT_3D('',#83697,#56289,#56290);
#47540=AXIS2_PLACEMENT_3D('',#83698,#56291,#56292);
#47541=AXIS2_PLACEMENT_3D('',#83699,#56293,#56294);
#47542=AXIS2_PLACEMENT_3D('',#83700,#56295,#56296);
#47543=AXIS2_PLACEMENT_3D('',#83701,#56297,#56298);
#47544=AXIS2_PLACEMENT_3D('',#83702,#56299,#56300);
#47545=AXIS2_PLACEMENT_3D('',#83703,#56301,#56302);
#47546=AXIS2_PLACEMENT_3D('',#83704,#56303,#56304);
#47547=AXIS2_PLACEMENT_3D('',#83705,#56305,#56306);
#47548=AXIS2_PLACEMENT_3D('',#83706,#56307,#56308);
#47549=AXIS2_PLACEMENT_3D('',#83707,#56309,#56310);
#47550=AXIS2_PLACEMENT_3D('',#83708,#56311,#56312);
#47551=AXIS2_PLACEMENT_3D('',#83709,#56313,#56314);
#47552=AXIS2_PLACEMENT_3D('',#83710,#56315,#56316);
#47553=AXIS2_PLACEMENT_3D('',#83711,#56317,#56318);
#47554=AXIS2_PLACEMENT_3D('',#83712,#56319,#56320);
#47555=AXIS2_PLACEMENT_3D('',#83713,#56321,#56322);
#47556=AXIS2_PLACEMENT_3D('',#83714,#56323,#56324);
#47557=AXIS2_PLACEMENT_3D('',#83715,#56325,#56326);
#47558=AXIS2_PLACEMENT_3D('',#83716,#56327,#56328);
#47559=AXIS2_PLACEMENT_3D('',#83717,#56329,#56330);
#47560=AXIS2_PLACEMENT_3D('',#83718,#56331,#56332);
#47561=AXIS2_PLACEMENT_3D('',#83719,#56333,#56334);
#47562=AXIS2_PLACEMENT_3D('',#83720,#56335,#56336);
#47563=AXIS2_PLACEMENT_3D('',#83721,#56337,#56338);
#47564=AXIS2_PLACEMENT_3D('',#83722,#56339,#56340);
#47565=AXIS2_PLACEMENT_3D('',#83723,#56341,#56342);
#47566=AXIS2_PLACEMENT_3D('',#83724,#56343,#56344);
#47567=AXIS2_PLACEMENT_3D('',#83725,#56345,#56346);
#47568=AXIS2_PLACEMENT_3D('',#83726,#56347,#56348);
#47569=AXIS2_PLACEMENT_3D('',#83727,#56349,#56350);
#47570=AXIS2_PLACEMENT_3D('',#83728,#56351,#56352);
#47571=AXIS2_PLACEMENT_3D('',#83729,#56353,#56354);
#47572=AXIS2_PLACEMENT_3D('',#83730,#56355,#56356);
#47573=AXIS2_PLACEMENT_3D('',#83731,#56357,#56358);
#47574=AXIS2_PLACEMENT_3D('',#83732,#56359,#56360);
#47575=AXIS2_PLACEMENT_3D('',#83733,#56361,#56362);
#47576=AXIS2_PLACEMENT_3D('',#83734,#56363,#56364);
#47577=AXIS2_PLACEMENT_3D('',#83735,#56365,#56366);
#47578=AXIS2_PLACEMENT_3D('',#83736,#56367,#56368);
#47579=AXIS2_PLACEMENT_3D('',#83737,#56369,#56370);
#47580=AXIS2_PLACEMENT_3D('',#83738,#56371,#56372);
#47581=AXIS2_PLACEMENT_3D('',#83739,#56373,#56374);
#47582=AXIS2_PLACEMENT_3D('',#83740,#56375,#56376);
#47583=AXIS2_PLACEMENT_3D('',#83741,#56377,#56378);
#47584=AXIS2_PLACEMENT_3D('',#83742,#56379,#56380);
#47585=AXIS2_PLACEMENT_3D('',#83743,#56381,#56382);
#47586=AXIS2_PLACEMENT_3D('',#83744,#56383,#56384);
#47587=AXIS2_PLACEMENT_3D('',#83745,#56385,#56386);
#47588=AXIS2_PLACEMENT_3D('',#83746,#56387,#56388);
#47589=AXIS2_PLACEMENT_3D('',#83747,#56389,#56390);
#47590=AXIS2_PLACEMENT_3D('',#83748,#56391,#56392);
#47591=AXIS2_PLACEMENT_3D('',#83749,#56393,#56394);
#47592=AXIS2_PLACEMENT_3D('',#83750,#56395,#56396);
#47593=AXIS2_PLACEMENT_3D('',#83751,#56397,#56398);
#47594=AXIS2_PLACEMENT_3D('',#83752,#56399,#56400);
#47595=AXIS2_PLACEMENT_3D('',#83753,#56401,#56402);
#47596=AXIS2_PLACEMENT_3D('',#83754,#56403,#56404);
#47597=AXIS2_PLACEMENT_3D('',#83755,#56405,#56406);
#47598=AXIS2_PLACEMENT_3D('',#83756,#56407,#56408);
#47599=AXIS2_PLACEMENT_3D('',#83757,#56409,#56410);
#47600=AXIS2_PLACEMENT_3D('',#83758,#56411,#56412);
#47601=AXIS2_PLACEMENT_3D('',#83759,#56413,#56414);
#47602=AXIS2_PLACEMENT_3D('',#83760,#56415,#56416);
#47603=AXIS2_PLACEMENT_3D('',#83761,#56417,#56418);
#47604=AXIS2_PLACEMENT_3D('',#83762,#56419,#56420);
#47605=AXIS2_PLACEMENT_3D('',#83763,#56421,#56422);
#47606=AXIS2_PLACEMENT_3D('',#83764,#56423,#56424);
#47607=AXIS2_PLACEMENT_3D('',#83765,#56425,#56426);
#47608=AXIS2_PLACEMENT_3D('',#83766,#56427,#56428);
#47609=AXIS2_PLACEMENT_3D('',#83767,#56429,#56430);
#47610=AXIS2_PLACEMENT_3D('',#83768,#56431,#56432);
#47611=AXIS2_PLACEMENT_3D('',#83769,#56433,#56434);
#47612=AXIS2_PLACEMENT_3D('',#83770,#56435,#56436);
#47613=AXIS2_PLACEMENT_3D('',#83771,#56437,#56438);
#47614=AXIS2_PLACEMENT_3D('',#83772,#56439,#56440);
#47615=AXIS2_PLACEMENT_3D('',#83773,#56441,#56442);
#47616=AXIS2_PLACEMENT_3D('',#83774,#56443,#56444);
#47617=AXIS2_PLACEMENT_3D('',#83775,#56445,#56446);
#47618=AXIS2_PLACEMENT_3D('',#83776,#56447,#56448);
#47619=AXIS2_PLACEMENT_3D('',#83777,#56449,#56450);
#47620=AXIS2_PLACEMENT_3D('',#83778,#56451,#56452);
#47621=AXIS2_PLACEMENT_3D('',#83779,#56453,#56454);
#47622=AXIS2_PLACEMENT_3D('',#83780,#56455,#56456);
#47623=AXIS2_PLACEMENT_3D('',#83781,#56457,#56458);
#47624=AXIS2_PLACEMENT_3D('',#83782,#56459,#56460);
#47625=AXIS2_PLACEMENT_3D('',#83783,#56461,#56462);
#47626=AXIS2_PLACEMENT_3D('',#83784,#56463,#56464);
#47627=AXIS2_PLACEMENT_3D('',#83785,#56465,#56466);
#47628=AXIS2_PLACEMENT_3D('',#83786,#56467,#56468);
#47629=AXIS2_PLACEMENT_3D('',#83787,#56469,#56470);
#47630=AXIS2_PLACEMENT_3D('',#83788,#56471,#56472);
#47631=AXIS2_PLACEMENT_3D('',#83789,#56473,#56474);
#47632=AXIS2_PLACEMENT_3D('',#83790,#56475,#56476);
#47633=AXIS2_PLACEMENT_3D('',#83791,#56477,#56478);
#47634=AXIS2_PLACEMENT_3D('',#83792,#56479,#56480);
#47635=AXIS2_PLACEMENT_3D('',#83793,#56481,#56482);
#47636=AXIS2_PLACEMENT_3D('',#83794,#56483,#56484);
#47637=AXIS2_PLACEMENT_3D('',#83795,#56485,#56486);
#47638=AXIS2_PLACEMENT_3D('',#83796,#56487,#56488);
#47639=AXIS2_PLACEMENT_3D('',#83797,#56489,#56490);
#47640=AXIS2_PLACEMENT_3D('',#83798,#56491,#56492);
#47641=AXIS2_PLACEMENT_3D('',#83799,#56493,#56494);
#47642=AXIS2_PLACEMENT_3D('',#83800,#56495,#56496);
#47643=AXIS2_PLACEMENT_3D('',#83801,#56497,#56498);
#47644=AXIS2_PLACEMENT_3D('',#83802,#56499,#56500);
#47645=AXIS2_PLACEMENT_3D('',#83803,#56501,#56502);
#47646=AXIS2_PLACEMENT_3D('',#83804,#56503,#56504);
#47647=AXIS2_PLACEMENT_3D('',#83805,#56505,#56506);
#47648=AXIS2_PLACEMENT_3D('',#83806,#56507,#56508);
#47649=AXIS2_PLACEMENT_3D('',#83807,#56509,#56510);
#47650=AXIS2_PLACEMENT_3D('',#83808,#56511,#56512);
#47651=AXIS2_PLACEMENT_3D('',#83809,#56513,#56514);
#47652=AXIS2_PLACEMENT_3D('',#83810,#56515,#56516);
#47653=AXIS2_PLACEMENT_3D('',#83811,#56517,#56518);
#47654=AXIS2_PLACEMENT_3D('',#83812,#56519,#56520);
#47655=AXIS2_PLACEMENT_3D('',#83813,#56521,#56522);
#47656=AXIS2_PLACEMENT_3D('',#83814,#56523,#56524);
#47657=AXIS2_PLACEMENT_3D('',#83815,#56525,#56526);
#47658=AXIS2_PLACEMENT_3D('',#83816,#56527,#56528);
#47659=AXIS2_PLACEMENT_3D('',#83817,#56529,#56530);
#47660=AXIS2_PLACEMENT_3D('',#83818,#56531,#56532);
#47661=AXIS2_PLACEMENT_3D('',#83819,#56533,#56534);
#47662=AXIS2_PLACEMENT_3D('',#83820,#56535,#56536);
#47663=AXIS2_PLACEMENT_3D('',#83821,#56537,#56538);
#47664=AXIS2_PLACEMENT_3D('',#83822,#56539,#56540);
#47665=AXIS2_PLACEMENT_3D('',#83823,#56541,#56542);
#47666=AXIS2_PLACEMENT_3D('',#83824,#56543,#56544);
#47667=AXIS2_PLACEMENT_3D('',#83825,#56545,#56546);
#47668=AXIS2_PLACEMENT_3D('',#83826,#56547,#56548);
#47669=AXIS2_PLACEMENT_3D('',#83827,#56549,#56550);
#47670=AXIS2_PLACEMENT_3D('',#83828,#56551,#56552);
#47671=AXIS2_PLACEMENT_3D('',#83829,#56553,#56554);
#47672=AXIS2_PLACEMENT_3D('',#83830,#56555,#56556);
#47673=AXIS2_PLACEMENT_3D('',#83831,#56557,#56558);
#47674=AXIS2_PLACEMENT_3D('',#83832,#56559,#56560);
#47675=AXIS2_PLACEMENT_3D('',#83833,#56561,#56562);
#47676=AXIS2_PLACEMENT_3D('',#83834,#56563,#56564);
#47677=AXIS2_PLACEMENT_3D('',#83835,#56565,#56566);
#47678=AXIS2_PLACEMENT_3D('',#83836,#56567,#56568);
#47679=AXIS2_PLACEMENT_3D('',#83837,#56569,#56570);
#47680=AXIS2_PLACEMENT_3D('',#83838,#56571,#56572);
#47681=AXIS2_PLACEMENT_3D('',#83839,#56573,#56574);
#47682=AXIS2_PLACEMENT_3D('',#83840,#56575,#56576);
#47683=AXIS2_PLACEMENT_3D('',#83841,#56577,#56578);
#47684=AXIS2_PLACEMENT_3D('',#83842,#56579,#56580);
#47685=AXIS2_PLACEMENT_3D('',#83843,#56581,#56582);
#47686=AXIS2_PLACEMENT_3D('',#83844,#56583,#56584);
#47687=AXIS2_PLACEMENT_3D('',#83845,#56585,#56586);
#47688=AXIS2_PLACEMENT_3D('',#83846,#56587,#56588);
#47689=AXIS2_PLACEMENT_3D('',#83847,#56589,#56590);
#47690=AXIS2_PLACEMENT_3D('',#83848,#56591,#56592);
#47691=AXIS2_PLACEMENT_3D('',#83849,#56593,#56594);
#47692=AXIS2_PLACEMENT_3D('',#83850,#56595,#56596);
#47693=AXIS2_PLACEMENT_3D('',#83851,#56597,#56598);
#47694=AXIS2_PLACEMENT_3D('',#83852,#56599,#56600);
#47695=AXIS2_PLACEMENT_3D('',#83853,#56601,#56602);
#47696=AXIS2_PLACEMENT_3D('',#83854,#56603,#56604);
#47697=AXIS2_PLACEMENT_3D('',#83855,#56605,#56606);
#47698=AXIS2_PLACEMENT_3D('',#83856,#56607,#56608);
#47699=AXIS2_PLACEMENT_3D('',#83857,#56609,#56610);
#47700=AXIS2_PLACEMENT_3D('',#83858,#56611,#56612);
#47701=AXIS2_PLACEMENT_3D('',#83859,#56613,#56614);
#47702=AXIS2_PLACEMENT_3D('',#83860,#56615,#56616);
#47703=AXIS2_PLACEMENT_3D('',#83861,#56617,#56618);
#47704=AXIS2_PLACEMENT_3D('',#83862,#56619,#56620);
#47705=AXIS2_PLACEMENT_3D('',#83863,#56621,#56622);
#47706=AXIS2_PLACEMENT_3D('',#83864,#56623,#56624);
#47707=AXIS2_PLACEMENT_3D('',#83865,#56625,#56626);
#47708=AXIS2_PLACEMENT_3D('',#83866,#56627,#56628);
#47709=AXIS2_PLACEMENT_3D('',#83867,#56629,#56630);
#47710=AXIS2_PLACEMENT_3D('',#83868,#56631,#56632);
#47711=AXIS2_PLACEMENT_3D('',#83869,#56633,#56634);
#47712=AXIS2_PLACEMENT_3D('',#83870,#56635,#56636);
#47713=AXIS2_PLACEMENT_3D('',#83871,#56637,#56638);
#47714=AXIS2_PLACEMENT_3D('',#83872,#56639,#56640);
#47715=AXIS2_PLACEMENT_3D('',#83873,#56641,#56642);
#47716=AXIS2_PLACEMENT_3D('',#83874,#56643,#56644);
#47717=AXIS2_PLACEMENT_3D('',#83875,#56645,#56646);
#47718=AXIS2_PLACEMENT_3D('',#83876,#56647,#56648);
#47719=AXIS2_PLACEMENT_3D('',#83877,#56649,#56650);
#47720=AXIS2_PLACEMENT_3D('',#83878,#56651,#56652);
#47721=AXIS2_PLACEMENT_3D('',#83879,#56653,#56654);
#47722=AXIS2_PLACEMENT_3D('',#83880,#56655,#56656);
#47723=AXIS2_PLACEMENT_3D('',#83881,#56657,#56658);
#47724=AXIS2_PLACEMENT_3D('',#83882,#56659,#56660);
#47725=AXIS2_PLACEMENT_3D('',#83883,#56661,#56662);
#47726=AXIS2_PLACEMENT_3D('',#83884,#56663,#56664);
#47727=AXIS2_PLACEMENT_3D('',#83885,#56665,#56666);
#47728=AXIS2_PLACEMENT_3D('',#83886,#56667,#56668);
#47729=AXIS2_PLACEMENT_3D('',#83887,#56669,#56670);
#47730=AXIS2_PLACEMENT_3D('',#83888,#56671,#56672);
#47731=AXIS2_PLACEMENT_3D('',#83889,#56673,#56674);
#47732=AXIS2_PLACEMENT_3D('',#83890,#56675,#56676);
#47733=AXIS2_PLACEMENT_3D('',#83891,#56677,#56678);
#47734=AXIS2_PLACEMENT_3D('',#83892,#56679,#56680);
#47735=AXIS2_PLACEMENT_3D('',#83893,#56681,#56682);
#47736=AXIS2_PLACEMENT_3D('',#83894,#56683,#56684);
#47737=AXIS2_PLACEMENT_3D('',#83895,#56685,#56686);
#47738=AXIS2_PLACEMENT_3D('',#83896,#56687,#56688);
#47739=AXIS2_PLACEMENT_3D('',#83897,#56689,#56690);
#47740=AXIS2_PLACEMENT_3D('',#83898,#56691,#56692);
#47741=AXIS2_PLACEMENT_3D('',#83899,#56693,#56694);
#47742=AXIS2_PLACEMENT_3D('',#83900,#56695,#56696);
#47743=AXIS2_PLACEMENT_3D('',#83901,#56697,#56698);
#47744=AXIS2_PLACEMENT_3D('',#83902,#56699,#56700);
#47745=AXIS2_PLACEMENT_3D('',#83903,#56701,#56702);
#47746=AXIS2_PLACEMENT_3D('',#83904,#56703,#56704);
#47747=AXIS2_PLACEMENT_3D('',#83905,#56705,#56706);
#47748=AXIS2_PLACEMENT_3D('',#83906,#56707,#56708);
#47749=AXIS2_PLACEMENT_3D('',#83907,#56709,#56710);
#47750=AXIS2_PLACEMENT_3D('',#83908,#56711,#56712);
#47751=AXIS2_PLACEMENT_3D('',#83909,#56713,#56714);
#47752=AXIS2_PLACEMENT_3D('',#83910,#56715,#56716);
#47753=AXIS2_PLACEMENT_3D('',#83911,#56717,#56718);
#47754=AXIS2_PLACEMENT_3D('',#83912,#56719,#56720);
#47755=AXIS2_PLACEMENT_3D('',#83913,#56721,#56722);
#47756=AXIS2_PLACEMENT_3D('',#83914,#56723,#56724);
#47757=AXIS2_PLACEMENT_3D('',#83915,#56725,#56726);
#47758=AXIS2_PLACEMENT_3D('',#83916,#56727,#56728);
#47759=AXIS2_PLACEMENT_3D('',#83917,#56729,#56730);
#47760=AXIS2_PLACEMENT_3D('',#83918,#56731,#56732);
#47761=AXIS2_PLACEMENT_3D('',#83919,#56733,#56734);
#47762=AXIS2_PLACEMENT_3D('',#83920,#56735,#56736);
#47763=AXIS2_PLACEMENT_3D('',#83921,#56737,#56738);
#47764=AXIS2_PLACEMENT_3D('',#83922,#56739,#56740);
#47765=AXIS2_PLACEMENT_3D('',#83923,#56741,#56742);
#47766=AXIS2_PLACEMENT_3D('',#83924,#56743,#56744);
#47767=AXIS2_PLACEMENT_3D('',#83925,#56745,#56746);
#47768=AXIS2_PLACEMENT_3D('',#83926,#56747,#56748);
#47769=AXIS2_PLACEMENT_3D('',#83927,#56749,#56750);
#47770=AXIS2_PLACEMENT_3D('',#83928,#56751,#56752);
#47771=AXIS2_PLACEMENT_3D('',#83929,#56753,#56754);
#47772=AXIS2_PLACEMENT_3D('',#83930,#56755,#56756);
#47773=AXIS2_PLACEMENT_3D('',#83931,#56757,#56758);
#47774=AXIS2_PLACEMENT_3D('',#83932,#56759,#56760);
#47775=AXIS2_PLACEMENT_3D('',#83933,#56761,#56762);
#47776=AXIS2_PLACEMENT_3D('',#83934,#56763,#56764);
#47777=AXIS2_PLACEMENT_3D('',#83935,#56765,#56766);
#47778=AXIS2_PLACEMENT_3D('',#83936,#56767,#56768);
#47779=AXIS2_PLACEMENT_3D('',#83937,#56769,#56770);
#47780=AXIS2_PLACEMENT_3D('',#83938,#56771,#56772);
#47781=AXIS2_PLACEMENT_3D('',#83939,#56773,#56774);
#47782=AXIS2_PLACEMENT_3D('',#83940,#56775,#56776);
#47783=AXIS2_PLACEMENT_3D('',#83941,#56777,#56778);
#47784=AXIS2_PLACEMENT_3D('',#83942,#56779,#56780);
#47785=AXIS2_PLACEMENT_3D('',#83943,#56781,#56782);
#47786=AXIS2_PLACEMENT_3D('',#83944,#56783,#56784);
#47787=AXIS2_PLACEMENT_3D('',#83945,#56785,#56786);
#47788=AXIS2_PLACEMENT_3D('',#83946,#56787,#56788);
#47789=AXIS2_PLACEMENT_3D('',#83947,#56789,#56790);
#47790=AXIS2_PLACEMENT_3D('',#83948,#56791,#56792);
#47791=AXIS2_PLACEMENT_3D('',#83949,#56793,#56794);
#47792=AXIS2_PLACEMENT_3D('',#83950,#56795,#56796);
#47793=AXIS2_PLACEMENT_3D('',#83951,#56797,#56798);
#47794=AXIS2_PLACEMENT_3D('',#83952,#56799,#56800);
#47795=AXIS2_PLACEMENT_3D('',#83953,#56801,#56802);
#47796=AXIS2_PLACEMENT_3D('',#83954,#56803,#56804);
#47797=AXIS2_PLACEMENT_3D('',#83955,#56805,#56806);
#47798=AXIS2_PLACEMENT_3D('',#83956,#56807,#56808);
#47799=AXIS2_PLACEMENT_3D('',#83957,#56809,#56810);
#47800=AXIS2_PLACEMENT_3D('',#83958,#56811,#56812);
#47801=AXIS2_PLACEMENT_3D('',#83959,#56813,#56814);
#47802=AXIS2_PLACEMENT_3D('',#83960,#56815,#56816);
#47803=AXIS2_PLACEMENT_3D('',#83961,#56817,#56818);
#47804=AXIS2_PLACEMENT_3D('',#83962,#56819,#56820);
#47805=AXIS2_PLACEMENT_3D('',#83963,#56821,#56822);
#47806=AXIS2_PLACEMENT_3D('',#83964,#56823,#56824);
#47807=AXIS2_PLACEMENT_3D('',#83965,#56825,#56826);
#47808=AXIS2_PLACEMENT_3D('',#83966,#56827,#56828);
#47809=AXIS2_PLACEMENT_3D('',#83967,#56829,#56830);
#47810=AXIS2_PLACEMENT_3D('',#83968,#56831,#56832);
#47811=AXIS2_PLACEMENT_3D('',#83969,#56833,#56834);
#47812=AXIS2_PLACEMENT_3D('',#83970,#56835,#56836);
#47813=AXIS2_PLACEMENT_3D('',#83971,#56837,#56838);
#47814=AXIS2_PLACEMENT_3D('',#83972,#56839,#56840);
#47815=AXIS2_PLACEMENT_3D('',#83973,#56841,#56842);
#47816=AXIS2_PLACEMENT_3D('',#83974,#56843,#56844);
#47817=AXIS2_PLACEMENT_3D('',#83975,#56845,#56846);
#47818=AXIS2_PLACEMENT_3D('',#83976,#56847,#56848);
#47819=AXIS2_PLACEMENT_3D('',#83977,#56849,#56850);
#47820=AXIS2_PLACEMENT_3D('',#83978,#56851,#56852);
#47821=AXIS2_PLACEMENT_3D('',#83979,#56853,#56854);
#47822=AXIS2_PLACEMENT_3D('',#83980,#56855,#56856);
#47823=AXIS2_PLACEMENT_3D('',#83981,#56857,#56858);
#47824=AXIS2_PLACEMENT_3D('',#83982,#56859,#56860);
#47825=AXIS2_PLACEMENT_3D('',#83983,#56861,#56862);
#47826=AXIS2_PLACEMENT_3D('',#83984,#56863,#56864);
#47827=AXIS2_PLACEMENT_3D('',#83985,#56865,#56866);
#47828=AXIS2_PLACEMENT_3D('',#83986,#56867,#56868);
#47829=AXIS2_PLACEMENT_3D('',#83987,#56869,#56870);
#47830=AXIS2_PLACEMENT_3D('',#83988,#56871,#56872);
#47831=AXIS2_PLACEMENT_3D('',#83989,#56873,#56874);
#47832=AXIS2_PLACEMENT_3D('',#83990,#56875,#56876);
#47833=AXIS2_PLACEMENT_3D('',#83991,#56877,#56878);
#47834=AXIS2_PLACEMENT_3D('',#83992,#56879,#56880);
#47835=AXIS2_PLACEMENT_3D('',#83993,#56881,#56882);
#47836=AXIS2_PLACEMENT_3D('',#83994,#56883,#56884);
#47837=AXIS2_PLACEMENT_3D('',#83995,#56885,#56886);
#47838=AXIS2_PLACEMENT_3D('',#83996,#56887,#56888);
#47839=AXIS2_PLACEMENT_3D('',#83997,#56889,#56890);
#47840=AXIS2_PLACEMENT_3D('',#83998,#56891,#56892);
#47841=AXIS2_PLACEMENT_3D('',#83999,#56893,#56894);
#47842=AXIS2_PLACEMENT_3D('',#84000,#56895,#56896);
#47843=AXIS2_PLACEMENT_3D('',#84001,#56897,#56898);
#47844=AXIS2_PLACEMENT_3D('',#84002,#56899,#56900);
#47845=AXIS2_PLACEMENT_3D('',#84003,#56901,#56902);
#47846=AXIS2_PLACEMENT_3D('',#84004,#56903,#56904);
#47847=AXIS2_PLACEMENT_3D('',#84005,#56905,#56906);
#47848=AXIS2_PLACEMENT_3D('',#84006,#56907,#56908);
#47849=AXIS2_PLACEMENT_3D('',#84007,#56909,#56910);
#47850=AXIS2_PLACEMENT_3D('',#84008,#56911,#56912);
#47851=AXIS2_PLACEMENT_3D('',#84009,#56913,#56914);
#47852=AXIS2_PLACEMENT_3D('',#84010,#56915,#56916);
#47853=AXIS2_PLACEMENT_3D('',#84011,#56917,#56918);
#47854=AXIS2_PLACEMENT_3D('',#84012,#56919,#56920);
#47855=AXIS2_PLACEMENT_3D('',#84013,#56921,#56922);
#47856=AXIS2_PLACEMENT_3D('',#84014,#56923,#56924);
#47857=AXIS2_PLACEMENT_3D('',#84015,#56925,#56926);
#47858=AXIS2_PLACEMENT_3D('',#84016,#56927,#56928);
#47859=AXIS2_PLACEMENT_3D('',#84017,#56929,#56930);
#47860=AXIS2_PLACEMENT_3D('',#84018,#56931,#56932);
#47861=AXIS2_PLACEMENT_3D('',#84019,#56933,#56934);
#47862=AXIS2_PLACEMENT_3D('',#84020,#56935,#56936);
#47863=AXIS2_PLACEMENT_3D('',#84021,#56937,#56938);
#47864=AXIS2_PLACEMENT_3D('',#84022,#56939,#56940);
#47865=AXIS2_PLACEMENT_3D('',#84023,#56941,#56942);
#47866=AXIS2_PLACEMENT_3D('',#84024,#56943,#56944);
#47867=AXIS2_PLACEMENT_3D('',#84025,#56945,#56946);
#47868=AXIS2_PLACEMENT_3D('',#84026,#56947,#56948);
#47869=AXIS2_PLACEMENT_3D('',#84027,#56949,#56950);
#47870=AXIS2_PLACEMENT_3D('',#84028,#56951,#56952);
#47871=AXIS2_PLACEMENT_3D('',#84029,#56953,#56954);
#47872=AXIS2_PLACEMENT_3D('',#84030,#56955,#56956);
#47873=AXIS2_PLACEMENT_3D('',#84031,#56957,#56958);
#47874=AXIS2_PLACEMENT_3D('',#84032,#56959,#56960);
#47875=AXIS2_PLACEMENT_3D('',#84033,#56961,#56962);
#47876=AXIS2_PLACEMENT_3D('',#84034,#56963,#56964);
#47877=AXIS2_PLACEMENT_3D('',#84035,#56965,#56966);
#47878=AXIS2_PLACEMENT_3D('',#84036,#56967,#56968);
#47879=AXIS2_PLACEMENT_3D('',#84037,#56969,#56970);
#47880=AXIS2_PLACEMENT_3D('',#84038,#56971,#56972);
#47881=AXIS2_PLACEMENT_3D('',#84039,#56973,#56974);
#47882=AXIS2_PLACEMENT_3D('',#84040,#56975,#56976);
#47883=AXIS2_PLACEMENT_3D('',#84041,#56977,#56978);
#47884=AXIS2_PLACEMENT_3D('',#84042,#56979,#56980);
#47885=AXIS2_PLACEMENT_3D('',#84043,#56981,#56982);
#47886=AXIS2_PLACEMENT_3D('',#84044,#56983,#56984);
#47887=AXIS2_PLACEMENT_3D('',#84045,#56985,#56986);
#47888=AXIS2_PLACEMENT_3D('',#84046,#56987,#56988);
#47889=AXIS2_PLACEMENT_3D('',#84047,#56989,#56990);
#47890=AXIS2_PLACEMENT_3D('',#84048,#56991,#56992);
#47891=AXIS2_PLACEMENT_3D('',#84049,#56993,#56994);
#47892=AXIS2_PLACEMENT_3D('',#84050,#56995,#56996);
#47893=AXIS2_PLACEMENT_3D('',#84051,#56997,#56998);
#47894=AXIS2_PLACEMENT_3D('',#84052,#56999,#57000);
#47895=AXIS2_PLACEMENT_3D('',#84053,#57001,#57002);
#47896=AXIS2_PLACEMENT_3D('',#84054,#57003,#57004);
#47897=AXIS2_PLACEMENT_3D('',#84055,#57005,#57006);
#47898=AXIS2_PLACEMENT_3D('',#84056,#57007,#57008);
#47899=AXIS2_PLACEMENT_3D('',#84057,#57009,#57010);
#47900=AXIS2_PLACEMENT_3D('',#84058,#57011,#57012);
#47901=AXIS2_PLACEMENT_3D('',#84059,#57013,#57014);
#47902=AXIS2_PLACEMENT_3D('',#84060,#57015,#57016);
#47903=AXIS2_PLACEMENT_3D('',#84061,#57017,#57018);
#47904=AXIS2_PLACEMENT_3D('',#84062,#57019,#57020);
#47905=AXIS2_PLACEMENT_3D('',#84063,#57021,#57022);
#47906=AXIS2_PLACEMENT_3D('',#84064,#57023,#57024);
#47907=AXIS2_PLACEMENT_3D('',#84065,#57025,#57026);
#47908=AXIS2_PLACEMENT_3D('',#84066,#57027,#57028);
#47909=AXIS2_PLACEMENT_3D('',#84067,#57029,#57030);
#47910=AXIS2_PLACEMENT_3D('',#84068,#57031,#57032);
#47911=AXIS2_PLACEMENT_3D('',#84069,#57033,#57034);
#47912=AXIS2_PLACEMENT_3D('',#84070,#57035,#57036);
#47913=AXIS2_PLACEMENT_3D('',#84071,#57037,#57038);
#47914=AXIS2_PLACEMENT_3D('',#84072,#57039,#57040);
#47915=AXIS2_PLACEMENT_3D('',#84073,#57041,#57042);
#47916=AXIS2_PLACEMENT_3D('',#84074,#57043,#57044);
#47917=AXIS2_PLACEMENT_3D('',#84075,#57045,#57046);
#47918=AXIS2_PLACEMENT_3D('',#84076,#57047,#57048);
#47919=AXIS2_PLACEMENT_3D('',#84077,#57049,#57050);
#47920=AXIS2_PLACEMENT_3D('',#84078,#57051,#57052);
#47921=AXIS2_PLACEMENT_3D('',#84079,#57053,#57054);
#47922=AXIS2_PLACEMENT_3D('',#84080,#57055,#57056);
#47923=AXIS2_PLACEMENT_3D('',#84081,#57057,#57058);
#47924=AXIS2_PLACEMENT_3D('',#84082,#57059,#57060);
#47925=AXIS2_PLACEMENT_3D('',#84083,#57061,#57062);
#47926=AXIS2_PLACEMENT_3D('',#84084,#57063,#57064);
#47927=AXIS2_PLACEMENT_3D('',#84085,#57065,#57066);
#47928=AXIS2_PLACEMENT_3D('',#84086,#57067,#57068);
#47929=AXIS2_PLACEMENT_3D('',#84087,#57069,#57070);
#47930=AXIS2_PLACEMENT_3D('',#84088,#57071,#57072);
#47931=AXIS2_PLACEMENT_3D('',#84089,#57073,#57074);
#47932=AXIS2_PLACEMENT_3D('',#84090,#57075,#57076);
#47933=AXIS2_PLACEMENT_3D('',#84091,#57077,#57078);
#47934=AXIS2_PLACEMENT_3D('',#84092,#57079,#57080);
#47935=AXIS2_PLACEMENT_3D('',#84093,#57081,#57082);
#47936=AXIS2_PLACEMENT_3D('',#84094,#57083,#57084);
#47937=AXIS2_PLACEMENT_3D('',#84095,#57085,#57086);
#47938=AXIS2_PLACEMENT_3D('',#84096,#57087,#57088);
#47939=AXIS2_PLACEMENT_3D('',#84097,#57089,#57090);
#47940=AXIS2_PLACEMENT_3D('',#84098,#57091,#57092);
#47941=AXIS2_PLACEMENT_3D('',#84099,#57093,#57094);
#47942=AXIS2_PLACEMENT_3D('',#84100,#57095,#57096);
#47943=AXIS2_PLACEMENT_3D('',#84101,#57097,#57098);
#47944=AXIS2_PLACEMENT_3D('',#84102,#57099,#57100);
#47945=AXIS2_PLACEMENT_3D('',#84103,#57101,#57102);
#47946=AXIS2_PLACEMENT_3D('',#84104,#57103,#57104);
#47947=AXIS2_PLACEMENT_3D('',#84105,#57105,#57106);
#47948=AXIS2_PLACEMENT_3D('',#84106,#57107,#57108);
#47949=AXIS2_PLACEMENT_3D('',#84107,#57109,#57110);
#47950=AXIS2_PLACEMENT_3D('',#84108,#57111,#57112);
#47951=AXIS2_PLACEMENT_3D('',#84109,#57113,#57114);
#47952=AXIS2_PLACEMENT_3D('',#84110,#57115,#57116);
#47953=AXIS2_PLACEMENT_3D('',#84111,#57117,#57118);
#47954=AXIS2_PLACEMENT_3D('',#84112,#57119,#57120);
#47955=AXIS2_PLACEMENT_3D('',#84113,#57121,#57122);
#47956=AXIS2_PLACEMENT_3D('',#84114,#57123,#57124);
#47957=AXIS2_PLACEMENT_3D('',#84115,#57125,#57126);
#47958=AXIS2_PLACEMENT_3D('',#84116,#57127,#57128);
#47959=AXIS2_PLACEMENT_3D('',#84117,#57129,#57130);
#47960=AXIS2_PLACEMENT_3D('',#84118,#57131,#57132);
#47961=AXIS2_PLACEMENT_3D('',#84119,#57133,#57134);
#47962=AXIS2_PLACEMENT_3D('',#84120,#57135,#57136);
#47963=AXIS2_PLACEMENT_3D('',#84121,#57137,#57138);
#47964=AXIS2_PLACEMENT_3D('',#84122,#57139,#57140);
#47965=AXIS2_PLACEMENT_3D('',#84123,#57141,#57142);
#47966=AXIS2_PLACEMENT_3D('',#84124,#57143,#57144);
#47967=AXIS2_PLACEMENT_3D('',#84125,#57145,#57146);
#47968=AXIS2_PLACEMENT_3D('',#84126,#57147,#57148);
#47969=AXIS2_PLACEMENT_3D('',#84127,#57149,#57150);
#47970=AXIS2_PLACEMENT_3D('',#84128,#57151,#57152);
#47971=AXIS2_PLACEMENT_3D('',#84129,#57153,#57154);
#47972=AXIS2_PLACEMENT_3D('',#84130,#57155,#57156);
#47973=AXIS2_PLACEMENT_3D('',#84131,#57157,#57158);
#47974=AXIS2_PLACEMENT_3D('',#84132,#57159,#57160);
#47975=AXIS2_PLACEMENT_3D('',#84133,#57161,#57162);
#47976=AXIS2_PLACEMENT_3D('',#84134,#57163,#57164);
#47977=AXIS2_PLACEMENT_3D('',#84135,#57165,#57166);
#47978=AXIS2_PLACEMENT_3D('',#84136,#57167,#57168);
#47979=AXIS2_PLACEMENT_3D('',#84137,#57169,#57170);
#47980=AXIS2_PLACEMENT_3D('',#84138,#57171,#57172);
#47981=AXIS2_PLACEMENT_3D('',#84139,#57173,#57174);
#47982=AXIS2_PLACEMENT_3D('',#84140,#57175,#57176);
#47983=AXIS2_PLACEMENT_3D('',#84141,#57177,#57178);
#47984=AXIS2_PLACEMENT_3D('',#84142,#57179,#57180);
#47985=AXIS2_PLACEMENT_3D('',#84143,#57181,#57182);
#47986=AXIS2_PLACEMENT_3D('',#84144,#57183,#57184);
#47987=AXIS2_PLACEMENT_3D('',#84145,#57185,#57186);
#47988=AXIS2_PLACEMENT_3D('',#84146,#57187,#57188);
#47989=AXIS2_PLACEMENT_3D('',#84147,#57189,#57190);
#47990=AXIS2_PLACEMENT_3D('',#84148,#57191,#57192);
#47991=AXIS2_PLACEMENT_3D('',#84149,#57193,#57194);
#47992=AXIS2_PLACEMENT_3D('',#84150,#57195,#57196);
#47993=AXIS2_PLACEMENT_3D('',#84151,#57197,#57198);
#47994=AXIS2_PLACEMENT_3D('',#84152,#57199,#57200);
#47995=AXIS2_PLACEMENT_3D('',#84153,#57201,#57202);
#47996=AXIS2_PLACEMENT_3D('',#84154,#57203,#57204);
#47997=AXIS2_PLACEMENT_3D('',#84155,#57205,#57206);
#47998=AXIS2_PLACEMENT_3D('',#84156,#57207,#57208);
#47999=AXIS2_PLACEMENT_3D('',#84157,#57209,#57210);
#48000=AXIS2_PLACEMENT_3D('',#84158,#57211,#57212);
#48001=AXIS2_PLACEMENT_3D('',#84159,#57213,#57214);
#48002=AXIS2_PLACEMENT_3D('',#84160,#57215,#57216);
#48003=AXIS2_PLACEMENT_3D('',#84161,#57217,#57218);
#48004=AXIS2_PLACEMENT_3D('',#84162,#57219,#57220);
#48005=AXIS2_PLACEMENT_3D('',#84163,#57221,#57222);
#48006=AXIS2_PLACEMENT_3D('',#84164,#57223,#57224);
#48007=AXIS2_PLACEMENT_3D('',#84165,#57225,#57226);
#48008=AXIS2_PLACEMENT_3D('',#84166,#57227,#57228);
#48009=AXIS2_PLACEMENT_3D('',#84167,#57229,#57230);
#48010=AXIS2_PLACEMENT_3D('',#84168,#57231,#57232);
#48011=AXIS2_PLACEMENT_3D('',#84169,#57233,#57234);
#48012=AXIS2_PLACEMENT_3D('',#84170,#57235,#57236);
#48013=AXIS2_PLACEMENT_3D('',#84171,#57237,#57238);
#48014=AXIS2_PLACEMENT_3D('',#84172,#57239,#57240);
#48015=AXIS2_PLACEMENT_3D('',#84173,#57241,#57242);
#48016=AXIS2_PLACEMENT_3D('',#84174,#57243,#57244);
#48017=AXIS2_PLACEMENT_3D('',#84175,#57245,#57246);
#48018=AXIS2_PLACEMENT_3D('',#84176,#57247,#57248);
#48019=AXIS2_PLACEMENT_3D('',#84177,#57249,#57250);
#48020=AXIS2_PLACEMENT_3D('',#84178,#57251,#57252);
#48021=AXIS2_PLACEMENT_3D('',#84179,#57253,#57254);
#48022=AXIS2_PLACEMENT_3D('',#84180,#57255,#57256);
#48023=AXIS2_PLACEMENT_3D('',#84181,#57257,#57258);
#48024=AXIS2_PLACEMENT_3D('',#84182,#57259,#57260);
#48025=AXIS2_PLACEMENT_3D('',#84183,#57261,#57262);
#48026=AXIS2_PLACEMENT_3D('',#84184,#57263,#57264);
#48027=AXIS2_PLACEMENT_3D('',#84185,#57265,#57266);
#48028=AXIS2_PLACEMENT_3D('',#84186,#57267,#57268);
#48029=AXIS2_PLACEMENT_3D('',#84187,#57269,#57270);
#48030=AXIS2_PLACEMENT_3D('',#84188,#57271,#57272);
#48031=AXIS2_PLACEMENT_3D('',#84189,#57273,#57274);
#48032=AXIS2_PLACEMENT_3D('',#84190,#57275,#57276);
#48033=AXIS2_PLACEMENT_3D('',#84191,#57277,#57278);
#48034=AXIS2_PLACEMENT_3D('',#84192,#57279,#57280);
#48035=AXIS2_PLACEMENT_3D('',#84193,#57281,#57282);
#48036=AXIS2_PLACEMENT_3D('',#84194,#57283,#57284);
#48037=AXIS2_PLACEMENT_3D('',#84195,#57285,#57286);
#48038=AXIS2_PLACEMENT_3D('',#84196,#57287,#57288);
#48039=AXIS2_PLACEMENT_3D('',#84197,#57289,#57290);
#48040=AXIS2_PLACEMENT_3D('',#84198,#57291,#57292);
#48041=AXIS2_PLACEMENT_3D('',#84199,#57293,#57294);
#48042=AXIS2_PLACEMENT_3D('',#84200,#57295,#57296);
#48043=AXIS2_PLACEMENT_3D('',#84201,#57297,#57298);
#48044=AXIS2_PLACEMENT_3D('',#84202,#57299,#57300);
#48045=AXIS2_PLACEMENT_3D('',#84203,#57301,#57302);
#48046=AXIS2_PLACEMENT_3D('',#84204,#57303,#57304);
#48047=AXIS2_PLACEMENT_3D('',#84205,#57305,#57306);
#48048=AXIS2_PLACEMENT_3D('',#84206,#57307,#57308);
#48049=AXIS2_PLACEMENT_3D('',#84207,#57309,#57310);
#48050=AXIS2_PLACEMENT_3D('',#84208,#57311,#57312);
#48051=AXIS2_PLACEMENT_3D('',#84209,#57313,#57314);
#48052=AXIS2_PLACEMENT_3D('',#84210,#57315,#57316);
#48053=AXIS2_PLACEMENT_3D('',#84211,#57317,#57318);
#48054=AXIS2_PLACEMENT_3D('',#84212,#57319,#57320);
#48055=AXIS2_PLACEMENT_3D('',#84225,#57321,#57322);
#48056=AXIS2_PLACEMENT_3D('',#84238,#57323,#57324);
#48057=AXIS2_PLACEMENT_3D('',#84251,#57325,#57326);
#48058=AXIS2_PLACEMENT_3D('',#84264,#57327,#57328);
#48059=AXIS2_PLACEMENT_3D('',#84277,#57329,#57330);
#48060=AXIS2_PLACEMENT_3D('',#84290,#57331,#57332);
#48061=AXIS2_PLACEMENT_3D('',#84303,#57333,#57334);
#48062=AXIS2_PLACEMENT_3D('',#84316,#57335,#57336);
#48063=AXIS2_PLACEMENT_3D('',#84329,#57337,#57338);
#48064=AXIS2_PLACEMENT_3D('',#84342,#57339,#57340);
#48065=AXIS2_PLACEMENT_3D('',#84355,#57341,#57342);
#48066=AXIS2_PLACEMENT_3D('',#84368,#57343,#57344);
#48067=AXIS2_PLACEMENT_3D('',#84381,#57345,#57346);
#48068=AXIS2_PLACEMENT_3D('',#84394,#57347,#57348);
#48069=AXIS2_PLACEMENT_3D('',#84395,#57349,#57350);
#48070=AXIS2_PLACEMENT_3D('',#84396,#57351,#57352);
#48071=AXIS2_PLACEMENT_3D('',#84409,#57353,#57354);
#48072=AXIS2_PLACEMENT_3D('',#84422,#57355,#57356);
#48073=AXIS2_PLACEMENT_3D('',#84423,#57357,#57358);
#48074=AXIS2_PLACEMENT_3D('',#84424,#57359,#57360);
#48075=AXIS2_PLACEMENT_3D('',#84437,#57361,#57362);
#48076=AXIS2_PLACEMENT_3D('',#84450,#57363,#57364);
#48077=AXIS2_PLACEMENT_3D('',#84451,#57365,#57366);
#48078=AXIS2_PLACEMENT_3D('',#84452,#57367,#57368);
#48079=AXIS2_PLACEMENT_3D('',#84453,#57369,#57370);
#48080=AXIS2_PLACEMENT_3D('',#84454,#57371,#57372);
#48081=AXIS2_PLACEMENT_3D('',#84467,#57373,#57374);
#48082=AXIS2_PLACEMENT_3D('',#84480,#57375,#57376);
#48083=AXIS2_PLACEMENT_3D('',#84481,#57377,#57378);
#48084=AXIS2_PLACEMENT_3D('',#84482,#57379,#57380);
#48085=AXIS2_PLACEMENT_3D('',#84483,#57381,#57382);
#48086=AXIS2_PLACEMENT_3D('',#84484,#57383,#57384);
#48087=AXIS2_PLACEMENT_3D('',#84497,#57385,#57386);
#48088=AXIS2_PLACEMENT_3D('',#84510,#57387,#57388);
#48089=AXIS2_PLACEMENT_3D('',#84523,#57389,#57390);
#48090=AXIS2_PLACEMENT_3D('',#84536,#57391,#57392);
#48091=AXIS2_PLACEMENT_3D('',#84549,#57393,#57394);
#48092=AXIS2_PLACEMENT_3D('',#84562,#57395,#57396);
#48093=AXIS2_PLACEMENT_3D('',#84575,#57397,#57398);
#48094=AXIS2_PLACEMENT_3D('',#84588,#57399,#57400);
#48095=AXIS2_PLACEMENT_3D('',#84601,#57401,#57402);
#48096=AXIS2_PLACEMENT_3D('',#84614,#57403,#57404);
#48097=AXIS2_PLACEMENT_3D('',#84627,#57405,#57406);
#48098=AXIS2_PLACEMENT_3D('',#84640,#57407,#57408);
#48099=AXIS2_PLACEMENT_3D('',#84653,#57409,#57410);
#48100=AXIS2_PLACEMENT_3D('',#84666,#57411,#57412);
#48101=AXIS2_PLACEMENT_3D('',#84679,#57413,#57414);
#48102=AXIS2_PLACEMENT_3D('',#84692,#57415,#57416);
#48103=AXIS2_PLACEMENT_3D('',#84705,#57417,#57418);
#48104=AXIS2_PLACEMENT_3D('',#84718,#57419,#57420);
#48105=AXIS2_PLACEMENT_3D('',#84731,#57421,#57422);
#48106=AXIS2_PLACEMENT_3D('',#84744,#57423,#57424);
#48107=AXIS2_PLACEMENT_3D('',#84757,#57425,#57426);
#48108=AXIS2_PLACEMENT_3D('',#84770,#57427,#57428);
#48109=AXIS2_PLACEMENT_3D('',#84783,#57429,#57430);
#48110=AXIS2_PLACEMENT_3D('',#84796,#57431,#57432);
#48111=AXIS2_PLACEMENT_3D('',#84809,#57433,#57434);
#48112=AXIS2_PLACEMENT_3D('',#84822,#57435,#57436);
#48113=AXIS2_PLACEMENT_3D('',#84835,#57437,#57438);
#48114=AXIS2_PLACEMENT_3D('',#84848,#57439,#57440);
#48115=AXIS2_PLACEMENT_3D('',#84861,#57441,#57442);
#48116=AXIS2_PLACEMENT_3D('',#84874,#57443,#57444);
#48117=AXIS2_PLACEMENT_3D('',#84887,#57445,#57446);
#48118=AXIS2_PLACEMENT_3D('',#84900,#57447,#57448);
#48119=AXIS2_PLACEMENT_3D('',#84913,#57449,#57450);
#48120=AXIS2_PLACEMENT_3D('',#84926,#57451,#57452);
#48121=AXIS2_PLACEMENT_3D('',#84939,#57453,#57454);
#48122=AXIS2_PLACEMENT_3D('',#84952,#57455,#57456);
#48123=AXIS2_PLACEMENT_3D('',#84965,#57457,#57458);
#48124=AXIS2_PLACEMENT_3D('',#84978,#57459,#57460);
#48125=AXIS2_PLACEMENT_3D('',#84991,#57461,#57462);
#48126=AXIS2_PLACEMENT_3D('',#84992,#57463,#57464);
#48127=AXIS2_PLACEMENT_3D('',#84993,#57465,#57466);
#48128=AXIS2_PLACEMENT_3D('',#84994,#57467,#57468);
#48129=AXIS2_PLACEMENT_3D('',#84995,#57469,#57470);
#48130=AXIS2_PLACEMENT_3D('',#84996,#57471,#57472);
#48131=AXIS2_PLACEMENT_3D('',#84997,#57473,#57474);
#48132=AXIS2_PLACEMENT_3D('',#84998,#57475,#57476);
#48133=AXIS2_PLACEMENT_3D('',#84999,#57477,#57478);
#48134=AXIS2_PLACEMENT_3D('',#85000,#57479,#57480);
#48135=AXIS2_PLACEMENT_3D('',#85001,#57481,#57482);
#48136=AXIS2_PLACEMENT_3D('',#85002,#57483,#57484);
#51642=DIRECTION('axis',(0.,0.,1.));
#51643=DIRECTION('refdir',(1.,0.,0.));
#51644=DIRECTION('center_axis',(0.,-0.0958457525203355,0.995396198367168));
#51645=DIRECTION('ref_axis',(1.,0.,0.));
#51646=DIRECTION('',(0.,-0.995396198367168,-0.0958457525203355));
#51647=DIRECTION('center_axis',(0.,0.0958457525203352,-0.995396198367168));
#51648=DIRECTION('ref_axis',(-9.08813207382089E-14,0.995396198367168,0.0958457525203352));
#51649=DIRECTION('',(0.,0.995396198367168,0.0958457525203355));
#51650=DIRECTION('',(-1.,0.,0.));
#51651=DIRECTION('center_axis',(0.,0.,1.));
#51652=DIRECTION('ref_axis',(1.,0.,0.));
#51653=DIRECTION('',(0.,1.,0.));
#51654=DIRECTION('center_axis',(0.,0.,1.));
#51655=DIRECTION('ref_axis',(1.,0.,0.));
#51656=DIRECTION('',(0.,-1.,0.));
#51657=DIRECTION('center_axis',(0.,0.,-1.));
#51658=DIRECTION('ref_axis',(-1.,0.,0.));
#51659=DIRECTION('',(0.,0.,-1.));
#51660=DIRECTION('',(0.,0.,-1.));
#51661=DIRECTION('center_axis',(-1.,0.,0.));
#51662=DIRECTION('ref_axis',(0.,0.,1.));
#51663=DIRECTION('center_axis',(1.,0.,0.));
#51664=DIRECTION('ref_axis',(0.,0.,-1.));
#51665=DIRECTION('center_axis',(0.,0.0958457525203355,-0.995396198367168));
#51666=DIRECTION('ref_axis',(-1.,0.,0.));
#51667=DIRECTION('',(0.,0.0958457525203355,-0.995396198367168));
#51668=DIRECTION('center_axis',(0.,0.0479781285213982,-0.998848386484948));
#51669=DIRECTION('ref_axis',(0.,0.998848386484948,0.0479781285213982));
#51670=DIRECTION('',(0.,0.0958457525203355,-0.995396198367168));
#51671=DIRECTION('center_axis',(0.,2.12953059333849E-15,1.));
#51672=DIRECTION('ref_axis',(0.,-1.,2.12953059333849E-15));
#51673=DIRECTION('center_axis',(1.,0.,0.));
#51674=DIRECTION('ref_axis',(0.,0.,-1.));
#51675=DIRECTION('',(0.,0.,-1.));
#51676=DIRECTION('',(0.,-1.,0.));
#51677=DIRECTION('center_axis',(-1.,0.,0.));
#51678=DIRECTION('ref_axis',(0.,0.,1.));
#51679=DIRECTION('',(0.,0.,-1.));
#51680=DIRECTION('',(0.,1.,0.));
#51681=DIRECTION('center_axis',(0.,0.,1.));
#51682=DIRECTION('ref_axis',(1.,0.,0.));
#51683=DIRECTION('center_axis',(0.,0.,1.));
#51684=DIRECTION('ref_axis',(1.,0.,0.));
#51685=DIRECTION('center_axis',(0.,0.,-1.));
#51686=DIRECTION('ref_axis',(-1.,0.,0.));
#51687=DIRECTION('center_axis',(0.,-0.333233134534162,0.94284446121751));
#51688=DIRECTION('ref_axis',(0.,-0.94284446121751,-0.333233134534162));
#51689=DIRECTION('center_axis',(0.,0.333233134534162,-0.94284446121751));
#51690=DIRECTION('ref_axis',(0.,-0.94284446121751,-0.333233134534162));
#51691=DIRECTION('',(0.,-0.333233134534162,0.94284446121751));
#51692=DIRECTION('center_axis',(0.,0.333233134534159,-0.942844461217511));
#51693=DIRECTION('ref_axis',(0.,-0.942844461217511,-0.333233134534159));
#51694=DIRECTION('center_axis',(0.,-0.333233134534162,0.94284446121751));
#51695=DIRECTION('ref_axis',(0.,-0.94284446121751,-0.333233134534162));
#51696=DIRECTION('center_axis',(0.,0.333233134534159,-0.942844461217511));
#51697=DIRECTION('ref_axis',(0.,-0.942844461217511,-0.333233134534159));
#51698=DIRECTION('',(0.,0.333233134534162,-0.94284446121751));
#51699=DIRECTION('center_axis',(0.,0.333233134534162,-0.94284446121751));
#51700=DIRECTION('ref_axis',(0.,-0.94284446121751,-0.333233134534162));
#51701=DIRECTION('center_axis',(0.,-0.333233134534162,0.94284446121751));
#51702=DIRECTION('ref_axis',(0.,-0.94284446121751,-0.333233134534162));
#51703=DIRECTION('center_axis',(0.,0.333233134534162,-0.94284446121751));
#51704=DIRECTION('ref_axis',(0.,-0.94284446121751,-0.333233134534162));
#51705=DIRECTION('',(0.,-0.333233134534162,0.94284446121751));
#51706=DIRECTION('center_axis',(0.,0.333233134534159,-0.942844461217511));
#51707=DIRECTION('ref_axis',(0.,-0.942844461217511,-0.333233134534159));
#51708=DIRECTION('center_axis',(0.,-0.333233134534162,0.94284446121751));
#51709=DIRECTION('ref_axis',(0.,-0.94284446121751,-0.333233134534162));
#51710=DIRECTION('center_axis',(0.,0.333233134534159,-0.942844461217511));
#51711=DIRECTION('ref_axis',(0.,-0.942844461217511,-0.333233134534159));
#51712=DIRECTION('',(0.,0.333233134534162,-0.94284446121751));
#51713=DIRECTION('center_axis',(0.,0.333233134534162,-0.94284446121751));
#51714=DIRECTION('ref_axis',(0.,-0.94284446121751,-0.333233134534162));
#51715=DIRECTION('center_axis',(0.,-0.333233134534162,0.94284446121751));
#51716=DIRECTION('ref_axis',(0.,-0.94284446121751,-0.333233134534162));
#51717=DIRECTION('center_axis',(0.,0.333233134534162,-0.94284446121751));
#51718=DIRECTION('ref_axis',(0.,-0.94284446121751,-0.333233134534162));
#51719=DIRECTION('',(0.,-0.333233134534162,0.94284446121751));
#51720=DIRECTION('center_axis',(0.,0.333233134534159,-0.942844461217511));
#51721=DIRECTION('ref_axis',(0.,-0.942844461217511,-0.333233134534159));
#51722=DIRECTION('center_axis',(0.,-0.333233134534162,0.94284446121751));
#51723=DIRECTION('ref_axis',(0.,-0.94284446121751,-0.333233134534162));
#51724=DIRECTION('center_axis',(0.,0.333233134534159,-0.942844461217511));
#51725=DIRECTION('ref_axis',(0.,-0.942844461217511,-0.333233134534159));
#51726=DIRECTION('',(0.,0.333233134534162,-0.94284446121751));
#51727=DIRECTION('center_axis',(0.,0.333233134534162,-0.94284446121751));
#51728=DIRECTION('ref_axis',(0.,-0.94284446121751,-0.333233134534162));
#51729=DIRECTION('center_axis',(0.,-0.333233134534162,0.94284446121751));
#51730=DIRECTION('ref_axis',(0.,-0.94284446121751,-0.333233134534162));
#51731=DIRECTION('center_axis',(0.,0.333233134534162,-0.94284446121751));
#51732=DIRECTION('ref_axis',(0.,-0.94284446121751,-0.333233134534162));
#51733=DIRECTION('',(0.,-0.333233134534162,0.94284446121751));
#51734=DIRECTION('center_axis',(0.,0.333233134534159,-0.942844461217511));
#51735=DIRECTION('ref_axis',(0.,-0.942844461217511,-0.333233134534159));
#51736=DIRECTION('center_axis',(0.,-0.333233134534162,0.94284446121751));
#51737=DIRECTION('ref_axis',(0.,-0.94284446121751,-0.333233134534162));
#51738=DIRECTION('center_axis',(0.,0.333233134534159,-0.942844461217511));
#51739=DIRECTION('ref_axis',(0.,-0.942844461217511,-0.333233134534159));
#51740=DIRECTION('',(0.,0.333233134534162,-0.94284446121751));
#51741=DIRECTION('center_axis',(0.,0.333233134534162,-0.94284446121751));
#51742=DIRECTION('ref_axis',(0.,-0.94284446121751,-0.333233134534162));
#51743=DIRECTION('center_axis',(0.,-0.333233134534162,0.94284446121751));
#51744=DIRECTION('ref_axis',(0.,-0.94284446121751,-0.333233134534162));
#51745=DIRECTION('center_axis',(0.,0.333233134534162,-0.94284446121751));
#51746=DIRECTION('ref_axis',(0.,-0.94284446121751,-0.333233134534162));
#51747=DIRECTION('',(0.,-0.333233134534162,0.94284446121751));
#51748=DIRECTION('center_axis',(0.,0.333233134534159,-0.942844461217511));
#51749=DIRECTION('ref_axis',(0.,-0.942844461217511,-0.333233134534159));
#51750=DIRECTION('center_axis',(0.,-0.333233134534162,0.94284446121751));
#51751=DIRECTION('ref_axis',(0.,-0.94284446121751,-0.333233134534162));
#51752=DIRECTION('center_axis',(0.,0.333233134534159,-0.942844461217511));
#51753=DIRECTION('ref_axis',(0.,-0.942844461217511,-0.333233134534159));
#51754=DIRECTION('',(0.,0.333233134534162,-0.94284446121751));
#51755=DIRECTION('center_axis',(0.,0.333233134534162,-0.94284446121751));
#51756=DIRECTION('ref_axis',(0.,-0.94284446121751,-0.333233134534162));
#51757=DIRECTION('center_axis',(0.,-0.333233134534162,0.94284446121751));
#51758=DIRECTION('ref_axis',(0.,-0.94284446121751,-0.333233134534162));
#51759=DIRECTION('center_axis',(0.,0.333233134534162,-0.94284446121751));
#51760=DIRECTION('ref_axis',(0.,-0.94284446121751,-0.333233134534162));
#51761=DIRECTION('',(0.,-0.333233134534162,0.94284446121751));
#51762=DIRECTION('center_axis',(0.,0.333233134534159,-0.942844461217511));
#51763=DIRECTION('ref_axis',(0.,-0.942844461217511,-0.333233134534159));
#51764=DIRECTION('center_axis',(0.,-0.333233134534162,0.94284446121751));
#51765=DIRECTION('ref_axis',(0.,-0.94284446121751,-0.333233134534162));
#51766=DIRECTION('center_axis',(0.,0.333233134534159,-0.942844461217511));
#51767=DIRECTION('ref_axis',(0.,-0.942844461217511,-0.333233134534159));
#51768=DIRECTION('',(0.,0.333233134534162,-0.94284446121751));
#51769=DIRECTION('center_axis',(0.,0.333233134534162,-0.94284446121751));
#51770=DIRECTION('ref_axis',(0.,-0.94284446121751,-0.333233134534162));
#51771=DIRECTION('center_axis',(0.,-0.333233134534162,0.94284446121751));
#51772=DIRECTION('ref_axis',(0.,-0.94284446121751,-0.333233134534161));
#51773=DIRECTION('',(0.,0.333233134534162,-0.94284446121751));
#51774=DIRECTION('center_axis',(0.,-0.333233134534162,0.94284446121751));
#51775=DIRECTION('ref_axis',(0.,-0.94284446121751,-0.333233134534162));
#51776=DIRECTION('center_axis',(0.,0.333233134534162,-0.94284446121751));
#51777=DIRECTION('ref_axis',(0.,0.94284446121751,0.333233134534162));
#51778=DIRECTION('',(0.,-0.333233134534162,0.94284446121751));
#51779=DIRECTION('center_axis',(0.,-0.333233134534162,0.94284446121751));
#51780=DIRECTION('ref_axis',(0.,-0.94284446121751,-0.333233134534162));
#51781=DIRECTION('',(0.,0.333233134534162,-0.94284446121751));
#51782=DIRECTION('center_axis',(0.,-0.333233134534162,0.94284446121751));
#51783=DIRECTION('ref_axis',(0.,-0.94284446121751,-0.333233134534162));
#51784=DIRECTION('center_axis',(0.,0.333233134534162,-0.94284446121751));
#51785=DIRECTION('ref_axis',(0.,0.94284446121751,0.333233134534162));
#51786=DIRECTION('',(0.,-0.333233134534162,0.94284446121751));
#51787=DIRECTION('center_axis',(0.,-0.333233134534162,0.94284446121751));
#51788=DIRECTION('ref_axis',(0.,-0.94284446121751,-0.333233134534162));
#51789=DIRECTION('',(0.,0.333233134534162,-0.94284446121751));
#51790=DIRECTION('center_axis',(0.,-0.333233134534162,0.94284446121751));
#51791=DIRECTION('ref_axis',(0.,-0.94284446121751,-0.333233134534162));
#51792=DIRECTION('center_axis',(0.,0.333233134534162,-0.94284446121751));
#51793=DIRECTION('ref_axis',(0.,0.94284446121751,0.333233134534162));
#51794=DIRECTION('',(0.,-0.333233134534162,0.94284446121751));
#51795=DIRECTION('center_axis',(0.,-0.333233134534162,0.94284446121751));
#51796=DIRECTION('ref_axis',(0.,-0.94284446121751,-0.333233134534162));
#51797=DIRECTION('',(0.,0.333233134534162,-0.94284446121751));
#51798=DIRECTION('center_axis',(0.,-0.333233134534162,0.94284446121751));
#51799=DIRECTION('ref_axis',(0.,-0.94284446121751,-0.333233134534162));
#51800=DIRECTION('center_axis',(0.,0.333233134534162,-0.94284446121751));
#51801=DIRECTION('ref_axis',(0.,0.94284446121751,0.333233134534162));
#51802=DIRECTION('',(0.,-0.333233134534162,0.94284446121751));
#51803=DIRECTION('center_axis',(0.,-0.333233134534162,0.94284446121751));
#51804=DIRECTION('ref_axis',(0.,-0.94284446121751,-0.333233134534162));
#51805=DIRECTION('',(0.,0.333233134534162,-0.94284446121751));
#51806=DIRECTION('center_axis',(0.,-0.333233134534162,0.94284446121751));
#51807=DIRECTION('ref_axis',(0.,-0.94284446121751,-0.333233134534162));
#51808=DIRECTION('center_axis',(0.,0.333233134534162,-0.94284446121751));
#51809=DIRECTION('ref_axis',(0.,0.94284446121751,0.333233134534162));
#51810=DIRECTION('',(0.,-0.333233134534162,0.94284446121751));
#51811=DIRECTION('center_axis',(0.,-0.333233134534162,0.94284446121751));
#51812=DIRECTION('ref_axis',(0.,-0.94284446121751,-0.333233134534162));
#51813=DIRECTION('',(0.,0.333233134534162,-0.94284446121751));
#51814=DIRECTION('center_axis',(0.,-0.333233134534162,0.94284446121751));
#51815=DIRECTION('ref_axis',(0.,-0.94284446121751,-0.333233134534162));
#51816=DIRECTION('center_axis',(0.,0.333233134534162,-0.94284446121751));
#51817=DIRECTION('ref_axis',(0.,0.94284446121751,0.333233134534162));
#51818=DIRECTION('',(0.,-0.333233134534162,0.94284446121751));
#51819=DIRECTION('center_axis',(0.,-0.333233134534162,0.94284446121751));
#51820=DIRECTION('ref_axis',(0.,-0.94284446121751,-0.333233134534161));
#51821=DIRECTION('',(0.,0.333233134534162,-0.94284446121751));
#51822=DIRECTION('center_axis',(0.,-0.333233134534162,0.94284446121751));
#51823=DIRECTION('ref_axis',(0.,-0.94284446121751,-0.333233134534162));
#51824=DIRECTION('center_axis',(0.,0.333233134534162,-0.94284446121751));
#51825=DIRECTION('ref_axis',(0.,0.94284446121751,0.333233134534162));
#51826=DIRECTION('',(0.,-0.333233134534162,0.94284446121751));
#51827=DIRECTION('center_axis',(0.,-0.333233134534162,0.94284446121751));
#51828=DIRECTION('ref_axis',(0.,-0.94284446121751,-0.333233134534162));
#51829=DIRECTION('',(0.,0.333233134534162,-0.94284446121751));
#51830=DIRECTION('center_axis',(0.,-0.333233134534162,0.94284446121751));
#51831=DIRECTION('ref_axis',(0.,-0.94284446121751,-0.333233134534162));
#51832=DIRECTION('center_axis',(0.,0.333233134534162,-0.94284446121751));
#51833=DIRECTION('ref_axis',(0.,0.94284446121751,0.333233134534162));
#51834=DIRECTION('',(0.,-0.333233134534162,0.94284446121751));
#51835=DIRECTION('center_axis',(0.,-0.333233134534162,0.94284446121751));
#51836=DIRECTION('ref_axis',(0.,-0.94284446121751,-0.333233134534161));
#51837=DIRECTION('',(0.,0.333233134534162,-0.94284446121751));
#51838=DIRECTION('center_axis',(0.,-0.333233134534162,0.94284446121751));
#51839=DIRECTION('ref_axis',(0.,-0.94284446121751,-0.333233134534162));
#51840=DIRECTION('center_axis',(0.,0.333233134534162,-0.94284446121751));
#51841=DIRECTION('ref_axis',(0.,0.94284446121751,0.333233134534162));
#51842=DIRECTION('',(0.,-0.333233134534162,0.94284446121751));
#51843=DIRECTION('center_axis',(0.,-0.333233134534162,0.94284446121751));
#51844=DIRECTION('ref_axis',(0.,-0.94284446121751,-0.333233134534162));
#51845=DIRECTION('',(0.,0.333233134534162,-0.94284446121751));
#51846=DIRECTION('center_axis',(0.,-0.333233134534162,0.94284446121751));
#51847=DIRECTION('ref_axis',(0.,-0.94284446121751,-0.333233134534162));
#51848=DIRECTION('center_axis',(0.,0.333233134534162,-0.94284446121751));
#51849=DIRECTION('ref_axis',(0.,0.94284446121751,0.333233134534162));
#51850=DIRECTION('',(0.,-0.333233134534162,0.94284446121751));
#51851=DIRECTION('center_axis',(0.,-0.333233134534162,0.94284446121751));
#51852=DIRECTION('ref_axis',(0.,-0.94284446121751,-0.333233134534161));
#51853=DIRECTION('',(0.,0.333233134534162,-0.94284446121751));
#51854=DIRECTION('center_axis',(0.,-0.333233134534162,0.94284446121751));
#51855=DIRECTION('ref_axis',(0.,-0.94284446121751,-0.333233134534162));
#51856=DIRECTION('center_axis',(0.,0.333233134534162,-0.94284446121751));
#51857=DIRECTION('ref_axis',(0.,0.94284446121751,0.333233134534162));
#51858=DIRECTION('',(0.,-0.333233134534162,0.94284446121751));
#51859=DIRECTION('center_axis',(0.,-0.333233134534162,0.94284446121751));
#51860=DIRECTION('ref_axis',(0.,-0.94284446121751,-0.333233134534162));
#51861=DIRECTION('',(0.,0.333233134534162,-0.94284446121751));
#51862=DIRECTION('center_axis',(0.,-0.333233134534162,0.94284446121751));
#51863=DIRECTION('ref_axis',(0.,-0.94284446121751,-0.333233134534162));
#51864=DIRECTION('center_axis',(0.,0.333233134534162,-0.94284446121751));
#51865=DIRECTION('ref_axis',(0.,0.94284446121751,0.333233134534162));
#51866=DIRECTION('',(0.,-0.333233134534162,0.94284446121751));
#51867=DIRECTION('center_axis',(0.,-0.333233134534162,0.94284446121751));
#51868=DIRECTION('ref_axis',(0.,-0.94284446121751,-0.333233134534161));
#51869=DIRECTION('',(0.,0.333233134534162,-0.94284446121751));
#51870=DIRECTION('center_axis',(0.,-0.333233134534162,0.94284446121751));
#51871=DIRECTION('ref_axis',(0.,-0.94284446121751,-0.333233134534162));
#51872=DIRECTION('center_axis',(0.,0.333233134534162,-0.94284446121751));
#51873=DIRECTION('ref_axis',(0.,0.94284446121751,0.333233134534162));
#51874=DIRECTION('',(0.,-0.333233134534162,0.94284446121751));
#51875=DIRECTION('center_axis',(0.,-0.333233134534162,0.94284446121751));
#51876=DIRECTION('ref_axis',(0.,-0.94284446121751,-0.333233134534162));
#51877=DIRECTION('',(0.,0.333233134534162,-0.94284446121751));
#51878=DIRECTION('center_axis',(0.,-0.333233134534162,0.94284446121751));
#51879=DIRECTION('ref_axis',(0.,-0.94284446121751,-0.333233134534162));
#51880=DIRECTION('center_axis',(0.,0.333233134534162,-0.94284446121751));
#51881=DIRECTION('ref_axis',(0.,0.94284446121751,0.333233134534162));
#51882=DIRECTION('',(0.,-0.333233134534162,0.94284446121751));
#51883=DIRECTION('center_axis',(0.,-0.333233134534162,0.94284446121751));
#51884=DIRECTION('ref_axis',(0.,-0.94284446121751,-0.333233134534162));
#51885=DIRECTION('',(0.,0.333233134534162,-0.94284446121751));
#51886=DIRECTION('center_axis',(0.,-0.333233134534162,0.94284446121751));
#51887=DIRECTION('ref_axis',(0.,-0.94284446121751,-0.333233134534162));
#51888=DIRECTION('center_axis',(0.,0.333233134534162,-0.94284446121751));
#51889=DIRECTION('ref_axis',(0.,0.94284446121751,0.333233134534162));
#51890=DIRECTION('',(0.,-0.333233134534162,0.94284446121751));
#51891=DIRECTION('center_axis',(0.,-0.333233134534162,0.94284446121751));
#51892=DIRECTION('ref_axis',(0.,-0.94284446121751,-0.333233134534162));
#51893=DIRECTION('',(0.,0.333233134534162,-0.94284446121751));
#51894=DIRECTION('center_axis',(0.,-0.333233134534162,0.94284446121751));
#51895=DIRECTION('ref_axis',(0.,-0.94284446121751,-0.333233134534162));
#51896=DIRECTION('center_axis',(0.,0.333233134534162,-0.94284446121751));
#51897=DIRECTION('ref_axis',(0.,0.94284446121751,0.333233134534162));
#51898=DIRECTION('',(0.,-0.333233134534162,0.94284446121751));
#51899=DIRECTION('center_axis',(0.,-0.333233134534162,0.94284446121751));
#51900=DIRECTION('ref_axis',(0.,-0.94284446121751,-0.333233134534161));
#51901=DIRECTION('',(0.,0.333233134534162,-0.94284446121751));
#51902=DIRECTION('center_axis',(0.,-0.333233134534162,0.94284446121751));
#51903=DIRECTION('ref_axis',(0.,-0.94284446121751,-0.333233134534162));
#51904=DIRECTION('center_axis',(0.,0.333233134534162,-0.94284446121751));
#51905=DIRECTION('ref_axis',(0.,0.94284446121751,0.333233134534162));
#51906=DIRECTION('',(0.,-0.333233134534162,0.94284446121751));
#51907=DIRECTION('center_axis',(0.,-0.333233134534162,0.94284446121751));
#51908=DIRECTION('ref_axis',(0.,-0.94284446121751,-0.333233134534162));
#51909=DIRECTION('',(0.,0.333233134534162,-0.94284446121751));
#51910=DIRECTION('center_axis',(0.,-0.333233134534162,0.94284446121751));
#51911=DIRECTION('ref_axis',(0.,-0.94284446121751,-0.333233134534162));
#51912=DIRECTION('center_axis',(0.,0.333233134534162,-0.94284446121751));
#51913=DIRECTION('ref_axis',(0.,0.94284446121751,0.333233134534162));
#51914=DIRECTION('',(0.,-0.333233134534162,0.94284446121751));
#51915=DIRECTION('center_axis',(0.,-0.333233134534162,0.94284446121751));
#51916=DIRECTION('ref_axis',(0.,-0.94284446121751,-0.333233134534162));
#51917=DIRECTION('',(0.,0.333233134534162,-0.94284446121751));
#51918=DIRECTION('center_axis',(0.,-0.333233134534162,0.94284446121751));
#51919=DIRECTION('ref_axis',(0.,-0.94284446121751,-0.333233134534162));
#51920=DIRECTION('center_axis',(0.,0.333233134534162,-0.94284446121751));
#51921=DIRECTION('ref_axis',(0.,0.94284446121751,0.333233134534162));
#51922=DIRECTION('',(0.,-0.333233134534162,0.94284446121751));
#51923=DIRECTION('center_axis',(0.,-0.333233134534162,0.94284446121751));
#51924=DIRECTION('ref_axis',(0.,-0.94284446121751,-0.333233134534162));
#51925=DIRECTION('',(0.,0.333233134534162,-0.94284446121751));
#51926=DIRECTION('center_axis',(0.,-0.333233134534162,0.94284446121751));
#51927=DIRECTION('ref_axis',(0.,-0.94284446121751,-0.333233134534162));
#51928=DIRECTION('center_axis',(0.,0.333233134534162,-0.94284446121751));
#51929=DIRECTION('ref_axis',(0.,0.94284446121751,0.333233134534162));
#51930=DIRECTION('',(0.,-0.333233134534162,0.94284446121751));
#51931=DIRECTION('center_axis',(0.,-0.333233134534162,0.94284446121751));
#51932=DIRECTION('ref_axis',(0.,-0.94284446121751,-0.333233134534162));
#51933=DIRECTION('',(0.,0.333233134534162,-0.94284446121751));
#51934=DIRECTION('center_axis',(0.,-0.333233134534162,0.94284446121751));
#51935=DIRECTION('ref_axis',(0.,-0.94284446121751,-0.333233134534162));
#51936=DIRECTION('center_axis',(0.,0.333233134534162,-0.94284446121751));
#51937=DIRECTION('ref_axis',(0.,0.94284446121751,0.333233134534162));
#51938=DIRECTION('',(0.,-0.333233134534162,0.94284446121751));
#51939=DIRECTION('center_axis',(0.,-0.333233134534162,0.94284446121751));
#51940=DIRECTION('ref_axis',(0.,-0.94284446121751,-0.333233134534162));
#51941=DIRECTION('',(0.,0.333233134534162,-0.94284446121751));
#51942=DIRECTION('center_axis',(0.,-0.333233134534162,0.94284446121751));
#51943=DIRECTION('ref_axis',(0.,-0.94284446121751,-0.333233134534162));
#51944=DIRECTION('center_axis',(0.,0.333233134534162,-0.94284446121751));
#51945=DIRECTION('ref_axis',(0.,0.94284446121751,0.333233134534162));
#51946=DIRECTION('',(0.,-0.333233134534162,0.94284446121751));
#51947=DIRECTION('center_axis',(0.,-0.333233134534162,0.94284446121751));
#51948=DIRECTION('ref_axis',(0.,-0.94284446121751,-0.333233134534161));
#51949=DIRECTION('',(0.,0.333233134534162,-0.94284446121751));
#51950=DIRECTION('center_axis',(0.,-0.333233134534162,0.94284446121751));
#51951=DIRECTION('ref_axis',(0.,-0.94284446121751,-0.333233134534162));
#51952=DIRECTION('center_axis',(0.,0.333233134534162,-0.94284446121751));
#51953=DIRECTION('ref_axis',(0.,0.94284446121751,0.333233134534162));
#51954=DIRECTION('',(0.,-0.333233134534162,0.94284446121751));
#51955=DIRECTION('center_axis',(0.,-0.333233134534162,0.94284446121751));
#51956=DIRECTION('ref_axis',(0.,-0.94284446121751,-0.333233134534162));
#51957=DIRECTION('',(0.,0.333233134534162,-0.94284446121751));
#51958=DIRECTION('center_axis',(0.,-0.333233134534162,0.94284446121751));
#51959=DIRECTION('ref_axis',(0.,-0.94284446121751,-0.333233134534162));
#51960=DIRECTION('center_axis',(0.,0.333233134534162,-0.94284446121751));
#51961=DIRECTION('ref_axis',(0.,0.94284446121751,0.333233134534162));
#51962=DIRECTION('',(0.,-0.333233134534162,0.94284446121751));
#51963=DIRECTION('center_axis',(0.,-0.333233134534162,0.94284446121751));
#51964=DIRECTION('ref_axis',(0.,-0.94284446121751,-0.333233134534161));
#51965=DIRECTION('',(0.,0.333233134534162,-0.94284446121751));
#51966=DIRECTION('center_axis',(0.,-0.333233134534162,0.94284446121751));
#51967=DIRECTION('ref_axis',(0.,-0.94284446121751,-0.333233134534162));
#51968=DIRECTION('center_axis',(0.,0.333233134534162,-0.94284446121751));
#51969=DIRECTION('ref_axis',(0.,0.94284446121751,0.333233134534162));
#51970=DIRECTION('',(0.,-0.333233134534162,0.94284446121751));
#51971=DIRECTION('center_axis',(0.,-0.333233134534162,0.94284446121751));
#51972=DIRECTION('ref_axis',(0.,-0.94284446121751,-0.333233134534162));
#51973=DIRECTION('',(0.,0.333233134534162,-0.94284446121751));
#51974=DIRECTION('center_axis',(0.,-0.333233134534162,0.94284446121751));
#51975=DIRECTION('ref_axis',(0.,-0.94284446121751,-0.333233134534162));
#51976=DIRECTION('center_axis',(0.,0.333233134534162,-0.94284446121751));
#51977=DIRECTION('ref_axis',(0.,0.94284446121751,0.333233134534162));
#51978=DIRECTION('',(0.,-0.333233134534162,0.94284446121751));
#51979=DIRECTION('center_axis',(0.,-0.333233134534162,0.94284446121751));
#51980=DIRECTION('ref_axis',(0.,-0.94284446121751,-0.333233134534162));
#51981=DIRECTION('',(0.,0.333233134534162,-0.94284446121751));
#51982=DIRECTION('center_axis',(0.,-0.333233134534162,0.94284446121751));
#51983=DIRECTION('ref_axis',(0.,-0.94284446121751,-0.333233134534162));
#51984=DIRECTION('center_axis',(0.,0.333233134534162,-0.94284446121751));
#51985=DIRECTION('ref_axis',(0.,0.94284446121751,0.333233134534162));
#51986=DIRECTION('',(0.,-0.333233134534162,0.94284446121751));
#51987=DIRECTION('center_axis',(0.,-0.333233134534162,0.94284446121751));
#51988=DIRECTION('ref_axis',(0.,-0.94284446121751,-0.333233134534162));
#51989=DIRECTION('',(0.,0.333233134534162,-0.94284446121751));
#51990=DIRECTION('center_axis',(0.,-0.333233134534162,0.94284446121751));
#51991=DIRECTION('ref_axis',(0.,-0.94284446121751,-0.333233134534162));
#51992=DIRECTION('center_axis',(0.,0.333233134534162,-0.94284446121751));
#51993=DIRECTION('ref_axis',(0.,0.94284446121751,0.333233134534162));
#51994=DIRECTION('',(0.,-0.333233134534162,0.94284446121751));
#51995=DIRECTION('center_axis',(0.,-0.333233134534162,0.94284446121751));
#51996=DIRECTION('ref_axis',(0.,-0.94284446121751,-0.333233134534161));
#51997=DIRECTION('',(0.,0.333233134534162,-0.94284446121751));
#51998=DIRECTION('center_axis',(0.,-0.333233134534162,0.94284446121751));
#51999=DIRECTION('ref_axis',(0.,-0.94284446121751,-0.333233134534162));
#52000=DIRECTION('center_axis',(0.,0.333233134534162,-0.94284446121751));
#52001=DIRECTION('ref_axis',(0.,0.94284446121751,0.333233134534162));
#52002=DIRECTION('',(0.,-0.333233134534162,0.94284446121751));
#52003=DIRECTION('center_axis',(0.,-0.333233134534162,0.94284446121751));
#52004=DIRECTION('ref_axis',(0.,-0.94284446121751,-0.333233134534162));
#52005=DIRECTION('',(0.,0.333233134534162,-0.94284446121751));
#52006=DIRECTION('center_axis',(0.,-0.333233134534162,0.94284446121751));
#52007=DIRECTION('ref_axis',(0.,-0.94284446121751,-0.333233134534162));
#52008=DIRECTION('center_axis',(0.,0.333233134534162,-0.94284446121751));
#52009=DIRECTION('ref_axis',(0.,0.94284446121751,0.333233134534162));
#52010=DIRECTION('',(0.,-0.333233134534162,0.94284446121751));
#52011=DIRECTION('center_axis',(0.,-0.333233134534162,0.94284446121751));
#52012=DIRECTION('ref_axis',(0.,-0.94284446121751,-0.333233134534162));
#52013=DIRECTION('',(0.,0.333233134534162,-0.94284446121751));
#52014=DIRECTION('center_axis',(0.,-0.333233134534162,0.94284446121751));
#52015=DIRECTION('ref_axis',(0.,-0.94284446121751,-0.333233134534162));
#52016=DIRECTION('center_axis',(0.,0.333233134534162,-0.94284446121751));
#52017=DIRECTION('ref_axis',(0.,0.94284446121751,0.333233134534162));
#52018=DIRECTION('',(0.,-0.333233134534162,0.94284446121751));
#52019=DIRECTION('center_axis',(0.,-0.333233134534162,0.94284446121751));
#52020=DIRECTION('ref_axis',(0.,-0.94284446121751,-0.333233134534162));
#52021=DIRECTION('',(0.,0.333233134534162,-0.94284446121751));
#52022=DIRECTION('center_axis',(0.,-0.333233134534162,0.94284446121751));
#52023=DIRECTION('ref_axis',(0.,-0.94284446121751,-0.333233134534162));
#52024=DIRECTION('center_axis',(0.,0.333233134534162,-0.94284446121751));
#52025=DIRECTION('ref_axis',(0.,0.94284446121751,0.333233134534162));
#52026=DIRECTION('',(0.,-0.333233134534162,0.94284446121751));
#52027=DIRECTION('center_axis',(0.,-0.333233134534162,0.94284446121751));
#52028=DIRECTION('ref_axis',(0.,-0.94284446121751,-0.333233134534162));
#52029=DIRECTION('',(0.,0.333233134534162,-0.94284446121751));
#52030=DIRECTION('center_axis',(0.,-0.333233134534162,0.94284446121751));
#52031=DIRECTION('ref_axis',(0.,-0.94284446121751,-0.333233134534162));
#52032=DIRECTION('center_axis',(0.,0.333233134534162,-0.94284446121751));
#52033=DIRECTION('ref_axis',(0.,0.94284446121751,0.333233134534162));
#52034=DIRECTION('',(0.,-0.333233134534162,0.94284446121751));
#52035=DIRECTION('center_axis',(0.,-0.333233134534162,0.94284446121751));
#52036=DIRECTION('ref_axis',(0.,-0.94284446121751,-0.333233134534162));
#52037=DIRECTION('',(0.,0.333233134534162,-0.94284446121751));
#52038=DIRECTION('center_axis',(0.,-0.333233134534162,0.94284446121751));
#52039=DIRECTION('ref_axis',(0.,-0.94284446121751,-0.333233134534162));
#52040=DIRECTION('center_axis',(0.,0.333233134534162,-0.94284446121751));
#52041=DIRECTION('ref_axis',(0.,0.94284446121751,0.333233134534162));
#52042=DIRECTION('',(0.,-0.333233134534162,0.94284446121751));
#52043=DIRECTION('center_axis',(0.,-0.333233134534162,0.94284446121751));
#52044=DIRECTION('ref_axis',(0.,-0.94284446121751,-0.333233134534162));
#52045=DIRECTION('',(0.,0.333233134534162,-0.94284446121751));
#52046=DIRECTION('center_axis',(0.,-0.333233134534162,0.94284446121751));
#52047=DIRECTION('ref_axis',(0.,-0.94284446121751,-0.333233134534162));
#52048=DIRECTION('center_axis',(0.,0.333233134534162,-0.94284446121751));
#52049=DIRECTION('ref_axis',(0.,0.94284446121751,0.333233134534162));
#52050=DIRECTION('',(0.,-0.333233134534162,0.94284446121751));
#52051=DIRECTION('center_axis',(0.,-0.333233134534162,0.94284446121751));
#52052=DIRECTION('ref_axis',(0.,-0.94284446121751,-0.333233134534162));
#52053=DIRECTION('',(0.,0.333233134534162,-0.94284446121751));
#52054=DIRECTION('center_axis',(0.,-0.333233134534162,0.94284446121751));
#52055=DIRECTION('ref_axis',(0.,-0.94284446121751,-0.333233134534162));
#52056=DIRECTION('center_axis',(0.,0.333233134534162,-0.94284446121751));
#52057=DIRECTION('ref_axis',(0.,0.94284446121751,0.333233134534162));
#52058=DIRECTION('',(0.,-0.333233134534162,0.94284446121751));
#52059=DIRECTION('center_axis',(0.,-0.333233134534162,0.94284446121751));
#52060=DIRECTION('ref_axis',(0.,-0.94284446121751,-0.333233134534161));
#52061=DIRECTION('',(0.,0.333233134534162,-0.94284446121751));
#52062=DIRECTION('center_axis',(0.,-0.333233134534162,0.94284446121751));
#52063=DIRECTION('ref_axis',(0.,-0.94284446121751,-0.333233134534162));
#52064=DIRECTION('center_axis',(0.,0.333233134534162,-0.94284446121751));
#52065=DIRECTION('ref_axis',(0.,0.94284446121751,0.333233134534162));
#52066=DIRECTION('',(0.,-0.333233134534162,0.94284446121751));
#52067=DIRECTION('center_axis',(0.,-0.333233134534162,0.94284446121751));
#52068=DIRECTION('ref_axis',(0.,-0.94284446121751,-0.333233134534162));
#52069=DIRECTION('',(0.,0.333233134534162,-0.94284446121751));
#52070=DIRECTION('center_axis',(0.,-0.333233134534162,0.94284446121751));
#52071=DIRECTION('ref_axis',(0.,-0.94284446121751,-0.333233134534162));
#52072=DIRECTION('center_axis',(0.,0.333233134534162,-0.94284446121751));
#52073=DIRECTION('ref_axis',(0.,0.94284446121751,0.333233134534162));
#52074=DIRECTION('',(0.,-0.333233134534162,0.94284446121751));
#52075=DIRECTION('center_axis',(0.,-0.333233134534162,0.94284446121751));
#52076=DIRECTION('ref_axis',(0.,-0.94284446121751,-0.333233134534162));
#52077=DIRECTION('',(0.,0.333233134534162,-0.94284446121751));
#52078=DIRECTION('center_axis',(0.,-0.333233134534162,0.94284446121751));
#52079=DIRECTION('ref_axis',(0.,-0.94284446121751,-0.333233134534162));
#52080=DIRECTION('center_axis',(0.,0.333233134534162,-0.94284446121751));
#52081=DIRECTION('ref_axis',(0.,0.94284446121751,0.333233134534162));
#52082=DIRECTION('',(0.,-0.333233134534162,0.94284446121751));
#52083=DIRECTION('center_axis',(0.,-0.333233134534162,0.94284446121751));
#52084=DIRECTION('ref_axis',(0.,-0.94284446121751,-0.333233134534162));
#52085=DIRECTION('center_axis',(0.,0.333233134534159,-0.942844461217511));
#52086=DIRECTION('ref_axis',(0.,-0.942844461217511,-0.333233134534159));
#52087=DIRECTION('',(0.,0.333233134534162,-0.94284446121751));
#52088=DIRECTION('center_axis',(0.,-0.333233134534162,0.94284446121751));
#52089=DIRECTION('ref_axis',(0.,-0.94284446121751,-0.333233134534162));
#52090=DIRECTION('center_axis',(0.,0.333233134534162,-0.94284446121751));
#52091=DIRECTION('ref_axis',(0.,0.94284446121751,0.333233134534162));
#52092=DIRECTION('',(0.,-0.333233134534162,0.94284446121751));
#52093=DIRECTION('center_axis',(0.,0.333233134534159,-0.942844461217511));
#52094=DIRECTION('ref_axis',(0.,-0.942844461217511,-0.333233134534159));
#52095=DIRECTION('center_axis',(0.,-0.333233134534162,0.94284446121751));
#52096=DIRECTION('ref_axis',(0.,-0.94284446121751,-0.333233134534162));
#52097=DIRECTION('center_axis',(0.,0.333233134534159,-0.942844461217511));
#52098=DIRECTION('ref_axis',(0.,-0.942844461217511,-0.333233134534159));
#52099=DIRECTION('',(0.,0.333233134534162,-0.94284446121751));
#52100=DIRECTION('center_axis',(0.,-0.333233134534162,0.94284446121751));
#52101=DIRECTION('ref_axis',(0.,-0.94284446121751,-0.333233134534162));
#52102=DIRECTION('center_axis',(0.,0.333233134534162,-0.94284446121751));
#52103=DIRECTION('ref_axis',(0.,0.94284446121751,0.333233134534162));
#52104=DIRECTION('',(0.,-0.333233134534162,0.94284446121751));
#52105=DIRECTION('center_axis',(0.,0.333233134534159,-0.942844461217511));
#52106=DIRECTION('ref_axis',(0.,-0.942844461217511,-0.333233134534159));
#52107=DIRECTION('center_axis',(0.,-0.333233134534162,0.94284446121751));
#52108=DIRECTION('ref_axis',(0.,-0.94284446121751,-0.333233134534162));
#52109=DIRECTION('',(0.,0.333233134534162,-0.94284446121751));
#52110=DIRECTION('center_axis',(0.,-0.333233134534162,0.94284446121751));
#52111=DIRECTION('ref_axis',(0.,-0.94284446121751,-0.333233134534162));
#52112=DIRECTION('center_axis',(0.,0.333233134534162,-0.94284446121751));
#52113=DIRECTION('ref_axis',(0.,0.94284446121751,0.333233134534162));
#52114=DIRECTION('',(0.,-0.333233134534162,0.94284446121751));
#52115=DIRECTION('center_axis',(0.,-0.333233134534162,0.94284446121751));
#52116=DIRECTION('ref_axis',(0.,-0.94284446121751,-0.333233134534162));
#52117=DIRECTION('',(0.,0.333233134534162,-0.94284446121751));
#52118=DIRECTION('center_axis',(0.,-0.333233134534162,0.94284446121751));
#52119=DIRECTION('ref_axis',(0.,-0.94284446121751,-0.333233134534162));
#52120=DIRECTION('center_axis',(0.,0.333233134534162,-0.94284446121751));
#52121=DIRECTION('ref_axis',(0.,0.94284446121751,0.333233134534162));
#52122=DIRECTION('',(0.,-0.333233134534162,0.94284446121751));
#52123=DIRECTION('center_axis',(0.,-0.333233134534162,0.94284446121751));
#52124=DIRECTION('ref_axis',(0.,-0.94284446121751,-0.333233134534162));
#52125=DIRECTION('center_axis',(0.,0.333233134534159,-0.942844461217511));
#52126=DIRECTION('ref_axis',(0.,-0.942844461217511,-0.333233134534159));
#52127=DIRECTION('',(0.,0.333233134534162,-0.94284446121751));
#52128=DIRECTION('center_axis',(0.,-0.333233134534162,0.94284446121751));
#52129=DIRECTION('ref_axis',(0.,-0.94284446121751,-0.333233134534162));
#52130=DIRECTION('center_axis',(0.,0.333233134534162,-0.94284446121751));
#52131=DIRECTION('ref_axis',(0.,0.94284446121751,0.333233134534162));
#52132=DIRECTION('',(0.,-0.333233134534162,0.94284446121751));
#52133=DIRECTION('center_axis',(0.,0.333233134534159,-0.942844461217511));
#52134=DIRECTION('ref_axis',(0.,-0.942844461217511,-0.333233134534159));
#52135=DIRECTION('center_axis',(0.,-0.333233134534162,0.94284446121751));
#52136=DIRECTION('ref_axis',(0.,-0.94284446121751,-0.333233134534162));
#52137=DIRECTION('center_axis',(0.,0.333233134534159,-0.942844461217511));
#52138=DIRECTION('ref_axis',(0.,-0.942844461217511,-0.333233134534159));
#52139=DIRECTION('',(0.,0.333233134534162,-0.94284446121751));
#52140=DIRECTION('center_axis',(0.,-0.333233134534162,0.94284446121751));
#52141=DIRECTION('ref_axis',(0.,-0.94284446121751,-0.333233134534162));
#52142=DIRECTION('center_axis',(0.,0.333233134534162,-0.94284446121751));
#52143=DIRECTION('ref_axis',(0.,0.94284446121751,0.333233134534162));
#52144=DIRECTION('',(0.,-0.333233134534162,0.94284446121751));
#52145=DIRECTION('center_axis',(0.,0.333233134534159,-0.942844461217511));
#52146=DIRECTION('ref_axis',(0.,-0.942844461217511,-0.333233134534159));
#52147=DIRECTION('center_axis',(0.,-0.333233134534162,0.94284446121751));
#52148=DIRECTION('ref_axis',(0.,-0.94284446121751,-0.333233134534162));
#52149=DIRECTION('',(0.,0.333233134534162,-0.94284446121751));
#52150=DIRECTION('center_axis',(0.,-0.333233134534162,0.94284446121751));
#52151=DIRECTION('ref_axis',(0.,-0.94284446121751,-0.333233134534162));
#52152=DIRECTION('center_axis',(0.,0.333233134534162,-0.94284446121751));
#52153=DIRECTION('ref_axis',(0.,0.94284446121751,0.333233134534162));
#52154=DIRECTION('',(0.,-0.333233134534162,0.94284446121751));
#52155=DIRECTION('center_axis',(0.,-0.333233134534162,0.94284446121751));
#52156=DIRECTION('ref_axis',(0.,-0.94284446121751,-0.333233134534162));
#52157=DIRECTION('',(0.,0.333233134534162,-0.94284446121751));
#52158=DIRECTION('center_axis',(0.,-0.333233134534162,0.94284446121751));
#52159=DIRECTION('ref_axis',(0.,-0.94284446121751,-0.333233134534162));
#52160=DIRECTION('center_axis',(0.,0.333233134534162,-0.94284446121751));
#52161=DIRECTION('ref_axis',(0.,0.94284446121751,0.333233134534162));
#52162=DIRECTION('',(0.,-0.333233134534162,0.94284446121751));
#52163=DIRECTION('center_axis',(0.,-0.333233134534162,0.94284446121751));
#52164=DIRECTION('ref_axis',(0.,-0.94284446121751,-0.333233134534162));
#52165=DIRECTION('center_axis',(0.,0.333233134534159,-0.942844461217511));
#52166=DIRECTION('ref_axis',(0.,-0.942844461217511,-0.333233134534159));
#52167=DIRECTION('',(0.,0.333233134534162,-0.94284446121751));
#52168=DIRECTION('center_axis',(0.,-0.333233134534162,0.94284446121751));
#52169=DIRECTION('ref_axis',(0.,-0.94284446121751,-0.333233134534162));
#52170=DIRECTION('center_axis',(0.,0.333233134534162,-0.94284446121751));
#52171=DIRECTION('ref_axis',(0.,0.94284446121751,0.333233134534162));
#52172=DIRECTION('',(0.,-0.333233134534162,0.94284446121751));
#52173=DIRECTION('center_axis',(0.,0.333233134534159,-0.942844461217511));
#52174=DIRECTION('ref_axis',(0.,-0.942844461217511,-0.333233134534159));
#52175=DIRECTION('center_axis',(0.,-0.333233134534162,0.94284446121751));
#52176=DIRECTION('ref_axis',(0.,-0.94284446121751,-0.333233134534162));
#52177=DIRECTION('',(0.,0.333233134534162,-0.94284446121751));
#52178=DIRECTION('center_axis',(0.,-0.333233134534162,0.94284446121751));
#52179=DIRECTION('ref_axis',(0.,-0.94284446121751,-0.333233134534162));
#52180=DIRECTION('center_axis',(0.,0.333233134534162,-0.94284446121751));
#52181=DIRECTION('ref_axis',(0.,0.94284446121751,0.333233134534162));
#52182=DIRECTION('',(0.,-0.333233134534162,0.94284446121751));
#52183=DIRECTION('center_axis',(0.,-0.333233134534162,0.94284446121751));
#52184=DIRECTION('ref_axis',(0.,-0.94284446121751,-0.333233134534162));
#52185=DIRECTION('',(0.,0.333233134534162,-0.94284446121751));
#52186=DIRECTION('center_axis',(0.,-0.333233134534162,0.94284446121751));
#52187=DIRECTION('ref_axis',(0.,-0.94284446121751,-0.333233134534162));
#52188=DIRECTION('center_axis',(0.,0.333233134534162,-0.94284446121751));
#52189=DIRECTION('ref_axis',(0.,0.94284446121751,0.333233134534162));
#52190=DIRECTION('',(0.,-0.333233134534162,0.94284446121751));
#52191=DIRECTION('center_axis',(0.,-0.333233134534162,0.94284446121751));
#52192=DIRECTION('ref_axis',(0.,-0.94284446121751,-0.333233134534162));
#52193=DIRECTION('center_axis',(0.,0.333233134534159,-0.942844461217511));
#52194=DIRECTION('ref_axis',(0.,-0.942844461217511,-0.333233134534159));
#52195=DIRECTION('',(0.,0.333233134534162,-0.94284446121751));
#52196=DIRECTION('center_axis',(0.,-0.333233134534162,0.94284446121751));
#52197=DIRECTION('ref_axis',(0.,-0.94284446121751,-0.333233134534162));
#52198=DIRECTION('center_axis',(0.,0.333233134534162,-0.94284446121751));
#52199=DIRECTION('ref_axis',(0.,0.94284446121751,0.333233134534162));
#52200=DIRECTION('',(0.,-0.333233134534162,0.94284446121751));
#52201=DIRECTION('center_axis',(0.,0.333233134534159,-0.942844461217511));
#52202=DIRECTION('ref_axis',(0.,-0.942844461217511,-0.333233134534159));
#52203=DIRECTION('center_axis',(0.,-0.333233134534162,0.94284446121751));
#52204=DIRECTION('ref_axis',(0.,-0.94284446121751,-0.333233134534162));
#52205=DIRECTION('',(0.,0.333233134534162,-0.94284446121751));
#52206=DIRECTION('center_axis',(0.,-0.333233134534162,0.94284446121751));
#52207=DIRECTION('ref_axis',(0.,-0.94284446121751,-0.333233134534162));
#52208=DIRECTION('center_axis',(0.,0.333233134534162,-0.94284446121751));
#52209=DIRECTION('ref_axis',(0.,0.94284446121751,0.333233134534162));
#52210=DIRECTION('',(0.,-0.333233134534162,0.94284446121751));
#52211=DIRECTION('center_axis',(0.,-0.333233134534162,0.94284446121751));
#52212=DIRECTION('ref_axis',(0.,-0.94284446121751,-0.333233134534161));
#52213=DIRECTION('',(0.,0.333233134534162,-0.94284446121751));
#52214=DIRECTION('center_axis',(0.,-0.333233134534162,0.94284446121751));
#52215=DIRECTION('ref_axis',(0.,-0.94284446121751,-0.333233134534162));
#52216=DIRECTION('center_axis',(0.,0.333233134534162,-0.94284446121751));
#52217=DIRECTION('ref_axis',(0.,0.94284446121751,0.333233134534162));
#52218=DIRECTION('',(0.,-0.333233134534162,0.94284446121751));
#52219=DIRECTION('center_axis',(0.,-0.333233134534162,0.94284446121751));
#52220=DIRECTION('ref_axis',(0.,-0.94284446121751,-0.333233134534162));
#52221=DIRECTION('',(0.,0.333233134534162,-0.94284446121751));
#52222=DIRECTION('center_axis',(0.,-0.333233134534162,0.94284446121751));
#52223=DIRECTION('ref_axis',(0.,-0.94284446121751,-0.333233134534162));
#52224=DIRECTION('center_axis',(0.,0.333233134534162,-0.94284446121751));
#52225=DIRECTION('ref_axis',(0.,0.94284446121751,0.333233134534162));
#52226=DIRECTION('',(0.,-0.333233134534162,0.94284446121751));
#52227=DIRECTION('center_axis',(0.,-0.333233134534162,0.94284446121751));
#52228=DIRECTION('ref_axis',(0.,-0.94284446121751,-0.333233134534162));
#52229=DIRECTION('',(0.,0.333233134534162,-0.94284446121751));
#52230=DIRECTION('center_axis',(0.,-0.333233134534162,0.94284446121751));
#52231=DIRECTION('ref_axis',(0.,-0.94284446121751,-0.333233134534162));
#52232=DIRECTION('center_axis',(0.,0.333233134534162,-0.94284446121751));
#52233=DIRECTION('ref_axis',(0.,0.94284446121751,0.333233134534162));
#52234=DIRECTION('',(0.,-0.333233134534162,0.94284446121751));
#52235=DIRECTION('center_axis',(0.,-0.333233134534162,0.94284446121751));
#52236=DIRECTION('ref_axis',(0.,-0.94284446121751,-0.333233134534162));
#52237=DIRECTION('',(0.,0.333233134534162,-0.94284446121751));
#52238=DIRECTION('center_axis',(0.,-0.333233134534162,0.94284446121751));
#52239=DIRECTION('ref_axis',(0.,-0.94284446121751,-0.333233134534162));
#52240=DIRECTION('center_axis',(0.,0.333233134534162,-0.94284446121751));
#52241=DIRECTION('ref_axis',(0.,0.94284446121751,0.333233134534162));
#52242=DIRECTION('',(0.,-0.333233134534162,0.94284446121751));
#52243=DIRECTION('center_axis',(0.,-0.333233134534162,0.94284446121751));
#52244=DIRECTION('ref_axis',(0.,-0.94284446121751,-0.333233134534161));
#52245=DIRECTION('',(0.,0.333233134534162,-0.94284446121751));
#52246=DIRECTION('center_axis',(0.,-0.333233134534162,0.94284446121751));
#52247=DIRECTION('ref_axis',(0.,-0.94284446121751,-0.333233134534162));
#52248=DIRECTION('center_axis',(0.,0.333233134534162,-0.94284446121751));
#52249=DIRECTION('ref_axis',(0.,0.94284446121751,0.333233134534162));
#52250=DIRECTION('',(0.,-0.333233134534162,0.94284446121751));
#52251=DIRECTION('center_axis',(0.,-0.333233134534162,0.94284446121751));
#52252=DIRECTION('ref_axis',(0.,-0.94284446121751,-0.333233134534162));
#52253=DIRECTION('',(0.,0.333233134534162,-0.94284446121751));
#52254=DIRECTION('center_axis',(0.,-0.333233134534162,0.94284446121751));
#52255=DIRECTION('ref_axis',(0.,-0.94284446121751,-0.333233134534162));
#52256=DIRECTION('center_axis',(0.,0.333233134534162,-0.94284446121751));
#52257=DIRECTION('ref_axis',(0.,0.94284446121751,0.333233134534162));
#52258=DIRECTION('',(0.,-0.333233134534162,0.94284446121751));
#52259=DIRECTION('center_axis',(0.,-0.333233134534162,0.94284446121751));
#52260=DIRECTION('ref_axis',(0.,-0.94284446121751,-0.333233134534162));
#52261=DIRECTION('',(0.,0.333233134534162,-0.94284446121751));
#52262=DIRECTION('center_axis',(0.,-0.333233134534162,0.94284446121751));
#52263=DIRECTION('ref_axis',(0.,-0.94284446121751,-0.333233134534162));
#52264=DIRECTION('center_axis',(0.,0.333233134534162,-0.94284446121751));
#52265=DIRECTION('ref_axis',(0.,0.94284446121751,0.333233134534162));
#52266=DIRECTION('',(0.,-0.333233134534162,0.94284446121751));
#52267=DIRECTION('center_axis',(0.,-0.333233134534162,0.94284446121751));
#52268=DIRECTION('ref_axis',(0.,-0.94284446121751,-0.333233134534162));
#52269=DIRECTION('',(0.,0.333233134534162,-0.94284446121751));
#52270=DIRECTION('center_axis',(0.,-0.333233134534162,0.94284446121751));
#52271=DIRECTION('ref_axis',(0.,-0.94284446121751,-0.333233134534162));
#52272=DIRECTION('center_axis',(0.,0.333233134534162,-0.94284446121751));
#52273=DIRECTION('ref_axis',(0.,0.94284446121751,0.333233134534162));
#52274=DIRECTION('',(0.,-0.333233134534162,0.94284446121751));
#52275=DIRECTION('center_axis',(0.,-0.333233134534162,0.94284446121751));
#52276=DIRECTION('ref_axis',(0.,-0.94284446121751,-0.333233134534161));
#52277=DIRECTION('',(0.,0.333233134534162,-0.94284446121751));
#52278=DIRECTION('center_axis',(0.,-0.333233134534162,0.94284446121751));
#52279=DIRECTION('ref_axis',(0.,-0.94284446121751,-0.333233134534162));
#52280=DIRECTION('center_axis',(0.,0.333233134534162,-0.94284446121751));
#52281=DIRECTION('ref_axis',(0.,0.94284446121751,0.333233134534162));
#52282=DIRECTION('',(0.,-0.333233134534162,0.94284446121751));
#52283=DIRECTION('center_axis',(0.,-0.333233134534162,0.94284446121751));
#52284=DIRECTION('ref_axis',(0.,-0.94284446121751,-0.333233134534162));
#52285=DIRECTION('',(0.,0.333233134534162,-0.94284446121751));
#52286=DIRECTION('center_axis',(0.,-0.333233134534162,0.94284446121751));
#52287=DIRECTION('ref_axis',(0.,-0.94284446121751,-0.333233134534162));
#52288=DIRECTION('center_axis',(0.,0.333233134534162,-0.94284446121751));
#52289=DIRECTION('ref_axis',(0.,0.94284446121751,0.333233134534162));
#52290=DIRECTION('',(0.,-0.333233134534162,0.94284446121751));
#52291=DIRECTION('center_axis',(0.,-0.333233134534162,0.94284446121751));
#52292=DIRECTION('ref_axis',(0.,-0.94284446121751,-0.333233134534162));
#52293=DIRECTION('',(0.,0.333233134534162,-0.94284446121751));
#52294=DIRECTION('center_axis',(0.,-0.333233134534162,0.94284446121751));
#52295=DIRECTION('ref_axis',(0.,-0.94284446121751,-0.333233134534162));
#52296=DIRECTION('center_axis',(0.,0.333233134534162,-0.94284446121751));
#52297=DIRECTION('ref_axis',(0.,0.94284446121751,0.333233134534162));
#52298=DIRECTION('',(0.,-0.333233134534162,0.94284446121751));
#52299=DIRECTION('center_axis',(0.,-0.333233134534162,0.94284446121751));
#52300=DIRECTION('ref_axis',(0.,-0.94284446121751,-0.333233134534161));
#52301=DIRECTION('',(0.,0.333233134534162,-0.94284446121751));
#52302=DIRECTION('center_axis',(0.,-0.333233134534162,0.94284446121751));
#52303=DIRECTION('ref_axis',(0.,-0.94284446121751,-0.333233134534162));
#52304=DIRECTION('center_axis',(0.,0.333233134534162,-0.94284446121751));
#52305=DIRECTION('ref_axis',(0.,0.94284446121751,0.333233134534162));
#52306=DIRECTION('',(0.,-0.333233134534162,0.94284446121751));
#52307=DIRECTION('center_axis',(0.,-0.333233134534162,0.94284446121751));
#52308=DIRECTION('ref_axis',(0.,-0.94284446121751,-0.333233134534162));
#52309=DIRECTION('',(0.,0.333233134534162,-0.94284446121751));
#52310=DIRECTION('center_axis',(0.,-0.333233134534162,0.94284446121751));
#52311=DIRECTION('ref_axis',(0.,-0.94284446121751,-0.333233134534162));
#52312=DIRECTION('center_axis',(0.,0.333233134534162,-0.94284446121751));
#52313=DIRECTION('ref_axis',(0.,0.94284446121751,0.333233134534162));
#52314=DIRECTION('',(0.,-0.333233134534162,0.94284446121751));
#52315=DIRECTION('center_axis',(0.,-0.333233134534162,0.94284446121751));
#52316=DIRECTION('ref_axis',(0.,-0.94284446121751,-0.333233134534161));
#52317=DIRECTION('center_axis',(0.,0.333233134534159,-0.942844461217511));
#52318=DIRECTION('ref_axis',(0.,-0.942844461217511,-0.333233134534159));
#52319=DIRECTION('',(0.,0.333233134534162,-0.94284446121751));
#52320=DIRECTION('center_axis',(0.,0.333233134534162,-0.94284446121751));
#52321=DIRECTION('ref_axis',(0.,-0.94284446121751,-0.333233134534162));
#52322=DIRECTION('center_axis',(0.,-0.333233134534162,0.94284446121751));
#52323=DIRECTION('ref_axis',(0.,-0.94284446121751,-0.333233134534162));
#52324=DIRECTION('center_axis',(0.,0.333233134534162,-0.94284446121751));
#52325=DIRECTION('ref_axis',(0.,0.94284446121751,0.333233134534162));
#52326=DIRECTION('',(0.,-0.333233134534162,0.94284446121751));
#52327=DIRECTION('center_axis',(0.,0.333233134534159,-0.942844461217511));
#52328=DIRECTION('ref_axis',(0.,-0.942844461217511,-0.333233134534159));
#52329=DIRECTION('center_axis',(0.,-0.333233134534162,0.94284446121751));
#52330=DIRECTION('ref_axis',(0.,-0.94284446121751,-0.333233134534162));
#52331=DIRECTION('center_axis',(0.,0.333233134534159,-0.942844461217511));
#52332=DIRECTION('ref_axis',(0.,-0.942844461217511,-0.333233134534159));
#52333=DIRECTION('',(0.,0.333233134534162,-0.94284446121751));
#52334=DIRECTION('center_axis',(0.,0.333233134534162,-0.94284446121751));
#52335=DIRECTION('ref_axis',(0.,-0.94284446121751,-0.333233134534162));
#52336=DIRECTION('center_axis',(0.,-0.333233134534162,0.94284446121751));
#52337=DIRECTION('ref_axis',(0.,-0.94284446121751,-0.333233134534162));
#52338=DIRECTION('center_axis',(0.,0.333233134534162,-0.94284446121751));
#52339=DIRECTION('ref_axis',(0.,0.94284446121751,0.333233134534162));
#52340=DIRECTION('',(0.,-0.333233134534162,0.94284446121751));
#52341=DIRECTION('center_axis',(0.,0.333233134534159,-0.942844461217511));
#52342=DIRECTION('ref_axis',(0.,-0.942844461217511,-0.333233134534159));
#52343=DIRECTION('center_axis',(0.,-0.333233134534162,0.94284446121751));
#52344=DIRECTION('ref_axis',(0.,-0.94284446121751,-0.333233134534162));
#52345=DIRECTION('center_axis',(0.,0.333233134534159,-0.942844461217511));
#52346=DIRECTION('ref_axis',(0.,-0.942844461217511,-0.333233134534159));
#52347=DIRECTION('',(0.,0.333233134534162,-0.94284446121751));
#52348=DIRECTION('center_axis',(0.,0.333233134534162,-0.94284446121751));
#52349=DIRECTION('ref_axis',(0.,-0.94284446121751,-0.333233134534162));
#52350=DIRECTION('center_axis',(0.,-0.333233134534162,0.94284446121751));
#52351=DIRECTION('ref_axis',(0.,-0.94284446121751,-0.333233134534162));
#52352=DIRECTION('center_axis',(0.,0.333233134534162,-0.94284446121751));
#52353=DIRECTION('ref_axis',(0.,0.94284446121751,0.333233134534162));
#52354=DIRECTION('',(0.,-0.333233134534162,0.94284446121751));
#52355=DIRECTION('center_axis',(0.,0.333233134534159,-0.942844461217511));
#52356=DIRECTION('ref_axis',(0.,-0.942844461217511,-0.333233134534159));
#52357=DIRECTION('center_axis',(0.,-0.333233134534162,0.94284446121751));
#52358=DIRECTION('ref_axis',(0.,-0.94284446121751,-0.333233134534162));
#52359=DIRECTION('center_axis',(0.,0.333233134534159,-0.942844461217511));
#52360=DIRECTION('ref_axis',(0.,-0.942844461217511,-0.333233134534159));
#52361=DIRECTION('',(0.,0.333233134534162,-0.94284446121751));
#52362=DIRECTION('center_axis',(0.,0.333233134534162,-0.94284446121751));
#52363=DIRECTION('ref_axis',(0.,-0.94284446121751,-0.333233134534162));
#52364=DIRECTION('center_axis',(0.,-0.333233134534162,0.94284446121751));
#52365=DIRECTION('ref_axis',(0.,-0.94284446121751,-0.333233134534162));
#52366=DIRECTION('center_axis',(0.,0.333233134534162,-0.94284446121751));
#52367=DIRECTION('ref_axis',(0.,0.94284446121751,0.333233134534162));
#52368=DIRECTION('',(0.,-0.333233134534162,0.94284446121751));
#52369=DIRECTION('center_axis',(0.,0.333233134534159,-0.942844461217511));
#52370=DIRECTION('ref_axis',(0.,-0.942844461217511,-0.333233134534159));
#52371=DIRECTION('center_axis',(0.,-0.333233134534162,0.94284446121751));
#52372=DIRECTION('ref_axis',(0.,-0.94284446121751,-0.333233134534162));
#52373=DIRECTION('center_axis',(0.,0.333233134534159,-0.942844461217511));
#52374=DIRECTION('ref_axis',(0.,-0.942844461217511,-0.333233134534159));
#52375=DIRECTION('',(0.,0.333233134534162,-0.94284446121751));
#52376=DIRECTION('center_axis',(0.,0.333233134534162,-0.94284446121751));
#52377=DIRECTION('ref_axis',(0.,-0.94284446121751,-0.333233134534162));
#52378=DIRECTION('center_axis',(0.,-0.333233134534162,0.94284446121751));
#52379=DIRECTION('ref_axis',(0.,-0.94284446121751,-0.333233134534162));
#52380=DIRECTION('center_axis',(0.,0.333233134534162,-0.94284446121751));
#52381=DIRECTION('ref_axis',(0.,0.94284446121751,0.333233134534162));
#52382=DIRECTION('',(0.,-0.333233134534162,0.94284446121751));
#52383=DIRECTION('center_axis',(0.,0.333233134534159,-0.942844461217511));
#52384=DIRECTION('ref_axis',(0.,-0.942844461217511,-0.333233134534159));
#52385=DIRECTION('center_axis',(0.,-0.333233134534162,0.94284446121751));
#52386=DIRECTION('ref_axis',(0.,-0.94284446121751,-0.333233134534162));
#52387=DIRECTION('center_axis',(0.,0.333233134534159,-0.942844461217511));
#52388=DIRECTION('ref_axis',(0.,-0.942844461217511,-0.333233134534159));
#52389=DIRECTION('',(0.,0.333233134534162,-0.94284446121751));
#52390=DIRECTION('center_axis',(0.,0.333233134534162,-0.94284446121751));
#52391=DIRECTION('ref_axis',(0.,-0.94284446121751,-0.333233134534162));
#52392=DIRECTION('center_axis',(0.,-0.333233134534162,0.94284446121751));
#52393=DIRECTION('ref_axis',(0.,-0.94284446121751,-0.333233134534162));
#52394=DIRECTION('center_axis',(0.,0.333233134534162,-0.94284446121751));
#52395=DIRECTION('ref_axis',(0.,0.94284446121751,0.333233134534162));
#52396=DIRECTION('',(0.,-0.333233134534162,0.94284446121751));
#52397=DIRECTION('center_axis',(0.,0.333233134534159,-0.942844461217511));
#52398=DIRECTION('ref_axis',(0.,-0.942844461217511,-0.333233134534159));
#52399=DIRECTION('center_axis',(0.,-0.333233134534162,0.94284446121751));
#52400=DIRECTION('ref_axis',(0.,-0.94284446121751,-0.333233134534162));
#52401=DIRECTION('center_axis',(0.,0.333233134534159,-0.942844461217511));
#52402=DIRECTION('ref_axis',(0.,-0.942844461217511,-0.333233134534159));
#52403=DIRECTION('',(0.,0.333233134534162,-0.94284446121751));
#52404=DIRECTION('center_axis',(0.,0.333233134534162,-0.94284446121751));
#52405=DIRECTION('ref_axis',(0.,-0.94284446121751,-0.333233134534162));
#52406=DIRECTION('center_axis',(0.,-0.333233134534162,0.94284446121751));
#52407=DIRECTION('ref_axis',(0.,-0.94284446121751,-0.333233134534162));
#52408=DIRECTION('center_axis',(0.,0.333233134534162,-0.94284446121751));
#52409=DIRECTION('ref_axis',(0.,0.94284446121751,0.333233134534162));
#52410=DIRECTION('',(0.,-0.333233134534162,0.94284446121751));
#52411=DIRECTION('center_axis',(0.,0.333233134534159,-0.942844461217511));
#52412=DIRECTION('ref_axis',(0.,-0.942844461217511,-0.333233134534159));
#52413=DIRECTION('center_axis',(0.,-0.333233134534162,0.94284446121751));
#52414=DIRECTION('ref_axis',(0.,-0.94284446121751,-0.333233134534162));
#52415=DIRECTION('center_axis',(0.,0.333233134534159,-0.942844461217511));
#52416=DIRECTION('ref_axis',(0.,-0.942844461217511,-0.333233134534159));
#52417=DIRECTION('',(0.,0.333233134534162,-0.94284446121751));
#52418=DIRECTION('center_axis',(0.,0.333233134534162,-0.94284446121751));
#52419=DIRECTION('ref_axis',(0.,-0.94284446121751,-0.333233134534162));
#52420=DIRECTION('center_axis',(0.,-0.333233134534162,0.94284446121751));
#52421=DIRECTION('ref_axis',(0.,-0.94284446121751,-0.333233134534162));
#52422=DIRECTION('center_axis',(0.,0.333233134534162,-0.94284446121751));
#52423=DIRECTION('ref_axis',(0.,0.94284446121751,0.333233134534162));
#52424=DIRECTION('',(0.,-0.333233134534162,0.94284446121751));
#52425=DIRECTION('center_axis',(0.,0.333233134534159,-0.942844461217511));
#52426=DIRECTION('ref_axis',(0.,-0.942844461217511,-0.333233134534159));
#52427=DIRECTION('center_axis',(0.,-0.333233134534162,0.94284446121751));
#52428=DIRECTION('ref_axis',(0.,-0.94284446121751,-0.333233134534162));
#52429=DIRECTION('center_axis',(0.,0.333233134534159,-0.942844461217511));
#52430=DIRECTION('ref_axis',(0.,-0.942844461217511,-0.333233134534159));
#52431=DIRECTION('',(0.,0.333233134534162,-0.94284446121751));
#52432=DIRECTION('center_axis',(0.,-0.333233134534162,0.94284446121751));
#52433=DIRECTION('ref_axis',(0.,-0.94284446121751,-0.333233134534162));
#52434=DIRECTION('center_axis',(0.,-0.333233134534162,0.94284446121751));
#52435=DIRECTION('ref_axis',(0.,-0.94284446121751,-0.333233134534162));
#52436=DIRECTION('center_axis',(0.,0.333233134534162,-0.94284446121751));
#52437=DIRECTION('ref_axis',(0.,0.94284446121751,0.333233134534162));
#52438=DIRECTION('',(0.,-0.333233134534162,0.94284446121751));
#52439=DIRECTION('center_axis',(0.,0.333233134534159,-0.942844461217511));
#52440=DIRECTION('ref_axis',(0.,-0.942844461217511,-0.333233134534159));
#52441=DIRECTION('center_axis',(0.,-0.333233134534162,0.94284446121751));
#52442=DIRECTION('ref_axis',(0.,-0.94284446121751,-0.333233134534161));
#52443=DIRECTION('center_axis',(0.,0.333233134534159,-0.942844461217511));
#52444=DIRECTION('ref_axis',(0.,-0.942844461217511,-0.333233134534159));
#52445=DIRECTION('',(0.,0.333233134534162,-0.94284446121751));
#52446=DIRECTION('center_axis',(0.,0.333233134534162,-0.94284446121751));
#52447=DIRECTION('ref_axis',(0.,-0.94284446121751,-0.333233134534162));
#52448=DIRECTION('center_axis',(0.,-0.333233134534162,0.94284446121751));
#52449=DIRECTION('ref_axis',(0.,-0.94284446121751,-0.333233134534162));
#52450=DIRECTION('center_axis',(0.,0.333233134534162,-0.94284446121751));
#52451=DIRECTION('ref_axis',(0.,0.94284446121751,0.333233134534162));
#52452=DIRECTION('',(0.,-0.333233134534162,0.94284446121751));
#52453=DIRECTION('center_axis',(0.,0.333233134534159,-0.942844461217511));
#52454=DIRECTION('ref_axis',(0.,-0.942844461217511,-0.333233134534159));
#52455=DIRECTION('center_axis',(0.,-0.333233134534162,0.94284446121751));
#52456=DIRECTION('ref_axis',(0.,-0.94284446121751,-0.333233134534162));
#52457=DIRECTION('center_axis',(0.,0.333233134534159,-0.942844461217511));
#52458=DIRECTION('ref_axis',(0.,-0.942844461217511,-0.333233134534159));
#52459=DIRECTION('',(0.,0.333233134534162,-0.94284446121751));
#52460=DIRECTION('center_axis',(0.,0.333233134534162,-0.94284446121751));
#52461=DIRECTION('ref_axis',(0.,-0.94284446121751,-0.333233134534162));
#52462=DIRECTION('center_axis',(0.,-0.333233134534162,0.94284446121751));
#52463=DIRECTION('ref_axis',(0.,-0.94284446121751,-0.333233134534162));
#52464=DIRECTION('center_axis',(0.,0.333233134534162,-0.94284446121751));
#52465=DIRECTION('ref_axis',(0.,0.94284446121751,0.333233134534162));
#52466=DIRECTION('',(0.,-0.333233134534162,0.94284446121751));
#52467=DIRECTION('center_axis',(0.,0.333233134534159,-0.942844461217511));
#52468=DIRECTION('ref_axis',(0.,-0.942844461217511,-0.333233134534159));
#52469=DIRECTION('center_axis',(0.,-0.333233134534162,0.94284446121751));
#52470=DIRECTION('ref_axis',(0.,-0.94284446121751,-0.333233134534162));
#52471=DIRECTION('center_axis',(0.,0.333233134534159,-0.942844461217511));
#52472=DIRECTION('ref_axis',(0.,-0.942844461217511,-0.333233134534159));
#52473=DIRECTION('',(0.,0.333233134534162,-0.94284446121751));
#52474=DIRECTION('center_axis',(0.,0.333233134534162,-0.94284446121751));
#52475=DIRECTION('ref_axis',(0.,-0.94284446121751,-0.333233134534162));
#52476=DIRECTION('center_axis',(0.,-0.333233134534162,0.94284446121751));
#52477=DIRECTION('ref_axis',(0.,-0.94284446121751,-0.333233134534162));
#52478=DIRECTION('center_axis',(0.,0.333233134534162,-0.94284446121751));
#52479=DIRECTION('ref_axis',(0.,0.94284446121751,0.333233134534162));
#52480=DIRECTION('',(0.,-0.333233134534162,0.94284446121751));
#52481=DIRECTION('center_axis',(0.,0.333233134534159,-0.942844461217511));
#52482=DIRECTION('ref_axis',(0.,-0.942844461217511,-0.333233134534159));
#52483=DIRECTION('center_axis',(0.,-0.333233134534162,0.94284446121751));
#52484=DIRECTION('ref_axis',(0.,-0.94284446121751,-0.333233134534162));
#52485=DIRECTION('center_axis',(0.,0.333233134534159,-0.942844461217511));
#52486=DIRECTION('ref_axis',(0.,-0.942844461217511,-0.333233134534159));
#52487=DIRECTION('',(0.,0.333233134534162,-0.94284446121751));
#52488=DIRECTION('center_axis',(0.,0.333233134534162,-0.94284446121751));
#52489=DIRECTION('ref_axis',(0.,-0.94284446121751,-0.333233134534162));
#52490=DIRECTION('center_axis',(0.,-0.333233134534162,0.94284446121751));
#52491=DIRECTION('ref_axis',(0.,-0.94284446121751,-0.333233134534162));
#52492=DIRECTION('center_axis',(0.,0.333233134534162,-0.94284446121751));
#52493=DIRECTION('ref_axis',(0.,0.94284446121751,0.333233134534162));
#52494=DIRECTION('',(0.,-0.333233134534162,0.94284446121751));
#52495=DIRECTION('center_axis',(0.,0.333233134534159,-0.942844461217511));
#52496=DIRECTION('ref_axis',(0.,-0.942844461217511,-0.333233134534159));
#52497=DIRECTION('center_axis',(0.,-0.333233134534162,0.94284446121751));
#52498=DIRECTION('ref_axis',(0.,-0.94284446121751,-0.333233134534162));
#52499=DIRECTION('center_axis',(0.,0.333233134534159,-0.942844461217511));
#52500=DIRECTION('ref_axis',(0.,-0.942844461217511,-0.333233134534159));
#52501=DIRECTION('',(0.,0.333233134534162,-0.94284446121751));
#52502=DIRECTION('center_axis',(0.,0.333233134534162,-0.94284446121751));
#52503=DIRECTION('ref_axis',(0.,-0.94284446121751,-0.333233134534162));
#52504=DIRECTION('center_axis',(0.,-0.333233134534162,0.94284446121751));
#52505=DIRECTION('ref_axis',(0.,-0.94284446121751,-0.333233134534162));
#52506=DIRECTION('center_axis',(0.,0.333233134534162,-0.94284446121751));
#52507=DIRECTION('ref_axis',(0.,0.94284446121751,0.333233134534162));
#52508=DIRECTION('',(0.,-0.333233134534162,0.94284446121751));
#52509=DIRECTION('center_axis',(0.,0.333233134534159,-0.942844461217511));
#52510=DIRECTION('ref_axis',(0.,-0.942844461217511,-0.333233134534159));
#52511=DIRECTION('center_axis',(0.,-0.333233134534162,0.94284446121751));
#52512=DIRECTION('ref_axis',(0.,-0.94284446121751,-0.333233134534162));
#52513=DIRECTION('center_axis',(0.,0.333233134534159,-0.942844461217511));
#52514=DIRECTION('ref_axis',(0.,-0.942844461217511,-0.333233134534159));
#52515=DIRECTION('',(0.,0.333233134534162,-0.94284446121751));
#52516=DIRECTION('center_axis',(0.,0.333233134534162,-0.94284446121751));
#52517=DIRECTION('ref_axis',(0.,-0.94284446121751,-0.333233134534162));
#52518=DIRECTION('center_axis',(0.,-0.333233134534162,0.94284446121751));
#52519=DIRECTION('ref_axis',(0.,-0.94284446121751,-0.333233134534162));
#52520=DIRECTION('center_axis',(0.,0.333233134534162,-0.94284446121751));
#52521=DIRECTION('ref_axis',(0.,0.94284446121751,0.333233134534162));
#52522=DIRECTION('',(0.,-0.333233134534162,0.94284446121751));
#52523=DIRECTION('center_axis',(0.,0.333233134534159,-0.942844461217511));
#52524=DIRECTION('ref_axis',(0.,-0.942844461217511,-0.333233134534159));
#52525=DIRECTION('center_axis',(0.,-0.333233134534162,0.94284446121751));
#52526=DIRECTION('ref_axis',(0.,-0.94284446121751,-0.333233134534162));
#52527=DIRECTION('center_axis',(0.,0.333233134534159,-0.942844461217511));
#52528=DIRECTION('ref_axis',(0.,-0.942844461217511,-0.333233134534159));
#52529=DIRECTION('',(0.,0.333233134534162,-0.94284446121751));
#52530=DIRECTION('center_axis',(0.,0.333233134534162,-0.94284446121751));
#52531=DIRECTION('ref_axis',(0.,-0.94284446121751,-0.333233134534162));
#52532=DIRECTION('center_axis',(0.,-0.333233134534162,0.94284446121751));
#52533=DIRECTION('ref_axis',(0.,-0.94284446121751,-0.333233134534162));
#52534=DIRECTION('center_axis',(0.,0.333233134534162,-0.94284446121751));
#52535=DIRECTION('ref_axis',(0.,0.94284446121751,0.333233134534162));
#52536=DIRECTION('',(0.,-0.333233134534162,0.94284446121751));
#52537=DIRECTION('center_axis',(0.,0.333233134534159,-0.942844461217511));
#52538=DIRECTION('ref_axis',(0.,-0.942844461217511,-0.333233134534159));
#52539=DIRECTION('center_axis',(0.,-0.333233134534162,0.94284446121751));
#52540=DIRECTION('ref_axis',(0.,-0.94284446121751,-0.333233134534162));
#52541=DIRECTION('center_axis',(0.,0.333233134534159,-0.942844461217511));
#52542=DIRECTION('ref_axis',(0.,-0.942844461217511,-0.333233134534159));
#52543=DIRECTION('',(0.,0.333233134534162,-0.94284446121751));
#52544=DIRECTION('center_axis',(0.,0.333233134534162,-0.94284446121751));
#52545=DIRECTION('ref_axis',(0.,-0.94284446121751,-0.333233134534162));
#52546=DIRECTION('center_axis',(0.,-0.333233134534162,0.94284446121751));
#52547=DIRECTION('ref_axis',(0.,-0.94284446121751,-0.333233134534162));
#52548=DIRECTION('center_axis',(0.,0.333233134534162,-0.94284446121751));
#52549=DIRECTION('ref_axis',(0.,0.94284446121751,0.333233134534162));
#52550=DIRECTION('',(0.,-0.333233134534162,0.94284446121751));
#52551=DIRECTION('center_axis',(0.,0.333233134534159,-0.942844461217511));
#52552=DIRECTION('ref_axis',(0.,-0.942844461217511,-0.333233134534159));
#52553=DIRECTION('center_axis',(0.,-0.333233134534162,0.94284446121751));
#52554=DIRECTION('ref_axis',(0.,-0.94284446121751,-0.333233134534162));
#52555=DIRECTION('center_axis',(0.,0.333233134534159,-0.942844461217511));
#52556=DIRECTION('ref_axis',(0.,-0.942844461217511,-0.333233134534159));
#52557=DIRECTION('',(0.,0.333233134534162,-0.94284446121751));
#52558=DIRECTION('center_axis',(0.,-0.333233134534162,0.94284446121751));
#52559=DIRECTION('ref_axis',(0.,-0.94284446121751,-0.333233134534162));
#52560=DIRECTION('center_axis',(0.,-0.333233134534162,0.94284446121751));
#52561=DIRECTION('ref_axis',(0.,-0.94284446121751,-0.333233134534162));
#52562=DIRECTION('center_axis',(0.,0.333233134534162,-0.94284446121751));
#52563=DIRECTION('ref_axis',(0.,0.94284446121751,0.333233134534162));
#52564=DIRECTION('',(0.,-0.333233134534162,0.94284446121751));
#52565=DIRECTION('center_axis',(0.,0.333233134534159,-0.942844461217511));
#52566=DIRECTION('ref_axis',(0.,-0.942844461217511,-0.333233134534159));
#52567=DIRECTION('center_axis',(0.,-0.333233134534162,0.94284446121751));
#52568=DIRECTION('ref_axis',(0.,-0.94284446121751,-0.333233134534161));
#52569=DIRECTION('center_axis',(0.,0.333233134534159,-0.942844461217511));
#52570=DIRECTION('ref_axis',(0.,-0.942844461217511,-0.333233134534159));
#52571=DIRECTION('',(0.,0.333233134534162,-0.94284446121751));
#52572=DIRECTION('center_axis',(0.,0.333233134534162,-0.94284446121751));
#52573=DIRECTION('ref_axis',(0.,-0.94284446121751,-0.333233134534162));
#52574=DIRECTION('center_axis',(0.,-0.333233134534162,0.94284446121751));
#52575=DIRECTION('ref_axis',(0.,-0.94284446121751,-0.333233134534162));
#52576=DIRECTION('center_axis',(0.,0.333233134534162,-0.94284446121751));
#52577=DIRECTION('ref_axis',(0.,0.94284446121751,0.333233134534162));
#52578=DIRECTION('',(0.,-0.333233134534162,0.94284446121751));
#52579=DIRECTION('center_axis',(0.,0.333233134534159,-0.942844461217511));
#52580=DIRECTION('ref_axis',(0.,-0.942844461217511,-0.333233134534159));
#52581=DIRECTION('center_axis',(0.,-0.333233134534162,0.94284446121751));
#52582=DIRECTION('ref_axis',(0.,-0.94284446121751,-0.333233134534162));
#52583=DIRECTION('center_axis',(0.,0.333233134534159,-0.942844461217511));
#52584=DIRECTION('ref_axis',(0.,-0.942844461217511,-0.333233134534159));
#52585=DIRECTION('',(0.,0.333233134534162,-0.94284446121751));
#52586=DIRECTION('center_axis',(0.,0.333233134534162,-0.94284446121751));
#52587=DIRECTION('ref_axis',(0.,-0.94284446121751,-0.333233134534162));
#52588=DIRECTION('center_axis',(0.,-0.333233134534162,0.94284446121751));
#52589=DIRECTION('ref_axis',(0.,-0.94284446121751,-0.333233134534162));
#52590=DIRECTION('center_axis',(0.,0.333233134534162,-0.94284446121751));
#52591=DIRECTION('ref_axis',(0.,0.94284446121751,0.333233134534162));
#52592=DIRECTION('',(0.,-0.333233134534162,0.94284446121751));
#52593=DIRECTION('center_axis',(0.,0.333233134534159,-0.942844461217511));
#52594=DIRECTION('ref_axis',(0.,-0.942844461217511,-0.333233134534159));
#52595=DIRECTION('center_axis',(0.,-0.333233134534162,0.94284446121751));
#52596=DIRECTION('ref_axis',(0.,-0.94284446121751,-0.333233134534162));
#52597=DIRECTION('center_axis',(0.,0.333233134534159,-0.942844461217511));
#52598=DIRECTION('ref_axis',(0.,-0.942844461217511,-0.333233134534159));
#52599=DIRECTION('',(0.,0.333233134534162,-0.94284446121751));
#52600=DIRECTION('center_axis',(0.,0.333233134534162,-0.94284446121751));
#52601=DIRECTION('ref_axis',(0.,-0.94284446121751,-0.333233134534162));
#52602=DIRECTION('center_axis',(0.,-0.333233134534162,0.94284446121751));
#52603=DIRECTION('ref_axis',(0.,-0.94284446121751,-0.333233134534162));
#52604=DIRECTION('center_axis',(0.,0.333233134534162,-0.94284446121751));
#52605=DIRECTION('ref_axis',(0.,0.94284446121751,0.333233134534162));
#52606=DIRECTION('',(0.,-0.333233134534162,0.94284446121751));
#52607=DIRECTION('center_axis',(0.,0.333233134534159,-0.942844461217511));
#52608=DIRECTION('ref_axis',(0.,-0.942844461217511,-0.333233134534159));
#52609=DIRECTION('center_axis',(0.,-0.333233134534162,0.94284446121751));
#52610=DIRECTION('ref_axis',(0.,-0.94284446121751,-0.333233134534162));
#52611=DIRECTION('center_axis',(0.,0.333233134534159,-0.942844461217511));
#52612=DIRECTION('ref_axis',(0.,-0.942844461217511,-0.333233134534159));
#52613=DIRECTION('',(0.,0.333233134534162,-0.94284446121751));
#52614=DIRECTION('center_axis',(0.,0.333233134534162,-0.94284446121751));
#52615=DIRECTION('ref_axis',(0.,-0.94284446121751,-0.333233134534162));
#52616=DIRECTION('center_axis',(0.,-0.333233134534162,0.94284446121751));
#52617=DIRECTION('ref_axis',(0.,-0.94284446121751,-0.333233134534162));
#52618=DIRECTION('center_axis',(0.,0.333233134534162,-0.94284446121751));
#52619=DIRECTION('ref_axis',(0.,0.94284446121751,0.333233134534162));
#52620=DIRECTION('',(0.,-0.333233134534162,0.94284446121751));
#52621=DIRECTION('center_axis',(0.,0.333233134534159,-0.942844461217511));
#52622=DIRECTION('ref_axis',(0.,-0.942844461217511,-0.333233134534159));
#52623=DIRECTION('center_axis',(0.,-0.333233134534162,0.94284446121751));
#52624=DIRECTION('ref_axis',(0.,-0.94284446121751,-0.333233134534162));
#52625=DIRECTION('center_axis',(0.,0.333233134534159,-0.942844461217511));
#52626=DIRECTION('ref_axis',(0.,-0.942844461217511,-0.333233134534159));
#52627=DIRECTION('',(0.,0.333233134534162,-0.94284446121751));
#52628=DIRECTION('center_axis',(0.,0.333233134534162,-0.94284446121751));
#52629=DIRECTION('ref_axis',(0.,-0.94284446121751,-0.333233134534162));
#52630=DIRECTION('center_axis',(0.,-0.333233134534162,0.94284446121751));
#52631=DIRECTION('ref_axis',(0.,-0.94284446121751,-0.333233134534162));
#52632=DIRECTION('center_axis',(0.,0.333233134534162,-0.94284446121751));
#52633=DIRECTION('ref_axis',(0.,0.94284446121751,0.333233134534162));
#52634=DIRECTION('',(0.,-0.333233134534162,0.94284446121751));
#52635=DIRECTION('center_axis',(0.,0.333233134534159,-0.942844461217511));
#52636=DIRECTION('ref_axis',(0.,-0.942844461217511,-0.333233134534159));
#52637=DIRECTION('center_axis',(0.,-0.333233134534162,0.94284446121751));
#52638=DIRECTION('ref_axis',(0.,-0.94284446121751,-0.333233134534162));
#52639=DIRECTION('center_axis',(0.,0.333233134534159,-0.942844461217511));
#52640=DIRECTION('ref_axis',(0.,-0.942844461217511,-0.333233134534159));
#52641=DIRECTION('',(0.,0.333233134534162,-0.94284446121751));
#52642=DIRECTION('center_axis',(0.,0.333233134534162,-0.94284446121751));
#52643=DIRECTION('ref_axis',(0.,-0.94284446121751,-0.333233134534162));
#52644=DIRECTION('center_axis',(0.,-0.333233134534162,0.94284446121751));
#52645=DIRECTION('ref_axis',(0.,-0.94284446121751,-0.333233134534162));
#52646=DIRECTION('center_axis',(0.,0.333233134534162,-0.94284446121751));
#52647=DIRECTION('ref_axis',(0.,0.94284446121751,0.333233134534162));
#52648=DIRECTION('',(0.,-0.333233134534162,0.94284446121751));
#52649=DIRECTION('center_axis',(0.,0.333233134534159,-0.942844461217511));
#52650=DIRECTION('ref_axis',(0.,-0.942844461217511,-0.333233134534159));
#52651=DIRECTION('center_axis',(0.,-0.333233134534162,0.94284446121751));
#52652=DIRECTION('ref_axis',(0.,-0.94284446121751,-0.333233134534162));
#52653=DIRECTION('center_axis',(0.,0.333233134534159,-0.942844461217511));
#52654=DIRECTION('ref_axis',(0.,-0.942844461217511,-0.333233134534159));
#52655=DIRECTION('',(0.,0.333233134534162,-0.94284446121751));
#52656=DIRECTION('center_axis',(0.,0.333233134534162,-0.94284446121751));
#52657=DIRECTION('ref_axis',(0.,-0.94284446121751,-0.333233134534162));
#52658=DIRECTION('center_axis',(0.,-0.333233134534162,0.94284446121751));
#52659=DIRECTION('ref_axis',(0.,-0.94284446121751,-0.333233134534162));
#52660=DIRECTION('center_axis',(0.,0.333233134534162,-0.94284446121751));
#52661=DIRECTION('ref_axis',(0.,0.94284446121751,0.333233134534162));
#52662=DIRECTION('',(0.,-0.333233134534162,0.94284446121751));
#52663=DIRECTION('center_axis',(0.,0.333233134534159,-0.942844461217511));
#52664=DIRECTION('ref_axis',(0.,-0.942844461217511,-0.333233134534159));
#52665=DIRECTION('center_axis',(0.,-0.333233134534162,0.94284446121751));
#52666=DIRECTION('ref_axis',(0.,-0.94284446121751,-0.333233134534162));
#52667=DIRECTION('center_axis',(0.,0.333233134534159,-0.942844461217511));
#52668=DIRECTION('ref_axis',(0.,-0.942844461217511,-0.333233134534159));
#52669=DIRECTION('',(0.,0.333233134534162,-0.94284446121751));
#52670=DIRECTION('center_axis',(0.,-0.333233134534162,0.94284446121751));
#52671=DIRECTION('ref_axis',(0.,-0.94284446121751,-0.333233134534162));
#52672=DIRECTION('center_axis',(0.,-0.333233134534162,0.94284446121751));
#52673=DIRECTION('ref_axis',(0.,-0.94284446121751,-0.333233134534162));
#52674=DIRECTION('center_axis',(0.,0.333233134534162,-0.94284446121751));
#52675=DIRECTION('ref_axis',(0.,0.94284446121751,0.333233134534162));
#52676=DIRECTION('',(0.,-0.333233134534162,0.94284446121751));
#52677=DIRECTION('center_axis',(0.,0.333233134534159,-0.942844461217511));
#52678=DIRECTION('ref_axis',(0.,-0.942844461217511,-0.333233134534159));
#52679=DIRECTION('center_axis',(0.,-0.333233134534162,0.94284446121751));
#52680=DIRECTION('ref_axis',(0.,-0.94284446121751,-0.333233134534162));
#52681=DIRECTION('center_axis',(0.,0.333233134534159,-0.942844461217511));
#52682=DIRECTION('ref_axis',(0.,-0.942844461217511,-0.333233134534159));
#52683=DIRECTION('',(0.,0.333233134534162,-0.94284446121751));
#52684=DIRECTION('center_axis',(0.,0.333233134534162,-0.94284446121751));
#52685=DIRECTION('ref_axis',(0.,-0.94284446121751,-0.333233134534162));
#52686=DIRECTION('center_axis',(0.,-0.333233134534162,0.94284446121751));
#52687=DIRECTION('ref_axis',(0.,-0.94284446121751,-0.333233134534162));
#52688=DIRECTION('center_axis',(0.,0.333233134534162,-0.94284446121751));
#52689=DIRECTION('ref_axis',(0.,0.94284446121751,0.333233134534162));
#52690=DIRECTION('',(0.,-0.333233134534162,0.94284446121751));
#52691=DIRECTION('center_axis',(0.,0.333233134534159,-0.942844461217511));
#52692=DIRECTION('ref_axis',(0.,-0.942844461217511,-0.333233134534159));
#52693=DIRECTION('center_axis',(0.,-0.333233134534162,0.94284446121751));
#52694=DIRECTION('ref_axis',(0.,-0.94284446121751,-0.333233134534162));
#52695=DIRECTION('center_axis',(0.,0.333233134534159,-0.942844461217511));
#52696=DIRECTION('ref_axis',(0.,-0.942844461217511,-0.333233134534159));
#52697=DIRECTION('',(0.,0.333233134534162,-0.94284446121751));
#52698=DIRECTION('center_axis',(0.,0.333233134534162,-0.94284446121751));
#52699=DIRECTION('ref_axis',(0.,-0.94284446121751,-0.333233134534162));
#52700=DIRECTION('center_axis',(0.,-0.333233134534162,0.94284446121751));
#52701=DIRECTION('ref_axis',(0.,-0.94284446121751,-0.333233134534161));
#52702=DIRECTION('center_axis',(0.,0.333233134534162,-0.94284446121751));
#52703=DIRECTION('ref_axis',(0.,0.94284446121751,0.333233134534162));
#52704=DIRECTION('',(0.,-0.333233134534162,0.94284446121751));
#52705=DIRECTION('center_axis',(0.,0.333233134534159,-0.942844461217511));
#52706=DIRECTION('ref_axis',(0.,-0.942844461217511,-0.333233134534159));
#52707=DIRECTION('center_axis',(0.,-0.333233134534162,0.94284446121751));
#52708=DIRECTION('ref_axis',(0.,-0.94284446121751,-0.333233134534162));
#52709=DIRECTION('center_axis',(0.,0.333233134534159,-0.942844461217511));
#52710=DIRECTION('ref_axis',(0.,-0.942844461217511,-0.333233134534159));
#52711=DIRECTION('',(0.,0.333233134534162,-0.94284446121751));
#52712=DIRECTION('center_axis',(0.,0.333233134534162,-0.94284446121751));
#52713=DIRECTION('ref_axis',(0.,-0.94284446121751,-0.333233134534162));
#52714=DIRECTION('center_axis',(0.,-0.333233134534162,0.94284446121751));
#52715=DIRECTION('ref_axis',(0.,-0.94284446121751,-0.333233134534162));
#52716=DIRECTION('center_axis',(0.,0.333233134534162,-0.94284446121751));
#52717=DIRECTION('ref_axis',(0.,0.94284446121751,0.333233134534162));
#52718=DIRECTION('',(0.,-0.333233134534162,0.94284446121751));
#52719=DIRECTION('center_axis',(0.,0.333233134534159,-0.942844461217511));
#52720=DIRECTION('ref_axis',(0.,-0.942844461217511,-0.333233134534159));
#52721=DIRECTION('center_axis',(0.,-0.333233134534162,0.94284446121751));
#52722=DIRECTION('ref_axis',(0.,-0.94284446121751,-0.333233134534162));
#52723=DIRECTION('center_axis',(0.,0.333233134534159,-0.942844461217511));
#52724=DIRECTION('ref_axis',(0.,-0.942844461217511,-0.333233134534159));
#52725=DIRECTION('',(0.,0.333233134534162,-0.94284446121751));
#52726=DIRECTION('center_axis',(0.,0.333233134534162,-0.94284446121751));
#52727=DIRECTION('ref_axis',(0.,-0.94284446121751,-0.333233134534162));
#52728=DIRECTION('center_axis',(0.,-0.333233134534162,0.94284446121751));
#52729=DIRECTION('ref_axis',(0.,-0.94284446121751,-0.333233134534162));
#52730=DIRECTION('center_axis',(0.,0.333233134534162,-0.94284446121751));
#52731=DIRECTION('ref_axis',(0.,0.94284446121751,0.333233134534162));
#52732=DIRECTION('',(0.,-0.333233134534162,0.94284446121751));
#52733=DIRECTION('center_axis',(0.,0.333233134534159,-0.942844461217511));
#52734=DIRECTION('ref_axis',(0.,-0.942844461217511,-0.333233134534159));
#52735=DIRECTION('center_axis',(0.,-0.333233134534162,0.94284446121751));
#52736=DIRECTION('ref_axis',(0.,-0.94284446121751,-0.333233134534162));
#52737=DIRECTION('center_axis',(0.,0.333233134534159,-0.942844461217511));
#52738=DIRECTION('ref_axis',(0.,-0.942844461217511,-0.333233134534159));
#52739=DIRECTION('',(0.,0.333233134534161,-0.94284446121751));
#52740=DIRECTION('center_axis',(0.,0.333233134534162,-0.94284446121751));
#52741=DIRECTION('ref_axis',(0.,-0.94284446121751,-0.333233134534162));
#52742=DIRECTION('center_axis',(0.,-0.333233134534162,0.94284446121751));
#52743=DIRECTION('ref_axis',(0.,-0.94284446121751,-0.333233134534162));
#52744=DIRECTION('center_axis',(0.,0.333233134534162,-0.94284446121751));
#52745=DIRECTION('ref_axis',(0.,0.94284446121751,0.333233134534162));
#52746=DIRECTION('',(0.,-0.333233134534162,0.94284446121751));
#52747=DIRECTION('center_axis',(0.,0.333233134534159,-0.942844461217511));
#52748=DIRECTION('ref_axis',(0.,-0.942844461217511,-0.333233134534159));
#52749=DIRECTION('center_axis',(0.,-0.333233134534162,0.94284446121751));
#52750=DIRECTION('ref_axis',(0.,-0.94284446121751,-0.333233134534162));
#52751=DIRECTION('center_axis',(0.,0.333233134534159,-0.942844461217511));
#52752=DIRECTION('ref_axis',(0.,-0.942844461217511,-0.333233134534159));
#52753=DIRECTION('',(0.,0.333233134534162,-0.94284446121751));
#52754=DIRECTION('center_axis',(0.,0.333233134534162,-0.94284446121751));
#52755=DIRECTION('ref_axis',(0.,-0.94284446121751,-0.333233134534162));
#52756=DIRECTION('center_axis',(0.,-0.333233134534162,0.94284446121751));
#52757=DIRECTION('ref_axis',(0.,-0.94284446121751,-0.333233134534162));
#52758=DIRECTION('center_axis',(0.,0.333233134534162,-0.94284446121751));
#52759=DIRECTION('ref_axis',(0.,0.94284446121751,0.333233134534162));
#52760=DIRECTION('',(0.,-0.333233134534162,0.94284446121751));
#52761=DIRECTION('center_axis',(0.,0.333233134534159,-0.942844461217511));
#52762=DIRECTION('ref_axis',(0.,-0.942844461217511,-0.333233134534159));
#52763=DIRECTION('center_axis',(0.,-0.333233134534162,0.94284446121751));
#52764=DIRECTION('ref_axis',(0.,-0.94284446121751,-0.333233134534162));
#52765=DIRECTION('center_axis',(0.,0.333233134534159,-0.942844461217511));
#52766=DIRECTION('ref_axis',(0.,-0.942844461217511,-0.333233134534159));
#52767=DIRECTION('',(0.,0.333233134534162,-0.94284446121751));
#52768=DIRECTION('center_axis',(0.,0.333233134534162,-0.94284446121751));
#52769=DIRECTION('ref_axis',(0.,-0.94284446121751,-0.333233134534162));
#52770=DIRECTION('center_axis',(0.,-0.333233134534162,0.94284446121751));
#52771=DIRECTION('ref_axis',(0.,-0.94284446121751,-0.333233134534162));
#52772=DIRECTION('center_axis',(0.,0.333233134534162,-0.94284446121751));
#52773=DIRECTION('ref_axis',(0.,0.94284446121751,0.333233134534162));
#52774=DIRECTION('',(0.,-0.333233134534162,0.94284446121751));
#52775=DIRECTION('center_axis',(0.,0.333233134534159,-0.942844461217511));
#52776=DIRECTION('ref_axis',(0.,-0.942844461217511,-0.333233134534159));
#52777=DIRECTION('center_axis',(0.,-0.333233134534162,0.94284446121751));
#52778=DIRECTION('ref_axis',(0.,-0.94284446121751,-0.333233134534162));
#52779=DIRECTION('center_axis',(0.,0.333233134534159,-0.942844461217511));
#52780=DIRECTION('ref_axis',(0.,-0.942844461217511,-0.333233134534159));
#52781=DIRECTION('',(0.,0.333233134534162,-0.94284446121751));
#52782=DIRECTION('center_axis',(0.,0.333233134534162,-0.94284446121751));
#52783=DIRECTION('ref_axis',(0.,-0.94284446121751,-0.333233134534162));
#52784=DIRECTION('center_axis',(0.,-0.333233134534162,0.94284446121751));
#52785=DIRECTION('ref_axis',(0.,-0.94284446121751,-0.333233134534162));
#52786=DIRECTION('center_axis',(0.,0.333233134534162,-0.94284446121751));
#52787=DIRECTION('ref_axis',(0.,0.94284446121751,0.333233134534162));
#52788=DIRECTION('',(0.,-0.333233134534162,0.94284446121751));
#52789=DIRECTION('center_axis',(0.,0.333233134534159,-0.942844461217511));
#52790=DIRECTION('ref_axis',(0.,-0.942844461217511,-0.333233134534159));
#52791=DIRECTION('center_axis',(0.,-0.333233134534162,0.94284446121751));
#52792=DIRECTION('ref_axis',(0.,-0.94284446121751,-0.333233134534162));
#52793=DIRECTION('center_axis',(0.,0.333233134534159,-0.942844461217511));
#52794=DIRECTION('ref_axis',(0.,-0.942844461217511,-0.333233134534159));
#52795=DIRECTION('',(0.,0.333233134534162,-0.94284446121751));
#52796=DIRECTION('center_axis',(0.,-0.333233134534162,0.94284446121751));
#52797=DIRECTION('ref_axis',(0.,-0.94284446121751,-0.333233134534162));
#52798=DIRECTION('center_axis',(0.,-0.333233134534162,0.94284446121751));
#52799=DIRECTION('ref_axis',(0.,-0.94284446121751,-0.333233134534162));
#52800=DIRECTION('center_axis',(0.,0.333233134534162,-0.94284446121751));
#52801=DIRECTION('ref_axis',(0.,0.94284446121751,0.333233134534162));
#52802=DIRECTION('',(0.,-0.333233134534162,0.94284446121751));
#52803=DIRECTION('center_axis',(0.,0.333233134534159,-0.942844461217511));
#52804=DIRECTION('ref_axis',(0.,-0.942844461217511,-0.333233134534159));
#52805=DIRECTION('center_axis',(0.,-0.333233134534162,0.94284446121751));
#52806=DIRECTION('ref_axis',(0.,-0.94284446121751,-0.333233134534162));
#52807=DIRECTION('center_axis',(0.,0.333233134534159,-0.942844461217511));
#52808=DIRECTION('ref_axis',(0.,-0.942844461217511,-0.333233134534159));
#52809=DIRECTION('',(0.,0.333233134534162,-0.94284446121751));
#52810=DIRECTION('center_axis',(0.,0.333233134534162,-0.94284446121751));
#52811=DIRECTION('ref_axis',(0.,-0.94284446121751,-0.333233134534162));
#52812=DIRECTION('center_axis',(0.,-0.333233134534162,0.94284446121751));
#52813=DIRECTION('ref_axis',(0.,-0.94284446121751,-0.333233134534162));
#52814=DIRECTION('center_axis',(0.,0.333233134534162,-0.94284446121751));
#52815=DIRECTION('ref_axis',(0.,0.94284446121751,0.333233134534162));
#52816=DIRECTION('',(0.,-0.333233134534162,0.94284446121751));
#52817=DIRECTION('center_axis',(0.,0.333233134534159,-0.942844461217511));
#52818=DIRECTION('ref_axis',(0.,-0.942844461217511,-0.333233134534159));
#52819=DIRECTION('center_axis',(0.,-0.333233134534162,0.94284446121751));
#52820=DIRECTION('ref_axis',(0.,-0.94284446121751,-0.333233134534162));
#52821=DIRECTION('center_axis',(0.,0.333233134534159,-0.942844461217511));
#52822=DIRECTION('ref_axis',(0.,-0.942844461217511,-0.333233134534159));
#52823=DIRECTION('',(0.,0.333233134534162,-0.94284446121751));
#52824=DIRECTION('center_axis',(0.,0.333233134534162,-0.94284446121751));
#52825=DIRECTION('ref_axis',(0.,-0.94284446121751,-0.333233134534162));
#52826=DIRECTION('center_axis',(0.,-0.333233134534162,0.94284446121751));
#52827=DIRECTION('ref_axis',(0.,-0.94284446121751,-0.333233134534162));
#52828=DIRECTION('center_axis',(0.,0.333233134534162,-0.94284446121751));
#52829=DIRECTION('ref_axis',(0.,0.94284446121751,0.333233134534162));
#52830=DIRECTION('',(0.,-0.333233134534162,0.942844461217511));
#52831=DIRECTION('center_axis',(0.,0.333233134534159,-0.942844461217511));
#52832=DIRECTION('ref_axis',(0.,-0.942844461217511,-0.333233134534159));
#52833=DIRECTION('center_axis',(0.,-0.333233134534162,0.94284446121751));
#52834=DIRECTION('ref_axis',(0.,-0.94284446121751,-0.333233134534162));
#52835=DIRECTION('center_axis',(0.,0.333233134534159,-0.942844461217511));
#52836=DIRECTION('ref_axis',(0.,-0.942844461217511,-0.333233134534159));
#52837=DIRECTION('',(0.,0.333233134534162,-0.94284446121751));
#52838=DIRECTION('center_axis',(0.,0.333233134534162,-0.94284446121751));
#52839=DIRECTION('ref_axis',(0.,-0.94284446121751,-0.333233134534162));
#52840=DIRECTION('center_axis',(0.,-0.333233134534162,0.94284446121751));
#52841=DIRECTION('ref_axis',(0.,-0.94284446121751,-0.333233134534162));
#52842=DIRECTION('center_axis',(0.,0.333233134534162,-0.94284446121751));
#52843=DIRECTION('ref_axis',(0.,0.94284446121751,0.333233134534162));
#52844=DIRECTION('',(0.,-0.333233134534162,0.94284446121751));
#52845=DIRECTION('center_axis',(0.,0.333233134534159,-0.942844461217511));
#52846=DIRECTION('ref_axis',(0.,-0.942844461217511,-0.333233134534159));
#52847=DIRECTION('center_axis',(0.,-0.333233134534162,0.94284446121751));
#52848=DIRECTION('ref_axis',(0.,-0.94284446121751,-0.333233134534162));
#52849=DIRECTION('center_axis',(0.,0.333233134534159,-0.942844461217511));
#52850=DIRECTION('ref_axis',(0.,-0.942844461217511,-0.333233134534159));
#52851=DIRECTION('',(0.,0.333233134534162,-0.94284446121751));
#52852=DIRECTION('center_axis',(0.,0.333233134534162,-0.94284446121751));
#52853=DIRECTION('ref_axis',(0.,-0.94284446121751,-0.333233134534162));
#52854=DIRECTION('center_axis',(0.,-0.333233134534162,0.94284446121751));
#52855=DIRECTION('ref_axis',(0.,-0.94284446121751,-0.333233134534162));
#52856=DIRECTION('center_axis',(0.,0.333233134534162,-0.94284446121751));
#52857=DIRECTION('ref_axis',(0.,0.94284446121751,0.333233134534162));
#52858=DIRECTION('',(0.,-0.333233134534162,0.94284446121751));
#52859=DIRECTION('center_axis',(0.,0.333233134534159,-0.942844461217511));
#52860=DIRECTION('ref_axis',(0.,-0.942844461217511,-0.333233134534159));
#52861=DIRECTION('center_axis',(0.,-0.333233134534162,0.94284446121751));
#52862=DIRECTION('ref_axis',(0.,-0.94284446121751,-0.333233134534162));
#52863=DIRECTION('center_axis',(0.,0.333233134534159,-0.942844461217511));
#52864=DIRECTION('ref_axis',(0.,-0.942844461217511,-0.333233134534159));
#52865=DIRECTION('',(0.,0.333233134534162,-0.94284446121751));
#52866=DIRECTION('center_axis',(0.,0.333233134534162,-0.94284446121751));
#52867=DIRECTION('ref_axis',(0.,-0.94284446121751,-0.333233134534162));
#52868=DIRECTION('center_axis',(0.,-0.333233134534162,0.94284446121751));
#52869=DIRECTION('ref_axis',(0.,-0.94284446121751,-0.333233134534162));
#52870=DIRECTION('center_axis',(0.,0.333233134534162,-0.94284446121751));
#52871=DIRECTION('ref_axis',(0.,0.94284446121751,0.333233134534162));
#52872=DIRECTION('',(0.,-0.333233134534162,0.94284446121751));
#52873=DIRECTION('center_axis',(0.,0.333233134534159,-0.942844461217511));
#52874=DIRECTION('ref_axis',(0.,-0.942844461217511,-0.333233134534159));
#52875=DIRECTION('center_axis',(0.,-0.333233134534162,0.94284446121751));
#52876=DIRECTION('ref_axis',(0.,-0.94284446121751,-0.333233134534162));
#52877=DIRECTION('center_axis',(0.,0.333233134534159,-0.942844461217511));
#52878=DIRECTION('ref_axis',(0.,-0.942844461217511,-0.333233134534159));
#52879=DIRECTION('',(0.,0.333233134534162,-0.94284446121751));
#52880=DIRECTION('center_axis',(0.,0.333233134534162,-0.94284446121751));
#52881=DIRECTION('ref_axis',(0.,-0.94284446121751,-0.333233134534162));
#52882=DIRECTION('center_axis',(0.,-0.333233134534162,0.94284446121751));
#52883=DIRECTION('ref_axis',(0.,-0.94284446121751,-0.333233134534162));
#52884=DIRECTION('center_axis',(0.,0.333233134534162,-0.94284446121751));
#52885=DIRECTION('ref_axis',(0.,0.94284446121751,0.333233134534162));
#52886=DIRECTION('',(0.,-0.333233134534162,0.94284446121751));
#52887=DIRECTION('center_axis',(0.,0.333233134534159,-0.942844461217511));
#52888=DIRECTION('ref_axis',(0.,-0.942844461217511,-0.333233134534159));
#52889=DIRECTION('center_axis',(0.,-0.333233134534162,0.94284446121751));
#52890=DIRECTION('ref_axis',(0.,-0.94284446121751,-0.333233134534162));
#52891=DIRECTION('center_axis',(0.,0.333233134534159,-0.942844461217511));
#52892=DIRECTION('ref_axis',(0.,-0.942844461217511,-0.333233134534159));
#52893=DIRECTION('',(0.,0.333233134534162,-0.94284446121751));
#52894=DIRECTION('center_axis',(0.,0.333233134534162,-0.94284446121751));
#52895=DIRECTION('ref_axis',(0.,-0.94284446121751,-0.333233134534162));
#52896=DIRECTION('center_axis',(0.,-0.333233134534162,0.94284446121751));
#52897=DIRECTION('ref_axis',(0.,-0.94284446121751,-0.333233134534162));
#52898=DIRECTION('center_axis',(0.,0.333233134534162,-0.94284446121751));
#52899=DIRECTION('ref_axis',(0.,0.94284446121751,0.333233134534162));
#52900=DIRECTION('',(0.,-0.333233134534162,0.94284446121751));
#52901=DIRECTION('center_axis',(0.,0.333233134534159,-0.942844461217511));
#52902=DIRECTION('ref_axis',(0.,-0.942844461217511,-0.333233134534159));
#52903=DIRECTION('center_axis',(0.,-0.333233134534162,0.94284446121751));
#52904=DIRECTION('ref_axis',(0.,-0.94284446121751,-0.333233134534162));
#52905=DIRECTION('center_axis',(0.,0.333233134534159,-0.942844461217511));
#52906=DIRECTION('ref_axis',(0.,-0.942844461217511,-0.333233134534159));
#52907=DIRECTION('',(0.,0.333233134534162,-0.94284446121751));
#52908=DIRECTION('center_axis',(0.,0.333233134534162,-0.94284446121751));
#52909=DIRECTION('ref_axis',(0.,-0.94284446121751,-0.333233134534162));
#52910=DIRECTION('center_axis',(0.,-0.333233134534162,0.94284446121751));
#52911=DIRECTION('ref_axis',(0.,-0.94284446121751,-0.333233134534162));
#52912=DIRECTION('center_axis',(0.,0.333233134534162,-0.94284446121751));
#52913=DIRECTION('ref_axis',(0.,0.94284446121751,0.333233134534162));
#52914=DIRECTION('',(0.,-0.333233134534162,0.94284446121751));
#52915=DIRECTION('center_axis',(0.,0.333233134534159,-0.942844461217511));
#52916=DIRECTION('ref_axis',(0.,-0.942844461217511,-0.333233134534159));
#52917=DIRECTION('center_axis',(0.,-0.333233134534162,0.94284446121751));
#52918=DIRECTION('ref_axis',(0.,-0.94284446121751,-0.333233134534162));
#52919=DIRECTION('center_axis',(0.,0.333233134534159,-0.942844461217511));
#52920=DIRECTION('ref_axis',(0.,-0.942844461217511,-0.333233134534159));
#52921=DIRECTION('',(0.,0.333233134534162,-0.94284446121751));
#52922=DIRECTION('center_axis',(0.,-0.333233134534162,0.94284446121751));
#52923=DIRECTION('ref_axis',(0.,-0.94284446121751,-0.333233134534162));
#52924=DIRECTION('center_axis',(0.,-0.333233134534162,0.94284446121751));
#52925=DIRECTION('ref_axis',(0.,-0.94284446121751,-0.333233134534162));
#52926=DIRECTION('center_axis',(0.,0.333233134534162,-0.94284446121751));
#52927=DIRECTION('ref_axis',(0.,0.94284446121751,0.333233134534162));
#52928=DIRECTION('',(0.,-0.333233134534162,0.94284446121751));
#52929=DIRECTION('center_axis',(0.,0.333233134534159,-0.942844461217511));
#52930=DIRECTION('ref_axis',(0.,-0.942844461217511,-0.333233134534159));
#52931=DIRECTION('center_axis',(0.,-0.333233134534162,0.94284446121751));
#52932=DIRECTION('ref_axis',(0.,-0.94284446121751,-0.333233134534162));
#52933=DIRECTION('center_axis',(0.,0.333233134534159,-0.942844461217511));
#52934=DIRECTION('ref_axis',(0.,-0.942844461217511,-0.333233134534159));
#52935=DIRECTION('',(0.,0.333233134534162,-0.94284446121751));
#52936=DIRECTION('center_axis',(0.,0.333233134534162,-0.94284446121751));
#52937=DIRECTION('ref_axis',(0.,-0.94284446121751,-0.333233134534162));
#52938=DIRECTION('center_axis',(0.,-0.333233134534162,0.94284446121751));
#52939=DIRECTION('ref_axis',(0.,-0.94284446121751,-0.333233134534162));
#52940=DIRECTION('center_axis',(0.,0.333233134534162,-0.94284446121751));
#52941=DIRECTION('ref_axis',(0.,0.94284446121751,0.333233134534162));
#52942=DIRECTION('',(0.,-0.333233134534162,0.94284446121751));
#52943=DIRECTION('center_axis',(0.,0.333233134534159,-0.942844461217511));
#52944=DIRECTION('ref_axis',(0.,-0.942844461217511,-0.333233134534159));
#52945=DIRECTION('center_axis',(0.,-0.333233134534162,0.94284446121751));
#52946=DIRECTION('ref_axis',(0.,-0.94284446121751,-0.333233134534162));
#52947=DIRECTION('center_axis',(0.,0.333233134534159,-0.942844461217511));
#52948=DIRECTION('ref_axis',(0.,-0.942844461217511,-0.333233134534159));
#52949=DIRECTION('',(0.,0.333233134534162,-0.94284446121751));
#52950=DIRECTION('center_axis',(0.,0.333233134534162,-0.94284446121751));
#52951=DIRECTION('ref_axis',(0.,-0.94284446121751,-0.333233134534162));
#52952=DIRECTION('center_axis',(0.,-0.333233134534162,0.94284446121751));
#52953=DIRECTION('ref_axis',(0.,-0.94284446121751,-0.333233134534162));
#52954=DIRECTION('center_axis',(0.,0.333233134534162,-0.94284446121751));
#52955=DIRECTION('ref_axis',(0.,0.94284446121751,0.333233134534162));
#52956=DIRECTION('',(0.,-0.333233134534162,0.94284446121751));
#52957=DIRECTION('center_axis',(0.,0.333233134534159,-0.942844461217511));
#52958=DIRECTION('ref_axis',(0.,-0.942844461217511,-0.333233134534159));
#52959=DIRECTION('center_axis',(0.,-0.333233134534162,0.94284446121751));
#52960=DIRECTION('ref_axis',(0.,-0.94284446121751,-0.333233134534162));
#52961=DIRECTION('center_axis',(0.,0.333233134534159,-0.942844461217511));
#52962=DIRECTION('ref_axis',(0.,-0.942844461217511,-0.333233134534159));
#52963=DIRECTION('',(0.,0.333233134534162,-0.94284446121751));
#52964=DIRECTION('center_axis',(0.,0.333233134534162,-0.94284446121751));
#52965=DIRECTION('ref_axis',(0.,-0.94284446121751,-0.333233134534162));
#52966=DIRECTION('center_axis',(0.,-0.333233134534162,0.94284446121751));
#52967=DIRECTION('ref_axis',(0.,-0.94284446121751,-0.333233134534162));
#52968=DIRECTION('center_axis',(0.,0.333233134534162,-0.94284446121751));
#52969=DIRECTION('ref_axis',(0.,0.94284446121751,0.333233134534162));
#52970=DIRECTION('',(0.,-0.333233134534162,0.94284446121751));
#52971=DIRECTION('center_axis',(0.,0.333233134534159,-0.942844461217511));
#52972=DIRECTION('ref_axis',(0.,-0.942844461217511,-0.333233134534159));
#52973=DIRECTION('center_axis',(0.,-0.333233134534162,0.94284446121751));
#52974=DIRECTION('ref_axis',(0.,-0.94284446121751,-0.333233134534162));
#52975=DIRECTION('center_axis',(0.,0.333233134534159,-0.942844461217511));
#52976=DIRECTION('ref_axis',(0.,-0.942844461217511,-0.333233134534159));
#52977=DIRECTION('',(0.,0.333233134534162,-0.94284446121751));
#52978=DIRECTION('center_axis',(0.,0.333233134534162,-0.94284446121751));
#52979=DIRECTION('ref_axis',(0.,-0.94284446121751,-0.333233134534162));
#52980=DIRECTION('center_axis',(0.,-0.333233134534162,0.94284446121751));
#52981=DIRECTION('ref_axis',(0.,-0.94284446121751,-0.333233134534162));
#52982=DIRECTION('center_axis',(0.,0.333233134534162,-0.94284446121751));
#52983=DIRECTION('ref_axis',(0.,0.94284446121751,0.333233134534162));
#52984=DIRECTION('',(0.,-0.333233134534162,0.94284446121751));
#52985=DIRECTION('center_axis',(0.,0.333233134534159,-0.942844461217511));
#52986=DIRECTION('ref_axis',(0.,-0.942844461217511,-0.333233134534159));
#52987=DIRECTION('center_axis',(0.,-0.333233134534162,0.94284446121751));
#52988=DIRECTION('ref_axis',(0.,-0.94284446121751,-0.333233134534162));
#52989=DIRECTION('center_axis',(0.,0.333233134534159,-0.942844461217511));
#52990=DIRECTION('ref_axis',(0.,-0.942844461217511,-0.333233134534159));
#52991=DIRECTION('',(0.,0.333233134534162,-0.94284446121751));
#52992=DIRECTION('center_axis',(0.,0.333233134534162,-0.94284446121751));
#52993=DIRECTION('ref_axis',(0.,-0.94284446121751,-0.333233134534162));
#52994=DIRECTION('center_axis',(0.,-0.333233134534162,0.94284446121751));
#52995=DIRECTION('ref_axis',(0.,-0.94284446121751,-0.333233134534162));
#52996=DIRECTION('center_axis',(0.,0.333233134534162,-0.94284446121751));
#52997=DIRECTION('ref_axis',(0.,0.94284446121751,0.333233134534162));
#52998=DIRECTION('',(0.,-0.333233134534162,0.94284446121751));
#52999=DIRECTION('center_axis',(0.,0.333233134534159,-0.942844461217511));
#53000=DIRECTION('ref_axis',(0.,-0.942844461217511,-0.333233134534159));
#53001=DIRECTION('center_axis',(0.,-0.333233134534162,0.94284446121751));
#53002=DIRECTION('ref_axis',(0.,-0.94284446121751,-0.333233134534162));
#53003=DIRECTION('center_axis',(0.,0.333233134534159,-0.942844461217511));
#53004=DIRECTION('ref_axis',(0.,-0.942844461217511,-0.333233134534159));
#53005=DIRECTION('',(0.,0.333233134534162,-0.94284446121751));
#53006=DIRECTION('center_axis',(0.,0.333233134534162,-0.94284446121751));
#53007=DIRECTION('ref_axis',(0.,-0.94284446121751,-0.333233134534162));
#53008=DIRECTION('center_axis',(0.,-0.333233134534162,0.94284446121751));
#53009=DIRECTION('ref_axis',(0.,-0.94284446121751,-0.333233134534162));
#53010=DIRECTION('center_axis',(0.,0.333233134534162,-0.94284446121751));
#53011=DIRECTION('ref_axis',(0.,0.94284446121751,0.333233134534162));
#53012=DIRECTION('',(0.,-0.333233134534162,0.94284446121751));
#53013=DIRECTION('center_axis',(0.,0.333233134534159,-0.942844461217511));
#53014=DIRECTION('ref_axis',(0.,-0.942844461217511,-0.333233134534159));
#53015=DIRECTION('center_axis',(0.,-0.333233134534162,0.94284446121751));
#53016=DIRECTION('ref_axis',(0.,-0.94284446121751,-0.333233134534162));
#53017=DIRECTION('center_axis',(0.,0.333233134534159,-0.942844461217511));
#53018=DIRECTION('ref_axis',(0.,-0.942844461217511,-0.333233134534159));
#53019=DIRECTION('',(0.,0.333233134534162,-0.94284446121751));
#53020=DIRECTION('center_axis',(0.,0.333233134534162,-0.94284446121751));
#53021=DIRECTION('ref_axis',(0.,-0.94284446121751,-0.333233134534162));
#53022=DIRECTION('center_axis',(0.,-0.333233134534162,0.94284446121751));
#53023=DIRECTION('ref_axis',(0.,-0.94284446121751,-0.333233134534162));
#53024=DIRECTION('center_axis',(0.,0.333233134534162,-0.94284446121751));
#53025=DIRECTION('ref_axis',(0.,0.94284446121751,0.333233134534162));
#53026=DIRECTION('',(0.,-0.333233134534162,0.94284446121751));
#53027=DIRECTION('center_axis',(0.,0.333233134534159,-0.942844461217511));
#53028=DIRECTION('ref_axis',(0.,-0.942844461217511,-0.333233134534159));
#53029=DIRECTION('center_axis',(0.,-0.333233134534162,0.94284446121751));
#53030=DIRECTION('ref_axis',(0.,-0.94284446121751,-0.333233134534162));
#53031=DIRECTION('center_axis',(0.,0.333233134534159,-0.942844461217511));
#53032=DIRECTION('ref_axis',(0.,-0.942844461217511,-0.333233134534159));
#53033=DIRECTION('',(0.,0.333233134534162,-0.94284446121751));
#53034=DIRECTION('center_axis',(0.,0.333233134534162,-0.94284446121751));
#53035=DIRECTION('ref_axis',(0.,-0.94284446121751,-0.333233134534162));
#53036=DIRECTION('center_axis',(0.,-0.333233134534162,0.94284446121751));
#53037=DIRECTION('ref_axis',(0.,-0.94284446121751,-0.333233134534162));
#53038=DIRECTION('center_axis',(0.,0.333233134534162,-0.94284446121751));
#53039=DIRECTION('ref_axis',(0.,0.94284446121751,0.333233134534162));
#53040=DIRECTION('',(0.,-0.333233134534162,0.94284446121751));
#53041=DIRECTION('center_axis',(0.,0.333233134534159,-0.942844461217511));
#53042=DIRECTION('ref_axis',(0.,-0.942844461217511,-0.333233134534159));
#53043=DIRECTION('center_axis',(0.,-0.333233134534162,0.94284446121751));
#53044=DIRECTION('ref_axis',(0.,-0.94284446121751,-0.333233134534162));
#53045=DIRECTION('center_axis',(0.,0.333233134534159,-0.942844461217511));
#53046=DIRECTION('ref_axis',(0.,-0.942844461217511,-0.333233134534159));
#53047=DIRECTION('',(0.,0.333233134534162,-0.94284446121751));
#53048=DIRECTION('center_axis',(0.,-0.333233134534162,0.94284446121751));
#53049=DIRECTION('ref_axis',(0.,-0.94284446121751,-0.333233134534162));
#53050=DIRECTION('center_axis',(0.,-0.333233134534162,0.94284446121751));
#53051=DIRECTION('ref_axis',(0.,-0.94284446121751,-0.333233134534162));
#53052=DIRECTION('center_axis',(0.,0.333233134534162,-0.94284446121751));
#53053=DIRECTION('ref_axis',(0.,0.94284446121751,0.333233134534162));
#53054=DIRECTION('',(0.,-0.333233134534162,0.94284446121751));
#53055=DIRECTION('center_axis',(0.,0.333233134534159,-0.942844461217511));
#53056=DIRECTION('ref_axis',(0.,-0.942844461217511,-0.333233134534159));
#53057=DIRECTION('center_axis',(0.,-0.333233134534162,0.94284446121751));
#53058=DIRECTION('ref_axis',(0.,-0.94284446121751,-0.333233134534161));
#53059=DIRECTION('center_axis',(0.,0.333233134534159,-0.942844461217511));
#53060=DIRECTION('ref_axis',(0.,-0.942844461217511,-0.333233134534159));
#53061=DIRECTION('',(0.,0.333233134534162,-0.94284446121751));
#53062=DIRECTION('center_axis',(0.,0.333233134534162,-0.94284446121751));
#53063=DIRECTION('ref_axis',(0.,-0.94284446121751,-0.333233134534162));
#53064=DIRECTION('center_axis',(0.,-0.333233134534162,0.94284446121751));
#53065=DIRECTION('ref_axis',(0.,-0.94284446121751,-0.333233134534162));
#53066=DIRECTION('center_axis',(0.,0.333233134534162,-0.94284446121751));
#53067=DIRECTION('ref_axis',(0.,0.94284446121751,0.333233134534162));
#53068=DIRECTION('',(0.,-0.333233134534162,0.94284446121751));
#53069=DIRECTION('center_axis',(0.,0.333233134534159,-0.942844461217511));
#53070=DIRECTION('ref_axis',(0.,-0.942844461217511,-0.333233134534159));
#53071=DIRECTION('center_axis',(0.,-0.333233134534162,0.94284446121751));
#53072=DIRECTION('ref_axis',(0.,-0.94284446121751,-0.333233134534162));
#53073=DIRECTION('center_axis',(0.,0.333233134534159,-0.942844461217511));
#53074=DIRECTION('ref_axis',(0.,-0.942844461217511,-0.333233134534159));
#53075=DIRECTION('',(0.,0.333233134534162,-0.94284446121751));
#53076=DIRECTION('center_axis',(0.,0.333233134534162,-0.94284446121751));
#53077=DIRECTION('ref_axis',(0.,-0.94284446121751,-0.333233134534162));
#53078=DIRECTION('center_axis',(0.,-0.333233134534162,0.94284446121751));
#53079=DIRECTION('ref_axis',(0.,-0.94284446121751,-0.333233134534162));
#53080=DIRECTION('center_axis',(0.,0.333233134534162,-0.94284446121751));
#53081=DIRECTION('ref_axis',(0.,0.94284446121751,0.333233134534162));
#53082=DIRECTION('',(0.,-0.333233134534162,0.94284446121751));
#53083=DIRECTION('center_axis',(0.,0.333233134534159,-0.942844461217511));
#53084=DIRECTION('ref_axis',(0.,-0.942844461217511,-0.333233134534159));
#53085=DIRECTION('center_axis',(0.,-0.333233134534162,0.94284446121751));
#53086=DIRECTION('ref_axis',(0.,-0.94284446121751,-0.333233134534162));
#53087=DIRECTION('center_axis',(0.,0.333233134534159,-0.942844461217511));
#53088=DIRECTION('ref_axis',(0.,-0.942844461217511,-0.333233134534159));
#53089=DIRECTION('',(0.,0.333233134534162,-0.94284446121751));
#53090=DIRECTION('center_axis',(0.,0.333233134534162,-0.94284446121751));
#53091=DIRECTION('ref_axis',(0.,-0.94284446121751,-0.333233134534162));
#53092=DIRECTION('center_axis',(0.,-0.333233134534162,0.94284446121751));
#53093=DIRECTION('ref_axis',(0.,-0.94284446121751,-0.333233134534162));
#53094=DIRECTION('center_axis',(0.,0.333233134534162,-0.94284446121751));
#53095=DIRECTION('ref_axis',(0.,0.94284446121751,0.333233134534162));
#53096=DIRECTION('',(0.,-0.333233134534162,0.94284446121751));
#53097=DIRECTION('center_axis',(0.,0.333233134534159,-0.942844461217511));
#53098=DIRECTION('ref_axis',(0.,-0.942844461217511,-0.333233134534159));
#53099=DIRECTION('center_axis',(0.,-0.333233134534162,0.94284446121751));
#53100=DIRECTION('ref_axis',(0.,-0.94284446121751,-0.333233134534162));
#53101=DIRECTION('center_axis',(0.,0.333233134534159,-0.942844461217511));
#53102=DIRECTION('ref_axis',(0.,-0.942844461217511,-0.333233134534159));
#53103=DIRECTION('',(0.,0.333233134534162,-0.94284446121751));
#53104=DIRECTION('center_axis',(0.,0.333233134534162,-0.94284446121751));
#53105=DIRECTION('ref_axis',(0.,-0.94284446121751,-0.333233134534162));
#53106=DIRECTION('center_axis',(0.,-0.333233134534162,0.94284446121751));
#53107=DIRECTION('ref_axis',(0.,-0.94284446121751,-0.333233134534162));
#53108=DIRECTION('center_axis',(0.,0.333233134534162,-0.94284446121751));
#53109=DIRECTION('ref_axis',(0.,0.94284446121751,0.333233134534162));
#53110=DIRECTION('',(0.,-0.333233134534162,0.94284446121751));
#53111=DIRECTION('center_axis',(0.,0.333233134534159,-0.942844461217511));
#53112=DIRECTION('ref_axis',(0.,-0.942844461217511,-0.333233134534159));
#53113=DIRECTION('center_axis',(0.,-0.333233134534162,0.94284446121751));
#53114=DIRECTION('ref_axis',(0.,-0.94284446121751,-0.333233134534162));
#53115=DIRECTION('center_axis',(0.,0.333233134534159,-0.942844461217511));
#53116=DIRECTION('ref_axis',(0.,-0.942844461217511,-0.333233134534159));
#53117=DIRECTION('',(0.,0.333233134534162,-0.94284446121751));
#53118=DIRECTION('center_axis',(0.,0.333233134534162,-0.94284446121751));
#53119=DIRECTION('ref_axis',(0.,-0.94284446121751,-0.333233134534162));
#53120=DIRECTION('center_axis',(0.,-0.333233134534162,0.94284446121751));
#53121=DIRECTION('ref_axis',(0.,-0.94284446121751,-0.333233134534162));
#53122=DIRECTION('center_axis',(0.,0.333233134534162,-0.94284446121751));
#53123=DIRECTION('ref_axis',(0.,0.94284446121751,0.333233134534162));
#53124=DIRECTION('',(0.,-0.333233134534162,0.94284446121751));
#53125=DIRECTION('center_axis',(0.,0.333233134534159,-0.942844461217511));
#53126=DIRECTION('ref_axis',(0.,-0.942844461217511,-0.333233134534159));
#53127=DIRECTION('center_axis',(0.,-0.333233134534162,0.94284446121751));
#53128=DIRECTION('ref_axis',(0.,-0.94284446121751,-0.333233134534162));
#53129=DIRECTION('center_axis',(0.,0.333233134534159,-0.942844461217511));
#53130=DIRECTION('ref_axis',(0.,-0.942844461217511,-0.333233134534159));
#53131=DIRECTION('',(0.,0.333233134534162,-0.94284446121751));
#53132=DIRECTION('center_axis',(0.,0.333233134534162,-0.94284446121751));
#53133=DIRECTION('ref_axis',(0.,-0.94284446121751,-0.333233134534162));
#53134=DIRECTION('center_axis',(0.,-0.333233134534162,0.94284446121751));
#53135=DIRECTION('ref_axis',(0.,-0.94284446121751,-0.333233134534162));
#53136=DIRECTION('center_axis',(0.,0.333233134534162,-0.94284446121751));
#53137=DIRECTION('ref_axis',(0.,0.94284446121751,0.333233134534162));
#53138=DIRECTION('',(0.,-0.333233134534162,0.94284446121751));
#53139=DIRECTION('center_axis',(0.,0.333233134534159,-0.942844461217511));
#53140=DIRECTION('ref_axis',(0.,-0.942844461217511,-0.333233134534159));
#53141=DIRECTION('center_axis',(0.,-0.333233134534162,0.94284446121751));
#53142=DIRECTION('ref_axis',(0.,-0.94284446121751,-0.333233134534162));
#53143=DIRECTION('center_axis',(0.,0.333233134534159,-0.942844461217511));
#53144=DIRECTION('ref_axis',(0.,-0.942844461217511,-0.333233134534159));
#53145=DIRECTION('',(0.,0.333233134534162,-0.94284446121751));
#53146=DIRECTION('center_axis',(0.,0.333233134534162,-0.94284446121751));
#53147=DIRECTION('ref_axis',(0.,-0.94284446121751,-0.333233134534162));
#53148=DIRECTION('center_axis',(0.,-0.333233134534162,0.94284446121751));
#53149=DIRECTION('ref_axis',(0.,-0.94284446121751,-0.333233134534162));
#53150=DIRECTION('center_axis',(0.,0.333233134534162,-0.94284446121751));
#53151=DIRECTION('ref_axis',(0.,0.94284446121751,0.333233134534162));
#53152=DIRECTION('',(0.,-0.333233134534162,0.94284446121751));
#53153=DIRECTION('center_axis',(0.,0.333233134534159,-0.942844461217511));
#53154=DIRECTION('ref_axis',(0.,-0.942844461217511,-0.333233134534159));
#53155=DIRECTION('center_axis',(0.,-0.333233134534162,0.94284446121751));
#53156=DIRECTION('ref_axis',(0.,-0.94284446121751,-0.333233134534162));
#53157=DIRECTION('center_axis',(0.,0.333233134534159,-0.942844461217511));
#53158=DIRECTION('ref_axis',(0.,-0.942844461217511,-0.333233134534159));
#53159=DIRECTION('',(0.,0.333233134534161,-0.94284446121751));
#53160=DIRECTION('center_axis',(0.,0.333233134534162,-0.94284446121751));
#53161=DIRECTION('ref_axis',(0.,-0.94284446121751,-0.333233134534162));
#53162=DIRECTION('center_axis',(0.,-0.333233134534162,0.94284446121751));
#53163=DIRECTION('ref_axis',(0.,-0.94284446121751,-0.333233134534162));
#53164=DIRECTION('center_axis',(0.,0.333233134534162,-0.94284446121751));
#53165=DIRECTION('ref_axis',(0.,0.94284446121751,0.333233134534162));
#53166=DIRECTION('',(0.,-0.333233134534162,0.94284446121751));
#53167=DIRECTION('center_axis',(0.,0.333233134534159,-0.942844461217511));
#53168=DIRECTION('ref_axis',(0.,-0.942844461217511,-0.333233134534159));
#53169=DIRECTION('center_axis',(0.,-0.333233134534162,0.94284446121751));
#53170=DIRECTION('ref_axis',(0.,-0.94284446121751,-0.333233134534162));
#53171=DIRECTION('center_axis',(0.,0.333233134534159,-0.942844461217511));
#53172=DIRECTION('ref_axis',(0.,-0.942844461217511,-0.333233134534159));
#53173=DIRECTION('',(0.,0.333233134534162,-0.94284446121751));
#53174=DIRECTION('center_axis',(0.,-0.333233134534162,0.94284446121751));
#53175=DIRECTION('ref_axis',(0.,-0.94284446121751,-0.333233134534162));
#53176=DIRECTION('center_axis',(0.,-0.333233134534162,0.94284446121751));
#53177=DIRECTION('ref_axis',(0.,-0.94284446121751,-0.333233134534162));
#53178=DIRECTION('center_axis',(0.,0.333233134534162,-0.94284446121751));
#53179=DIRECTION('ref_axis',(0.,0.94284446121751,0.333233134534162));
#53180=DIRECTION('',(0.,-0.333233134534162,0.94284446121751));
#53181=DIRECTION('center_axis',(0.,0.333233134534159,-0.942844461217511));
#53182=DIRECTION('ref_axis',(0.,-0.942844461217511,-0.333233134534159));
#53183=DIRECTION('center_axis',(0.,-0.333233134534162,0.94284446121751));
#53184=DIRECTION('ref_axis',(0.,-0.94284446121751,-0.333233134534161));
#53185=DIRECTION('center_axis',(0.,0.333233134534159,-0.942844461217511));
#53186=DIRECTION('ref_axis',(0.,-0.942844461217511,-0.333233134534159));
#53187=DIRECTION('',(0.,0.333233134534162,-0.94284446121751));
#53188=DIRECTION('center_axis',(0.,0.333233134534162,-0.94284446121751));
#53189=DIRECTION('ref_axis',(0.,-0.94284446121751,-0.333233134534162));
#53190=DIRECTION('center_axis',(0.,-0.333233134534162,0.94284446121751));
#53191=DIRECTION('ref_axis',(0.,-0.94284446121751,-0.333233134534162));
#53192=DIRECTION('center_axis',(0.,0.333233134534162,-0.94284446121751));
#53193=DIRECTION('ref_axis',(0.,0.94284446121751,0.333233134534162));
#53194=DIRECTION('',(0.,-0.333233134534162,0.94284446121751));
#53195=DIRECTION('center_axis',(0.,0.333233134534159,-0.942844461217511));
#53196=DIRECTION('ref_axis',(0.,-0.942844461217511,-0.333233134534159));
#53197=DIRECTION('center_axis',(0.,-0.333233134534162,0.94284446121751));
#53198=DIRECTION('ref_axis',(0.,-0.94284446121751,-0.333233134534162));
#53199=DIRECTION('center_axis',(0.,0.333233134534159,-0.942844461217511));
#53200=DIRECTION('ref_axis',(0.,-0.942844461217511,-0.333233134534159));
#53201=DIRECTION('',(0.,0.333233134534162,-0.94284446121751));
#53202=DIRECTION('center_axis',(0.,0.333233134534162,-0.94284446121751));
#53203=DIRECTION('ref_axis',(0.,-0.94284446121751,-0.333233134534162));
#53204=DIRECTION('center_axis',(0.,-0.333233134534162,0.94284446121751));
#53205=DIRECTION('ref_axis',(0.,-0.94284446121751,-0.333233134534162));
#53206=DIRECTION('center_axis',(0.,0.333233134534162,-0.94284446121751));
#53207=DIRECTION('ref_axis',(0.,0.94284446121751,0.333233134534162));
#53208=DIRECTION('',(0.,-0.333233134534162,0.94284446121751));
#53209=DIRECTION('center_axis',(0.,0.333233134534159,-0.942844461217511));
#53210=DIRECTION('ref_axis',(0.,-0.942844461217511,-0.333233134534159));
#53211=DIRECTION('center_axis',(0.,-0.333233134534162,0.94284446121751));
#53212=DIRECTION('ref_axis',(0.,-0.94284446121751,-0.333233134534162));
#53213=DIRECTION('center_axis',(0.,0.333233134534159,-0.942844461217511));
#53214=DIRECTION('ref_axis',(0.,-0.942844461217511,-0.333233134534159));
#53215=DIRECTION('',(0.,0.333233134534162,-0.94284446121751));
#53216=DIRECTION('center_axis',(0.,0.333233134534162,-0.94284446121751));
#53217=DIRECTION('ref_axis',(0.,-0.94284446121751,-0.333233134534162));
#53218=DIRECTION('center_axis',(0.,-0.333233134534162,0.94284446121751));
#53219=DIRECTION('ref_axis',(0.,-0.94284446121751,-0.333233134534162));
#53220=DIRECTION('center_axis',(0.,0.333233134534162,-0.94284446121751));
#53221=DIRECTION('ref_axis',(0.,0.94284446121751,0.333233134534162));
#53222=DIRECTION('',(0.,-0.333233134534162,0.94284446121751));
#53223=DIRECTION('center_axis',(0.,0.333233134534159,-0.942844461217511));
#53224=DIRECTION('ref_axis',(0.,-0.942844461217511,-0.333233134534159));
#53225=DIRECTION('center_axis',(0.,-0.333233134534162,0.94284446121751));
#53226=DIRECTION('ref_axis',(0.,-0.94284446121751,-0.333233134534162));
#53227=DIRECTION('center_axis',(0.,0.333233134534159,-0.942844461217511));
#53228=DIRECTION('ref_axis',(0.,-0.942844461217511,-0.333233134534159));
#53229=DIRECTION('',(0.,0.333233134534162,-0.94284446121751));
#53230=DIRECTION('center_axis',(0.,0.333233134534162,-0.94284446121751));
#53231=DIRECTION('ref_axis',(0.,-0.94284446121751,-0.333233134534162));
#53232=DIRECTION('center_axis',(0.,-0.333233134534162,0.94284446121751));
#53233=DIRECTION('ref_axis',(0.,-0.94284446121751,-0.333233134534162));
#53234=DIRECTION('center_axis',(0.,0.333233134534162,-0.94284446121751));
#53235=DIRECTION('ref_axis',(0.,0.94284446121751,0.333233134534162));
#53236=DIRECTION('',(0.,-0.333233134534162,0.94284446121751));
#53237=DIRECTION('center_axis',(0.,0.333233134534159,-0.942844461217511));
#53238=DIRECTION('ref_axis',(0.,-0.942844461217511,-0.333233134534159));
#53239=DIRECTION('center_axis',(0.,-0.333233134534162,0.94284446121751));
#53240=DIRECTION('ref_axis',(0.,-0.94284446121751,-0.333233134534162));
#53241=DIRECTION('center_axis',(0.,0.333233134534159,-0.942844461217511));
#53242=DIRECTION('ref_axis',(0.,-0.942844461217511,-0.333233134534159));
#53243=DIRECTION('',(0.,0.333233134534162,-0.94284446121751));
#53244=DIRECTION('center_axis',(0.,0.333233134534162,-0.94284446121751));
#53245=DIRECTION('ref_axis',(0.,-0.94284446121751,-0.333233134534162));
#53246=DIRECTION('center_axis',(0.,-0.333233134534162,0.94284446121751));
#53247=DIRECTION('ref_axis',(0.,-0.94284446121751,-0.333233134534162));
#53248=DIRECTION('center_axis',(0.,0.333233134534162,-0.94284446121751));
#53249=DIRECTION('ref_axis',(0.,0.94284446121751,0.333233134534162));
#53250=DIRECTION('',(0.,-0.333233134534162,0.94284446121751));
#53251=DIRECTION('center_axis',(0.,0.333233134534159,-0.942844461217511));
#53252=DIRECTION('ref_axis',(0.,-0.942844461217511,-0.333233134534159));
#53253=DIRECTION('center_axis',(0.,-0.333233134534162,0.94284446121751));
#53254=DIRECTION('ref_axis',(0.,-0.94284446121751,-0.333233134534161));
#53255=DIRECTION('center_axis',(0.,0.333233134534159,-0.942844461217511));
#53256=DIRECTION('ref_axis',(0.,-0.942844461217511,-0.333233134534159));
#53257=DIRECTION('',(0.,0.333233134534162,-0.94284446121751));
#53258=DIRECTION('center_axis',(0.,0.333233134534162,-0.94284446121751));
#53259=DIRECTION('ref_axis',(0.,-0.94284446121751,-0.333233134534162));
#53260=DIRECTION('center_axis',(0.,-0.333233134534162,0.94284446121751));
#53261=DIRECTION('ref_axis',(0.,-0.94284446121751,-0.333233134534162));
#53262=DIRECTION('center_axis',(0.,0.333233134534162,-0.94284446121751));
#53263=DIRECTION('ref_axis',(0.,0.94284446121751,0.333233134534162));
#53264=DIRECTION('',(0.,-0.333233134534162,0.94284446121751));
#53265=DIRECTION('center_axis',(0.,0.333233134534159,-0.942844461217511));
#53266=DIRECTION('ref_axis',(0.,-0.942844461217511,-0.333233134534159));
#53267=DIRECTION('center_axis',(0.,-0.333233134534162,0.94284446121751));
#53268=DIRECTION('ref_axis',(0.,-0.94284446121751,-0.333233134534162));
#53269=DIRECTION('center_axis',(0.,0.333233134534159,-0.942844461217511));
#53270=DIRECTION('ref_axis',(0.,-0.942844461217511,-0.333233134534159));
#53271=DIRECTION('',(0.,0.333233134534162,-0.94284446121751));
#53272=DIRECTION('center_axis',(0.,0.333233134534162,-0.94284446121751));
#53273=DIRECTION('ref_axis',(0.,-0.94284446121751,-0.333233134534162));
#53274=DIRECTION('center_axis',(0.,-0.333233134534162,0.94284446121751));
#53275=DIRECTION('ref_axis',(0.,-0.94284446121751,-0.333233134534162));
#53276=DIRECTION('center_axis',(0.,0.333233134534162,-0.94284446121751));
#53277=DIRECTION('ref_axis',(0.,0.94284446121751,0.333233134534162));
#53278=DIRECTION('',(0.,-0.333233134534162,0.94284446121751));
#53279=DIRECTION('center_axis',(0.,0.333233134534159,-0.942844461217511));
#53280=DIRECTION('ref_axis',(0.,-0.942844461217511,-0.333233134534159));
#53281=DIRECTION('center_axis',(0.,-0.333233134534162,0.94284446121751));
#53282=DIRECTION('ref_axis',(0.,-0.94284446121751,-0.333233134534162));
#53283=DIRECTION('center_axis',(0.,0.333233134534159,-0.942844461217511));
#53284=DIRECTION('ref_axis',(0.,-0.942844461217511,-0.333233134534159));
#53285=DIRECTION('',(0.,0.333233134534162,-0.94284446121751));
#53286=DIRECTION('center_axis',(0.,-0.333233134534162,0.94284446121751));
#53287=DIRECTION('ref_axis',(0.,-0.94284446121751,-0.333233134534162));
#53288=DIRECTION('center_axis',(0.,-0.333233134534162,0.94284446121751));
#53289=DIRECTION('ref_axis',(0.,-0.94284446121751,-0.333233134534162));
#53290=DIRECTION('center_axis',(0.,0.333233134534162,-0.94284446121751));
#53291=DIRECTION('ref_axis',(0.,0.94284446121751,0.333233134534162));
#53292=DIRECTION('',(0.,-0.333233134534162,0.94284446121751));
#53293=DIRECTION('center_axis',(0.,0.333233134534159,-0.942844461217511));
#53294=DIRECTION('ref_axis',(0.,-0.942844461217511,-0.333233134534159));
#53295=DIRECTION('center_axis',(0.,-0.333233134534162,0.94284446121751));
#53296=DIRECTION('ref_axis',(0.,-0.94284446121751,-0.333233134534162));
#53297=DIRECTION('center_axis',(0.,0.333233134534159,-0.942844461217511));
#53298=DIRECTION('ref_axis',(0.,-0.942844461217511,-0.333233134534159));
#53299=DIRECTION('',(0.,0.333233134534162,-0.94284446121751));
#53300=DIRECTION('center_axis',(0.,0.333233134534162,-0.94284446121751));
#53301=DIRECTION('ref_axis',(0.,-0.94284446121751,-0.333233134534162));
#53302=DIRECTION('center_axis',(0.,-0.333233134534162,0.94284446121751));
#53303=DIRECTION('ref_axis',(0.,-0.94284446121751,-0.333233134534162));
#53304=DIRECTION('center_axis',(0.,0.333233134534162,-0.94284446121751));
#53305=DIRECTION('ref_axis',(0.,0.94284446121751,0.333233134534162));
#53306=DIRECTION('',(0.,-0.333233134534162,0.94284446121751));
#53307=DIRECTION('center_axis',(0.,0.333233134534159,-0.942844461217511));
#53308=DIRECTION('ref_axis',(0.,-0.942844461217511,-0.333233134534159));
#53309=DIRECTION('center_axis',(0.,-0.333233134534162,0.94284446121751));
#53310=DIRECTION('ref_axis',(0.,-0.94284446121751,-0.333233134534162));
#53311=DIRECTION('center_axis',(0.,0.333233134534159,-0.942844461217511));
#53312=DIRECTION('ref_axis',(0.,-0.942844461217511,-0.333233134534159));
#53313=DIRECTION('',(0.,0.333233134534162,-0.94284446121751));
#53314=DIRECTION('center_axis',(0.,0.333233134534162,-0.94284446121751));
#53315=DIRECTION('ref_axis',(0.,-0.94284446121751,-0.333233134534162));
#53316=DIRECTION('center_axis',(0.,-0.333233134534162,0.94284446121751));
#53317=DIRECTION('ref_axis',(0.,-0.94284446121751,-0.333233134534162));
#53318=DIRECTION('center_axis',(0.,0.333233134534162,-0.94284446121751));
#53319=DIRECTION('ref_axis',(0.,0.94284446121751,0.333233134534162));
#53320=DIRECTION('',(0.,-0.333233134534162,0.94284446121751));
#53321=DIRECTION('center_axis',(0.,0.333233134534159,-0.942844461217511));
#53322=DIRECTION('ref_axis',(0.,-0.942844461217511,-0.333233134534159));
#53323=DIRECTION('center_axis',(0.,-0.333233134534162,0.94284446121751));
#53324=DIRECTION('ref_axis',(0.,-0.94284446121751,-0.333233134534162));
#53325=DIRECTION('center_axis',(0.,0.333233134534159,-0.942844461217511));
#53326=DIRECTION('ref_axis',(0.,-0.942844461217511,-0.333233134534159));
#53327=DIRECTION('',(0.,0.333233134534162,-0.94284446121751));
#53328=DIRECTION('center_axis',(0.,0.333233134534162,-0.94284446121751));
#53329=DIRECTION('ref_axis',(0.,-0.94284446121751,-0.333233134534162));
#53330=DIRECTION('center_axis',(0.,-0.333233134534162,0.94284446121751));
#53331=DIRECTION('ref_axis',(0.,-0.94284446121751,-0.333233134534162));
#53332=DIRECTION('center_axis',(0.,0.333233134534162,-0.94284446121751));
#53333=DIRECTION('ref_axis',(0.,0.94284446121751,0.333233134534162));
#53334=DIRECTION('',(0.,-0.333233134534162,0.94284446121751));
#53335=DIRECTION('center_axis',(0.,0.333233134534159,-0.942844461217511));
#53336=DIRECTION('ref_axis',(0.,-0.942844461217511,-0.333233134534159));
#53337=DIRECTION('center_axis',(0.,-0.333233134534162,0.94284446121751));
#53338=DIRECTION('ref_axis',(0.,-0.94284446121751,-0.333233134534162));
#53339=DIRECTION('center_axis',(0.,0.333233134534159,-0.942844461217511));
#53340=DIRECTION('ref_axis',(0.,-0.942844461217511,-0.333233134534159));
#53341=DIRECTION('',(0.,0.333233134534162,-0.94284446121751));
#53342=DIRECTION('center_axis',(0.,0.333233134534162,-0.94284446121751));
#53343=DIRECTION('ref_axis',(0.,-0.94284446121751,-0.333233134534162));
#53344=DIRECTION('center_axis',(0.,-0.333233134534162,0.94284446121751));
#53345=DIRECTION('ref_axis',(0.,-0.94284446121751,-0.333233134534162));
#53346=DIRECTION('center_axis',(0.,0.333233134534162,-0.94284446121751));
#53347=DIRECTION('ref_axis',(0.,0.94284446121751,0.333233134534162));
#53348=DIRECTION('',(0.,-0.333233134534162,0.94284446121751));
#53349=DIRECTION('center_axis',(0.,0.333233134534159,-0.942844461217511));
#53350=DIRECTION('ref_axis',(0.,-0.942844461217511,-0.333233134534159));
#53351=DIRECTION('center_axis',(0.,-0.333233134534162,0.94284446121751));
#53352=DIRECTION('ref_axis',(0.,-0.94284446121751,-0.333233134534162));
#53353=DIRECTION('center_axis',(0.,0.333233134534159,-0.942844461217511));
#53354=DIRECTION('ref_axis',(0.,-0.942844461217511,-0.333233134534159));
#53355=DIRECTION('',(0.,0.333233134534162,-0.94284446121751));
#53356=DIRECTION('center_axis',(0.,0.333233134534162,-0.94284446121751));
#53357=DIRECTION('ref_axis',(0.,-0.94284446121751,-0.333233134534162));
#53358=DIRECTION('center_axis',(0.,-0.333233134534162,0.94284446121751));
#53359=DIRECTION('ref_axis',(0.,-0.94284446121751,-0.333233134534162));
#53360=DIRECTION('center_axis',(0.,0.333233134534162,-0.94284446121751));
#53361=DIRECTION('ref_axis',(0.,0.94284446121751,0.333233134534162));
#53362=DIRECTION('',(0.,-0.333233134534162,0.94284446121751));
#53363=DIRECTION('center_axis',(0.,0.333233134534159,-0.942844461217511));
#53364=DIRECTION('ref_axis',(0.,-0.942844461217511,-0.333233134534159));
#53365=DIRECTION('center_axis',(0.,-0.333233134534162,0.94284446121751));
#53366=DIRECTION('ref_axis',(0.,-0.94284446121751,-0.333233134534162));
#53367=DIRECTION('center_axis',(0.,0.333233134534159,-0.942844461217511));
#53368=DIRECTION('ref_axis',(0.,-0.942844461217511,-0.333233134534159));
#53369=DIRECTION('',(0.,0.333233134534162,-0.94284446121751));
#53370=DIRECTION('center_axis',(0.,0.333233134534162,-0.94284446121751));
#53371=DIRECTION('ref_axis',(0.,-0.94284446121751,-0.333233134534162));
#53372=DIRECTION('center_axis',(0.,-0.333233134534162,0.94284446121751));
#53373=DIRECTION('ref_axis',(0.,-0.94284446121751,-0.333233134534162));
#53374=DIRECTION('center_axis',(0.,0.333233134534162,-0.94284446121751));
#53375=DIRECTION('ref_axis',(0.,0.94284446121751,0.333233134534162));
#53376=DIRECTION('',(0.,-0.333233134534162,0.94284446121751));
#53377=DIRECTION('center_axis',(0.,0.333233134534159,-0.942844461217511));
#53378=DIRECTION('ref_axis',(0.,-0.942844461217511,-0.333233134534159));
#53379=DIRECTION('center_axis',(0.,-0.333233134534162,0.94284446121751));
#53380=DIRECTION('ref_axis',(0.,-0.94284446121751,-0.333233134534162));
#53381=DIRECTION('center_axis',(0.,0.333233134534159,-0.942844461217511));
#53382=DIRECTION('ref_axis',(0.,-0.942844461217511,-0.333233134534159));
#53383=DIRECTION('',(0.,0.333233134534162,-0.94284446121751));
#53384=DIRECTION('center_axis',(0.,0.333233134534162,-0.94284446121751));
#53385=DIRECTION('ref_axis',(0.,-0.94284446121751,-0.333233134534162));
#53386=DIRECTION('center_axis',(0.,-0.333233134534162,0.94284446121751));
#53387=DIRECTION('ref_axis',(0.,-0.94284446121751,-0.333233134534162));
#53388=DIRECTION('center_axis',(0.,0.333233134534162,-0.94284446121751));
#53389=DIRECTION('ref_axis',(0.,0.94284446121751,0.333233134534162));
#53390=DIRECTION('',(0.,-0.333233134534162,0.94284446121751));
#53391=DIRECTION('center_axis',(0.,0.333233134534159,-0.942844461217511));
#53392=DIRECTION('ref_axis',(0.,-0.942844461217511,-0.333233134534159));
#53393=DIRECTION('center_axis',(0.,-0.333233134534162,0.94284446121751));
#53394=DIRECTION('ref_axis',(0.,-0.94284446121751,-0.333233134534162));
#53395=DIRECTION('center_axis',(0.,0.333233134534159,-0.942844461217511));
#53396=DIRECTION('ref_axis',(0.,-0.942844461217511,-0.333233134534159));
#53397=DIRECTION('',(0.,0.333233134534162,-0.94284446121751));
#53398=DIRECTION('center_axis',(0.,0.333233134534162,-0.94284446121751));
#53399=DIRECTION('ref_axis',(0.,-0.94284446121751,-0.333233134534162));
#53400=DIRECTION('center_axis',(0.,-0.333233134534162,0.94284446121751));
#53401=DIRECTION('ref_axis',(0.,-0.94284446121751,-0.333233134534162));
#53402=DIRECTION('center_axis',(0.,0.333233134534162,-0.94284446121751));
#53403=DIRECTION('ref_axis',(0.,0.94284446121751,0.333233134534162));
#53404=DIRECTION('',(0.,-0.333233134534162,0.94284446121751));
#53405=DIRECTION('center_axis',(0.,0.333233134534159,-0.942844461217511));
#53406=DIRECTION('ref_axis',(0.,-0.942844461217511,-0.333233134534159));
#53407=DIRECTION('center_axis',(0.,-0.333233134534162,0.94284446121751));
#53408=DIRECTION('ref_axis',(0.,-0.94284446121751,-0.333233134534162));
#53409=DIRECTION('center_axis',(0.,0.333233134534159,-0.942844461217511));
#53410=DIRECTION('ref_axis',(0.,-0.942844461217511,-0.333233134534159));
#53411=DIRECTION('',(0.,0.333233134534162,-0.94284446121751));
#53412=DIRECTION('center_axis',(0.,-0.333233134534162,0.94284446121751));
#53413=DIRECTION('ref_axis',(0.,-0.94284446121751,-0.333233134534162));
#53414=DIRECTION('center_axis',(0.,-0.333233134534162,0.94284446121751));
#53415=DIRECTION('ref_axis',(0.,-0.94284446121751,-0.333233134534162));
#53416=DIRECTION('center_axis',(0.,0.333233134534162,-0.94284446121751));
#53417=DIRECTION('ref_axis',(0.,0.94284446121751,0.333233134534162));
#53418=DIRECTION('',(0.,-0.333233134534162,0.94284446121751));
#53419=DIRECTION('center_axis',(0.,0.333233134534159,-0.942844461217511));
#53420=DIRECTION('ref_axis',(0.,-0.942844461217511,-0.333233134534159));
#53421=DIRECTION('center_axis',(0.,-0.333233134534162,0.94284446121751));
#53422=DIRECTION('ref_axis',(0.,-0.94284446121751,-0.333233134534162));
#53423=DIRECTION('center_axis',(0.,0.333233134534159,-0.942844461217511));
#53424=DIRECTION('ref_axis',(0.,-0.942844461217511,-0.333233134534159));
#53425=DIRECTION('',(0.,0.333233134534162,-0.94284446121751));
#53426=DIRECTION('center_axis',(0.,0.333233134534162,-0.94284446121751));
#53427=DIRECTION('ref_axis',(0.,-0.94284446121751,-0.333233134534162));
#53428=DIRECTION('center_axis',(0.,-0.333233134534162,0.94284446121751));
#53429=DIRECTION('ref_axis',(0.,-0.94284446121751,-0.333233134534162));
#53430=DIRECTION('center_axis',(0.,0.333233134534162,-0.94284446121751));
#53431=DIRECTION('ref_axis',(0.,0.94284446121751,0.333233134534162));
#53432=DIRECTION('',(0.,-0.333233134534162,0.94284446121751));
#53433=DIRECTION('center_axis',(0.,0.333233134534159,-0.942844461217511));
#53434=DIRECTION('ref_axis',(0.,-0.942844461217511,-0.333233134534159));
#53435=DIRECTION('center_axis',(0.,-0.333233134534162,0.94284446121751));
#53436=DIRECTION('ref_axis',(0.,-0.94284446121751,-0.333233134534162));
#53437=DIRECTION('center_axis',(0.,0.333233134534159,-0.942844461217511));
#53438=DIRECTION('ref_axis',(0.,-0.942844461217511,-0.333233134534159));
#53439=DIRECTION('',(0.,0.333233134534162,-0.94284446121751));
#53440=DIRECTION('center_axis',(0.,0.333233134534162,-0.94284446121751));
#53441=DIRECTION('ref_axis',(0.,-0.94284446121751,-0.333233134534162));
#53442=DIRECTION('center_axis',(0.,-0.333233134534162,0.94284446121751));
#53443=DIRECTION('ref_axis',(0.,-0.94284446121751,-0.333233134534162));
#53444=DIRECTION('center_axis',(0.,0.333233134534162,-0.94284446121751));
#53445=DIRECTION('ref_axis',(0.,0.94284446121751,0.333233134534162));
#53446=DIRECTION('',(0.,-0.333233134534162,0.94284446121751));
#53447=DIRECTION('center_axis',(0.,0.333233134534159,-0.942844461217511));
#53448=DIRECTION('ref_axis',(0.,-0.942844461217511,-0.333233134534159));
#53449=DIRECTION('center_axis',(0.,-0.333233134534162,0.94284446121751));
#53450=DIRECTION('ref_axis',(0.,-0.94284446121751,-0.333233134534162));
#53451=DIRECTION('center_axis',(0.,0.333233134534159,-0.942844461217511));
#53452=DIRECTION('ref_axis',(0.,-0.942844461217511,-0.333233134534159));
#53453=DIRECTION('',(0.,0.333233134534162,-0.94284446121751));
#53454=DIRECTION('center_axis',(0.,0.333233134534162,-0.94284446121751));
#53455=DIRECTION('ref_axis',(0.,-0.94284446121751,-0.333233134534162));
#53456=DIRECTION('center_axis',(0.,-0.333233134534162,0.94284446121751));
#53457=DIRECTION('ref_axis',(0.,-0.94284446121751,-0.333233134534162));
#53458=DIRECTION('center_axis',(0.,0.333233134534162,-0.94284446121751));
#53459=DIRECTION('ref_axis',(0.,0.94284446121751,0.333233134534162));
#53460=DIRECTION('',(0.,-0.333233134534162,0.94284446121751));
#53461=DIRECTION('center_axis',(0.,0.333233134534159,-0.942844461217511));
#53462=DIRECTION('ref_axis',(0.,-0.942844461217511,-0.333233134534159));
#53463=DIRECTION('center_axis',(0.,-0.333233134534162,0.94284446121751));
#53464=DIRECTION('ref_axis',(0.,-0.94284446121751,-0.333233134534162));
#53465=DIRECTION('center_axis',(0.,0.333233134534159,-0.942844461217511));
#53466=DIRECTION('ref_axis',(0.,-0.942844461217511,-0.333233134534159));
#53467=DIRECTION('',(0.,0.333233134534162,-0.94284446121751));
#53468=DIRECTION('center_axis',(0.,0.333233134534162,-0.94284446121751));
#53469=DIRECTION('ref_axis',(0.,-0.94284446121751,-0.333233134534162));
#53470=DIRECTION('center_axis',(0.,-0.333233134534162,0.94284446121751));
#53471=DIRECTION('ref_axis',(0.,-0.94284446121751,-0.333233134534162));
#53472=DIRECTION('center_axis',(0.,0.333233134534162,-0.94284446121751));
#53473=DIRECTION('ref_axis',(0.,0.94284446121751,0.333233134534162));
#53474=DIRECTION('',(0.,-0.333233134534162,0.94284446121751));
#53475=DIRECTION('center_axis',(0.,0.333233134534159,-0.942844461217511));
#53476=DIRECTION('ref_axis',(0.,-0.942844461217511,-0.333233134534159));
#53477=DIRECTION('center_axis',(0.,-0.333233134534162,0.94284446121751));
#53478=DIRECTION('ref_axis',(0.,-0.94284446121751,-0.333233134534162));
#53479=DIRECTION('center_axis',(0.,0.333233134534159,-0.942844461217511));
#53480=DIRECTION('ref_axis',(0.,-0.942844461217511,-0.333233134534159));
#53481=DIRECTION('',(0.,0.333233134534162,-0.94284446121751));
#53482=DIRECTION('center_axis',(0.,0.333233134534162,-0.94284446121751));
#53483=DIRECTION('ref_axis',(0.,-0.94284446121751,-0.333233134534162));
#53484=DIRECTION('center_axis',(0.,-0.333233134534162,0.94284446121751));
#53485=DIRECTION('ref_axis',(0.,-0.94284446121751,-0.333233134534162));
#53486=DIRECTION('center_axis',(0.,0.333233134534162,-0.94284446121751));
#53487=DIRECTION('ref_axis',(0.,0.94284446121751,0.333233134534162));
#53488=DIRECTION('',(0.,-0.333233134534162,0.94284446121751));
#53489=DIRECTION('center_axis',(0.,0.333233134534159,-0.942844461217511));
#53490=DIRECTION('ref_axis',(0.,-0.942844461217511,-0.333233134534159));
#53491=DIRECTION('center_axis',(0.,-0.333233134534162,0.94284446121751));
#53492=DIRECTION('ref_axis',(0.,-0.94284446121751,-0.333233134534162));
#53493=DIRECTION('center_axis',(0.,0.333233134534159,-0.942844461217511));
#53494=DIRECTION('ref_axis',(0.,-0.942844461217511,-0.333233134534159));
#53495=DIRECTION('',(0.,0.333233134534162,-0.94284446121751));
#53496=DIRECTION('center_axis',(0.,0.333233134534162,-0.94284446121751));
#53497=DIRECTION('ref_axis',(0.,-0.94284446121751,-0.333233134534162));
#53498=DIRECTION('center_axis',(0.,-0.333233134534162,0.94284446121751));
#53499=DIRECTION('ref_axis',(0.,-0.94284446121751,-0.333233134534162));
#53500=DIRECTION('center_axis',(0.,0.333233134534162,-0.94284446121751));
#53501=DIRECTION('ref_axis',(0.,0.94284446121751,0.333233134534162));
#53502=DIRECTION('',(0.,-0.333233134534162,0.94284446121751));
#53503=DIRECTION('center_axis',(0.,0.333233134534159,-0.942844461217511));
#53504=DIRECTION('ref_axis',(0.,-0.942844461217511,-0.333233134534159));
#53505=DIRECTION('center_axis',(0.,-0.333233134534162,0.94284446121751));
#53506=DIRECTION('ref_axis',(0.,-0.94284446121751,-0.333233134534162));
#53507=DIRECTION('center_axis',(0.,0.333233134534159,-0.942844461217511));
#53508=DIRECTION('ref_axis',(0.,-0.942844461217511,-0.333233134534159));
#53509=DIRECTION('',(0.,0.333233134534162,-0.94284446121751));
#53510=DIRECTION('center_axis',(0.,0.333233134534162,-0.94284446121751));
#53511=DIRECTION('ref_axis',(0.,-0.94284446121751,-0.333233134534162));
#53512=DIRECTION('center_axis',(0.,-0.333233134534162,0.94284446121751));
#53513=DIRECTION('ref_axis',(0.,-0.94284446121751,-0.333233134534162));
#53514=DIRECTION('center_axis',(0.,0.333233134534162,-0.94284446121751));
#53515=DIRECTION('ref_axis',(0.,0.94284446121751,0.333233134534162));
#53516=DIRECTION('',(0.,-0.333233134534162,0.94284446121751));
#53517=DIRECTION('center_axis',(0.,0.333233134534159,-0.942844461217511));
#53518=DIRECTION('ref_axis',(0.,-0.942844461217511,-0.333233134534159));
#53519=DIRECTION('center_axis',(0.,-0.333233134534162,0.94284446121751));
#53520=DIRECTION('ref_axis',(0.,-0.94284446121751,-0.333233134534162));
#53521=DIRECTION('center_axis',(0.,0.333233134534159,-0.942844461217511));
#53522=DIRECTION('ref_axis',(0.,-0.942844461217511,-0.333233134534159));
#53523=DIRECTION('',(0.,0.333233134534161,-0.94284446121751));
#53524=DIRECTION('center_axis',(0.,0.333233134534162,-0.94284446121751));
#53525=DIRECTION('ref_axis',(0.,-0.94284446121751,-0.333233134534162));
#53526=DIRECTION('center_axis',(0.,-0.333233134534162,0.94284446121751));
#53527=DIRECTION('ref_axis',(0.,-0.94284446121751,-0.333233134534162));
#53528=DIRECTION('center_axis',(0.,0.333233134534162,-0.94284446121751));
#53529=DIRECTION('ref_axis',(0.,0.94284446121751,0.333233134534162));
#53530=DIRECTION('',(0.,-0.333233134534162,0.94284446121751));
#53531=DIRECTION('center_axis',(0.,0.333233134534159,-0.942844461217511));
#53532=DIRECTION('ref_axis',(0.,-0.942844461217511,-0.333233134534159));
#53533=DIRECTION('center_axis',(0.,-0.333233134534162,0.94284446121751));
#53534=DIRECTION('ref_axis',(0.,-0.94284446121751,-0.333233134534162));
#53535=DIRECTION('center_axis',(0.,0.333233134534159,-0.942844461217511));
#53536=DIRECTION('ref_axis',(0.,-0.942844461217511,-0.333233134534159));
#53537=DIRECTION('',(0.,0.333233134534162,-0.94284446121751));
#53538=DIRECTION('center_axis',(0.,-0.333233134534162,0.94284446121751));
#53539=DIRECTION('ref_axis',(0.,-0.94284446121751,-0.333233134534162));
#53540=DIRECTION('center_axis',(0.,-0.333233134534162,0.94284446121751));
#53541=DIRECTION('ref_axis',(0.,-0.94284446121751,-0.333233134534162));
#53542=DIRECTION('center_axis',(0.,0.333233134534162,-0.94284446121751));
#53543=DIRECTION('ref_axis',(0.,0.94284446121751,0.333233134534162));
#53544=DIRECTION('',(0.,-0.333233134534162,0.94284446121751));
#53545=DIRECTION('center_axis',(0.,0.333233134534159,-0.942844461217511));
#53546=DIRECTION('ref_axis',(0.,-0.942844461217511,-0.333233134534159));
#53547=DIRECTION('center_axis',(0.,-0.333233134534162,0.94284446121751));
#53548=DIRECTION('ref_axis',(0.,-0.94284446121751,-0.333233134534162));
#53549=DIRECTION('center_axis',(0.,0.333233134534159,-0.942844461217511));
#53550=DIRECTION('ref_axis',(0.,-0.942844461217511,-0.333233134534159));
#53551=DIRECTION('',(0.,0.333233134534162,-0.94284446121751));
#53552=DIRECTION('center_axis',(0.,0.333233134534162,-0.94284446121751));
#53553=DIRECTION('ref_axis',(0.,-0.94284446121751,-0.333233134534162));
#53554=DIRECTION('center_axis',(0.,-0.333233134534162,0.94284446121751));
#53555=DIRECTION('ref_axis',(0.,-0.94284446121751,-0.333233134534162));
#53556=DIRECTION('center_axis',(0.,0.333233134534162,-0.94284446121751));
#53557=DIRECTION('ref_axis',(0.,0.94284446121751,0.333233134534162));
#53558=DIRECTION('',(0.,-0.333233134534162,0.94284446121751));
#53559=DIRECTION('center_axis',(0.,0.333233134534159,-0.942844461217511));
#53560=DIRECTION('ref_axis',(0.,-0.942844461217511,-0.333233134534159));
#53561=DIRECTION('center_axis',(0.,-0.333233134534162,0.94284446121751));
#53562=DIRECTION('ref_axis',(0.,-0.94284446121751,-0.333233134534162));
#53563=DIRECTION('center_axis',(0.,0.333233134534159,-0.942844461217511));
#53564=DIRECTION('ref_axis',(0.,-0.942844461217511,-0.333233134534159));
#53565=DIRECTION('',(0.,0.333233134534162,-0.94284446121751));
#53566=DIRECTION('center_axis',(0.,0.333233134534162,-0.94284446121751));
#53567=DIRECTION('ref_axis',(0.,-0.94284446121751,-0.333233134534162));
#53568=DIRECTION('center_axis',(0.,-0.333233134534162,0.94284446121751));
#53569=DIRECTION('ref_axis',(0.,-0.94284446121751,-0.333233134534162));
#53570=DIRECTION('center_axis',(0.,0.333233134534162,-0.94284446121751));
#53571=DIRECTION('ref_axis',(0.,0.94284446121751,0.333233134534162));
#53572=DIRECTION('',(0.,-0.333233134534162,0.94284446121751));
#53573=DIRECTION('center_axis',(0.,0.333233134534159,-0.942844461217511));
#53574=DIRECTION('ref_axis',(0.,-0.942844461217511,-0.333233134534159));
#53575=DIRECTION('center_axis',(0.,-0.333233134534162,0.94284446121751));
#53576=DIRECTION('ref_axis',(0.,-0.94284446121751,-0.333233134534162));
#53577=DIRECTION('center_axis',(0.,0.333233134534159,-0.942844461217511));
#53578=DIRECTION('ref_axis',(0.,-0.942844461217511,-0.333233134534159));
#53579=DIRECTION('',(0.,0.333233134534162,-0.94284446121751));
#53580=DIRECTION('center_axis',(0.,0.333233134534162,-0.94284446121751));
#53581=DIRECTION('ref_axis',(0.,-0.94284446121751,-0.333233134534162));
#53582=DIRECTION('center_axis',(0.,-0.333233134534162,0.94284446121751));
#53583=DIRECTION('ref_axis',(0.,-0.94284446121751,-0.333233134534162));
#53584=DIRECTION('center_axis',(0.,0.333233134534162,-0.94284446121751));
#53585=DIRECTION('ref_axis',(0.,0.94284446121751,0.333233134534162));
#53586=DIRECTION('',(0.,-0.333233134534162,0.94284446121751));
#53587=DIRECTION('center_axis',(0.,0.333233134534159,-0.942844461217511));
#53588=DIRECTION('ref_axis',(0.,-0.942844461217511,-0.333233134534159));
#53589=DIRECTION('center_axis',(0.,-0.333233134534162,0.94284446121751));
#53590=DIRECTION('ref_axis',(0.,-0.94284446121751,-0.333233134534162));
#53591=DIRECTION('center_axis',(0.,0.333233134534159,-0.942844461217511));
#53592=DIRECTION('ref_axis',(0.,-0.942844461217511,-0.333233134534159));
#53593=DIRECTION('',(0.,0.333233134534162,-0.94284446121751));
#53594=DIRECTION('center_axis',(0.,0.333233134534162,-0.94284446121751));
#53595=DIRECTION('ref_axis',(0.,-0.94284446121751,-0.333233134534162));
#53596=DIRECTION('center_axis',(0.,-0.333233134534162,0.94284446121751));
#53597=DIRECTION('ref_axis',(0.,-0.94284446121751,-0.333233134534162));
#53598=DIRECTION('center_axis',(0.,0.333233134534162,-0.94284446121751));
#53599=DIRECTION('ref_axis',(0.,0.94284446121751,0.333233134534162));
#53600=DIRECTION('',(0.,-0.333233134534162,0.94284446121751));
#53601=DIRECTION('center_axis',(0.,0.333233134534159,-0.942844461217511));
#53602=DIRECTION('ref_axis',(0.,-0.942844461217511,-0.333233134534159));
#53603=DIRECTION('center_axis',(0.,-0.333233134534162,0.94284446121751));
#53604=DIRECTION('ref_axis',(0.,-0.94284446121751,-0.333233134534162));
#53605=DIRECTION('center_axis',(0.,0.333233134534159,-0.942844461217511));
#53606=DIRECTION('ref_axis',(0.,-0.942844461217511,-0.333233134534159));
#53607=DIRECTION('',(0.,0.333233134534162,-0.94284446121751));
#53608=DIRECTION('center_axis',(0.,0.333233134534162,-0.94284446121751));
#53609=DIRECTION('ref_axis',(0.,-0.94284446121751,-0.333233134534162));
#53610=DIRECTION('center_axis',(0.,-0.333233134534162,0.94284446121751));
#53611=DIRECTION('ref_axis',(0.,-0.94284446121751,-0.333233134534162));
#53612=DIRECTION('center_axis',(0.,0.333233134534162,-0.94284446121751));
#53613=DIRECTION('ref_axis',(0.,0.94284446121751,0.333233134534162));
#53614=DIRECTION('',(0.,-0.333233134534162,0.94284446121751));
#53615=DIRECTION('center_axis',(0.,0.333233134534159,-0.942844461217511));
#53616=DIRECTION('ref_axis',(0.,-0.942844461217511,-0.333233134534159));
#53617=DIRECTION('center_axis',(0.,-0.333233134534162,0.94284446121751));
#53618=DIRECTION('ref_axis',(0.,-0.94284446121751,-0.333233134534162));
#53619=DIRECTION('center_axis',(0.,0.333233134534159,-0.942844461217511));
#53620=DIRECTION('ref_axis',(0.,-0.942844461217511,-0.333233134534159));
#53621=DIRECTION('',(0.,0.333233134534162,-0.94284446121751));
#53622=DIRECTION('center_axis',(0.,0.333233134534162,-0.94284446121751));
#53623=DIRECTION('ref_axis',(0.,-0.94284446121751,-0.333233134534162));
#53624=DIRECTION('center_axis',(0.,-0.333233134534162,0.94284446121751));
#53625=DIRECTION('ref_axis',(0.,-0.94284446121751,-0.333233134534162));
#53626=DIRECTION('center_axis',(0.,0.333233134534162,-0.94284446121751));
#53627=DIRECTION('ref_axis',(0.,0.94284446121751,0.333233134534162));
#53628=DIRECTION('',(0.,-0.333233134534162,0.94284446121751));
#53629=DIRECTION('center_axis',(0.,0.333233134534159,-0.942844461217511));
#53630=DIRECTION('ref_axis',(0.,-0.942844461217511,-0.333233134534159));
#53631=DIRECTION('center_axis',(0.,-0.333233134534162,0.94284446121751));
#53632=DIRECTION('ref_axis',(0.,-0.94284446121751,-0.333233134534162));
#53633=DIRECTION('center_axis',(0.,0.333233134534159,-0.942844461217511));
#53634=DIRECTION('ref_axis',(0.,-0.942844461217511,-0.333233134534159));
#53635=DIRECTION('',(0.,0.333233134534162,-0.94284446121751));
#53636=DIRECTION('center_axis',(0.,0.333233134534162,-0.94284446121751));
#53637=DIRECTION('ref_axis',(0.,-0.94284446121751,-0.333233134534162));
#53638=DIRECTION('center_axis',(0.,-0.333233134534162,0.94284446121751));
#53639=DIRECTION('ref_axis',(0.,-0.94284446121751,-0.333233134534162));
#53640=DIRECTION('center_axis',(0.,0.333233134534162,-0.94284446121751));
#53641=DIRECTION('ref_axis',(0.,0.94284446121751,0.333233134534162));
#53642=DIRECTION('',(0.,-0.333233134534162,0.94284446121751));
#53643=DIRECTION('center_axis',(0.,0.333233134534159,-0.942844461217511));
#53644=DIRECTION('ref_axis',(0.,-0.942844461217511,-0.333233134534159));
#53645=DIRECTION('center_axis',(0.,-0.333233134534162,0.94284446121751));
#53646=DIRECTION('ref_axis',(0.,-0.94284446121751,-0.333233134534162));
#53647=DIRECTION('center_axis',(0.,0.333233134534159,-0.942844461217511));
#53648=DIRECTION('ref_axis',(0.,-0.942844461217511,-0.333233134534159));
#53649=DIRECTION('',(0.,0.333233134534162,-0.94284446121751));
#53650=DIRECTION('center_axis',(0.,0.333233134534162,-0.94284446121751));
#53651=DIRECTION('ref_axis',(0.,-0.94284446121751,-0.333233134534162));
#53652=DIRECTION('center_axis',(0.,-0.333233134534162,0.94284446121751));
#53653=DIRECTION('ref_axis',(0.,-0.94284446121751,-0.333233134534162));
#53654=DIRECTION('center_axis',(0.,0.333233134534162,-0.94284446121751));
#53655=DIRECTION('ref_axis',(0.,0.94284446121751,0.333233134534162));
#53656=DIRECTION('',(0.,-0.333233134534162,0.94284446121751));
#53657=DIRECTION('center_axis',(0.,0.333233134534159,-0.942844461217511));
#53658=DIRECTION('ref_axis',(0.,-0.942844461217511,-0.333233134534159));
#53659=DIRECTION('center_axis',(0.,-0.333233134534162,0.94284446121751));
#53660=DIRECTION('ref_axis',(0.,-0.94284446121751,-0.333233134534162));
#53661=DIRECTION('center_axis',(0.,0.333233134534159,-0.942844461217511));
#53662=DIRECTION('ref_axis',(0.,-0.942844461217511,-0.333233134534159));
#53663=DIRECTION('',(0.,0.333233134534162,-0.94284446121751));
#53664=DIRECTION('center_axis',(0.,-0.333233134534162,0.94284446121751));
#53665=DIRECTION('ref_axis',(0.,-0.94284446121751,-0.333233134534162));
#53666=DIRECTION('center_axis',(0.,-0.333233134534162,0.94284446121751));
#53667=DIRECTION('ref_axis',(0.,-0.94284446121751,-0.333233134534162));
#53668=DIRECTION('center_axis',(0.,0.333233134534162,-0.94284446121751));
#53669=DIRECTION('ref_axis',(0.,0.94284446121751,0.333233134534162));
#53670=DIRECTION('',(0.,-0.333233134534162,0.94284446121751));
#53671=DIRECTION('center_axis',(0.,0.333233134534159,-0.942844461217511));
#53672=DIRECTION('ref_axis',(0.,-0.942844461217511,-0.333233134534159));
#53673=DIRECTION('center_axis',(0.,-0.333233134534162,0.94284446121751));
#53674=DIRECTION('ref_axis',(0.,-0.94284446121751,-0.333233134534161));
#53675=DIRECTION('center_axis',(0.,0.333233134534159,-0.942844461217511));
#53676=DIRECTION('ref_axis',(0.,-0.942844461217511,-0.333233134534159));
#53677=DIRECTION('',(0.,0.333233134534162,-0.94284446121751));
#53678=DIRECTION('center_axis',(0.,0.333233134534162,-0.94284446121751));
#53679=DIRECTION('ref_axis',(0.,-0.94284446121751,-0.333233134534162));
#53680=DIRECTION('center_axis',(0.,-0.333233134534162,0.94284446121751));
#53681=DIRECTION('ref_axis',(0.,-0.94284446121751,-0.333233134534162));
#53682=DIRECTION('center_axis',(0.,0.333233134534162,-0.94284446121751));
#53683=DIRECTION('ref_axis',(0.,0.94284446121751,0.333233134534162));
#53684=DIRECTION('',(0.,-0.333233134534162,0.94284446121751));
#53685=DIRECTION('center_axis',(0.,0.333233134534159,-0.942844461217511));
#53686=DIRECTION('ref_axis',(0.,-0.942844461217511,-0.333233134534159));
#53687=DIRECTION('center_axis',(0.,-0.333233134534162,0.94284446121751));
#53688=DIRECTION('ref_axis',(0.,-0.94284446121751,-0.333233134534162));
#53689=DIRECTION('center_axis',(0.,0.333233134534159,-0.942844461217511));
#53690=DIRECTION('ref_axis',(0.,-0.942844461217511,-0.333233134534159));
#53691=DIRECTION('',(0.,0.333233134534162,-0.94284446121751));
#53692=DIRECTION('center_axis',(0.,0.333233134534162,-0.94284446121751));
#53693=DIRECTION('ref_axis',(0.,-0.94284446121751,-0.333233134534162));
#53694=DIRECTION('center_axis',(0.,-0.333233134534162,0.94284446121751));
#53695=DIRECTION('ref_axis',(0.,-0.94284446121751,-0.333233134534162));
#53696=DIRECTION('center_axis',(0.,0.333233134534162,-0.94284446121751));
#53697=DIRECTION('ref_axis',(0.,0.94284446121751,0.333233134534162));
#53698=DIRECTION('',(0.,-0.333233134534162,0.94284446121751));
#53699=DIRECTION('center_axis',(0.,0.333233134534159,-0.942844461217511));
#53700=DIRECTION('ref_axis',(0.,-0.942844461217511,-0.333233134534159));
#53701=DIRECTION('center_axis',(0.,-0.333233134534162,0.94284446121751));
#53702=DIRECTION('ref_axis',(0.,-0.94284446121751,-0.333233134534162));
#53703=DIRECTION('center_axis',(0.,0.333233134534159,-0.942844461217511));
#53704=DIRECTION('ref_axis',(0.,-0.942844461217511,-0.333233134534159));
#53705=DIRECTION('',(0.,0.333233134534162,-0.94284446121751));
#53706=DIRECTION('center_axis',(0.,0.333233134534162,-0.94284446121751));
#53707=DIRECTION('ref_axis',(0.,-0.94284446121751,-0.333233134534162));
#53708=DIRECTION('center_axis',(0.,-0.333233134534162,0.94284446121751));
#53709=DIRECTION('ref_axis',(0.,-0.94284446121751,-0.333233134534162));
#53710=DIRECTION('center_axis',(0.,0.333233134534162,-0.94284446121751));
#53711=DIRECTION('ref_axis',(0.,0.94284446121751,0.333233134534162));
#53712=DIRECTION('',(0.,-0.333233134534162,0.94284446121751));
#53713=DIRECTION('center_axis',(0.,0.333233134534159,-0.942844461217511));
#53714=DIRECTION('ref_axis',(0.,-0.942844461217511,-0.333233134534159));
#53715=DIRECTION('center_axis',(0.,-0.333233134534162,0.94284446121751));
#53716=DIRECTION('ref_axis',(0.,-0.94284446121751,-0.333233134534162));
#53717=DIRECTION('center_axis',(0.,0.333233134534159,-0.942844461217511));
#53718=DIRECTION('ref_axis',(0.,-0.942844461217511,-0.333233134534159));
#53719=DIRECTION('',(0.,0.333233134534162,-0.94284446121751));
#53720=DIRECTION('center_axis',(0.,0.333233134534162,-0.94284446121751));
#53721=DIRECTION('ref_axis',(0.,-0.94284446121751,-0.333233134534162));
#53722=DIRECTION('center_axis',(0.,-0.333233134534162,0.94284446121751));
#53723=DIRECTION('ref_axis',(0.,-0.94284446121751,-0.333233134534162));
#53724=DIRECTION('center_axis',(0.,0.333233134534162,-0.94284446121751));
#53725=DIRECTION('ref_axis',(0.,0.94284446121751,0.333233134534162));
#53726=DIRECTION('',(0.,-0.333233134534162,0.94284446121751));
#53727=DIRECTION('center_axis',(0.,0.333233134534159,-0.942844461217511));
#53728=DIRECTION('ref_axis',(0.,-0.942844461217511,-0.333233134534159));
#53729=DIRECTION('center_axis',(0.,-0.333233134534162,0.94284446121751));
#53730=DIRECTION('ref_axis',(0.,-0.94284446121751,-0.333233134534162));
#53731=DIRECTION('center_axis',(0.,0.333233134534159,-0.942844461217511));
#53732=DIRECTION('ref_axis',(0.,-0.942844461217511,-0.333233134534159));
#53733=DIRECTION('',(0.,0.333233134534162,-0.94284446121751));
#53734=DIRECTION('center_axis',(0.,0.333233134534162,-0.94284446121751));
#53735=DIRECTION('ref_axis',(0.,-0.94284446121751,-0.333233134534162));
#53736=DIRECTION('center_axis',(0.,-0.333233134534162,0.94284446121751));
#53737=DIRECTION('ref_axis',(0.,-0.94284446121751,-0.333233134534162));
#53738=DIRECTION('center_axis',(0.,0.333233134534162,-0.94284446121751));
#53739=DIRECTION('ref_axis',(0.,0.94284446121751,0.333233134534162));
#53740=DIRECTION('',(0.,-0.333233134534162,0.94284446121751));
#53741=DIRECTION('center_axis',(0.,0.333233134534159,-0.942844461217511));
#53742=DIRECTION('ref_axis',(0.,-0.942844461217511,-0.333233134534159));
#53743=DIRECTION('center_axis',(0.,-0.333233134534162,0.94284446121751));
#53744=DIRECTION('ref_axis',(0.,-0.94284446121751,-0.333233134534162));
#53745=DIRECTION('center_axis',(0.,0.333233134534159,-0.942844461217511));
#53746=DIRECTION('ref_axis',(0.,-0.942844461217511,-0.333233134534159));
#53747=DIRECTION('',(0.,0.333233134534162,-0.94284446121751));
#53748=DIRECTION('center_axis',(0.,0.333233134534162,-0.94284446121751));
#53749=DIRECTION('ref_axis',(0.,-0.94284446121751,-0.333233134534162));
#53750=DIRECTION('center_axis',(0.,-0.333233134534162,0.94284446121751));
#53751=DIRECTION('ref_axis',(0.,-0.94284446121751,-0.333233134534162));
#53752=DIRECTION('center_axis',(0.,0.333233134534162,-0.94284446121751));
#53753=DIRECTION('ref_axis',(0.,0.94284446121751,0.333233134534162));
#53754=DIRECTION('',(0.,-0.333233134534162,0.94284446121751));
#53755=DIRECTION('center_axis',(0.,0.333233134534159,-0.942844461217511));
#53756=DIRECTION('ref_axis',(0.,-0.942844461217511,-0.333233134534159));
#53757=DIRECTION('center_axis',(0.,-0.333233134534162,0.94284446121751));
#53758=DIRECTION('ref_axis',(0.,-0.94284446121751,-0.333233134534162));
#53759=DIRECTION('center_axis',(0.,0.333233134534159,-0.942844461217511));
#53760=DIRECTION('ref_axis',(0.,-0.942844461217511,-0.333233134534159));
#53761=DIRECTION('',(0.,0.333233134534162,-0.94284446121751));
#53762=DIRECTION('center_axis',(0.,0.333233134534162,-0.94284446121751));
#53763=DIRECTION('ref_axis',(0.,-0.94284446121751,-0.333233134534162));
#53764=DIRECTION('center_axis',(0.,-0.333233134534162,0.94284446121751));
#53765=DIRECTION('ref_axis',(0.,-0.94284446121751,-0.333233134534162));
#53766=DIRECTION('center_axis',(0.,0.333233134534162,-0.94284446121751));
#53767=DIRECTION('ref_axis',(0.,0.94284446121751,0.333233134534162));
#53768=DIRECTION('',(0.,-0.333233134534162,0.94284446121751));
#53769=DIRECTION('center_axis',(0.,0.333233134534159,-0.942844461217511));
#53770=DIRECTION('ref_axis',(0.,-0.942844461217511,-0.333233134534159));
#53771=DIRECTION('center_axis',(0.,-0.333233134534162,0.94284446121751));
#53772=DIRECTION('ref_axis',(0.,-0.94284446121751,-0.333233134534162));
#53773=DIRECTION('center_axis',(0.,0.333233134534159,-0.942844461217511));
#53774=DIRECTION('ref_axis',(0.,-0.942844461217511,-0.333233134534159));
#53775=DIRECTION('',(0.,0.333233134534162,-0.94284446121751));
#53776=DIRECTION('center_axis',(0.,0.333233134534162,-0.94284446121751));
#53777=DIRECTION('ref_axis',(0.,-0.94284446121751,-0.333233134534162));
#53778=DIRECTION('center_axis',(0.,-0.333233134534162,0.94284446121751));
#53779=DIRECTION('ref_axis',(0.,-0.94284446121751,-0.333233134534162));
#53780=DIRECTION('center_axis',(0.,0.333233134534162,-0.94284446121751));
#53781=DIRECTION('ref_axis',(0.,0.94284446121751,0.333233134534162));
#53782=DIRECTION('',(0.,-0.333233134534162,0.94284446121751));
#53783=DIRECTION('center_axis',(0.,0.333233134534159,-0.942844461217511));
#53784=DIRECTION('ref_axis',(0.,-0.942844461217511,-0.333233134534159));
#53785=DIRECTION('center_axis',(0.,-0.333233134534162,0.94284446121751));
#53786=DIRECTION('ref_axis',(0.,-0.94284446121751,-0.333233134534162));
#53787=DIRECTION('center_axis',(0.,0.333233134534159,-0.942844461217511));
#53788=DIRECTION('ref_axis',(0.,-0.942844461217511,-0.333233134534159));
#53789=DIRECTION('',(0.,0.333233134534162,-0.94284446121751));
#53790=DIRECTION('center_axis',(0.,-0.333233134534162,0.94284446121751));
#53791=DIRECTION('ref_axis',(0.,-0.94284446121751,-0.333233134534162));
#53792=DIRECTION('center_axis',(0.,-0.333233134534162,0.94284446121751));
#53793=DIRECTION('ref_axis',(0.,-0.94284446121751,-0.333233134534162));
#53794=DIRECTION('center_axis',(0.,0.333233134534162,-0.94284446121751));
#53795=DIRECTION('ref_axis',(0.,0.94284446121751,0.333233134534162));
#53796=DIRECTION('',(0.,-0.333233134534162,0.94284446121751));
#53797=DIRECTION('center_axis',(0.,0.333233134534159,-0.942844461217511));
#53798=DIRECTION('ref_axis',(0.,-0.942844461217511,-0.333233134534159));
#53799=DIRECTION('center_axis',(0.,-0.333233134534162,0.94284446121751));
#53800=DIRECTION('ref_axis',(0.,-0.94284446121751,-0.333233134534161));
#53801=DIRECTION('center_axis',(0.,0.333233134534159,-0.942844461217511));
#53802=DIRECTION('ref_axis',(0.,-0.942844461217511,-0.333233134534159));
#53803=DIRECTION('',(0.,0.333233134534162,-0.94284446121751));
#53804=DIRECTION('center_axis',(0.,0.333233134534162,-0.94284446121751));
#53805=DIRECTION('ref_axis',(0.,-0.94284446121751,-0.333233134534162));
#53806=DIRECTION('center_axis',(0.,-0.333233134534162,0.94284446121751));
#53807=DIRECTION('ref_axis',(0.,-0.94284446121751,-0.333233134534162));
#53808=DIRECTION('center_axis',(0.,0.333233134534162,-0.94284446121751));
#53809=DIRECTION('ref_axis',(0.,0.94284446121751,0.333233134534162));
#53810=DIRECTION('',(0.,-0.333233134534162,0.94284446121751));
#53811=DIRECTION('center_axis',(0.,0.333233134534159,-0.942844461217511));
#53812=DIRECTION('ref_axis',(0.,-0.942844461217511,-0.333233134534159));
#53813=DIRECTION('center_axis',(0.,-0.333233134534162,0.94284446121751));
#53814=DIRECTION('ref_axis',(0.,-0.94284446121751,-0.333233134534162));
#53815=DIRECTION('center_axis',(0.,0.333233134534159,-0.942844461217511));
#53816=DIRECTION('ref_axis',(0.,-0.942844461217511,-0.333233134534159));
#53817=DIRECTION('',(0.,0.333233134534162,-0.94284446121751));
#53818=DIRECTION('center_axis',(0.,0.333233134534162,-0.94284446121751));
#53819=DIRECTION('ref_axis',(0.,-0.94284446121751,-0.333233134534162));
#53820=DIRECTION('center_axis',(0.,-0.333233134534162,0.94284446121751));
#53821=DIRECTION('ref_axis',(0.,-0.94284446121751,-0.333233134534161));
#53822=DIRECTION('center_axis',(0.,0.333233134534162,-0.94284446121751));
#53823=DIRECTION('ref_axis',(0.,0.94284446121751,0.333233134534162));
#53824=DIRECTION('',(0.,-0.333233134534162,0.94284446121751));
#53825=DIRECTION('center_axis',(0.,0.333233134534159,-0.942844461217511));
#53826=DIRECTION('ref_axis',(0.,-0.942844461217511,-0.333233134534159));
#53827=DIRECTION('center_axis',(0.,-0.333233134534162,0.94284446121751));
#53828=DIRECTION('ref_axis',(0.,-0.94284446121751,-0.333233134534162));
#53829=DIRECTION('center_axis',(0.,0.333233134534159,-0.942844461217511));
#53830=DIRECTION('ref_axis',(0.,-0.942844461217511,-0.333233134534159));
#53831=DIRECTION('',(0.,0.333233134534162,-0.94284446121751));
#53832=DIRECTION('center_axis',(0.,0.333233134534162,-0.94284446121751));
#53833=DIRECTION('ref_axis',(0.,-0.94284446121751,-0.333233134534162));
#53834=DIRECTION('center_axis',(0.,-0.333233134534162,0.94284446121751));
#53835=DIRECTION('ref_axis',(0.,-0.94284446121751,-0.333233134534162));
#53836=DIRECTION('center_axis',(0.,0.333233134534162,-0.94284446121751));
#53837=DIRECTION('ref_axis',(0.,0.94284446121751,0.333233134534162));
#53838=DIRECTION('',(0.,-0.333233134534162,0.94284446121751));
#53839=DIRECTION('center_axis',(0.,0.333233134534159,-0.942844461217511));
#53840=DIRECTION('ref_axis',(0.,-0.942844461217511,-0.333233134534159));
#53841=DIRECTION('center_axis',(0.,-0.333233134534162,0.94284446121751));
#53842=DIRECTION('ref_axis',(0.,-0.94284446121751,-0.333233134534162));
#53843=DIRECTION('center_axis',(0.,0.333233134534159,-0.942844461217511));
#53844=DIRECTION('ref_axis',(0.,-0.942844461217511,-0.333233134534159));
#53845=DIRECTION('',(0.,0.333233134534162,-0.94284446121751));
#53846=DIRECTION('center_axis',(0.,0.333233134534162,-0.94284446121751));
#53847=DIRECTION('ref_axis',(0.,-0.94284446121751,-0.333233134534162));
#53848=DIRECTION('center_axis',(0.,-0.333233134534162,0.94284446121751));
#53849=DIRECTION('ref_axis',(0.,-0.94284446121751,-0.333233134534162));
#53850=DIRECTION('center_axis',(0.,0.333233134534162,-0.94284446121751));
#53851=DIRECTION('ref_axis',(0.,0.94284446121751,0.333233134534162));
#53852=DIRECTION('',(0.,-0.333233134534162,0.94284446121751));
#53853=DIRECTION('center_axis',(0.,0.333233134534159,-0.942844461217511));
#53854=DIRECTION('ref_axis',(0.,-0.942844461217511,-0.333233134534159));
#53855=DIRECTION('center_axis',(0.,-0.333233134534162,0.94284446121751));
#53856=DIRECTION('ref_axis',(0.,-0.94284446121751,-0.333233134534162));
#53857=DIRECTION('center_axis',(0.,0.333233134534159,-0.942844461217511));
#53858=DIRECTION('ref_axis',(0.,-0.942844461217511,-0.333233134534159));
#53859=DIRECTION('',(0.,0.333233134534162,-0.94284446121751));
#53860=DIRECTION('center_axis',(0.,0.333233134534162,-0.94284446121751));
#53861=DIRECTION('ref_axis',(0.,-0.94284446121751,-0.333233134534162));
#53862=DIRECTION('center_axis',(0.,-0.333233134534162,0.94284446121751));
#53863=DIRECTION('ref_axis',(0.,-0.94284446121751,-0.333233134534162));
#53864=DIRECTION('center_axis',(0.,0.333233134534162,-0.94284446121751));
#53865=DIRECTION('ref_axis',(0.,0.94284446121751,0.333233134534162));
#53866=DIRECTION('',(0.,-0.333233134534162,0.94284446121751));
#53867=DIRECTION('center_axis',(0.,0.333233134534159,-0.942844461217511));
#53868=DIRECTION('ref_axis',(0.,-0.942844461217511,-0.333233134534159));
#53869=DIRECTION('center_axis',(0.,-0.333233134534162,0.94284446121751));
#53870=DIRECTION('ref_axis',(0.,-0.94284446121751,-0.333233134534162));
#53871=DIRECTION('center_axis',(0.,0.333233134534159,-0.942844461217511));
#53872=DIRECTION('ref_axis',(0.,-0.942844461217511,-0.333233134534159));
#53873=DIRECTION('',(0.,0.333233134534162,-0.94284446121751));
#53874=DIRECTION('center_axis',(0.,0.333233134534162,-0.94284446121751));
#53875=DIRECTION('ref_axis',(0.,-0.94284446121751,-0.333233134534162));
#53876=DIRECTION('center_axis',(0.,-0.333233134534162,0.94284446121751));
#53877=DIRECTION('ref_axis',(0.,-0.94284446121751,-0.333233134534162));
#53878=DIRECTION('center_axis',(0.,0.333233134534162,-0.94284446121751));
#53879=DIRECTION('ref_axis',(0.,0.94284446121751,0.333233134534162));
#53880=DIRECTION('',(0.,-0.333233134534162,0.94284446121751));
#53881=DIRECTION('center_axis',(0.,0.333233134534159,-0.942844461217511));
#53882=DIRECTION('ref_axis',(0.,-0.942844461217511,-0.333233134534159));
#53883=DIRECTION('center_axis',(0.,-0.333233134534162,0.94284446121751));
#53884=DIRECTION('ref_axis',(0.,-0.94284446121751,-0.333233134534162));
#53885=DIRECTION('center_axis',(0.,0.333233134534159,-0.942844461217511));
#53886=DIRECTION('ref_axis',(0.,-0.942844461217511,-0.333233134534159));
#53887=DIRECTION('',(0.,0.333233134534162,-0.94284446121751));
#53888=DIRECTION('center_axis',(0.,0.333233134534162,-0.94284446121751));
#53889=DIRECTION('ref_axis',(0.,-0.94284446121751,-0.333233134534162));
#53890=DIRECTION('center_axis',(0.,-0.333233134534162,0.94284446121751));
#53891=DIRECTION('ref_axis',(0.,-0.94284446121751,-0.333233134534162));
#53892=DIRECTION('center_axis',(0.,0.333233134534162,-0.94284446121751));
#53893=DIRECTION('ref_axis',(0.,0.94284446121751,0.333233134534162));
#53894=DIRECTION('',(0.,-0.333233134534162,0.94284446121751));
#53895=DIRECTION('center_axis',(0.,0.333233134534159,-0.942844461217511));
#53896=DIRECTION('ref_axis',(0.,-0.942844461217511,-0.333233134534159));
#53897=DIRECTION('center_axis',(0.,-0.333233134534162,0.94284446121751));
#53898=DIRECTION('ref_axis',(0.,-0.94284446121751,-0.333233134534162));
#53899=DIRECTION('center_axis',(0.,0.333233134534159,-0.942844461217511));
#53900=DIRECTION('ref_axis',(0.,-0.942844461217511,-0.333233134534159));
#53901=DIRECTION('',(0.,0.333233134534162,-0.94284446121751));
#53902=DIRECTION('center_axis',(0.,-0.333233134534162,0.94284446121751));
#53903=DIRECTION('ref_axis',(0.,-0.94284446121751,-0.333233134534162));
#53904=DIRECTION('center_axis',(0.,-0.333233134534162,0.94284446121751));
#53905=DIRECTION('ref_axis',(0.,-0.94284446121751,-0.333233134534162));
#53906=DIRECTION('center_axis',(0.,0.333233134534162,-0.94284446121751));
#53907=DIRECTION('ref_axis',(0.,0.94284446121751,0.333233134534162));
#53908=DIRECTION('',(0.,-0.333233134534162,0.94284446121751));
#53909=DIRECTION('center_axis',(0.,0.333233134534159,-0.942844461217511));
#53910=DIRECTION('ref_axis',(0.,-0.942844461217511,-0.333233134534159));
#53911=DIRECTION('center_axis',(0.,-0.333233134534162,0.94284446121751));
#53912=DIRECTION('ref_axis',(0.,-0.94284446121751,-0.333233134534162));
#53913=DIRECTION('center_axis',(0.,0.333233134534159,-0.942844461217511));
#53914=DIRECTION('ref_axis',(0.,-0.942844461217511,-0.333233134534159));
#53915=DIRECTION('',(0.,0.333233134534162,-0.94284446121751));
#53916=DIRECTION('center_axis',(0.,0.333233134534162,-0.94284446121751));
#53917=DIRECTION('ref_axis',(0.,-0.94284446121751,-0.333233134534162));
#53918=DIRECTION('center_axis',(0.,-0.333233134534162,0.94284446121751));
#53919=DIRECTION('ref_axis',(0.,-0.94284446121751,-0.333233134534162));
#53920=DIRECTION('center_axis',(0.,0.333233134534162,-0.94284446121751));
#53921=DIRECTION('ref_axis',(0.,0.94284446121751,0.333233134534162));
#53922=DIRECTION('',(0.,-0.333233134534162,0.94284446121751));
#53923=DIRECTION('center_axis',(0.,0.333233134534159,-0.942844461217511));
#53924=DIRECTION('ref_axis',(0.,-0.942844461217511,-0.333233134534159));
#53925=DIRECTION('center_axis',(0.,-0.333233134534162,0.94284446121751));
#53926=DIRECTION('ref_axis',(0.,-0.94284446121751,-0.333233134534162));
#53927=DIRECTION('center_axis',(0.,0.333233134534159,-0.942844461217511));
#53928=DIRECTION('ref_axis',(0.,-0.942844461217511,-0.333233134534159));
#53929=DIRECTION('',(0.,0.333233134534162,-0.94284446121751));
#53930=DIRECTION('center_axis',(0.,0.333233134534162,-0.94284446121751));
#53931=DIRECTION('ref_axis',(0.,-0.94284446121751,-0.333233134534162));
#53932=DIRECTION('center_axis',(0.,-0.333233134534162,0.94284446121751));
#53933=DIRECTION('ref_axis',(0.,-0.94284446121751,-0.333233134534162));
#53934=DIRECTION('center_axis',(0.,0.333233134534162,-0.94284446121751));
#53935=DIRECTION('ref_axis',(0.,0.94284446121751,0.333233134534162));
#53936=DIRECTION('',(0.,-0.333233134534162,0.94284446121751));
#53937=DIRECTION('center_axis',(0.,0.333233134534159,-0.942844461217511));
#53938=DIRECTION('ref_axis',(0.,-0.942844461217511,-0.333233134534159));
#53939=DIRECTION('center_axis',(0.,-0.333233134534162,0.94284446121751));
#53940=DIRECTION('ref_axis',(0.,-0.94284446121751,-0.333233134534162));
#53941=DIRECTION('center_axis',(0.,0.333233134534159,-0.942844461217511));
#53942=DIRECTION('ref_axis',(0.,-0.942844461217511,-0.333233134534159));
#53943=DIRECTION('',(0.,0.333233134534162,-0.94284446121751));
#53944=DIRECTION('center_axis',(0.,0.333233134534162,-0.94284446121751));
#53945=DIRECTION('ref_axis',(0.,-0.94284446121751,-0.333233134534162));
#53946=DIRECTION('center_axis',(0.,-0.333233134534162,0.94284446121751));
#53947=DIRECTION('ref_axis',(0.,-0.94284446121751,-0.333233134534162));
#53948=DIRECTION('center_axis',(0.,0.333233134534162,-0.94284446121751));
#53949=DIRECTION('ref_axis',(0.,0.94284446121751,0.333233134534162));
#53950=DIRECTION('',(0.,-0.333233134534162,0.94284446121751));
#53951=DIRECTION('center_axis',(0.,0.333233134534159,-0.942844461217511));
#53952=DIRECTION('ref_axis',(0.,-0.942844461217511,-0.333233134534159));
#53953=DIRECTION('center_axis',(0.,-0.333233134534162,0.94284446121751));
#53954=DIRECTION('ref_axis',(0.,-0.94284446121751,-0.333233134534162));
#53955=DIRECTION('center_axis',(0.,0.333233134534159,-0.942844461217511));
#53956=DIRECTION('ref_axis',(0.,-0.942844461217511,-0.333233134534159));
#53957=DIRECTION('',(0.,0.333233134534162,-0.94284446121751));
#53958=DIRECTION('center_axis',(0.,0.333233134534162,-0.94284446121751));
#53959=DIRECTION('ref_axis',(0.,-0.94284446121751,-0.333233134534162));
#53960=DIRECTION('center_axis',(0.,-0.333233134534162,0.94284446121751));
#53961=DIRECTION('ref_axis',(0.,-0.94284446121751,-0.333233134534162));
#53962=DIRECTION('center_axis',(0.,0.333233134534162,-0.94284446121751));
#53963=DIRECTION('ref_axis',(0.,0.94284446121751,0.333233134534162));
#53964=DIRECTION('',(0.,-0.333233134534162,0.94284446121751));
#53965=DIRECTION('center_axis',(0.,0.333233134534159,-0.942844461217511));
#53966=DIRECTION('ref_axis',(0.,-0.942844461217511,-0.333233134534159));
#53967=DIRECTION('center_axis',(0.,-0.333233134534162,0.94284446121751));
#53968=DIRECTION('ref_axis',(0.,-0.94284446121751,-0.333233134534162));
#53969=DIRECTION('center_axis',(0.,0.333233134534159,-0.942844461217511));
#53970=DIRECTION('ref_axis',(0.,-0.942844461217511,-0.333233134534159));
#53971=DIRECTION('',(0.,0.333233134534162,-0.94284446121751));
#53972=DIRECTION('center_axis',(0.,0.333233134534162,-0.94284446121751));
#53973=DIRECTION('ref_axis',(0.,-0.94284446121751,-0.333233134534162));
#53974=DIRECTION('center_axis',(0.,-0.333233134534162,0.94284446121751));
#53975=DIRECTION('ref_axis',(0.,-0.94284446121751,-0.333233134534162));
#53976=DIRECTION('center_axis',(0.,0.333233134534162,-0.94284446121751));
#53977=DIRECTION('ref_axis',(0.,0.94284446121751,0.333233134534162));
#53978=DIRECTION('',(0.,-0.333233134534162,0.94284446121751));
#53979=DIRECTION('center_axis',(0.,0.333233134534159,-0.942844461217511));
#53980=DIRECTION('ref_axis',(0.,-0.942844461217511,-0.333233134534159));
#53981=DIRECTION('center_axis',(0.,-0.333233134534162,0.94284446121751));
#53982=DIRECTION('ref_axis',(0.,-0.94284446121751,-0.333233134534162));
#53983=DIRECTION('center_axis',(0.,0.333233134534159,-0.942844461217511));
#53984=DIRECTION('ref_axis',(0.,-0.942844461217511,-0.333233134534159));
#53985=DIRECTION('',(0.,0.333233134534162,-0.94284446121751));
#53986=DIRECTION('center_axis',(0.,0.333233134534162,-0.94284446121751));
#53987=DIRECTION('ref_axis',(0.,-0.94284446121751,-0.333233134534162));
#53988=DIRECTION('center_axis',(0.,-0.333233134534162,0.94284446121751));
#53989=DIRECTION('ref_axis',(0.,-0.94284446121751,-0.333233134534162));
#53990=DIRECTION('center_axis',(0.,0.333233134534162,-0.94284446121751));
#53991=DIRECTION('ref_axis',(0.,0.94284446121751,0.333233134534162));
#53992=DIRECTION('',(0.,-0.333233134534162,0.94284446121751));
#53993=DIRECTION('center_axis',(0.,0.333233134534159,-0.942844461217511));
#53994=DIRECTION('ref_axis',(0.,-0.942844461217511,-0.333233134534159));
#53995=DIRECTION('center_axis',(0.,-0.333233134534162,0.94284446121751));
#53996=DIRECTION('ref_axis',(0.,-0.94284446121751,-0.333233134534161));
#53997=DIRECTION('center_axis',(0.,0.333233134534159,-0.942844461217511));
#53998=DIRECTION('ref_axis',(0.,-0.942844461217511,-0.333233134534159));
#53999=DIRECTION('',(0.,0.333233134534162,-0.94284446121751));
#54000=DIRECTION('center_axis',(0.,0.333233134534162,-0.94284446121751));
#54001=DIRECTION('ref_axis',(0.,-0.94284446121751,-0.333233134534162));
#54002=DIRECTION('center_axis',(0.,-0.333233134534162,0.94284446121751));
#54003=DIRECTION('ref_axis',(0.,-0.94284446121751,-0.333233134534162));
#54004=DIRECTION('center_axis',(0.,0.333233134534162,-0.94284446121751));
#54005=DIRECTION('ref_axis',(0.,0.94284446121751,0.333233134534162));
#54006=DIRECTION('',(0.,-0.333233134534162,0.94284446121751));
#54007=DIRECTION('center_axis',(0.,0.333233134534159,-0.942844461217511));
#54008=DIRECTION('ref_axis',(0.,-0.942844461217511,-0.333233134534159));
#54009=DIRECTION('center_axis',(0.,-0.333233134534162,0.94284446121751));
#54010=DIRECTION('ref_axis',(0.,-0.94284446121751,-0.333233134534162));
#54011=DIRECTION('center_axis',(0.,0.333233134534159,-0.942844461217511));
#54012=DIRECTION('ref_axis',(0.,-0.942844461217511,-0.333233134534159));
#54013=DIRECTION('',(0.,0.333233134534162,-0.94284446121751));
#54014=DIRECTION('center_axis',(0.,0.333233134534162,-0.94284446121751));
#54015=DIRECTION('ref_axis',(0.,-0.94284446121751,-0.333233134534162));
#54016=DIRECTION('center_axis',(0.,-0.333233134534162,0.94284446121751));
#54017=DIRECTION('ref_axis',(0.,-0.94284446121751,-0.333233134534162));
#54018=DIRECTION('center_axis',(0.,0.333233134534162,-0.94284446121751));
#54019=DIRECTION('ref_axis',(0.,0.94284446121751,0.333233134534162));
#54020=DIRECTION('',(0.,-0.333233134534162,0.94284446121751));
#54021=DIRECTION('center_axis',(0.,0.333233134534159,-0.942844461217511));
#54022=DIRECTION('ref_axis',(0.,-0.942844461217511,-0.333233134534159));
#54023=DIRECTION('center_axis',(0.,-0.333233134534162,0.94284446121751));
#54024=DIRECTION('ref_axis',(0.,-0.94284446121751,-0.333233134534162));
#54025=DIRECTION('center_axis',(0.,0.333233134534159,-0.942844461217511));
#54026=DIRECTION('ref_axis',(0.,-0.942844461217511,-0.333233134534159));
#54027=DIRECTION('',(0.,0.333233134534162,-0.94284446121751));
#54028=DIRECTION('center_axis',(0.,-0.333233134534162,0.94284446121751));
#54029=DIRECTION('ref_axis',(0.,-0.94284446121751,-0.333233134534162));
#54030=DIRECTION('center_axis',(0.,-0.333233134534162,0.94284446121751));
#54031=DIRECTION('ref_axis',(0.,-0.94284446121751,-0.333233134534162));
#54032=DIRECTION('center_axis',(0.,0.333233134534162,-0.94284446121751));
#54033=DIRECTION('ref_axis',(0.,0.94284446121751,0.333233134534162));
#54034=DIRECTION('',(0.,-0.333233134534162,0.94284446121751));
#54035=DIRECTION('center_axis',(0.,0.333233134534159,-0.942844461217511));
#54036=DIRECTION('ref_axis',(0.,-0.942844461217511,-0.333233134534159));
#54037=DIRECTION('center_axis',(0.,-0.333233134534162,0.94284446121751));
#54038=DIRECTION('ref_axis',(0.,-0.94284446121751,-0.333233134534161));
#54039=DIRECTION('center_axis',(0.,0.333233134534159,-0.942844461217511));
#54040=DIRECTION('ref_axis',(0.,-0.942844461217511,-0.333233134534159));
#54041=DIRECTION('',(0.,0.333233134534162,-0.94284446121751));
#54042=DIRECTION('center_axis',(0.,0.333233134534162,-0.94284446121751));
#54043=DIRECTION('ref_axis',(0.,-0.94284446121751,-0.333233134534162));
#54044=DIRECTION('center_axis',(0.,-0.333233134534162,0.94284446121751));
#54045=DIRECTION('ref_axis',(0.,-0.94284446121751,-0.333233134534162));
#54046=DIRECTION('center_axis',(0.,0.333233134534162,-0.94284446121751));
#54047=DIRECTION('ref_axis',(0.,0.94284446121751,0.333233134534162));
#54048=DIRECTION('',(0.,-0.333233134534162,0.94284446121751));
#54049=DIRECTION('center_axis',(0.,0.333233134534159,-0.942844461217511));
#54050=DIRECTION('ref_axis',(0.,-0.942844461217511,-0.333233134534159));
#54051=DIRECTION('center_axis',(0.,-0.333233134534162,0.94284446121751));
#54052=DIRECTION('ref_axis',(0.,-0.94284446121751,-0.333233134534162));
#54053=DIRECTION('center_axis',(0.,0.333233134534159,-0.942844461217511));
#54054=DIRECTION('ref_axis',(0.,-0.942844461217511,-0.333233134534159));
#54055=DIRECTION('',(0.,0.333233134534162,-0.94284446121751));
#54056=DIRECTION('center_axis',(0.,0.333233134534162,-0.94284446121751));
#54057=DIRECTION('ref_axis',(0.,-0.94284446121751,-0.333233134534162));
#54058=DIRECTION('center_axis',(0.,-0.333233134534162,0.94284446121751));
#54059=DIRECTION('ref_axis',(0.,-0.94284446121751,-0.333233134534162));
#54060=DIRECTION('center_axis',(0.,0.333233134534162,-0.94284446121751));
#54061=DIRECTION('ref_axis',(0.,0.94284446121751,0.333233134534162));
#54062=DIRECTION('',(0.,-0.333233134534162,0.94284446121751));
#54063=DIRECTION('center_axis',(0.,0.333233134534159,-0.942844461217511));
#54064=DIRECTION('ref_axis',(0.,-0.942844461217511,-0.333233134534159));
#54065=DIRECTION('center_axis',(0.,-0.333233134534162,0.94284446121751));
#54066=DIRECTION('ref_axis',(0.,-0.94284446121751,-0.333233134534161));
#54067=DIRECTION('center_axis',(0.,0.333233134534159,-0.942844461217511));
#54068=DIRECTION('ref_axis',(0.,-0.942844461217511,-0.333233134534159));
#54069=DIRECTION('',(0.,0.333233134534162,-0.94284446121751));
#54070=DIRECTION('center_axis',(0.,0.333233134534162,-0.94284446121751));
#54071=DIRECTION('ref_axis',(0.,-0.94284446121751,-0.333233134534162));
#54072=DIRECTION('center_axis',(0.,-0.333233134534162,0.94284446121751));
#54073=DIRECTION('ref_axis',(0.,-0.94284446121751,-0.333233134534162));
#54074=DIRECTION('center_axis',(0.,0.333233134534162,-0.94284446121751));
#54075=DIRECTION('ref_axis',(0.,0.94284446121751,0.333233134534162));
#54076=DIRECTION('',(0.,-0.333233134534162,0.94284446121751));
#54077=DIRECTION('center_axis',(0.,0.333233134534159,-0.942844461217511));
#54078=DIRECTION('ref_axis',(0.,-0.942844461217511,-0.333233134534159));
#54079=DIRECTION('center_axis',(0.,-0.333233134534162,0.94284446121751));
#54080=DIRECTION('ref_axis',(0.,-0.94284446121751,-0.333233134534162));
#54081=DIRECTION('center_axis',(0.,0.333233134534159,-0.942844461217511));
#54082=DIRECTION('ref_axis',(0.,-0.942844461217511,-0.333233134534159));
#54083=DIRECTION('',(0.,0.333233134534162,-0.94284446121751));
#54084=DIRECTION('center_axis',(0.,0.333233134534162,-0.94284446121751));
#54085=DIRECTION('ref_axis',(0.,-0.94284446121751,-0.333233134534162));
#54086=DIRECTION('center_axis',(0.,-0.333233134534162,0.94284446121751));
#54087=DIRECTION('ref_axis',(0.,-0.94284446121751,-0.333233134534162));
#54088=DIRECTION('center_axis',(0.,0.333233134534162,-0.94284446121751));
#54089=DIRECTION('ref_axis',(0.,0.94284446121751,0.333233134534162));
#54090=DIRECTION('',(0.,-0.333233134534162,0.94284446121751));
#54091=DIRECTION('center_axis',(0.,0.333233134534159,-0.942844461217511));
#54092=DIRECTION('ref_axis',(0.,-0.942844461217511,-0.333233134534159));
#54093=DIRECTION('center_axis',(0.,-0.333233134534162,0.94284446121751));
#54094=DIRECTION('ref_axis',(0.,-0.94284446121751,-0.333233134534162));
#54095=DIRECTION('center_axis',(0.,0.333233134534159,-0.942844461217511));
#54096=DIRECTION('ref_axis',(0.,-0.942844461217511,-0.333233134534159));
#54097=DIRECTION('',(0.,0.333233134534162,-0.94284446121751));
#54098=DIRECTION('center_axis',(0.,0.333233134534162,-0.94284446121751));
#54099=DIRECTION('ref_axis',(0.,-0.94284446121751,-0.333233134534162));
#54100=DIRECTION('center_axis',(0.,-0.333233134534162,0.94284446121751));
#54101=DIRECTION('ref_axis',(0.,-0.94284446121751,-0.333233134534162));
#54102=DIRECTION('center_axis',(0.,0.333233134534162,-0.94284446121751));
#54103=DIRECTION('ref_axis',(0.,0.94284446121751,0.333233134534162));
#54104=DIRECTION('',(0.,-0.333233134534162,0.94284446121751));
#54105=DIRECTION('center_axis',(0.,0.333233134534159,-0.942844461217511));
#54106=DIRECTION('ref_axis',(0.,-0.942844461217511,-0.333233134534159));
#54107=DIRECTION('center_axis',(0.,-0.333233134534162,0.94284446121751));
#54108=DIRECTION('ref_axis',(0.,-0.94284446121751,-0.333233134534162));
#54109=DIRECTION('center_axis',(0.,0.333233134534159,-0.942844461217511));
#54110=DIRECTION('ref_axis',(0.,-0.942844461217511,-0.333233134534159));
#54111=DIRECTION('',(0.,0.333233134534162,-0.94284446121751));
#54112=DIRECTION('center_axis',(0.,0.333233134534162,-0.94284446121751));
#54113=DIRECTION('ref_axis',(0.,-0.94284446121751,-0.333233134534162));
#54114=DIRECTION('center_axis',(0.,-0.333233134534162,0.94284446121751));
#54115=DIRECTION('ref_axis',(0.,-0.94284446121751,-0.333233134534162));
#54116=DIRECTION('center_axis',(0.,0.333233134534162,-0.94284446121751));
#54117=DIRECTION('ref_axis',(0.,0.94284446121751,0.333233134534162));
#54118=DIRECTION('',(0.,-0.333233134534162,0.94284446121751));
#54119=DIRECTION('center_axis',(0.,0.333233134534159,-0.942844461217511));
#54120=DIRECTION('ref_axis',(0.,-0.942844461217511,-0.333233134534159));
#54121=DIRECTION('center_axis',(0.,-0.333233134534162,0.94284446121751));
#54122=DIRECTION('ref_axis',(0.,-0.94284446121751,-0.333233134534162));
#54123=DIRECTION('center_axis',(0.,0.333233134534159,-0.942844461217511));
#54124=DIRECTION('ref_axis',(0.,-0.942844461217511,-0.333233134534159));
#54125=DIRECTION('',(0.,0.333233134534162,-0.94284446121751));
#54126=DIRECTION('center_axis',(0.,0.333233134534162,-0.94284446121751));
#54127=DIRECTION('ref_axis',(0.,-0.94284446121751,-0.333233134534162));
#54128=DIRECTION('center_axis',(0.,-0.333233134534162,0.94284446121751));
#54129=DIRECTION('ref_axis',(0.,-0.94284446121751,-0.333233134534162));
#54130=DIRECTION('center_axis',(0.,0.333233134534162,-0.94284446121751));
#54131=DIRECTION('ref_axis',(0.,0.94284446121751,0.333233134534162));
#54132=DIRECTION('',(0.,-0.333233134534162,0.94284446121751));
#54133=DIRECTION('center_axis',(0.,0.333233134534159,-0.942844461217511));
#54134=DIRECTION('ref_axis',(0.,-0.942844461217511,-0.333233134534159));
#54135=DIRECTION('center_axis',(0.,-0.333233134534162,0.94284446121751));
#54136=DIRECTION('ref_axis',(0.,-0.94284446121751,-0.333233134534162));
#54137=DIRECTION('center_axis',(0.,0.333233134534159,-0.942844461217511));
#54138=DIRECTION('ref_axis',(0.,-0.942844461217511,-0.333233134534159));
#54139=DIRECTION('',(0.,0.333233134534162,-0.94284446121751));
#54140=DIRECTION('center_axis',(0.,0.333233134534162,-0.94284446121751));
#54141=DIRECTION('ref_axis',(0.,-0.94284446121751,-0.333233134534162));
#54142=DIRECTION('center_axis',(0.,-0.333233134534162,0.94284446121751));
#54143=DIRECTION('ref_axis',(0.,-0.94284446121751,-0.333233134534162));
#54144=DIRECTION('center_axis',(0.,0.333233134534162,-0.94284446121751));
#54145=DIRECTION('ref_axis',(0.,0.94284446121751,0.333233134534162));
#54146=DIRECTION('',(0.,-0.333233134534162,0.94284446121751));
#54147=DIRECTION('center_axis',(0.,0.333233134534159,-0.942844461217511));
#54148=DIRECTION('ref_axis',(0.,-0.942844461217511,-0.333233134534159));
#54149=DIRECTION('center_axis',(0.,-0.333233134534162,0.94284446121751));
#54150=DIRECTION('ref_axis',(0.,-0.94284446121751,-0.333233134534162));
#54151=DIRECTION('center_axis',(0.,0.333233134534159,-0.942844461217511));
#54152=DIRECTION('ref_axis',(0.,-0.942844461217511,-0.333233134534159));
#54153=DIRECTION('',(0.,0.333233134534162,-0.94284446121751));
#54154=DIRECTION('center_axis',(0.,-0.333233134534162,0.94284446121751));
#54155=DIRECTION('ref_axis',(0.,-0.94284446121751,-0.333233134534162));
#54156=DIRECTION('center_axis',(0.,-0.333233134534162,0.94284446121751));
#54157=DIRECTION('ref_axis',(0.,-0.94284446121751,-0.333233134534162));
#54158=DIRECTION('center_axis',(0.,0.333233134534162,-0.94284446121751));
#54159=DIRECTION('ref_axis',(0.,0.94284446121751,0.333233134534162));
#54160=DIRECTION('',(0.,-0.333233134534162,0.94284446121751));
#54161=DIRECTION('center_axis',(0.,0.333233134534159,-0.942844461217511));
#54162=DIRECTION('ref_axis',(0.,-0.942844461217511,-0.333233134534159));
#54163=DIRECTION('center_axis',(0.,-0.333233134534162,0.94284446121751));
#54164=DIRECTION('ref_axis',(0.,-0.94284446121751,-0.333233134534161));
#54165=DIRECTION('center_axis',(0.,0.333233134534159,-0.942844461217511));
#54166=DIRECTION('ref_axis',(0.,-0.942844461217511,-0.333233134534159));
#54167=DIRECTION('',(0.,0.333233134534162,-0.94284446121751));
#54168=DIRECTION('center_axis',(0.,0.333233134534162,-0.94284446121751));
#54169=DIRECTION('ref_axis',(0.,-0.94284446121751,-0.333233134534162));
#54170=DIRECTION('center_axis',(0.,-0.333233134534162,0.94284446121751));
#54171=DIRECTION('ref_axis',(0.,-0.94284446121751,-0.333233134534162));
#54172=DIRECTION('center_axis',(0.,0.333233134534162,-0.94284446121751));
#54173=DIRECTION('ref_axis',(0.,0.94284446121751,0.333233134534162));
#54174=DIRECTION('',(0.,-0.333233134534162,0.94284446121751));
#54175=DIRECTION('center_axis',(0.,0.333233134534159,-0.942844461217511));
#54176=DIRECTION('ref_axis',(0.,-0.942844461217511,-0.333233134534159));
#54177=DIRECTION('center_axis',(0.,-0.333233134534162,0.94284446121751));
#54178=DIRECTION('ref_axis',(0.,-0.94284446121751,-0.333233134534162));
#54179=DIRECTION('center_axis',(0.,0.333233134534159,-0.942844461217511));
#54180=DIRECTION('ref_axis',(0.,-0.942844461217511,-0.333233134534159));
#54181=DIRECTION('',(0.,0.333233134534162,-0.94284446121751));
#54182=DIRECTION('center_axis',(0.,0.333233134534162,-0.94284446121751));
#54183=DIRECTION('ref_axis',(0.,-0.94284446121751,-0.333233134534162));
#54184=DIRECTION('center_axis',(0.,-0.333233134534162,0.94284446121751));
#54185=DIRECTION('ref_axis',(0.,-0.94284446121751,-0.333233134534162));
#54186=DIRECTION('center_axis',(0.,0.333233134534162,-0.94284446121751));
#54187=DIRECTION('ref_axis',(0.,0.94284446121751,0.333233134534162));
#54188=DIRECTION('',(0.,-0.333233134534162,0.94284446121751));
#54189=DIRECTION('center_axis',(0.,0.333233134534159,-0.942844461217511));
#54190=DIRECTION('ref_axis',(0.,-0.942844461217511,-0.333233134534159));
#54191=DIRECTION('center_axis',(0.,-0.333233134534162,0.94284446121751));
#54192=DIRECTION('ref_axis',(0.,-0.94284446121751,-0.333233134534162));
#54193=DIRECTION('center_axis',(0.,0.333233134534159,-0.942844461217511));
#54194=DIRECTION('ref_axis',(0.,-0.942844461217511,-0.333233134534159));
#54195=DIRECTION('',(0.,0.333233134534162,-0.94284446121751));
#54196=DIRECTION('center_axis',(0.,0.333233134534162,-0.94284446121751));
#54197=DIRECTION('ref_axis',(0.,-0.94284446121751,-0.333233134534162));
#54198=DIRECTION('center_axis',(0.,-0.333233134534162,0.94284446121751));
#54199=DIRECTION('ref_axis',(0.,-0.94284446121751,-0.333233134534162));
#54200=DIRECTION('center_axis',(0.,0.333233134534162,-0.94284446121751));
#54201=DIRECTION('ref_axis',(0.,0.94284446121751,0.333233134534162));
#54202=DIRECTION('',(0.,-0.333233134534162,0.94284446121751));
#54203=DIRECTION('center_axis',(0.,0.333233134534159,-0.942844461217511));
#54204=DIRECTION('ref_axis',(0.,-0.942844461217511,-0.333233134534159));
#54205=DIRECTION('center_axis',(0.,-0.333233134534162,0.94284446121751));
#54206=DIRECTION('ref_axis',(0.,-0.94284446121751,-0.333233134534162));
#54207=DIRECTION('center_axis',(0.,0.333233134534159,-0.942844461217511));
#54208=DIRECTION('ref_axis',(0.,-0.942844461217511,-0.333233134534159));
#54209=DIRECTION('',(0.,0.333233134534162,-0.94284446121751));
#54210=DIRECTION('center_axis',(0.,0.333233134534162,-0.94284446121751));
#54211=DIRECTION('ref_axis',(0.,-0.94284446121751,-0.333233134534162));
#54212=DIRECTION('center_axis',(0.,-0.333233134534162,0.94284446121751));
#54213=DIRECTION('ref_axis',(0.,-0.94284446121751,-0.333233134534162));
#54214=DIRECTION('center_axis',(0.,0.333233134534162,-0.94284446121751));
#54215=DIRECTION('ref_axis',(0.,0.94284446121751,0.333233134534162));
#54216=DIRECTION('',(0.,-0.333233134534162,0.94284446121751));
#54217=DIRECTION('center_axis',(0.,0.333233134534159,-0.942844461217511));
#54218=DIRECTION('ref_axis',(0.,-0.942844461217511,-0.333233134534159));
#54219=DIRECTION('center_axis',(0.,-0.333233134534162,0.94284446121751));
#54220=DIRECTION('ref_axis',(0.,-0.94284446121751,-0.333233134534162));
#54221=DIRECTION('center_axis',(0.,0.333233134534159,-0.942844461217511));
#54222=DIRECTION('ref_axis',(0.,-0.942844461217511,-0.333233134534159));
#54223=DIRECTION('',(0.,0.333233134534162,-0.94284446121751));
#54224=DIRECTION('center_axis',(0.,0.333233134534162,-0.94284446121751));
#54225=DIRECTION('ref_axis',(0.,-0.94284446121751,-0.333233134534162));
#54226=DIRECTION('center_axis',(0.,-0.333233134534162,0.94284446121751));
#54227=DIRECTION('ref_axis',(0.,-0.94284446121751,-0.333233134534162));
#54228=DIRECTION('center_axis',(0.,0.333233134534162,-0.94284446121751));
#54229=DIRECTION('ref_axis',(0.,0.94284446121751,0.333233134534162));
#54230=DIRECTION('',(0.,-0.333233134534162,0.94284446121751));
#54231=DIRECTION('center_axis',(0.,0.333233134534159,-0.942844461217511));
#54232=DIRECTION('ref_axis',(0.,-0.942844461217511,-0.333233134534159));
#54233=DIRECTION('center_axis',(0.,-0.333233134534162,0.94284446121751));
#54234=DIRECTION('ref_axis',(0.,-0.94284446121751,-0.333233134534162));
#54235=DIRECTION('center_axis',(0.,0.333233134534159,-0.942844461217511));
#54236=DIRECTION('ref_axis',(0.,-0.942844461217511,-0.333233134534159));
#54237=DIRECTION('',(0.,0.333233134534162,-0.94284446121751));
#54238=DIRECTION('center_axis',(0.,0.333233134534162,-0.94284446121751));
#54239=DIRECTION('ref_axis',(0.,-0.94284446121751,-0.333233134534162));
#54240=DIRECTION('center_axis',(0.,-0.333233134534162,0.94284446121751));
#54241=DIRECTION('ref_axis',(0.,-0.94284446121751,-0.333233134534162));
#54242=DIRECTION('center_axis',(0.,0.333233134534162,-0.94284446121751));
#54243=DIRECTION('ref_axis',(0.,0.94284446121751,0.333233134534162));
#54244=DIRECTION('',(0.,-0.333233134534162,0.94284446121751));
#54245=DIRECTION('center_axis',(0.,0.333233134534159,-0.942844461217511));
#54246=DIRECTION('ref_axis',(0.,-0.942844461217511,-0.333233134534159));
#54247=DIRECTION('center_axis',(0.,-0.333233134534162,0.94284446121751));
#54248=DIRECTION('ref_axis',(0.,-0.94284446121751,-0.333233134534162));
#54249=DIRECTION('center_axis',(0.,0.333233134534159,-0.942844461217511));
#54250=DIRECTION('ref_axis',(0.,-0.942844461217511,-0.333233134534159));
#54251=DIRECTION('',(0.,0.333233134534162,-0.94284446121751));
#54252=DIRECTION('center_axis',(0.,0.333233134534162,-0.94284446121751));
#54253=DIRECTION('ref_axis',(0.,-0.94284446121751,-0.333233134534162));
#54254=DIRECTION('center_axis',(0.,-0.333233134534162,0.94284446121751));
#54255=DIRECTION('ref_axis',(0.,-0.94284446121751,-0.333233134534162));
#54256=DIRECTION('center_axis',(0.,0.333233134534162,-0.94284446121751));
#54257=DIRECTION('ref_axis',(0.,0.94284446121751,0.333233134534162));
#54258=DIRECTION('',(0.,-0.333233134534162,0.94284446121751));
#54259=DIRECTION('center_axis',(0.,0.333233134534159,-0.942844461217511));
#54260=DIRECTION('ref_axis',(0.,-0.942844461217511,-0.333233134534159));
#54261=DIRECTION('center_axis',(0.,-0.333233134534162,0.94284446121751));
#54262=DIRECTION('ref_axis',(0.,-0.94284446121751,-0.333233134534162));
#54263=DIRECTION('center_axis',(0.,0.333233134534159,-0.942844461217511));
#54264=DIRECTION('ref_axis',(0.,-0.942844461217511,-0.333233134534159));
#54265=DIRECTION('',(0.,0.333233134534162,-0.94284446121751));
#54266=DIRECTION('center_axis',(0.,0.333233134534162,-0.94284446121751));
#54267=DIRECTION('ref_axis',(0.,-0.94284446121751,-0.333233134534162));
#54268=DIRECTION('center_axis',(0.,-0.333233134534162,0.94284446121751));
#54269=DIRECTION('ref_axis',(0.,-0.94284446121751,-0.333233134534162));
#54270=DIRECTION('center_axis',(0.,0.333233134534162,-0.94284446121751));
#54271=DIRECTION('ref_axis',(0.,0.94284446121751,0.333233134534162));
#54272=DIRECTION('',(0.,-0.333233134534162,0.94284446121751));
#54273=DIRECTION('center_axis',(0.,0.333233134534159,-0.942844461217511));
#54274=DIRECTION('ref_axis',(0.,-0.942844461217511,-0.333233134534159));
#54275=DIRECTION('center_axis',(0.,-0.333233134534162,0.94284446121751));
#54276=DIRECTION('ref_axis',(0.,-0.94284446121751,-0.333233134534162));
#54277=DIRECTION('center_axis',(0.,0.333233134534159,-0.942844461217511));
#54278=DIRECTION('ref_axis',(0.,-0.942844461217511,-0.333233134534159));
#54279=DIRECTION('',(0.,0.333233134534162,-0.94284446121751));
#54280=DIRECTION('center_axis',(0.,-0.333233134534162,0.94284446121751));
#54281=DIRECTION('ref_axis',(0.,-0.94284446121751,-0.333233134534162));
#54282=DIRECTION('center_axis',(0.,-0.333233134534162,0.94284446121751));
#54283=DIRECTION('ref_axis',(0.,-0.94284446121751,-0.333233134534162));
#54284=DIRECTION('center_axis',(0.,0.333233134534162,-0.94284446121751));
#54285=DIRECTION('ref_axis',(0.,0.94284446121751,0.333233134534162));
#54286=DIRECTION('',(0.,-0.333233134534162,0.94284446121751));
#54287=DIRECTION('center_axis',(0.,0.333233134534159,-0.942844461217511));
#54288=DIRECTION('ref_axis',(0.,-0.942844461217511,-0.333233134534159));
#54289=DIRECTION('center_axis',(0.,-0.333233134534162,0.94284446121751));
#54290=DIRECTION('ref_axis',(0.,-0.94284446121751,-0.333233134534162));
#54291=DIRECTION('center_axis',(0.,0.333233134534159,-0.942844461217511));
#54292=DIRECTION('ref_axis',(0.,-0.942844461217511,-0.333233134534159));
#54293=DIRECTION('',(0.,0.333233134534162,-0.94284446121751));
#54294=DIRECTION('center_axis',(0.,0.333233134534162,-0.94284446121751));
#54295=DIRECTION('ref_axis',(0.,-0.94284446121751,-0.333233134534162));
#54296=DIRECTION('center_axis',(0.,-0.333233134534162,0.94284446121751));
#54297=DIRECTION('ref_axis',(0.,-0.94284446121751,-0.333233134534162));
#54298=DIRECTION('center_axis',(0.,0.333233134534162,-0.94284446121751));
#54299=DIRECTION('ref_axis',(0.,0.94284446121751,0.333233134534162));
#54300=DIRECTION('',(0.,-0.333233134534162,0.94284446121751));
#54301=DIRECTION('center_axis',(0.,0.333233134534159,-0.942844461217511));
#54302=DIRECTION('ref_axis',(0.,-0.942844461217511,-0.333233134534159));
#54303=DIRECTION('center_axis',(0.,-0.333233134534162,0.94284446121751));
#54304=DIRECTION('ref_axis',(0.,-0.94284446121751,-0.333233134534162));
#54305=DIRECTION('center_axis',(0.,0.333233134534159,-0.942844461217511));
#54306=DIRECTION('ref_axis',(0.,-0.942844461217511,-0.333233134534159));
#54307=DIRECTION('',(0.,0.333233134534162,-0.94284446121751));
#54308=DIRECTION('center_axis',(0.,0.333233134534162,-0.94284446121751));
#54309=DIRECTION('ref_axis',(0.,-0.94284446121751,-0.333233134534162));
#54310=DIRECTION('center_axis',(0.,-0.333233134534162,0.94284446121751));
#54311=DIRECTION('ref_axis',(0.,-0.94284446121751,-0.333233134534162));
#54312=DIRECTION('center_axis',(0.,0.333233134534162,-0.94284446121751));
#54313=DIRECTION('ref_axis',(0.,0.94284446121751,0.333233134534162));
#54314=DIRECTION('',(0.,-0.333233134534162,0.94284446121751));
#54315=DIRECTION('center_axis',(0.,0.333233134534159,-0.942844461217511));
#54316=DIRECTION('ref_axis',(0.,-0.942844461217511,-0.333233134534159));
#54317=DIRECTION('center_axis',(0.,-0.333233134534162,0.94284446121751));
#54318=DIRECTION('ref_axis',(0.,-0.94284446121751,-0.333233134534162));
#54319=DIRECTION('center_axis',(0.,0.333233134534159,-0.942844461217511));
#54320=DIRECTION('ref_axis',(0.,-0.942844461217511,-0.333233134534159));
#54321=DIRECTION('',(0.,0.333233134534162,-0.94284446121751));
#54322=DIRECTION('center_axis',(0.,0.333233134534162,-0.94284446121751));
#54323=DIRECTION('ref_axis',(0.,-0.94284446121751,-0.333233134534162));
#54324=DIRECTION('center_axis',(0.,-0.333233134534162,0.94284446121751));
#54325=DIRECTION('ref_axis',(0.,-0.94284446121751,-0.333233134534162));
#54326=DIRECTION('center_axis',(0.,0.333233134534162,-0.94284446121751));
#54327=DIRECTION('ref_axis',(0.,0.94284446121751,0.333233134534162));
#54328=DIRECTION('',(0.,-0.333233134534162,0.94284446121751));
#54329=DIRECTION('center_axis',(0.,0.333233134534159,-0.942844461217511));
#54330=DIRECTION('ref_axis',(0.,-0.942844461217511,-0.333233134534159));
#54331=DIRECTION('center_axis',(0.,-0.333233134534162,0.94284446121751));
#54332=DIRECTION('ref_axis',(0.,-0.94284446121751,-0.333233134534162));
#54333=DIRECTION('center_axis',(0.,0.333233134534159,-0.942844461217511));
#54334=DIRECTION('ref_axis',(0.,-0.942844461217511,-0.333233134534159));
#54335=DIRECTION('',(0.,0.333233134534162,-0.94284446121751));
#54336=DIRECTION('center_axis',(0.,0.333233134534162,-0.94284446121751));
#54337=DIRECTION('ref_axis',(0.,-0.94284446121751,-0.333233134534162));
#54338=DIRECTION('center_axis',(0.,-0.333233134534162,0.94284446121751));
#54339=DIRECTION('ref_axis',(0.,-0.94284446121751,-0.333233134534162));
#54340=DIRECTION('center_axis',(0.,0.333233134534162,-0.94284446121751));
#54341=DIRECTION('ref_axis',(0.,0.94284446121751,0.333233134534162));
#54342=DIRECTION('',(0.,-0.333233134534162,0.94284446121751));
#54343=DIRECTION('center_axis',(0.,0.333233134534159,-0.942844461217511));
#54344=DIRECTION('ref_axis',(0.,-0.942844461217511,-0.333233134534159));
#54345=DIRECTION('center_axis',(0.,-0.333233134534162,0.94284446121751));
#54346=DIRECTION('ref_axis',(0.,-0.94284446121751,-0.333233134534162));
#54347=DIRECTION('center_axis',(0.,0.333233134534159,-0.942844461217511));
#54348=DIRECTION('ref_axis',(0.,-0.942844461217511,-0.333233134534159));
#54349=DIRECTION('',(0.,0.333233134534162,-0.94284446121751));
#54350=DIRECTION('center_axis',(0.,0.333233134534162,-0.94284446121751));
#54351=DIRECTION('ref_axis',(0.,-0.94284446121751,-0.333233134534162));
#54352=DIRECTION('center_axis',(0.,-0.333233134534162,0.94284446121751));
#54353=DIRECTION('ref_axis',(0.,-0.94284446121751,-0.333233134534162));
#54354=DIRECTION('center_axis',(0.,0.333233134534162,-0.94284446121751));
#54355=DIRECTION('ref_axis',(0.,0.94284446121751,0.333233134534162));
#54356=DIRECTION('',(0.,-0.333233134534162,0.94284446121751));
#54357=DIRECTION('center_axis',(0.,0.333233134534159,-0.942844461217511));
#54358=DIRECTION('ref_axis',(0.,-0.942844461217511,-0.333233134534159));
#54359=DIRECTION('center_axis',(0.,-0.333233134534162,0.94284446121751));
#54360=DIRECTION('ref_axis',(0.,-0.94284446121751,-0.333233134534162));
#54361=DIRECTION('center_axis',(0.,0.333233134534159,-0.942844461217511));
#54362=DIRECTION('ref_axis',(0.,-0.942844461217511,-0.333233134534159));
#54363=DIRECTION('',(0.,0.333233134534162,-0.94284446121751));
#54364=DIRECTION('center_axis',(0.,0.333233134534162,-0.94284446121751));
#54365=DIRECTION('ref_axis',(0.,-0.94284446121751,-0.333233134534162));
#54366=DIRECTION('center_axis',(0.,-0.333233134534162,0.94284446121751));
#54367=DIRECTION('ref_axis',(0.,-0.94284446121751,-0.333233134534162));
#54368=DIRECTION('center_axis',(0.,0.333233134534162,-0.94284446121751));
#54369=DIRECTION('ref_axis',(0.,0.94284446121751,0.333233134534162));
#54370=DIRECTION('',(0.,-0.333233134534162,0.94284446121751));
#54371=DIRECTION('center_axis',(0.,0.333233134534159,-0.942844461217511));
#54372=DIRECTION('ref_axis',(0.,-0.942844461217511,-0.333233134534159));
#54373=DIRECTION('center_axis',(0.,-0.333233134534162,0.94284446121751));
#54374=DIRECTION('ref_axis',(0.,-0.94284446121751,-0.333233134534162));
#54375=DIRECTION('center_axis',(0.,0.333233134534159,-0.942844461217511));
#54376=DIRECTION('ref_axis',(0.,-0.942844461217511,-0.333233134534159));
#54377=DIRECTION('',(0.,0.333233134534162,-0.94284446121751));
#54378=DIRECTION('center_axis',(0.,0.333233134534162,-0.94284446121751));
#54379=DIRECTION('ref_axis',(0.,-0.94284446121751,-0.333233134534162));
#54380=DIRECTION('center_axis',(0.,-0.333233134534162,0.94284446121751));
#54381=DIRECTION('ref_axis',(0.,-0.94284446121751,-0.333233134534162));
#54382=DIRECTION('center_axis',(0.,0.333233134534162,-0.94284446121751));
#54383=DIRECTION('ref_axis',(0.,0.94284446121751,0.333233134534162));
#54384=DIRECTION('',(0.,-0.333233134534162,0.94284446121751));
#54385=DIRECTION('center_axis',(0.,0.333233134534159,-0.942844461217511));
#54386=DIRECTION('ref_axis',(0.,-0.942844461217511,-0.333233134534159));
#54387=DIRECTION('center_axis',(0.,-0.333233134534162,0.94284446121751));
#54388=DIRECTION('ref_axis',(0.,-0.94284446121751,-0.333233134534162));
#54389=DIRECTION('center_axis',(0.,0.333233134534159,-0.942844461217511));
#54390=DIRECTION('ref_axis',(0.,-0.942844461217511,-0.333233134534159));
#54391=DIRECTION('',(0.,0.333233134534162,-0.94284446121751));
#54392=DIRECTION('center_axis',(0.,0.333233134534162,-0.94284446121751));
#54393=DIRECTION('ref_axis',(0.,-0.94284446121751,-0.333233134534162));
#54394=DIRECTION('center_axis',(0.,-0.333233134534162,0.94284446121751));
#54395=DIRECTION('ref_axis',(0.,-0.94284446121751,-0.333233134534162));
#54396=DIRECTION('center_axis',(0.,0.333233134534162,-0.94284446121751));
#54397=DIRECTION('ref_axis',(0.,0.94284446121751,0.333233134534162));
#54398=DIRECTION('',(0.,-0.333233134534162,0.94284446121751));
#54399=DIRECTION('center_axis',(0.,0.333233134534159,-0.942844461217511));
#54400=DIRECTION('ref_axis',(0.,-0.942844461217511,-0.333233134534159));
#54401=DIRECTION('center_axis',(0.,-0.333233134534162,0.94284446121751));
#54402=DIRECTION('ref_axis',(0.,-0.94284446121751,-0.333233134534162));
#54403=DIRECTION('center_axis',(0.,0.333233134534159,-0.942844461217511));
#54404=DIRECTION('ref_axis',(0.,-0.942844461217511,-0.333233134534159));
#54405=DIRECTION('',(0.,0.333233134534162,-0.94284446121751));
#54406=DIRECTION('center_axis',(0.,-0.333233134534162,0.94284446121751));
#54407=DIRECTION('ref_axis',(0.,-0.94284446121751,-0.333233134534162));
#54408=DIRECTION('center_axis',(0.,-0.333233134534162,0.94284446121751));
#54409=DIRECTION('ref_axis',(0.,-0.94284446121751,-0.333233134534162));
#54410=DIRECTION('center_axis',(0.,0.333233134534162,-0.94284446121751));
#54411=DIRECTION('ref_axis',(0.,0.94284446121751,0.333233134534162));
#54412=DIRECTION('',(0.,-0.333233134534162,0.94284446121751));
#54413=DIRECTION('center_axis',(0.,0.333233134534159,-0.942844461217511));
#54414=DIRECTION('ref_axis',(0.,-0.942844461217511,-0.333233134534159));
#54415=DIRECTION('center_axis',(0.,-0.333233134534162,0.94284446121751));
#54416=DIRECTION('ref_axis',(0.,-0.94284446121751,-0.333233134534162));
#54417=DIRECTION('center_axis',(0.,0.333233134534159,-0.942844461217511));
#54418=DIRECTION('ref_axis',(0.,-0.942844461217511,-0.333233134534159));
#54419=DIRECTION('',(0.,0.333233134534162,-0.94284446121751));
#54420=DIRECTION('center_axis',(0.,0.333233134534162,-0.94284446121751));
#54421=DIRECTION('ref_axis',(0.,-0.94284446121751,-0.333233134534162));
#54422=DIRECTION('center_axis',(0.,-0.333233134534162,0.94284446121751));
#54423=DIRECTION('ref_axis',(0.,-0.94284446121751,-0.333233134534162));
#54424=DIRECTION('center_axis',(0.,0.333233134534162,-0.94284446121751));
#54425=DIRECTION('ref_axis',(0.,0.94284446121751,0.333233134534162));
#54426=DIRECTION('',(0.,-0.333233134534162,0.94284446121751));
#54427=DIRECTION('center_axis',(0.,0.333233134534159,-0.942844461217511));
#54428=DIRECTION('ref_axis',(0.,-0.942844461217511,-0.333233134534159));
#54429=DIRECTION('center_axis',(0.,-0.333233134534162,0.94284446121751));
#54430=DIRECTION('ref_axis',(0.,-0.94284446121751,-0.333233134534162));
#54431=DIRECTION('center_axis',(0.,0.333233134534159,-0.942844461217511));
#54432=DIRECTION('ref_axis',(0.,-0.942844461217511,-0.333233134534159));
#54433=DIRECTION('',(0.,0.333233134534162,-0.94284446121751));
#54434=DIRECTION('center_axis',(0.,0.333233134534162,-0.94284446121751));
#54435=DIRECTION('ref_axis',(0.,-0.94284446121751,-0.333233134534162));
#54436=DIRECTION('center_axis',(0.,-0.333233134534162,0.94284446121751));
#54437=DIRECTION('ref_axis',(0.,-0.94284446121751,-0.333233134534162));
#54438=DIRECTION('center_axis',(0.,0.333233134534162,-0.94284446121751));
#54439=DIRECTION('ref_axis',(0.,0.94284446121751,0.333233134534162));
#54440=DIRECTION('',(0.,-0.333233134534162,0.94284446121751));
#54441=DIRECTION('center_axis',(0.,0.333233134534159,-0.942844461217511));
#54442=DIRECTION('ref_axis',(0.,-0.942844461217511,-0.333233134534159));
#54443=DIRECTION('center_axis',(0.,-0.333233134534162,0.94284446121751));
#54444=DIRECTION('ref_axis',(0.,-0.94284446121751,-0.333233134534162));
#54445=DIRECTION('center_axis',(0.,0.333233134534159,-0.942844461217511));
#54446=DIRECTION('ref_axis',(0.,-0.942844461217511,-0.333233134534159));
#54447=DIRECTION('',(0.,0.333233134534162,-0.94284446121751));
#54448=DIRECTION('center_axis',(0.,0.333233134534162,-0.94284446121751));
#54449=DIRECTION('ref_axis',(0.,-0.94284446121751,-0.333233134534162));
#54450=DIRECTION('center_axis',(0.,-0.333233134534162,0.94284446121751));
#54451=DIRECTION('ref_axis',(0.,-0.94284446121751,-0.333233134534162));
#54452=DIRECTION('center_axis',(0.,0.333233134534162,-0.94284446121751));
#54453=DIRECTION('ref_axis',(0.,0.94284446121751,0.333233134534162));
#54454=DIRECTION('',(0.,-0.333233134534162,0.94284446121751));
#54455=DIRECTION('center_axis',(0.,0.333233134534159,-0.942844461217511));
#54456=DIRECTION('ref_axis',(0.,-0.942844461217511,-0.333233134534159));
#54457=DIRECTION('center_axis',(0.,-0.333233134534162,0.94284446121751));
#54458=DIRECTION('ref_axis',(0.,-0.94284446121751,-0.333233134534162));
#54459=DIRECTION('center_axis',(0.,0.333233134534159,-0.942844461217511));
#54460=DIRECTION('ref_axis',(0.,-0.942844461217511,-0.333233134534159));
#54461=DIRECTION('',(0.,0.333233134534162,-0.94284446121751));
#54462=DIRECTION('center_axis',(0.,0.333233134534162,-0.94284446121751));
#54463=DIRECTION('ref_axis',(0.,-0.94284446121751,-0.333233134534162));
#54464=DIRECTION('center_axis',(0.,-0.333233134534162,0.94284446121751));
#54465=DIRECTION('ref_axis',(0.,-0.94284446121751,-0.333233134534162));
#54466=DIRECTION('center_axis',(0.,0.333233134534162,-0.94284446121751));
#54467=DIRECTION('ref_axis',(0.,0.94284446121751,0.333233134534162));
#54468=DIRECTION('',(0.,-0.333233134534162,0.94284446121751));
#54469=DIRECTION('center_axis',(0.,0.333233134534159,-0.942844461217511));
#54470=DIRECTION('ref_axis',(0.,-0.942844461217511,-0.333233134534159));
#54471=DIRECTION('center_axis',(0.,-0.333233134534162,0.94284446121751));
#54472=DIRECTION('ref_axis',(0.,-0.94284446121751,-0.333233134534162));
#54473=DIRECTION('center_axis',(0.,0.333233134534159,-0.942844461217511));
#54474=DIRECTION('ref_axis',(0.,-0.942844461217511,-0.333233134534159));
#54475=DIRECTION('',(0.,0.333233134534162,-0.94284446121751));
#54476=DIRECTION('center_axis',(0.,0.333233134534162,-0.94284446121751));
#54477=DIRECTION('ref_axis',(0.,-0.94284446121751,-0.333233134534162));
#54478=DIRECTION('center_axis',(0.,-0.333233134534162,0.94284446121751));
#54479=DIRECTION('ref_axis',(0.,-0.94284446121751,-0.333233134534162));
#54480=DIRECTION('center_axis',(0.,0.333233134534162,-0.94284446121751));
#54481=DIRECTION('ref_axis',(0.,0.94284446121751,0.333233134534162));
#54482=DIRECTION('',(0.,-0.333233134534162,0.94284446121751));
#54483=DIRECTION('center_axis',(0.,0.333233134534159,-0.942844461217511));
#54484=DIRECTION('ref_axis',(0.,-0.942844461217511,-0.333233134534159));
#54485=DIRECTION('center_axis',(0.,-0.333233134534162,0.94284446121751));
#54486=DIRECTION('ref_axis',(0.,-0.94284446121751,-0.333233134534162));
#54487=DIRECTION('center_axis',(0.,0.333233134534159,-0.942844461217511));
#54488=DIRECTION('ref_axis',(0.,-0.942844461217511,-0.333233134534159));
#54489=DIRECTION('',(0.,0.333233134534162,-0.94284446121751));
#54490=DIRECTION('center_axis',(0.,0.333233134534162,-0.94284446121751));
#54491=DIRECTION('ref_axis',(0.,-0.94284446121751,-0.333233134534162));
#54492=DIRECTION('center_axis',(0.,-0.333233134534162,0.94284446121751));
#54493=DIRECTION('ref_axis',(0.,-0.94284446121751,-0.333233134534162));
#54494=DIRECTION('center_axis',(0.,0.333233134534162,-0.94284446121751));
#54495=DIRECTION('ref_axis',(0.,0.94284446121751,0.333233134534162));
#54496=DIRECTION('',(0.,-0.333233134534162,0.94284446121751));
#54497=DIRECTION('center_axis',(0.,0.333233134534159,-0.942844461217511));
#54498=DIRECTION('ref_axis',(0.,-0.942844461217511,-0.333233134534159));
#54499=DIRECTION('center_axis',(0.,-0.333233134534162,0.94284446121751));
#54500=DIRECTION('ref_axis',(0.,-0.94284446121751,-0.333233134534162));
#54501=DIRECTION('center_axis',(0.,0.333233134534159,-0.942844461217511));
#54502=DIRECTION('ref_axis',(0.,-0.942844461217511,-0.333233134534159));
#54503=DIRECTION('',(0.,0.333233134534162,-0.94284446121751));
#54504=DIRECTION('center_axis',(0.,0.333233134534162,-0.94284446121751));
#54505=DIRECTION('ref_axis',(0.,-0.94284446121751,-0.333233134534162));
#54506=DIRECTION('center_axis',(0.,-0.333233134534162,0.94284446121751));
#54507=DIRECTION('ref_axis',(0.,-0.94284446121751,-0.333233134534162));
#54508=DIRECTION('center_axis',(0.,0.333233134534162,-0.94284446121751));
#54509=DIRECTION('ref_axis',(0.,0.94284446121751,0.333233134534162));
#54510=DIRECTION('',(0.,-0.333233134534162,0.94284446121751));
#54511=DIRECTION('center_axis',(0.,0.333233134534159,-0.942844461217511));
#54512=DIRECTION('ref_axis',(0.,-0.942844461217511,-0.333233134534159));
#54513=DIRECTION('center_axis',(0.,-0.333233134534162,0.94284446121751));
#54514=DIRECTION('ref_axis',(0.,-0.94284446121751,-0.333233134534162));
#54515=DIRECTION('center_axis',(0.,0.333233134534159,-0.942844461217511));
#54516=DIRECTION('ref_axis',(0.,-0.942844461217511,-0.333233134534159));
#54517=DIRECTION('',(0.,0.333233134534162,-0.94284446121751));
#54518=DIRECTION('center_axis',(0.,-0.333233134534162,0.94284446121751));
#54519=DIRECTION('ref_axis',(0.,-0.94284446121751,-0.333233134534162));
#54520=DIRECTION('center_axis',(0.,-0.333233134534162,0.94284446121751));
#54521=DIRECTION('ref_axis',(0.,-0.94284446121751,-0.333233134534162));
#54522=DIRECTION('center_axis',(0.,0.333233134534162,-0.94284446121751));
#54523=DIRECTION('ref_axis',(0.,0.94284446121751,0.333233134534162));
#54524=DIRECTION('',(0.,-0.333233134534162,0.94284446121751));
#54525=DIRECTION('center_axis',(0.,0.333233134534159,-0.942844461217511));
#54526=DIRECTION('ref_axis',(0.,-0.942844461217511,-0.333233134534159));
#54527=DIRECTION('center_axis',(0.,-0.333233134534162,0.94284446121751));
#54528=DIRECTION('ref_axis',(0.,-0.94284446121751,-0.333233134534162));
#54529=DIRECTION('center_axis',(0.,0.333233134534159,-0.942844461217511));
#54530=DIRECTION('ref_axis',(0.,-0.942844461217511,-0.333233134534159));
#54531=DIRECTION('',(0.,0.333233134534162,-0.94284446121751));
#54532=DIRECTION('center_axis',(0.,0.333233134534162,-0.94284446121751));
#54533=DIRECTION('ref_axis',(0.,-0.94284446121751,-0.333233134534162));
#54534=DIRECTION('center_axis',(0.,-0.333233134534162,0.94284446121751));
#54535=DIRECTION('ref_axis',(0.,-0.94284446121751,-0.333233134534162));
#54536=DIRECTION('center_axis',(0.,0.333233134534162,-0.94284446121751));
#54537=DIRECTION('ref_axis',(0.,0.94284446121751,0.333233134534162));
#54538=DIRECTION('',(0.,-0.333233134534162,0.94284446121751));
#54539=DIRECTION('center_axis',(0.,0.333233134534159,-0.942844461217511));
#54540=DIRECTION('ref_axis',(0.,-0.942844461217511,-0.333233134534159));
#54541=DIRECTION('center_axis',(0.,-0.333233134534162,0.94284446121751));
#54542=DIRECTION('ref_axis',(0.,-0.94284446121751,-0.333233134534162));
#54543=DIRECTION('center_axis',(0.,0.333233134534159,-0.942844461217511));
#54544=DIRECTION('ref_axis',(0.,-0.942844461217511,-0.333233134534159));
#54545=DIRECTION('',(0.,0.333233134534162,-0.94284446121751));
#54546=DIRECTION('center_axis',(0.,0.333233134534162,-0.94284446121751));
#54547=DIRECTION('ref_axis',(0.,-0.94284446121751,-0.333233134534162));
#54548=DIRECTION('center_axis',(0.,-0.333233134534162,0.94284446121751));
#54549=DIRECTION('ref_axis',(0.,-0.94284446121751,-0.333233134534162));
#54550=DIRECTION('center_axis',(0.,0.333233134534162,-0.94284446121751));
#54551=DIRECTION('ref_axis',(0.,0.94284446121751,0.333233134534162));
#54552=DIRECTION('',(0.,-0.333233134534162,0.94284446121751));
#54553=DIRECTION('center_axis',(0.,0.333233134534159,-0.942844461217511));
#54554=DIRECTION('ref_axis',(0.,-0.942844461217511,-0.333233134534159));
#54555=DIRECTION('center_axis',(0.,-0.333233134534162,0.94284446121751));
#54556=DIRECTION('ref_axis',(0.,-0.94284446121751,-0.333233134534162));
#54557=DIRECTION('center_axis',(0.,0.333233134534159,-0.942844461217511));
#54558=DIRECTION('ref_axis',(0.,-0.942844461217511,-0.333233134534159));
#54559=DIRECTION('',(0.,0.333233134534162,-0.94284446121751));
#54560=DIRECTION('center_axis',(0.,0.333233134534162,-0.94284446121751));
#54561=DIRECTION('ref_axis',(0.,-0.94284446121751,-0.333233134534162));
#54562=DIRECTION('center_axis',(0.,-0.333233134534162,0.94284446121751));
#54563=DIRECTION('ref_axis',(0.,-0.94284446121751,-0.333233134534162));
#54564=DIRECTION('center_axis',(0.,0.333233134534162,-0.94284446121751));
#54565=DIRECTION('ref_axis',(0.,0.94284446121751,0.333233134534162));
#54566=DIRECTION('',(0.,-0.333233134534162,0.94284446121751));
#54567=DIRECTION('center_axis',(0.,0.333233134534159,-0.942844461217511));
#54568=DIRECTION('ref_axis',(0.,-0.942844461217511,-0.333233134534159));
#54569=DIRECTION('center_axis',(0.,-0.333233134534162,0.94284446121751));
#54570=DIRECTION('ref_axis',(0.,-0.94284446121751,-0.333233134534162));
#54571=DIRECTION('center_axis',(0.,0.333233134534159,-0.942844461217511));
#54572=DIRECTION('ref_axis',(0.,-0.942844461217511,-0.333233134534159));
#54573=DIRECTION('',(0.,0.333233134534162,-0.94284446121751));
#54574=DIRECTION('center_axis',(0.,0.333233134534162,-0.94284446121751));
#54575=DIRECTION('ref_axis',(0.,-0.94284446121751,-0.333233134534162));
#54576=DIRECTION('center_axis',(0.,-0.333233134534162,0.94284446121751));
#54577=DIRECTION('ref_axis',(0.,-0.94284446121751,-0.333233134534162));
#54578=DIRECTION('center_axis',(0.,0.333233134534162,-0.94284446121751));
#54579=DIRECTION('ref_axis',(0.,0.94284446121751,0.333233134534162));
#54580=DIRECTION('',(0.,-0.333233134534162,0.94284446121751));
#54581=DIRECTION('center_axis',(0.,0.333233134534159,-0.942844461217511));
#54582=DIRECTION('ref_axis',(0.,-0.942844461217511,-0.333233134534159));
#54583=DIRECTION('center_axis',(0.,-0.333233134534162,0.94284446121751));
#54584=DIRECTION('ref_axis',(0.,-0.94284446121751,-0.333233134534162));
#54585=DIRECTION('center_axis',(0.,0.333233134534159,-0.942844461217511));
#54586=DIRECTION('ref_axis',(0.,-0.942844461217511,-0.333233134534159));
#54587=DIRECTION('',(0.,0.333233134534162,-0.94284446121751));
#54588=DIRECTION('center_axis',(0.,0.333233134534162,-0.94284446121751));
#54589=DIRECTION('ref_axis',(0.,-0.94284446121751,-0.333233134534162));
#54590=DIRECTION('center_axis',(0.,-0.333233134534162,0.94284446121751));
#54591=DIRECTION('ref_axis',(0.,-0.94284446121751,-0.333233134534162));
#54592=DIRECTION('center_axis',(0.,0.333233134534162,-0.94284446121751));
#54593=DIRECTION('ref_axis',(0.,0.94284446121751,0.333233134534162));
#54594=DIRECTION('',(0.,-0.333233134534162,0.94284446121751));
#54595=DIRECTION('center_axis',(0.,0.333233134534159,-0.942844461217511));
#54596=DIRECTION('ref_axis',(0.,-0.942844461217511,-0.333233134534159));
#54597=DIRECTION('center_axis',(0.,-0.333233134534162,0.94284446121751));
#54598=DIRECTION('ref_axis',(0.,-0.94284446121751,-0.333233134534162));
#54599=DIRECTION('center_axis',(0.,0.333233134534159,-0.942844461217511));
#54600=DIRECTION('ref_axis',(0.,-0.942844461217511,-0.333233134534159));
#54601=DIRECTION('',(0.,0.333233134534162,-0.94284446121751));
#54602=DIRECTION('center_axis',(0.,0.333233134534162,-0.94284446121751));
#54603=DIRECTION('ref_axis',(0.,-0.94284446121751,-0.333233134534162));
#54604=DIRECTION('center_axis',(0.,-0.333233134534162,0.94284446121751));
#54605=DIRECTION('ref_axis',(0.,-0.94284446121751,-0.333233134534162));
#54606=DIRECTION('center_axis',(0.,0.333233134534162,-0.94284446121751));
#54607=DIRECTION('ref_axis',(0.,0.94284446121751,0.333233134534162));
#54608=DIRECTION('',(0.,-0.333233134534162,0.94284446121751));
#54609=DIRECTION('center_axis',(0.,0.333233134534159,-0.942844461217511));
#54610=DIRECTION('ref_axis',(0.,-0.942844461217511,-0.333233134534159));
#54611=DIRECTION('center_axis',(0.,-0.333233134534162,0.94284446121751));
#54612=DIRECTION('ref_axis',(0.,-0.94284446121751,-0.333233134534162));
#54613=DIRECTION('center_axis',(0.,0.333233134534159,-0.942844461217511));
#54614=DIRECTION('ref_axis',(0.,-0.942844461217511,-0.333233134534159));
#54615=DIRECTION('',(0.,0.333233134534162,-0.94284446121751));
#54616=DIRECTION('center_axis',(0.,0.333233134534162,-0.94284446121751));
#54617=DIRECTION('ref_axis',(0.,-0.94284446121751,-0.333233134534162));
#54618=DIRECTION('center_axis',(0.,-0.333233134534162,0.94284446121751));
#54619=DIRECTION('ref_axis',(0.,-0.94284446121751,-0.333233134534161));
#54620=DIRECTION('center_axis',(0.,0.333233134534162,-0.94284446121751));
#54621=DIRECTION('ref_axis',(0.,0.94284446121751,0.333233134534162));
#54622=DIRECTION('',(0.,-0.333233134534162,0.94284446121751));
#54623=DIRECTION('center_axis',(0.,0.333233134534159,-0.942844461217511));
#54624=DIRECTION('ref_axis',(0.,-0.942844461217511,-0.333233134534159));
#54625=DIRECTION('center_axis',(0.,-0.333233134534162,0.94284446121751));
#54626=DIRECTION('ref_axis',(0.,-0.94284446121751,-0.333233134534162));
#54627=DIRECTION('center_axis',(0.,0.333233134534159,-0.942844461217511));
#54628=DIRECTION('ref_axis',(0.,-0.942844461217511,-0.333233134534159));
#54629=DIRECTION('',(0.,0.333233134534162,-0.94284446121751));
#54630=DIRECTION('center_axis',(0.,0.333233134534162,-0.94284446121751));
#54631=DIRECTION('ref_axis',(0.,-0.94284446121751,-0.333233134534162));
#54632=DIRECTION('center_axis',(0.,-0.333233134534162,0.94284446121751));
#54633=DIRECTION('ref_axis',(0.,-0.94284446121751,-0.333233134534162));
#54634=DIRECTION('center_axis',(0.,0.333233134534162,-0.94284446121751));
#54635=DIRECTION('ref_axis',(0.,0.94284446121751,0.333233134534162));
#54636=DIRECTION('',(0.,-0.333233134534162,0.94284446121751));
#54637=DIRECTION('center_axis',(0.,0.333233134534159,-0.942844461217511));
#54638=DIRECTION('ref_axis',(0.,-0.942844461217511,-0.333233134534159));
#54639=DIRECTION('center_axis',(0.,-0.333233134534162,0.94284446121751));
#54640=DIRECTION('ref_axis',(0.,-0.94284446121751,-0.333233134534162));
#54641=DIRECTION('center_axis',(0.,0.333233134534159,-0.942844461217511));
#54642=DIRECTION('ref_axis',(0.,-0.942844461217511,-0.333233134534159));
#54643=DIRECTION('',(0.,0.333233134534162,-0.94284446121751));
#54644=DIRECTION('center_axis',(0.,-0.333233134534162,0.94284446121751));
#54645=DIRECTION('ref_axis',(0.,-0.94284446121751,-0.333233134534162));
#54646=DIRECTION('center_axis',(0.,-0.333233134534162,0.94284446121751));
#54647=DIRECTION('ref_axis',(0.,-0.94284446121751,-0.333233134534162));
#54648=DIRECTION('center_axis',(0.,-0.333233134534162,0.94284446121751));
#54649=DIRECTION('ref_axis',(0.,-0.94284446121751,-0.333233134534162));
#54650=DIRECTION('center_axis',(0.,0.333233134534162,-0.94284446121751));
#54651=DIRECTION('ref_axis',(0.,0.94284446121751,0.333233134534162));
#54652=DIRECTION('',(0.,-0.333233134534162,0.94284446121751));
#54653=DIRECTION('center_axis',(0.,0.333233134534159,-0.942844461217511));
#54654=DIRECTION('ref_axis',(0.,-0.942844461217511,-0.333233134534159));
#54655=DIRECTION('center_axis',(0.,-0.333233134534162,0.94284446121751));
#54656=DIRECTION('ref_axis',(0.,-0.94284446121751,-0.333233134534161));
#54657=DIRECTION('center_axis',(0.,0.333233134534159,-0.942844461217511));
#54658=DIRECTION('ref_axis',(0.,-0.942844461217511,-0.333233134534159));
#54659=DIRECTION('',(0.,0.333233134534162,-0.94284446121751));
#54660=DIRECTION('center_axis',(0.,0.333233134534162,-0.94284446121751));
#54661=DIRECTION('ref_axis',(0.,-0.94284446121751,-0.333233134534162));
#54662=DIRECTION('center_axis',(0.,-0.333233134534162,0.94284446121751));
#54663=DIRECTION('ref_axis',(0.,-0.94284446121751,-0.333233134534162));
#54664=DIRECTION('center_axis',(0.,0.333233134534162,-0.94284446121751));
#54665=DIRECTION('ref_axis',(0.,0.94284446121751,0.333233134534162));
#54666=DIRECTION('',(0.,-0.333233134534162,0.94284446121751));
#54667=DIRECTION('center_axis',(0.,0.333233134534159,-0.942844461217511));
#54668=DIRECTION('ref_axis',(0.,-0.942844461217511,-0.333233134534159));
#54669=DIRECTION('center_axis',(0.,-0.333233134534162,0.94284446121751));
#54670=DIRECTION('ref_axis',(0.,-0.94284446121751,-0.333233134534162));
#54671=DIRECTION('center_axis',(0.,0.333233134534159,-0.942844461217511));
#54672=DIRECTION('ref_axis',(0.,-0.942844461217511,-0.333233134534159));
#54673=DIRECTION('',(0.,0.333233134534162,-0.94284446121751));
#54674=DIRECTION('center_axis',(0.,0.333233134534162,-0.94284446121751));
#54675=DIRECTION('ref_axis',(0.,-0.94284446121751,-0.333233134534162));
#54676=DIRECTION('center_axis',(0.,-0.333233134534162,0.94284446121751));
#54677=DIRECTION('ref_axis',(0.,-0.94284446121751,-0.333233134534162));
#54678=DIRECTION('center_axis',(0.,0.333233134534162,-0.94284446121751));
#54679=DIRECTION('ref_axis',(0.,0.94284446121751,0.333233134534162));
#54680=DIRECTION('',(0.,-0.333233134534162,0.94284446121751));
#54681=DIRECTION('center_axis',(0.,0.333233134534159,-0.942844461217511));
#54682=DIRECTION('ref_axis',(0.,-0.942844461217511,-0.333233134534159));
#54683=DIRECTION('center_axis',(0.,-0.333233134534162,0.94284446121751));
#54684=DIRECTION('ref_axis',(0.,-0.94284446121751,-0.333233134534162));
#54685=DIRECTION('center_axis',(0.,0.333233134534159,-0.942844461217511));
#54686=DIRECTION('ref_axis',(0.,-0.942844461217511,-0.333233134534159));
#54687=DIRECTION('',(0.,0.333233134534161,-0.94284446121751));
#54688=DIRECTION('center_axis',(0.,0.333233134534162,-0.94284446121751));
#54689=DIRECTION('ref_axis',(0.,-0.94284446121751,-0.333233134534162));
#54690=DIRECTION('center_axis',(0.,-0.333233134534162,0.94284446121751));
#54691=DIRECTION('ref_axis',(0.,-0.94284446121751,-0.333233134534162));
#54692=DIRECTION('center_axis',(0.,0.333233134534162,-0.94284446121751));
#54693=DIRECTION('ref_axis',(0.,0.94284446121751,0.333233134534162));
#54694=DIRECTION('',(0.,-0.333233134534162,0.94284446121751));
#54695=DIRECTION('center_axis',(0.,0.333233134534159,-0.942844461217511));
#54696=DIRECTION('ref_axis',(0.,-0.942844461217511,-0.333233134534159));
#54697=DIRECTION('center_axis',(0.,-0.333233134534162,0.94284446121751));
#54698=DIRECTION('ref_axis',(0.,-0.94284446121751,-0.333233134534162));
#54699=DIRECTION('center_axis',(0.,0.333233134534159,-0.942844461217511));
#54700=DIRECTION('ref_axis',(0.,-0.942844461217511,-0.333233134534159));
#54701=DIRECTION('',(0.,0.333233134534162,-0.94284446121751));
#54702=DIRECTION('center_axis',(0.,0.333233134534162,-0.94284446121751));
#54703=DIRECTION('ref_axis',(0.,-0.94284446121751,-0.333233134534162));
#54704=DIRECTION('center_axis',(0.,-0.333233134534162,0.94284446121751));
#54705=DIRECTION('ref_axis',(0.,-0.94284446121751,-0.333233134534162));
#54706=DIRECTION('center_axis',(0.,0.333233134534162,-0.94284446121751));
#54707=DIRECTION('ref_axis',(0.,0.94284446121751,0.333233134534162));
#54708=DIRECTION('',(0.,-0.333233134534162,0.94284446121751));
#54709=DIRECTION('center_axis',(0.,0.333233134534159,-0.942844461217511));
#54710=DIRECTION('ref_axis',(0.,-0.942844461217511,-0.333233134534159));
#54711=DIRECTION('center_axis',(0.,-0.333233134534162,0.94284446121751));
#54712=DIRECTION('ref_axis',(0.,-0.94284446121751,-0.333233134534162));
#54713=DIRECTION('center_axis',(0.,0.333233134534159,-0.942844461217511));
#54714=DIRECTION('ref_axis',(0.,-0.942844461217511,-0.333233134534159));
#54715=DIRECTION('',(0.,0.333233134534162,-0.94284446121751));
#54716=DIRECTION('center_axis',(0.,0.333233134534162,-0.94284446121751));
#54717=DIRECTION('ref_axis',(0.,-0.94284446121751,-0.333233134534162));
#54718=DIRECTION('center_axis',(0.,-0.333233134534162,0.94284446121751));
#54719=DIRECTION('ref_axis',(0.,-0.94284446121751,-0.333233134534162));
#54720=DIRECTION('center_axis',(0.,0.333233134534162,-0.94284446121751));
#54721=DIRECTION('ref_axis',(0.,0.94284446121751,0.333233134534162));
#54722=DIRECTION('',(0.,-0.333233134534162,0.94284446121751));
#54723=DIRECTION('center_axis',(0.,0.333233134534159,-0.942844461217511));
#54724=DIRECTION('ref_axis',(0.,-0.942844461217511,-0.333233134534159));
#54725=DIRECTION('center_axis',(0.,-0.333233134534162,0.94284446121751));
#54726=DIRECTION('ref_axis',(0.,-0.94284446121751,-0.333233134534162));
#54727=DIRECTION('center_axis',(0.,0.333233134534159,-0.942844461217511));
#54728=DIRECTION('ref_axis',(0.,-0.942844461217511,-0.333233134534159));
#54729=DIRECTION('',(0.,0.333233134534162,-0.94284446121751));
#54730=DIRECTION('center_axis',(0.,0.333233134534162,-0.94284446121751));
#54731=DIRECTION('ref_axis',(0.,-0.94284446121751,-0.333233134534162));
#54732=DIRECTION('center_axis',(0.,-0.333233134534162,0.94284446121751));
#54733=DIRECTION('ref_axis',(0.,-0.94284446121751,-0.333233134534162));
#54734=DIRECTION('center_axis',(0.,0.333233134534162,-0.94284446121751));
#54735=DIRECTION('ref_axis',(0.,0.94284446121751,0.333233134534162));
#54736=DIRECTION('',(0.,-0.333233134534162,0.94284446121751));
#54737=DIRECTION('center_axis',(0.,0.333233134534159,-0.942844461217511));
#54738=DIRECTION('ref_axis',(0.,-0.942844461217511,-0.333233134534159));
#54739=DIRECTION('center_axis',(0.,-0.333233134534162,0.94284446121751));
#54740=DIRECTION('ref_axis',(0.,-0.94284446121751,-0.333233134534162));
#54741=DIRECTION('center_axis',(0.,0.333233134534159,-0.942844461217511));
#54742=DIRECTION('ref_axis',(0.,-0.942844461217511,-0.333233134534159));
#54743=DIRECTION('',(0.,0.333233134534162,-0.94284446121751));
#54744=DIRECTION('center_axis',(0.,0.333233134534162,-0.94284446121751));
#54745=DIRECTION('ref_axis',(0.,-0.94284446121751,-0.333233134534162));
#54746=DIRECTION('center_axis',(0.,-0.333233134534162,0.94284446121751));
#54747=DIRECTION('ref_axis',(0.,-0.94284446121751,-0.333233134534162));
#54748=DIRECTION('center_axis',(0.,0.333233134534162,-0.94284446121751));
#54749=DIRECTION('ref_axis',(0.,0.94284446121751,0.333233134534162));
#54750=DIRECTION('',(0.,-0.333233134534162,0.94284446121751));
#54751=DIRECTION('center_axis',(0.,0.333233134534159,-0.942844461217511));
#54752=DIRECTION('ref_axis',(0.,-0.942844461217511,-0.333233134534159));
#54753=DIRECTION('center_axis',(0.,-0.333233134534162,0.94284446121751));
#54754=DIRECTION('ref_axis',(0.,-0.94284446121751,-0.333233134534162));
#54755=DIRECTION('center_axis',(0.,0.333233134534159,-0.942844461217511));
#54756=DIRECTION('ref_axis',(0.,-0.942844461217511,-0.333233134534159));
#54757=DIRECTION('',(0.,0.333233134534162,-0.94284446121751));
#54758=DIRECTION('center_axis',(0.,-0.333233134534162,0.94284446121751));
#54759=DIRECTION('ref_axis',(0.,-0.94284446121751,-0.333233134534162));
#54760=DIRECTION('center_axis',(0.,-0.333233134534162,0.94284446121751));
#54761=DIRECTION('ref_axis',(0.,-0.94284446121751,-0.333233134534162));
#54762=DIRECTION('center_axis',(0.,-0.333233134534162,0.94284446121751));
#54763=DIRECTION('ref_axis',(0.,-0.94284446121751,-0.333233134534162));
#54764=DIRECTION('center_axis',(0.,0.333233134534162,-0.94284446121751));
#54765=DIRECTION('ref_axis',(0.,0.94284446121751,0.333233134534162));
#54766=DIRECTION('',(0.,-0.333233134534162,0.94284446121751));
#54767=DIRECTION('center_axis',(0.,0.333233134534159,-0.942844461217511));
#54768=DIRECTION('ref_axis',(0.,-0.942844461217511,-0.333233134534159));
#54769=DIRECTION('center_axis',(0.,-0.333233134534162,0.94284446121751));
#54770=DIRECTION('ref_axis',(0.,-0.94284446121751,-0.333233134534162));
#54771=DIRECTION('center_axis',(0.,0.333233134534159,-0.942844461217511));
#54772=DIRECTION('ref_axis',(0.,-0.942844461217511,-0.333233134534159));
#54773=DIRECTION('',(0.,0.333233134534162,-0.94284446121751));
#54774=DIRECTION('center_axis',(0.,-0.333233134534162,0.94284446121751));
#54775=DIRECTION('ref_axis',(0.,-0.94284446121751,-0.333233134534162));
#54776=DIRECTION('center_axis',(0.,-0.333233134534162,0.94284446121751));
#54777=DIRECTION('ref_axis',(0.,-0.94284446121751,-0.333233134534162));
#54778=DIRECTION('center_axis',(0.,-0.333233134534162,0.94284446121751));
#54779=DIRECTION('ref_axis',(0.,-0.94284446121751,-0.333233134534162));
#54780=DIRECTION('center_axis',(0.,0.333233134534162,-0.94284446121751));
#54781=DIRECTION('ref_axis',(0.,0.94284446121751,0.333233134534162));
#54782=DIRECTION('',(0.,-0.333233134534162,0.94284446121751));
#54783=DIRECTION('center_axis',(0.,0.333233134534159,-0.942844461217511));
#54784=DIRECTION('ref_axis',(0.,-0.942844461217511,-0.333233134534159));
#54785=DIRECTION('center_axis',(0.,-0.333233134534162,0.94284446121751));
#54786=DIRECTION('ref_axis',(0.,-0.94284446121751,-0.333233134534162));
#54787=DIRECTION('center_axis',(0.,0.333233134534159,-0.942844461217511));
#54788=DIRECTION('ref_axis',(0.,-0.942844461217511,-0.333233134534159));
#54789=DIRECTION('',(0.,0.333233134534162,-0.94284446121751));
#54790=DIRECTION('center_axis',(0.,0.333233134534162,-0.94284446121751));
#54791=DIRECTION('ref_axis',(0.,-0.94284446121751,-0.333233134534162));
#54792=DIRECTION('center_axis',(0.,-0.333233134534162,0.94284446121751));
#54793=DIRECTION('ref_axis',(0.,-0.94284446121751,-0.333233134534162));
#54794=DIRECTION('center_axis',(0.,0.333233134534162,-0.94284446121751));
#54795=DIRECTION('ref_axis',(0.,0.94284446121751,0.333233134534162));
#54796=DIRECTION('',(0.,-0.333233134534162,0.94284446121751));
#54797=DIRECTION('center_axis',(0.,0.333233134534159,-0.942844461217511));
#54798=DIRECTION('ref_axis',(0.,-0.942844461217511,-0.333233134534159));
#54799=DIRECTION('center_axis',(0.,-0.333233134534162,0.94284446121751));
#54800=DIRECTION('ref_axis',(0.,-0.94284446121751,-0.333233134534162));
#54801=DIRECTION('center_axis',(0.,0.333233134534159,-0.942844461217511));
#54802=DIRECTION('ref_axis',(0.,-0.942844461217511,-0.333233134534159));
#54803=DIRECTION('',(0.,0.333233134534162,-0.94284446121751));
#54804=DIRECTION('center_axis',(0.,0.333233134534162,-0.94284446121751));
#54805=DIRECTION('ref_axis',(0.,-0.94284446121751,-0.333233134534162));
#54806=DIRECTION('center_axis',(0.,-0.333233134534162,0.94284446121751));
#54807=DIRECTION('ref_axis',(0.,-0.94284446121751,-0.333233134534162));
#54808=DIRECTION('center_axis',(0.,0.333233134534162,-0.94284446121751));
#54809=DIRECTION('ref_axis',(0.,0.94284446121751,0.333233134534162));
#54810=DIRECTION('',(0.,-0.333233134534162,0.94284446121751));
#54811=DIRECTION('center_axis',(0.,0.333233134534159,-0.942844461217511));
#54812=DIRECTION('ref_axis',(0.,-0.942844461217511,-0.333233134534159));
#54813=DIRECTION('center_axis',(0.,-0.333233134534162,0.94284446121751));
#54814=DIRECTION('ref_axis',(0.,-0.94284446121751,-0.333233134534162));
#54815=DIRECTION('center_axis',(0.,0.333233134534159,-0.942844461217511));
#54816=DIRECTION('ref_axis',(0.,-0.942844461217511,-0.333233134534159));
#54817=DIRECTION('',(0.,0.333233134534162,-0.94284446121751));
#54818=DIRECTION('center_axis',(0.,0.333233134534162,-0.94284446121751));
#54819=DIRECTION('ref_axis',(0.,-0.94284446121751,-0.333233134534162));
#54820=DIRECTION('center_axis',(0.,-0.333233134534162,0.94284446121751));
#54821=DIRECTION('ref_axis',(0.,-0.94284446121751,-0.333233134534162));
#54822=DIRECTION('center_axis',(0.,0.333233134534162,-0.94284446121751));
#54823=DIRECTION('ref_axis',(0.,0.94284446121751,0.333233134534162));
#54824=DIRECTION('',(0.,-0.333233134534162,0.94284446121751));
#54825=DIRECTION('center_axis',(0.,0.333233134534159,-0.942844461217511));
#54826=DIRECTION('ref_axis',(0.,-0.942844461217511,-0.333233134534159));
#54827=DIRECTION('center_axis',(0.,-0.333233134534162,0.94284446121751));
#54828=DIRECTION('ref_axis',(0.,-0.94284446121751,-0.333233134534162));
#54829=DIRECTION('center_axis',(0.,0.333233134534159,-0.942844461217511));
#54830=DIRECTION('ref_axis',(0.,-0.942844461217511,-0.333233134534159));
#54831=DIRECTION('',(0.,0.333233134534162,-0.94284446121751));
#54832=DIRECTION('center_axis',(0.,0.333233134534162,-0.94284446121751));
#54833=DIRECTION('ref_axis',(0.,-0.94284446121751,-0.333233134534162));
#54834=DIRECTION('center_axis',(0.,-0.333233134534162,0.94284446121751));
#54835=DIRECTION('ref_axis',(0.,-0.94284446121751,-0.333233134534162));
#54836=DIRECTION('center_axis',(0.,0.333233134534162,-0.94284446121751));
#54837=DIRECTION('ref_axis',(0.,0.94284446121751,0.333233134534162));
#54838=DIRECTION('',(0.,-0.333233134534162,0.94284446121751));
#54839=DIRECTION('center_axis',(0.,0.333233134534159,-0.942844461217511));
#54840=DIRECTION('ref_axis',(0.,-0.942844461217511,-0.333233134534159));
#54841=DIRECTION('center_axis',(0.,-0.333233134534162,0.94284446121751));
#54842=DIRECTION('ref_axis',(0.,-0.94284446121751,-0.333233134534162));
#54843=DIRECTION('center_axis',(0.,0.333233134534159,-0.942844461217511));
#54844=DIRECTION('ref_axis',(0.,-0.942844461217511,-0.333233134534159));
#54845=DIRECTION('',(0.,0.333233134534162,-0.94284446121751));
#54846=DIRECTION('center_axis',(0.,0.333233134534162,-0.94284446121751));
#54847=DIRECTION('ref_axis',(0.,-0.94284446121751,-0.333233134534162));
#54848=DIRECTION('center_axis',(0.,-0.333233134534162,0.94284446121751));
#54849=DIRECTION('ref_axis',(0.,-0.94284446121751,-0.333233134534162));
#54850=DIRECTION('center_axis',(0.,0.333233134534162,-0.94284446121751));
#54851=DIRECTION('ref_axis',(0.,0.94284446121751,0.333233134534162));
#54852=DIRECTION('',(0.,-0.333233134534162,0.94284446121751));
#54853=DIRECTION('center_axis',(0.,0.333233134534159,-0.942844461217511));
#54854=DIRECTION('ref_axis',(0.,-0.942844461217511,-0.333233134534159));
#54855=DIRECTION('center_axis',(0.,-0.333233134534162,0.94284446121751));
#54856=DIRECTION('ref_axis',(0.,-0.94284446121751,-0.333233134534162));
#54857=DIRECTION('center_axis',(0.,0.333233134534159,-0.942844461217511));
#54858=DIRECTION('ref_axis',(0.,-0.942844461217511,-0.333233134534159));
#54859=DIRECTION('',(0.,0.333233134534162,-0.94284446121751));
#54860=DIRECTION('center_axis',(0.,0.333233134534162,-0.94284446121751));
#54861=DIRECTION('ref_axis',(0.,-0.94284446121751,-0.333233134534162));
#54862=DIRECTION('center_axis',(0.,-0.333233134534162,0.94284446121751));
#54863=DIRECTION('ref_axis',(0.,-0.94284446121751,-0.333233134534162));
#54864=DIRECTION('center_axis',(0.,0.333233134534162,-0.94284446121751));
#54865=DIRECTION('ref_axis',(0.,0.94284446121751,0.333233134534162));
#54866=DIRECTION('',(0.,-0.333233134534162,0.94284446121751));
#54867=DIRECTION('center_axis',(0.,0.333233134534159,-0.942844461217511));
#54868=DIRECTION('ref_axis',(0.,-0.942844461217511,-0.333233134534159));
#54869=DIRECTION('center_axis',(0.,-0.333233134534162,0.94284446121751));
#54870=DIRECTION('ref_axis',(0.,-0.94284446121751,-0.333233134534162));
#54871=DIRECTION('center_axis',(0.,0.333233134534159,-0.942844461217511));
#54872=DIRECTION('ref_axis',(0.,-0.942844461217511,-0.333233134534159));
#54873=DIRECTION('',(0.,0.333233134534162,-0.94284446121751));
#54874=DIRECTION('center_axis',(0.,-0.333233134534162,0.94284446121751));
#54875=DIRECTION('ref_axis',(0.,-0.94284446121751,-0.333233134534162));
#54876=DIRECTION('center_axis',(0.,-0.333233134534162,0.94284446121751));
#54877=DIRECTION('ref_axis',(0.,-0.94284446121751,-0.333233134534162));
#54878=DIRECTION('center_axis',(0.,-0.333233134534162,0.94284446121751));
#54879=DIRECTION('ref_axis',(0.,-0.94284446121751,-0.333233134534162));
#54880=DIRECTION('center_axis',(0.,0.333233134534162,-0.94284446121751));
#54881=DIRECTION('ref_axis',(0.,0.94284446121751,0.333233134534162));
#54882=DIRECTION('',(0.,-0.333233134534162,0.94284446121751));
#54883=DIRECTION('center_axis',(0.,0.333233134534159,-0.942844461217511));
#54884=DIRECTION('ref_axis',(0.,-0.942844461217511,-0.333233134534159));
#54885=DIRECTION('center_axis',(0.,-0.333233134534162,0.94284446121751));
#54886=DIRECTION('ref_axis',(0.,-0.94284446121751,-0.333233134534161));
#54887=DIRECTION('center_axis',(0.,0.333233134534159,-0.942844461217511));
#54888=DIRECTION('ref_axis',(0.,-0.942844461217511,-0.333233134534159));
#54889=DIRECTION('',(0.,0.333233134534162,-0.94284446121751));
#54890=DIRECTION('center_axis',(0.,0.333233134534162,-0.94284446121751));
#54891=DIRECTION('ref_axis',(0.,-0.94284446121751,-0.333233134534162));
#54892=DIRECTION('center_axis',(0.,-0.333233134534162,0.94284446121751));
#54893=DIRECTION('ref_axis',(0.,-0.94284446121751,-0.333233134534162));
#54894=DIRECTION('center_axis',(0.,0.333233134534162,-0.94284446121751));
#54895=DIRECTION('ref_axis',(0.,0.94284446121751,0.333233134534162));
#54896=DIRECTION('',(0.,-0.333233134534162,0.94284446121751));
#54897=DIRECTION('center_axis',(0.,0.333233134534159,-0.942844461217511));
#54898=DIRECTION('ref_axis',(0.,-0.942844461217511,-0.333233134534159));
#54899=DIRECTION('center_axis',(0.,-0.333233134534162,0.94284446121751));
#54900=DIRECTION('ref_axis',(0.,-0.94284446121751,-0.333233134534162));
#54901=DIRECTION('center_axis',(0.,0.333233134534159,-0.942844461217511));
#54902=DIRECTION('ref_axis',(0.,-0.942844461217511,-0.333233134534159));
#54903=DIRECTION('',(0.,0.333233134534162,-0.94284446121751));
#54904=DIRECTION('center_axis',(0.,0.333233134534162,-0.94284446121751));
#54905=DIRECTION('ref_axis',(0.,-0.94284446121751,-0.333233134534162));
#54906=DIRECTION('center_axis',(0.,-0.333233134534162,0.94284446121751));
#54907=DIRECTION('ref_axis',(0.,-0.94284446121751,-0.333233134534162));
#54908=DIRECTION('center_axis',(0.,0.333233134534162,-0.94284446121751));
#54909=DIRECTION('ref_axis',(0.,0.94284446121751,0.333233134534162));
#54910=DIRECTION('',(0.,-0.333233134534162,0.94284446121751));
#54911=DIRECTION('center_axis',(0.,0.333233134534159,-0.942844461217511));
#54912=DIRECTION('ref_axis',(0.,-0.942844461217511,-0.333233134534159));
#54913=DIRECTION('center_axis',(0.,-0.333233134534162,0.94284446121751));
#54914=DIRECTION('ref_axis',(0.,-0.94284446121751,-0.333233134534161));
#54915=DIRECTION('center_axis',(0.,0.333233134534159,-0.942844461217511));
#54916=DIRECTION('ref_axis',(0.,-0.942844461217511,-0.333233134534159));
#54917=DIRECTION('',(0.,0.333233134534162,-0.94284446121751));
#54918=DIRECTION('center_axis',(0.,0.333233134534162,-0.94284446121751));
#54919=DIRECTION('ref_axis',(0.,-0.94284446121751,-0.333233134534162));
#54920=DIRECTION('center_axis',(0.,-0.333233134534162,0.94284446121751));
#54921=DIRECTION('ref_axis',(0.,-0.94284446121751,-0.333233134534162));
#54922=DIRECTION('center_axis',(0.,0.333233134534162,-0.94284446121751));
#54923=DIRECTION('ref_axis',(0.,0.94284446121751,0.333233134534162));
#54924=DIRECTION('',(0.,-0.333233134534162,0.94284446121751));
#54925=DIRECTION('center_axis',(0.,0.333233134534159,-0.942844461217511));
#54926=DIRECTION('ref_axis',(0.,-0.942844461217511,-0.333233134534159));
#54927=DIRECTION('center_axis',(0.,-0.333233134534162,0.94284446121751));
#54928=DIRECTION('ref_axis',(0.,-0.94284446121751,-0.333233134534162));
#54929=DIRECTION('center_axis',(0.,0.333233134534159,-0.942844461217511));
#54930=DIRECTION('ref_axis',(0.,-0.942844461217511,-0.333233134534159));
#54931=DIRECTION('',(0.,0.333233134534162,-0.94284446121751));
#54932=DIRECTION('center_axis',(0.,0.333233134534162,-0.94284446121751));
#54933=DIRECTION('ref_axis',(0.,-0.94284446121751,-0.333233134534162));
#54934=DIRECTION('center_axis',(0.,-0.333233134534162,0.94284446121751));
#54935=DIRECTION('ref_axis',(0.,-0.94284446121751,-0.333233134534162));
#54936=DIRECTION('center_axis',(0.,0.333233134534162,-0.94284446121751));
#54937=DIRECTION('ref_axis',(0.,0.94284446121751,0.333233134534162));
#54938=DIRECTION('',(0.,-0.333233134534162,0.94284446121751));
#54939=DIRECTION('center_axis',(0.,0.333233134534159,-0.942844461217511));
#54940=DIRECTION('ref_axis',(0.,-0.942844461217511,-0.333233134534159));
#54941=DIRECTION('center_axis',(0.,-0.333233134534162,0.94284446121751));
#54942=DIRECTION('ref_axis',(0.,-0.94284446121751,-0.333233134534162));
#54943=DIRECTION('center_axis',(0.,0.333233134534159,-0.942844461217511));
#54944=DIRECTION('ref_axis',(0.,-0.942844461217511,-0.333233134534159));
#54945=DIRECTION('',(0.,0.333233134534162,-0.94284446121751));
#54946=DIRECTION('center_axis',(0.,0.333233134534162,-0.94284446121751));
#54947=DIRECTION('ref_axis',(0.,-0.94284446121751,-0.333233134534162));
#54948=DIRECTION('center_axis',(0.,-0.333233134534162,0.94284446121751));
#54949=DIRECTION('ref_axis',(0.,-0.94284446121751,-0.333233134534162));
#54950=DIRECTION('center_axis',(0.,0.333233134534162,-0.94284446121751));
#54951=DIRECTION('ref_axis',(0.,0.94284446121751,0.333233134534162));
#54952=DIRECTION('',(0.,-0.333233134534162,0.94284446121751));
#54953=DIRECTION('center_axis',(0.,0.333233134534159,-0.942844461217511));
#54954=DIRECTION('ref_axis',(0.,-0.942844461217511,-0.333233134534159));
#54955=DIRECTION('center_axis',(0.,-0.333233134534162,0.94284446121751));
#54956=DIRECTION('ref_axis',(0.,-0.94284446121751,-0.333233134534162));
#54957=DIRECTION('center_axis',(0.,0.333233134534159,-0.942844461217511));
#54958=DIRECTION('ref_axis',(0.,-0.942844461217511,-0.333233134534159));
#54959=DIRECTION('',(0.,0.333233134534162,-0.94284446121751));
#54960=DIRECTION('center_axis',(0.,0.333233134534162,-0.94284446121751));
#54961=DIRECTION('ref_axis',(0.,-0.94284446121751,-0.333233134534162));
#54962=DIRECTION('center_axis',(0.,-0.333233134534162,0.94284446121751));
#54963=DIRECTION('ref_axis',(0.,-0.94284446121751,-0.333233134534162));
#54964=DIRECTION('center_axis',(0.,0.333233134534162,-0.94284446121751));
#54965=DIRECTION('ref_axis',(0.,0.94284446121751,0.333233134534162));
#54966=DIRECTION('',(0.,-0.333233134534162,0.94284446121751));
#54967=DIRECTION('center_axis',(0.,0.333233134534159,-0.942844461217511));
#54968=DIRECTION('ref_axis',(0.,-0.942844461217511,-0.333233134534159));
#54969=DIRECTION('center_axis',(0.,-0.333233134534162,0.94284446121751));
#54970=DIRECTION('ref_axis',(0.,-0.94284446121751,-0.333233134534162));
#54971=DIRECTION('center_axis',(0.,0.333233134534159,-0.942844461217511));
#54972=DIRECTION('ref_axis',(0.,-0.942844461217511,-0.333233134534159));
#54973=DIRECTION('',(0.,0.333233134534162,-0.94284446121751));
#54974=DIRECTION('center_axis',(0.,0.333233134534162,-0.94284446121751));
#54975=DIRECTION('ref_axis',(0.,-0.94284446121751,-0.333233134534162));
#54976=DIRECTION('center_axis',(0.,-0.333233134534162,0.94284446121751));
#54977=DIRECTION('ref_axis',(0.,-0.94284446121751,-0.333233134534162));
#54978=DIRECTION('center_axis',(0.,0.333233134534162,-0.94284446121751));
#54979=DIRECTION('ref_axis',(0.,0.94284446121751,0.333233134534162));
#54980=DIRECTION('',(0.,-0.333233134534162,0.94284446121751));
#54981=DIRECTION('center_axis',(0.,0.333233134534159,-0.942844461217511));
#54982=DIRECTION('ref_axis',(0.,-0.942844461217511,-0.333233134534159));
#54983=DIRECTION('center_axis',(0.,-0.333233134534162,0.94284446121751));
#54984=DIRECTION('ref_axis',(0.,-0.94284446121751,-0.333233134534161));
#54985=DIRECTION('center_axis',(0.,0.333233134534159,-0.942844461217511));
#54986=DIRECTION('ref_axis',(0.,-0.942844461217511,-0.333233134534159));
#54987=DIRECTION('',(0.,0.333233134534162,-0.94284446121751));
#54988=DIRECTION('center_axis',(0.,0.333233134534162,-0.94284446121751));
#54989=DIRECTION('ref_axis',(0.,-0.94284446121751,-0.333233134534162));
#54990=DIRECTION('center_axis',(0.,-0.333233134534162,0.94284446121751));
#54991=DIRECTION('ref_axis',(0.,-0.94284446121751,-0.333233134534162));
#54992=DIRECTION('center_axis',(0.,0.333233134534162,-0.94284446121751));
#54993=DIRECTION('ref_axis',(0.,0.94284446121751,0.333233134534162));
#54994=DIRECTION('',(0.,-0.333233134534162,0.94284446121751));
#54995=DIRECTION('center_axis',(0.,0.333233134534159,-0.942844461217511));
#54996=DIRECTION('ref_axis',(0.,-0.942844461217511,-0.333233134534159));
#54997=DIRECTION('center_axis',(0.,-0.333233134534162,0.94284446121751));
#54998=DIRECTION('ref_axis',(0.,-0.94284446121751,-0.333233134534162));
#54999=DIRECTION('center_axis',(0.,0.333233134534159,-0.942844461217511));
#55000=DIRECTION('ref_axis',(0.,-0.942844461217511,-0.333233134534159));
#55001=DIRECTION('',(0.,0.333233134534162,-0.94284446121751));
#55002=DIRECTION('center_axis',(0.,0.333233134534162,-0.94284446121751));
#55003=DIRECTION('ref_axis',(0.,-0.94284446121751,-0.333233134534162));
#55004=DIRECTION('center_axis',(0.,-0.333233134534162,0.94284446121751));
#55005=DIRECTION('ref_axis',(0.,-0.94284446121751,-0.333233134534162));
#55006=DIRECTION('center_axis',(0.,0.333233134534162,-0.94284446121751));
#55007=DIRECTION('ref_axis',(0.,0.94284446121751,0.333233134534162));
#55008=DIRECTION('',(0.,-0.333233134534162,0.94284446121751));
#55009=DIRECTION('center_axis',(0.,0.333233134534159,-0.942844461217511));
#55010=DIRECTION('ref_axis',(0.,-0.942844461217511,-0.333233134534159));
#55011=DIRECTION('center_axis',(0.,-0.333233134534162,0.94284446121751));
#55012=DIRECTION('ref_axis',(0.,-0.94284446121751,-0.333233134534162));
#55013=DIRECTION('center_axis',(0.,0.333233134534159,-0.942844461217511));
#55014=DIRECTION('ref_axis',(0.,-0.942844461217511,-0.333233134534159));
#55015=DIRECTION('',(0.,0.333233134534162,-0.94284446121751));
#55016=DIRECTION('center_axis',(0.,0.333233134534162,-0.94284446121751));
#55017=DIRECTION('ref_axis',(0.,-0.94284446121751,-0.333233134534162));
#55018=DIRECTION('center_axis',(0.,-0.333233134534162,0.94284446121751));
#55019=DIRECTION('ref_axis',(0.,-0.94284446121751,-0.333233134534162));
#55020=DIRECTION('center_axis',(0.,0.333233134534162,-0.94284446121751));
#55021=DIRECTION('ref_axis',(0.,0.94284446121751,0.333233134534162));
#55022=DIRECTION('',(0.,-0.333233134534162,0.94284446121751));
#55023=DIRECTION('center_axis',(0.,0.333233134534159,-0.942844461217511));
#55024=DIRECTION('ref_axis',(0.,-0.942844461217511,-0.333233134534159));
#55025=DIRECTION('center_axis',(0.,-0.333233134534162,0.94284446121751));
#55026=DIRECTION('ref_axis',(0.,-0.94284446121751,-0.333233134534162));
#55027=DIRECTION('center_axis',(0.,0.333233134534159,-0.942844461217511));
#55028=DIRECTION('ref_axis',(0.,-0.942844461217511,-0.333233134534159));
#55029=DIRECTION('',(0.,0.333233134534162,-0.94284446121751));
#55030=DIRECTION('center_axis',(0.,0.333233134534162,-0.94284446121751));
#55031=DIRECTION('ref_axis',(0.,-0.94284446121751,-0.333233134534162));
#55032=DIRECTION('center_axis',(0.,-0.333233134534162,0.94284446121751));
#55033=DIRECTION('ref_axis',(0.,-0.94284446121751,-0.333233134534162));
#55034=DIRECTION('center_axis',(0.,0.333233134534162,-0.94284446121751));
#55035=DIRECTION('ref_axis',(0.,0.94284446121751,0.333233134534162));
#55036=DIRECTION('',(0.,-0.333233134534162,0.94284446121751));
#55037=DIRECTION('center_axis',(0.,0.333233134534159,-0.942844461217511));
#55038=DIRECTION('ref_axis',(0.,-0.942844461217511,-0.333233134534159));
#55039=DIRECTION('center_axis',(0.,-0.333233134534162,0.94284446121751));
#55040=DIRECTION('ref_axis',(0.,-0.94284446121751,-0.333233134534162));
#55041=DIRECTION('center_axis',(0.,0.333233134534159,-0.942844461217511));
#55042=DIRECTION('ref_axis',(0.,-0.942844461217511,-0.333233134534159));
#55043=DIRECTION('',(0.,0.333233134534162,-0.94284446121751));
#55044=DIRECTION('center_axis',(0.,0.333233134534162,-0.94284446121751));
#55045=DIRECTION('ref_axis',(0.,-0.94284446121751,-0.333233134534162));
#55046=DIRECTION('center_axis',(0.,-0.333233134534162,0.94284446121751));
#55047=DIRECTION('ref_axis',(0.,-0.94284446121751,-0.333233134534162));
#55048=DIRECTION('center_axis',(0.,0.333233134534162,-0.94284446121751));
#55049=DIRECTION('ref_axis',(0.,0.94284446121751,0.333233134534162));
#55050=DIRECTION('',(0.,-0.333233134534162,0.94284446121751));
#55051=DIRECTION('center_axis',(0.,0.333233134534159,-0.942844461217511));
#55052=DIRECTION('ref_axis',(0.,-0.942844461217511,-0.333233134534159));
#55053=DIRECTION('center_axis',(0.,-0.333233134534162,0.94284446121751));
#55054=DIRECTION('ref_axis',(0.,-0.94284446121751,-0.333233134534162));
#55055=DIRECTION('center_axis',(0.,0.333233134534159,-0.942844461217511));
#55056=DIRECTION('ref_axis',(0.,-0.942844461217511,-0.333233134534159));
#55057=DIRECTION('',(0.,0.333233134534162,-0.94284446121751));
#55058=DIRECTION('center_axis',(0.,0.333233134534162,-0.94284446121751));
#55059=DIRECTION('ref_axis',(0.,-0.94284446121751,-0.333233134534162));
#55060=DIRECTION('center_axis',(0.,-0.333233134534162,0.94284446121751));
#55061=DIRECTION('ref_axis',(0.,-0.94284446121751,-0.333233134534162));
#55062=DIRECTION('center_axis',(0.,0.333233134534162,-0.94284446121751));
#55063=DIRECTION('ref_axis',(0.,0.94284446121751,0.333233134534162));
#55064=DIRECTION('',(0.,-0.333233134534162,0.94284446121751));
#55065=DIRECTION('center_axis',(0.,0.333233134534159,-0.942844461217511));
#55066=DIRECTION('ref_axis',(0.,-0.942844461217511,-0.333233134534159));
#55067=DIRECTION('center_axis',(0.,-0.333233134534162,0.94284446121751));
#55068=DIRECTION('ref_axis',(0.,-0.94284446121751,-0.333233134534162));
#55069=DIRECTION('center_axis',(0.,0.333233134534159,-0.942844461217511));
#55070=DIRECTION('ref_axis',(0.,-0.942844461217511,-0.333233134534159));
#55071=DIRECTION('',(0.,0.333233134534162,-0.94284446121751));
#55072=DIRECTION('center_axis',(0.,-0.333233134534162,0.94284446121751));
#55073=DIRECTION('ref_axis',(0.,-0.94284446121751,-0.333233134534162));
#55074=DIRECTION('center_axis',(0.,-0.333233134534162,0.94284446121751));
#55075=DIRECTION('ref_axis',(0.,-0.94284446121751,-0.333233134534162));
#55076=DIRECTION('center_axis',(0.,-0.333233134534162,0.94284446121751));
#55077=DIRECTION('ref_axis',(0.,-0.94284446121751,-0.333233134534162));
#55078=DIRECTION('center_axis',(0.,0.333233134534162,-0.94284446121751));
#55079=DIRECTION('ref_axis',(0.,0.94284446121751,0.333233134534162));
#55080=DIRECTION('',(0.,-0.333233134534162,0.94284446121751));
#55081=DIRECTION('center_axis',(0.,0.333233134534159,-0.942844461217511));
#55082=DIRECTION('ref_axis',(0.,-0.942844461217511,-0.333233134534159));
#55083=DIRECTION('center_axis',(0.,-0.333233134534162,0.94284446121751));
#55084=DIRECTION('ref_axis',(0.,-0.94284446121751,-0.333233134534162));
#55085=DIRECTION('center_axis',(0.,0.333233134534159,-0.942844461217511));
#55086=DIRECTION('ref_axis',(0.,-0.942844461217511,-0.333233134534159));
#55087=DIRECTION('',(0.,0.333233134534162,-0.94284446121751));
#55088=DIRECTION('center_axis',(0.,0.333233134534162,-0.94284446121751));
#55089=DIRECTION('ref_axis',(0.,-0.94284446121751,-0.333233134534162));
#55090=DIRECTION('center_axis',(0.,-0.333233134534162,0.94284446121751));
#55091=DIRECTION('ref_axis',(0.,-0.94284446121751,-0.333233134534162));
#55092=DIRECTION('center_axis',(0.,0.333233134534162,-0.94284446121751));
#55093=DIRECTION('ref_axis',(0.,0.94284446121751,0.333233134534162));
#55094=DIRECTION('',(0.,-0.333233134534162,0.94284446121751));
#55095=DIRECTION('center_axis',(0.,0.333233134534159,-0.942844461217511));
#55096=DIRECTION('ref_axis',(0.,-0.942844461217511,-0.333233134534159));
#55097=DIRECTION('center_axis',(0.,-0.333233134534162,0.94284446121751));
#55098=DIRECTION('ref_axis',(0.,-0.94284446121751,-0.333233134534162));
#55099=DIRECTION('center_axis',(0.,0.333233134534159,-0.942844461217511));
#55100=DIRECTION('ref_axis',(0.,-0.942844461217511,-0.333233134534159));
#55101=DIRECTION('',(0.,0.333233134534162,-0.94284446121751));
#55102=DIRECTION('center_axis',(0.,0.333233134534162,-0.94284446121751));
#55103=DIRECTION('ref_axis',(0.,-0.94284446121751,-0.333233134534162));
#55104=DIRECTION('center_axis',(0.,-0.333233134534162,0.94284446121751));
#55105=DIRECTION('ref_axis',(0.,-0.94284446121751,-0.333233134534162));
#55106=DIRECTION('center_axis',(0.,0.333233134534162,-0.94284446121751));
#55107=DIRECTION('ref_axis',(0.,0.94284446121751,0.333233134534162));
#55108=DIRECTION('',(0.,-0.333233134534162,0.94284446121751));
#55109=DIRECTION('center_axis',(0.,0.333233134534159,-0.942844461217511));
#55110=DIRECTION('ref_axis',(0.,-0.942844461217511,-0.333233134534159));
#55111=DIRECTION('center_axis',(0.,-0.333233134534162,0.94284446121751));
#55112=DIRECTION('ref_axis',(0.,-0.94284446121751,-0.333233134534161));
#55113=DIRECTION('center_axis',(0.,0.333233134534159,-0.942844461217511));
#55114=DIRECTION('ref_axis',(0.,-0.942844461217511,-0.333233134534159));
#55115=DIRECTION('',(0.,0.333233134534162,-0.94284446121751));
#55116=DIRECTION('center_axis',(0.,0.333233134534162,-0.94284446121751));
#55117=DIRECTION('ref_axis',(0.,-0.94284446121751,-0.333233134534162));
#55118=DIRECTION('center_axis',(0.,-0.333233134534162,0.94284446121751));
#55119=DIRECTION('ref_axis',(0.,-0.94284446121751,-0.333233134534162));
#55120=DIRECTION('center_axis',(0.,0.333233134534162,-0.94284446121751));
#55121=DIRECTION('ref_axis',(0.,0.94284446121751,0.333233134534162));
#55122=DIRECTION('',(0.,-0.333233134534162,0.94284446121751));
#55123=DIRECTION('center_axis',(0.,0.333233134534159,-0.942844461217511));
#55124=DIRECTION('ref_axis',(0.,-0.942844461217511,-0.333233134534159));
#55125=DIRECTION('center_axis',(0.,-0.333233134534162,0.94284446121751));
#55126=DIRECTION('ref_axis',(0.,-0.94284446121751,-0.333233134534162));
#55127=DIRECTION('center_axis',(0.,0.333233134534159,-0.942844461217511));
#55128=DIRECTION('ref_axis',(0.,-0.942844461217511,-0.333233134534159));
#55129=DIRECTION('',(0.,0.333233134534162,-0.94284446121751));
#55130=DIRECTION('center_axis',(0.,0.333233134534162,-0.94284446121751));
#55131=DIRECTION('ref_axis',(0.,-0.94284446121751,-0.333233134534162));
#55132=DIRECTION('center_axis',(0.,-0.333233134534162,0.94284446121751));
#55133=DIRECTION('ref_axis',(0.,-0.94284446121751,-0.333233134534162));
#55134=DIRECTION('center_axis',(0.,0.333233134534162,-0.94284446121751));
#55135=DIRECTION('ref_axis',(0.,0.94284446121751,0.333233134534162));
#55136=DIRECTION('',(0.,-0.333233134534162,0.94284446121751));
#55137=DIRECTION('center_axis',(0.,0.333233134534159,-0.942844461217511));
#55138=DIRECTION('ref_axis',(0.,-0.942844461217511,-0.333233134534159));
#55139=DIRECTION('center_axis',(0.,-0.333233134534162,0.94284446121751));
#55140=DIRECTION('ref_axis',(0.,-0.94284446121751,-0.333233134534162));
#55141=DIRECTION('center_axis',(0.,0.333233134534159,-0.942844461217511));
#55142=DIRECTION('ref_axis',(0.,-0.942844461217511,-0.333233134534159));
#55143=DIRECTION('',(0.,0.333233134534162,-0.94284446121751));
#55144=DIRECTION('center_axis',(0.,0.333233134534162,-0.94284446121751));
#55145=DIRECTION('ref_axis',(0.,-0.94284446121751,-0.333233134534162));
#55146=DIRECTION('center_axis',(0.,-0.333233134534162,0.94284446121751));
#55147=DIRECTION('ref_axis',(0.,-0.94284446121751,-0.333233134534162));
#55148=DIRECTION('center_axis',(0.,0.333233134534162,-0.94284446121751));
#55149=DIRECTION('ref_axis',(0.,0.94284446121751,0.333233134534162));
#55150=DIRECTION('',(0.,-0.333233134534162,0.94284446121751));
#55151=DIRECTION('center_axis',(0.,0.333233134534159,-0.942844461217511));
#55152=DIRECTION('ref_axis',(0.,-0.942844461217511,-0.333233134534159));
#55153=DIRECTION('center_axis',(0.,-0.333233134534162,0.94284446121751));
#55154=DIRECTION('ref_axis',(0.,-0.94284446121751,-0.333233134534162));
#55155=DIRECTION('center_axis',(0.,0.333233134534159,-0.942844461217511));
#55156=DIRECTION('ref_axis',(0.,-0.942844461217511,-0.333233134534159));
#55157=DIRECTION('',(0.,0.333233134534162,-0.94284446121751));
#55158=DIRECTION('center_axis',(0.,0.333233134534162,-0.94284446121751));
#55159=DIRECTION('ref_axis',(0.,-0.94284446121751,-0.333233134534162));
#55160=DIRECTION('center_axis',(0.,-0.333233134534162,0.94284446121751));
#55161=DIRECTION('ref_axis',(0.,-0.94284446121751,-0.333233134534162));
#55162=DIRECTION('center_axis',(0.,0.333233134534162,-0.94284446121751));
#55163=DIRECTION('ref_axis',(0.,0.94284446121751,0.333233134534162));
#55164=DIRECTION('',(0.,-0.333233134534162,0.94284446121751));
#55165=DIRECTION('center_axis',(0.,0.333233134534159,-0.942844461217511));
#55166=DIRECTION('ref_axis',(0.,-0.942844461217511,-0.333233134534159));
#55167=DIRECTION('center_axis',(0.,-0.333233134534162,0.94284446121751));
#55168=DIRECTION('ref_axis',(0.,-0.94284446121751,-0.333233134534162));
#55169=DIRECTION('center_axis',(0.,0.333233134534159,-0.942844461217511));
#55170=DIRECTION('ref_axis',(0.,-0.942844461217511,-0.333233134534159));
#55171=DIRECTION('',(0.,0.333233134534162,-0.94284446121751));
#55172=DIRECTION('center_axis',(0.,0.333233134534162,-0.94284446121751));
#55173=DIRECTION('ref_axis',(0.,-0.94284446121751,-0.333233134534162));
#55174=DIRECTION('center_axis',(0.,-0.333233134534162,0.94284446121751));
#55175=DIRECTION('ref_axis',(0.,-0.94284446121751,-0.333233134534162));
#55176=DIRECTION('center_axis',(0.,0.333233134534162,-0.94284446121751));
#55177=DIRECTION('ref_axis',(0.,0.94284446121751,0.333233134534162));
#55178=DIRECTION('',(0.,-0.333233134534162,0.94284446121751));
#55179=DIRECTION('center_axis',(0.,0.333233134534159,-0.942844461217511));
#55180=DIRECTION('ref_axis',(0.,-0.942844461217511,-0.333233134534159));
#55181=DIRECTION('center_axis',(0.,-0.333233134534162,0.94284446121751));
#55182=DIRECTION('ref_axis',(0.,-0.94284446121751,-0.333233134534162));
#55183=DIRECTION('center_axis',(0.,0.333233134534159,-0.942844461217511));
#55184=DIRECTION('ref_axis',(0.,-0.942844461217511,-0.333233134534159));
#55185=DIRECTION('',(0.,0.333233134534162,-0.94284446121751));
#55186=DIRECTION('center_axis',(0.,0.333233134534162,-0.94284446121751));
#55187=DIRECTION('ref_axis',(0.,-0.94284446121751,-0.333233134534162));
#55188=DIRECTION('center_axis',(0.,-0.333233134534162,0.94284446121751));
#55189=DIRECTION('ref_axis',(0.,-0.94284446121751,-0.333233134534162));
#55190=DIRECTION('center_axis',(0.,0.333233134534162,-0.94284446121751));
#55191=DIRECTION('ref_axis',(0.,0.94284446121751,0.333233134534162));
#55192=DIRECTION('',(0.,-0.333233134534162,0.94284446121751));
#55193=DIRECTION('center_axis',(0.,0.333233134534159,-0.942844461217511));
#55194=DIRECTION('ref_axis',(0.,-0.942844461217511,-0.333233134534159));
#55195=DIRECTION('center_axis',(0.,-0.333233134534162,0.94284446121751));
#55196=DIRECTION('ref_axis',(0.,-0.94284446121751,-0.333233134534162));
#55197=DIRECTION('center_axis',(0.,0.333233134534159,-0.942844461217511));
#55198=DIRECTION('ref_axis',(0.,-0.942844461217511,-0.333233134534159));
#55199=DIRECTION('',(0.,0.333233134534162,-0.94284446121751));
#55200=DIRECTION('center_axis',(0.,0.333233134534162,-0.94284446121751));
#55201=DIRECTION('ref_axis',(0.,-0.94284446121751,-0.333233134534162));
#55202=DIRECTION('center_axis',(0.,-0.333233134534162,0.94284446121751));
#55203=DIRECTION('ref_axis',(0.,-0.94284446121751,-0.333233134534162));
#55204=DIRECTION('center_axis',(0.,0.333233134534162,-0.94284446121751));
#55205=DIRECTION('ref_axis',(0.,0.94284446121751,0.333233134534162));
#55206=DIRECTION('',(0.,-0.333233134534162,0.94284446121751));
#55207=DIRECTION('center_axis',(0.,0.333233134534159,-0.942844461217511));
#55208=DIRECTION('ref_axis',(0.,-0.942844461217511,-0.333233134534159));
#55209=DIRECTION('center_axis',(0.,-0.333233134534162,0.94284446121751));
#55210=DIRECTION('ref_axis',(0.,-0.94284446121751,-0.333233134534162));
#55211=DIRECTION('center_axis',(0.,0.333233134534159,-0.942844461217511));
#55212=DIRECTION('ref_axis',(0.,-0.942844461217511,-0.333233134534159));
#55213=DIRECTION('',(0.,0.333233134534162,-0.94284446121751));
#55214=DIRECTION('center_axis',(0.,0.333233134534162,-0.94284446121751));
#55215=DIRECTION('ref_axis',(0.,-0.94284446121751,-0.333233134534162));
#55216=DIRECTION('center_axis',(0.,-0.333233134534162,0.94284446121751));
#55217=DIRECTION('ref_axis',(0.,-0.94284446121751,-0.333233134534162));
#55218=DIRECTION('center_axis',(0.,0.333233134534162,-0.94284446121751));
#55219=DIRECTION('ref_axis',(0.,0.94284446121751,0.333233134534162));
#55220=DIRECTION('',(0.,-0.333233134534162,0.94284446121751));
#55221=DIRECTION('center_axis',(0.,0.333233134534159,-0.942844461217511));
#55222=DIRECTION('ref_axis',(0.,-0.942844461217511,-0.333233134534159));
#55223=DIRECTION('center_axis',(0.,-0.333233134534162,0.94284446121751));
#55224=DIRECTION('ref_axis',(0.,-0.94284446121751,-0.333233134534162));
#55225=DIRECTION('center_axis',(0.,0.333233134534159,-0.942844461217511));
#55226=DIRECTION('ref_axis',(0.,-0.942844461217511,-0.333233134534159));
#55227=DIRECTION('',(0.,0.333233134534162,-0.94284446121751));
#55228=DIRECTION('center_axis',(0.,0.333233134534162,-0.94284446121751));
#55229=DIRECTION('ref_axis',(0.,-0.94284446121751,-0.333233134534162));
#55230=DIRECTION('center_axis',(0.,-0.333233134534162,0.94284446121751));
#55231=DIRECTION('ref_axis',(0.,-0.94284446121751,-0.333233134534162));
#55232=DIRECTION('center_axis',(0.,0.333233134534162,-0.94284446121751));
#55233=DIRECTION('ref_axis',(0.,0.94284446121751,0.333233134534162));
#55234=DIRECTION('',(0.,-0.333233134534162,0.94284446121751));
#55235=DIRECTION('center_axis',(0.,0.333233134534159,-0.942844461217511));
#55236=DIRECTION('ref_axis',(0.,-0.942844461217511,-0.333233134534159));
#55237=DIRECTION('center_axis',(0.,-0.333233134534162,0.94284446121751));
#55238=DIRECTION('ref_axis',(0.,-0.94284446121751,-0.333233134534162));
#55239=DIRECTION('center_axis',(0.,0.333233134534159,-0.942844461217511));
#55240=DIRECTION('ref_axis',(0.,-0.942844461217511,-0.333233134534159));
#55241=DIRECTION('',(0.,0.333233134534162,-0.94284446121751));
#55242=DIRECTION('center_axis',(0.,0.333233134534162,-0.94284446121751));
#55243=DIRECTION('ref_axis',(0.,-0.94284446121751,-0.333233134534162));
#55244=DIRECTION('center_axis',(0.,-0.333233134534162,0.94284446121751));
#55245=DIRECTION('ref_axis',(0.,-0.94284446121751,-0.333233134534162));
#55246=DIRECTION('center_axis',(0.,0.333233134534162,-0.94284446121751));
#55247=DIRECTION('ref_axis',(0.,0.94284446121751,0.333233134534162));
#55248=DIRECTION('',(0.,-0.333233134534162,0.94284446121751));
#55249=DIRECTION('center_axis',(0.,0.333233134534159,-0.942844461217511));
#55250=DIRECTION('ref_axis',(0.,-0.942844461217511,-0.333233134534159));
#55251=DIRECTION('center_axis',(0.,-0.333233134534162,0.94284446121751));
#55252=DIRECTION('ref_axis',(0.,-0.94284446121751,-0.333233134534162));
#55253=DIRECTION('center_axis',(0.,0.333233134534159,-0.942844461217511));
#55254=DIRECTION('ref_axis',(0.,-0.942844461217511,-0.333233134534159));
#55255=DIRECTION('',(0.,0.333233134534162,-0.94284446121751));
#55256=DIRECTION('center_axis',(0.,0.333233134534162,-0.94284446121751));
#55257=DIRECTION('ref_axis',(0.,-0.94284446121751,-0.333233134534162));
#55258=DIRECTION('center_axis',(0.,-0.333233134534162,0.94284446121751));
#55259=DIRECTION('ref_axis',(0.,-0.94284446121751,-0.333233134534162));
#55260=DIRECTION('center_axis',(0.,0.333233134534162,-0.94284446121751));
#55261=DIRECTION('ref_axis',(0.,0.94284446121751,0.333233134534162));
#55262=DIRECTION('',(0.,-0.333233134534162,0.94284446121751));
#55263=DIRECTION('center_axis',(0.,0.333233134534159,-0.942844461217511));
#55264=DIRECTION('ref_axis',(0.,-0.942844461217511,-0.333233134534159));
#55265=DIRECTION('center_axis',(0.,-0.333233134534162,0.94284446121751));
#55266=DIRECTION('ref_axis',(0.,-0.94284446121751,-0.333233134534162));
#55267=DIRECTION('center_axis',(0.,0.333233134534159,-0.942844461217511));
#55268=DIRECTION('ref_axis',(0.,-0.942844461217511,-0.333233134534159));
#55269=DIRECTION('',(0.,0.333233134534162,-0.94284446121751));
#55270=DIRECTION('center_axis',(0.,0.333233134534162,-0.94284446121751));
#55271=DIRECTION('ref_axis',(0.,-0.94284446121751,-0.333233134534162));
#55272=DIRECTION('center_axis',(0.,-0.333233134534162,0.94284446121751));
#55273=DIRECTION('ref_axis',(0.,-0.94284446121751,-0.333233134534162));
#55274=DIRECTION('center_axis',(0.,0.333233134534162,-0.94284446121751));
#55275=DIRECTION('ref_axis',(0.,0.94284446121751,0.333233134534162));
#55276=DIRECTION('',(0.,-0.333233134534162,0.94284446121751));
#55277=DIRECTION('center_axis',(0.,0.333233134534159,-0.942844461217511));
#55278=DIRECTION('ref_axis',(0.,-0.942844461217511,-0.333233134534159));
#55279=DIRECTION('center_axis',(0.,-0.333233134534162,0.94284446121751));
#55280=DIRECTION('ref_axis',(0.,-0.94284446121751,-0.333233134534162));
#55281=DIRECTION('center_axis',(0.,0.333233134534159,-0.942844461217511));
#55282=DIRECTION('ref_axis',(0.,-0.942844461217511,-0.333233134534159));
#55283=DIRECTION('',(0.,0.333233134534162,-0.94284446121751));
#55284=DIRECTION('center_axis',(0.,0.333233134534162,-0.94284446121751));
#55285=DIRECTION('ref_axis',(0.,-0.94284446121751,-0.333233134534162));
#55286=DIRECTION('center_axis',(0.,-0.333233134534162,0.94284446121751));
#55287=DIRECTION('ref_axis',(0.,-0.94284446121751,-0.333233134534162));
#55288=DIRECTION('center_axis',(0.,0.333233134534162,-0.94284446121751));
#55289=DIRECTION('ref_axis',(0.,0.94284446121751,0.333233134534162));
#55290=DIRECTION('',(0.,-0.333233134534162,0.94284446121751));
#55291=DIRECTION('center_axis',(0.,0.333233134534159,-0.942844461217511));
#55292=DIRECTION('ref_axis',(0.,-0.942844461217511,-0.333233134534159));
#55293=DIRECTION('center_axis',(0.,-0.333233134534162,0.94284446121751));
#55294=DIRECTION('ref_axis',(0.,-0.94284446121751,-0.333233134534162));
#55295=DIRECTION('center_axis',(0.,0.333233134534159,-0.942844461217511));
#55296=DIRECTION('ref_axis',(0.,-0.942844461217511,-0.333233134534159));
#55297=DIRECTION('',(0.,0.333233134534162,-0.94284446121751));
#55298=DIRECTION('center_axis',(0.,0.333233134534162,-0.94284446121751));
#55299=DIRECTION('ref_axis',(0.,-0.94284446121751,-0.333233134534162));
#55300=DIRECTION('center_axis',(0.,-0.333233134534162,0.94284446121751));
#55301=DIRECTION('ref_axis',(0.,-0.94284446121751,-0.333233134534162));
#55302=DIRECTION('center_axis',(0.,0.333233134534162,-0.94284446121751));
#55303=DIRECTION('ref_axis',(0.,0.94284446121751,0.333233134534162));
#55304=DIRECTION('',(0.,-0.333233134534162,0.94284446121751));
#55305=DIRECTION('center_axis',(0.,0.333233134534159,-0.942844461217511));
#55306=DIRECTION('ref_axis',(0.,-0.942844461217511,-0.333233134534159));
#55307=DIRECTION('center_axis',(0.,-0.333233134534162,0.94284446121751));
#55308=DIRECTION('ref_axis',(0.,-0.94284446121751,-0.333233134534162));
#55309=DIRECTION('center_axis',(0.,0.333233134534159,-0.942844461217511));
#55310=DIRECTION('ref_axis',(0.,-0.942844461217511,-0.333233134534159));
#55311=DIRECTION('',(0.,0.333233134534162,-0.94284446121751));
#55312=DIRECTION('center_axis',(0.,-0.333233134534162,0.94284446121751));
#55313=DIRECTION('ref_axis',(0.,-0.94284446121751,-0.333233134534162));
#55314=DIRECTION('center_axis',(0.,-0.333233134534162,0.94284446121751));
#55315=DIRECTION('ref_axis',(0.,-0.94284446121751,-0.333233134534162));
#55316=DIRECTION('center_axis',(0.,-0.333233134534162,0.94284446121751));
#55317=DIRECTION('ref_axis',(0.,-0.94284446121751,-0.333233134534162));
#55318=DIRECTION('center_axis',(0.,0.333233134534162,-0.94284446121751));
#55319=DIRECTION('ref_axis',(0.,0.94284446121751,0.333233134534162));
#55320=DIRECTION('',(0.,-0.333233134534162,0.94284446121751));
#55321=DIRECTION('center_axis',(0.,0.333233134534159,-0.942844461217511));
#55322=DIRECTION('ref_axis',(0.,-0.942844461217511,-0.333233134534159));
#55323=DIRECTION('center_axis',(0.,-0.333233134534162,0.94284446121751));
#55324=DIRECTION('ref_axis',(0.,-0.94284446121751,-0.333233134534162));
#55325=DIRECTION('center_axis',(0.,0.333233134534159,-0.942844461217511));
#55326=DIRECTION('ref_axis',(0.,-0.942844461217511,-0.333233134534159));
#55327=DIRECTION('',(0.,0.333233134534162,-0.94284446121751));
#55328=DIRECTION('center_axis',(0.,0.333233134534162,-0.94284446121751));
#55329=DIRECTION('ref_axis',(0.,-0.94284446121751,-0.333233134534162));
#55330=DIRECTION('center_axis',(0.,-0.333233134534162,0.94284446121751));
#55331=DIRECTION('ref_axis',(0.,-0.94284446121751,-0.333233134534162));
#55332=DIRECTION('center_axis',(0.,0.333233134534162,-0.94284446121751));
#55333=DIRECTION('ref_axis',(0.,0.94284446121751,0.333233134534162));
#55334=DIRECTION('',(0.,-0.333233134534162,0.94284446121751));
#55335=DIRECTION('center_axis',(0.,0.333233134534159,-0.942844461217511));
#55336=DIRECTION('ref_axis',(0.,-0.942844461217511,-0.333233134534159));
#55337=DIRECTION('center_axis',(0.,-0.333233134534162,0.94284446121751));
#55338=DIRECTION('ref_axis',(0.,-0.94284446121751,-0.333233134534162));
#55339=DIRECTION('center_axis',(0.,0.333233134534159,-0.942844461217511));
#55340=DIRECTION('ref_axis',(0.,-0.942844461217511,-0.333233134534159));
#55341=DIRECTION('',(0.,0.333233134534162,-0.94284446121751));
#55342=DIRECTION('center_axis',(0.,0.333233134534162,-0.94284446121751));
#55343=DIRECTION('ref_axis',(0.,-0.94284446121751,-0.333233134534162));
#55344=DIRECTION('center_axis',(0.,-0.333233134534162,0.94284446121751));
#55345=DIRECTION('ref_axis',(0.,-0.94284446121751,-0.333233134534162));
#55346=DIRECTION('center_axis',(0.,0.333233134534162,-0.94284446121751));
#55347=DIRECTION('ref_axis',(0.,0.94284446121751,0.333233134534162));
#55348=DIRECTION('',(0.,-0.333233134534162,0.94284446121751));
#55349=DIRECTION('center_axis',(0.,0.333233134534159,-0.942844461217511));
#55350=DIRECTION('ref_axis',(0.,-0.942844461217511,-0.333233134534159));
#55351=DIRECTION('center_axis',(0.,-0.333233134534162,0.94284446121751));
#55352=DIRECTION('ref_axis',(0.,-0.94284446121751,-0.333233134534161));
#55353=DIRECTION('center_axis',(0.,0.333233134534159,-0.942844461217511));
#55354=DIRECTION('ref_axis',(0.,-0.942844461217511,-0.333233134534159));
#55355=DIRECTION('',(0.,0.333233134534162,-0.94284446121751));
#55356=DIRECTION('center_axis',(0.,0.333233134534162,-0.94284446121751));
#55357=DIRECTION('ref_axis',(0.,-0.94284446121751,-0.333233134534162));
#55358=DIRECTION('center_axis',(0.,-0.333233134534162,0.94284446121751));
#55359=DIRECTION('ref_axis',(0.,-0.94284446121751,-0.333233134534162));
#55360=DIRECTION('center_axis',(0.,0.333233134534162,-0.94284446121751));
#55361=DIRECTION('ref_axis',(0.,0.94284446121751,0.333233134534162));
#55362=DIRECTION('',(0.,-0.333233134534162,0.94284446121751));
#55363=DIRECTION('center_axis',(0.,0.333233134534159,-0.942844461217511));
#55364=DIRECTION('ref_axis',(0.,-0.942844461217511,-0.333233134534159));
#55365=DIRECTION('center_axis',(0.,-0.333233134534162,0.94284446121751));
#55366=DIRECTION('ref_axis',(0.,-0.94284446121751,-0.333233134534162));
#55367=DIRECTION('center_axis',(0.,0.333233134534159,-0.942844461217511));
#55368=DIRECTION('ref_axis',(0.,-0.942844461217511,-0.333233134534159));
#55369=DIRECTION('',(0.,0.333233134534162,-0.94284446121751));
#55370=DIRECTION('center_axis',(0.,0.333233134534162,-0.94284446121751));
#55371=DIRECTION('ref_axis',(0.,-0.94284446121751,-0.333233134534162));
#55372=DIRECTION('center_axis',(0.,-0.333233134534162,0.94284446121751));
#55373=DIRECTION('ref_axis',(0.,-0.94284446121751,-0.333233134534162));
#55374=DIRECTION('center_axis',(0.,0.333233134534162,-0.94284446121751));
#55375=DIRECTION('ref_axis',(0.,0.94284446121751,0.333233134534162));
#55376=DIRECTION('',(0.,-0.333233134534162,0.94284446121751));
#55377=DIRECTION('center_axis',(0.,0.333233134534159,-0.942844461217511));
#55378=DIRECTION('ref_axis',(0.,-0.942844461217511,-0.333233134534159));
#55379=DIRECTION('center_axis',(0.,-0.333233134534162,0.94284446121751));
#55380=DIRECTION('ref_axis',(0.,-0.94284446121751,-0.333233134534162));
#55381=DIRECTION('center_axis',(0.,0.333233134534159,-0.942844461217511));
#55382=DIRECTION('ref_axis',(0.,-0.942844461217511,-0.333233134534159));
#55383=DIRECTION('',(0.,0.333233134534162,-0.94284446121751));
#55384=DIRECTION('center_axis',(0.,0.333233134534162,-0.94284446121751));
#55385=DIRECTION('ref_axis',(0.,-0.94284446121751,-0.333233134534162));
#55386=DIRECTION('center_axis',(0.,-0.333233134534162,0.94284446121751));
#55387=DIRECTION('ref_axis',(0.,-0.94284446121751,-0.333233134534162));
#55388=DIRECTION('center_axis',(0.,0.333233134534162,-0.94284446121751));
#55389=DIRECTION('ref_axis',(0.,0.94284446121751,0.333233134534162));
#55390=DIRECTION('',(0.,-0.333233134534162,0.94284446121751));
#55391=DIRECTION('center_axis',(0.,0.333233134534159,-0.942844461217511));
#55392=DIRECTION('ref_axis',(0.,-0.942844461217511,-0.333233134534159));
#55393=DIRECTION('center_axis',(0.,-0.333233134534162,0.94284446121751));
#55394=DIRECTION('ref_axis',(0.,-0.94284446121751,-0.333233134534162));
#55395=DIRECTION('center_axis',(0.,0.333233134534159,-0.942844461217511));
#55396=DIRECTION('ref_axis',(0.,-0.942844461217511,-0.333233134534159));
#55397=DIRECTION('',(0.,0.333233134534162,-0.94284446121751));
#55398=DIRECTION('center_axis',(0.,0.333233134534162,-0.94284446121751));
#55399=DIRECTION('ref_axis',(0.,-0.94284446121751,-0.333233134534162));
#55400=DIRECTION('center_axis',(0.,-0.333233134534162,0.94284446121751));
#55401=DIRECTION('ref_axis',(0.,-0.94284446121751,-0.333233134534162));
#55402=DIRECTION('center_axis',(0.,0.333233134534162,-0.94284446121751));
#55403=DIRECTION('ref_axis',(0.,0.94284446121751,0.333233134534162));
#55404=DIRECTION('',(0.,-0.333233134534162,0.94284446121751));
#55405=DIRECTION('center_axis',(0.,0.333233134534159,-0.942844461217511));
#55406=DIRECTION('ref_axis',(0.,-0.942844461217511,-0.333233134534159));
#55407=DIRECTION('center_axis',(0.,-0.333233134534162,0.94284446121751));
#55408=DIRECTION('ref_axis',(0.,-0.94284446121751,-0.333233134534162));
#55409=DIRECTION('center_axis',(0.,0.333233134534159,-0.942844461217511));
#55410=DIRECTION('ref_axis',(0.,-0.942844461217511,-0.333233134534159));
#55411=DIRECTION('',(0.,0.333233134534162,-0.94284446121751));
#55412=DIRECTION('center_axis',(0.,0.333233134534162,-0.94284446121751));
#55413=DIRECTION('ref_axis',(0.,-0.94284446121751,-0.333233134534162));
#55414=DIRECTION('center_axis',(0.,-0.333233134534162,0.94284446121751));
#55415=DIRECTION('ref_axis',(0.,-0.94284446121751,-0.333233134534162));
#55416=DIRECTION('center_axis',(0.,0.333233134534162,-0.94284446121751));
#55417=DIRECTION('ref_axis',(0.,0.94284446121751,0.333233134534162));
#55418=DIRECTION('',(0.,-0.333233134534162,0.94284446121751));
#55419=DIRECTION('center_axis',(0.,0.333233134534159,-0.942844461217511));
#55420=DIRECTION('ref_axis',(0.,-0.942844461217511,-0.333233134534159));
#55421=DIRECTION('center_axis',(0.,-0.333233134534162,0.94284446121751));
#55422=DIRECTION('ref_axis',(0.,-0.94284446121751,-0.333233134534162));
#55423=DIRECTION('center_axis',(0.,0.333233134534159,-0.942844461217511));
#55424=DIRECTION('ref_axis',(0.,-0.942844461217511,-0.333233134534159));
#55425=DIRECTION('',(0.,0.333233134534162,-0.94284446121751));
#55426=DIRECTION('center_axis',(0.,0.333233134534162,-0.94284446121751));
#55427=DIRECTION('ref_axis',(0.,-0.94284446121751,-0.333233134534162));
#55428=DIRECTION('center_axis',(0.,-0.333233134534162,0.94284446121751));
#55429=DIRECTION('ref_axis',(0.,-0.94284446121751,-0.333233134534162));
#55430=DIRECTION('center_axis',(0.,0.333233134534162,-0.94284446121751));
#55431=DIRECTION('ref_axis',(0.,0.94284446121751,0.333233134534162));
#55432=DIRECTION('',(0.,-0.333233134534162,0.94284446121751));
#55433=DIRECTION('center_axis',(0.,0.333233134534159,-0.942844461217511));
#55434=DIRECTION('ref_axis',(0.,-0.942844461217511,-0.333233134534159));
#55435=DIRECTION('center_axis',(0.,-0.333233134534162,0.94284446121751));
#55436=DIRECTION('ref_axis',(0.,-0.94284446121751,-0.333233134534162));
#55437=DIRECTION('center_axis',(0.,0.333233134534159,-0.942844461217511));
#55438=DIRECTION('ref_axis',(0.,-0.942844461217511,-0.333233134534159));
#55439=DIRECTION('',(0.,0.333233134534162,-0.94284446121751));
#55440=DIRECTION('center_axis',(0.,-0.333233134534162,0.94284446121751));
#55441=DIRECTION('ref_axis',(0.,-0.94284446121751,-0.333233134534162));
#55442=DIRECTION('center_axis',(0.,-0.333233134534162,0.94284446121751));
#55443=DIRECTION('ref_axis',(0.,-0.94284446121751,-0.333233134534162));
#55444=DIRECTION('center_axis',(0.,-0.333233134534162,0.94284446121751));
#55445=DIRECTION('ref_axis',(0.,-0.94284446121751,-0.333233134534162));
#55446=DIRECTION('center_axis',(0.,0.333233134534162,-0.94284446121751));
#55447=DIRECTION('ref_axis',(0.,0.94284446121751,0.333233134534162));
#55448=DIRECTION('',(0.,-0.333233134534162,0.94284446121751));
#55449=DIRECTION('center_axis',(0.,0.333233134534159,-0.942844461217511));
#55450=DIRECTION('ref_axis',(0.,-0.942844461217511,-0.333233134534159));
#55451=DIRECTION('center_axis',(0.,-0.333233134534162,0.94284446121751));
#55452=DIRECTION('ref_axis',(0.,-0.94284446121751,-0.333233134534161));
#55453=DIRECTION('center_axis',(0.,0.333233134534159,-0.942844461217511));
#55454=DIRECTION('ref_axis',(0.,-0.942844461217511,-0.333233134534159));
#55455=DIRECTION('',(0.,0.333233134534162,-0.94284446121751));
#55456=DIRECTION('center_axis',(0.,0.333233134534162,-0.94284446121751));
#55457=DIRECTION('ref_axis',(0.,-0.94284446121751,-0.333233134534162));
#55458=DIRECTION('center_axis',(0.,-0.333233134534162,0.94284446121751));
#55459=DIRECTION('ref_axis',(0.,-0.94284446121751,-0.333233134534162));
#55460=DIRECTION('center_axis',(0.,0.333233134534162,-0.94284446121751));
#55461=DIRECTION('ref_axis',(0.,0.94284446121751,0.333233134534162));
#55462=DIRECTION('',(0.,-0.333233134534162,0.94284446121751));
#55463=DIRECTION('center_axis',(0.,0.333233134534159,-0.942844461217511));
#55464=DIRECTION('ref_axis',(0.,-0.942844461217511,-0.333233134534159));
#55465=DIRECTION('center_axis',(0.,-0.333233134534162,0.94284446121751));
#55466=DIRECTION('ref_axis',(0.,-0.94284446121751,-0.333233134534162));
#55467=DIRECTION('center_axis',(0.,0.333233134534159,-0.942844461217511));
#55468=DIRECTION('ref_axis',(0.,-0.942844461217511,-0.333233134534159));
#55469=DIRECTION('',(0.,0.333233134534162,-0.94284446121751));
#55470=DIRECTION('center_axis',(0.,0.333233134534162,-0.94284446121751));
#55471=DIRECTION('ref_axis',(0.,-0.94284446121751,-0.333233134534162));
#55472=DIRECTION('center_axis',(0.,-0.333233134534162,0.94284446121751));
#55473=DIRECTION('ref_axis',(0.,-0.94284446121751,-0.333233134534162));
#55474=DIRECTION('center_axis',(0.,0.333233134534162,-0.94284446121751));
#55475=DIRECTION('ref_axis',(0.,0.94284446121751,0.333233134534162));
#55476=DIRECTION('',(0.,-0.333233134534162,0.942844461217511));
#55477=DIRECTION('center_axis',(0.,0.333233134534159,-0.942844461217511));
#55478=DIRECTION('ref_axis',(0.,-0.942844461217511,-0.333233134534159));
#55479=DIRECTION('center_axis',(0.,-0.333233134534162,0.94284446121751));
#55480=DIRECTION('ref_axis',(0.,-0.94284446121751,-0.333233134534162));
#55481=DIRECTION('center_axis',(0.,0.333233134534159,-0.942844461217511));
#55482=DIRECTION('ref_axis',(0.,-0.942844461217511,-0.333233134534159));
#55483=DIRECTION('',(0.,0.333233134534162,-0.94284446121751));
#55484=DIRECTION('center_axis',(0.,0.333233134534162,-0.94284446121751));
#55485=DIRECTION('ref_axis',(0.,-0.94284446121751,-0.333233134534162));
#55486=DIRECTION('center_axis',(0.,-0.333233134534162,0.94284446121751));
#55487=DIRECTION('ref_axis',(0.,-0.94284446121751,-0.333233134534162));
#55488=DIRECTION('center_axis',(0.,0.333233134534162,-0.94284446121751));
#55489=DIRECTION('ref_axis',(0.,0.94284446121751,0.333233134534162));
#55490=DIRECTION('',(0.,-0.333233134534162,0.94284446121751));
#55491=DIRECTION('center_axis',(0.,0.333233134534159,-0.942844461217511));
#55492=DIRECTION('ref_axis',(0.,-0.942844461217511,-0.333233134534159));
#55493=DIRECTION('center_axis',(0.,-0.333233134534162,0.94284446121751));
#55494=DIRECTION('ref_axis',(0.,-0.94284446121751,-0.333233134534162));
#55495=DIRECTION('center_axis',(0.,0.333233134534159,-0.942844461217511));
#55496=DIRECTION('ref_axis',(0.,-0.942844461217511,-0.333233134534159));
#55497=DIRECTION('',(0.,0.333233134534162,-0.94284446121751));
#55498=DIRECTION('center_axis',(0.,0.333233134534162,-0.94284446121751));
#55499=DIRECTION('ref_axis',(0.,-0.94284446121751,-0.333233134534162));
#55500=DIRECTION('center_axis',(0.,-0.333233134534162,0.94284446121751));
#55501=DIRECTION('ref_axis',(0.,-0.94284446121751,-0.333233134534162));
#55502=DIRECTION('center_axis',(0.,0.333233134534162,-0.94284446121751));
#55503=DIRECTION('ref_axis',(0.,0.94284446121751,0.333233134534162));
#55504=DIRECTION('',(0.,-0.333233134534162,0.94284446121751));
#55505=DIRECTION('center_axis',(0.,0.333233134534159,-0.942844461217511));
#55506=DIRECTION('ref_axis',(0.,-0.942844461217511,-0.333233134534159));
#55507=DIRECTION('center_axis',(0.,-0.333233134534162,0.94284446121751));
#55508=DIRECTION('ref_axis',(0.,-0.94284446121751,-0.333233134534162));
#55509=DIRECTION('center_axis',(0.,0.333233134534159,-0.942844461217511));
#55510=DIRECTION('ref_axis',(0.,-0.942844461217511,-0.333233134534159));
#55511=DIRECTION('',(0.,0.333233134534162,-0.94284446121751));
#55512=DIRECTION('center_axis',(0.,0.333233134534162,-0.94284446121751));
#55513=DIRECTION('ref_axis',(0.,-0.94284446121751,-0.333233134534162));
#55514=DIRECTION('center_axis',(0.,-0.333233134534162,0.94284446121751));
#55515=DIRECTION('ref_axis',(0.,-0.94284446121751,-0.333233134534162));
#55516=DIRECTION('center_axis',(0.,0.333233134534162,-0.94284446121751));
#55517=DIRECTION('ref_axis',(0.,0.94284446121751,0.333233134534162));
#55518=DIRECTION('',(0.,-0.333233134534162,0.94284446121751));
#55519=DIRECTION('center_axis',(0.,0.333233134534159,-0.942844461217511));
#55520=DIRECTION('ref_axis',(0.,-0.942844461217511,-0.333233134534159));
#55521=DIRECTION('center_axis',(0.,-0.333233134534162,0.94284446121751));
#55522=DIRECTION('ref_axis',(0.,-0.94284446121751,-0.333233134534162));
#55523=DIRECTION('center_axis',(0.,0.333233134534159,-0.942844461217511));
#55524=DIRECTION('ref_axis',(0.,-0.942844461217511,-0.333233134534159));
#55525=DIRECTION('',(0.,0.333233134534162,-0.94284446121751));
#55526=DIRECTION('center_axis',(0.,0.333233134534162,-0.94284446121751));
#55527=DIRECTION('ref_axis',(0.,-0.94284446121751,-0.333233134534162));
#55528=DIRECTION('center_axis',(0.,-0.333233134534162,0.94284446121751));
#55529=DIRECTION('ref_axis',(0.,-0.94284446121751,-0.333233134534162));
#55530=DIRECTION('center_axis',(0.,0.333233134534162,-0.94284446121751));
#55531=DIRECTION('ref_axis',(0.,0.94284446121751,0.333233134534162));
#55532=DIRECTION('',(0.,-0.333233134534162,0.94284446121751));
#55533=DIRECTION('center_axis',(0.,0.333233134534159,-0.942844461217511));
#55534=DIRECTION('ref_axis',(0.,-0.942844461217511,-0.333233134534159));
#55535=DIRECTION('center_axis',(0.,-0.333233134534162,0.94284446121751));
#55536=DIRECTION('ref_axis',(0.,-0.94284446121751,-0.333233134534162));
#55537=DIRECTION('center_axis',(0.,0.333233134534159,-0.942844461217511));
#55538=DIRECTION('ref_axis',(0.,-0.942844461217511,-0.333233134534159));
#55539=DIRECTION('',(0.,0.333233134534162,-0.94284446121751));
#55540=DIRECTION('center_axis',(0.,0.333233134534162,-0.94284446121751));
#55541=DIRECTION('ref_axis',(0.,-0.94284446121751,-0.333233134534162));
#55542=DIRECTION('center_axis',(0.,-0.333233134534162,0.94284446121751));
#55543=DIRECTION('ref_axis',(0.,-0.94284446121751,-0.333233134534162));
#55544=DIRECTION('center_axis',(0.,0.333233134534162,-0.94284446121751));
#55545=DIRECTION('ref_axis',(0.,0.94284446121751,0.333233134534162));
#55546=DIRECTION('',(0.,-0.333233134534162,0.94284446121751));
#55547=DIRECTION('center_axis',(0.,0.333233134534159,-0.942844461217511));
#55548=DIRECTION('ref_axis',(0.,-0.942844461217511,-0.333233134534159));
#55549=DIRECTION('center_axis',(0.,-0.333233134534162,0.94284446121751));
#55550=DIRECTION('ref_axis',(0.,-0.94284446121751,-0.333233134534162));
#55551=DIRECTION('center_axis',(0.,0.333233134534159,-0.942844461217511));
#55552=DIRECTION('ref_axis',(0.,-0.942844461217511,-0.333233134534159));
#55553=DIRECTION('',(0.,0.333233134534162,-0.94284446121751));
#55554=DIRECTION('center_axis',(0.,0.333233134534162,-0.94284446121751));
#55555=DIRECTION('ref_axis',(0.,-0.94284446121751,-0.333233134534162));
#55556=DIRECTION('center_axis',(0.,-0.333233134534162,0.94284446121751));
#55557=DIRECTION('ref_axis',(0.,-0.94284446121751,-0.333233134534162));
#55558=DIRECTION('center_axis',(0.,0.333233134534162,-0.94284446121751));
#55559=DIRECTION('ref_axis',(0.,0.94284446121751,0.333233134534162));
#55560=DIRECTION('',(0.,-0.333233134534162,0.94284446121751));
#55561=DIRECTION('center_axis',(0.,0.333233134534159,-0.942844461217511));
#55562=DIRECTION('ref_axis',(0.,-0.942844461217511,-0.333233134534159));
#55563=DIRECTION('center_axis',(0.,-0.333233134534162,0.94284446121751));
#55564=DIRECTION('ref_axis',(0.,-0.94284446121751,-0.333233134534162));
#55565=DIRECTION('center_axis',(0.,0.333233134534159,-0.942844461217511));
#55566=DIRECTION('ref_axis',(0.,-0.942844461217511,-0.333233134534159));
#55567=DIRECTION('',(0.,0.333233134534162,-0.94284446121751));
#55568=DIRECTION('center_axis',(0.,-0.333233134534162,0.94284446121751));
#55569=DIRECTION('ref_axis',(0.,-0.94284446121751,-0.333233134534162));
#55570=DIRECTION('center_axis',(0.,-0.333233134534162,0.94284446121751));
#55571=DIRECTION('ref_axis',(0.,-0.94284446121751,-0.333233134534162));
#55572=DIRECTION('center_axis',(0.,0.333233134534162,-0.94284446121751));
#55573=DIRECTION('ref_axis',(0.,0.94284446121751,0.333233134534162));
#55574=DIRECTION('',(0.,-0.333233134534162,0.94284446121751));
#55575=DIRECTION('center_axis',(0.,0.333233134534159,-0.942844461217511));
#55576=DIRECTION('ref_axis',(0.,-0.942844461217511,-0.333233134534159));
#55577=DIRECTION('center_axis',(0.,-0.333233134534162,0.94284446121751));
#55578=DIRECTION('ref_axis',(0.,-0.94284446121751,-0.333233134534162));
#55579=DIRECTION('center_axis',(0.,0.333233134534159,-0.942844461217511));
#55580=DIRECTION('ref_axis',(0.,-0.942844461217511,-0.333233134534159));
#55581=DIRECTION('',(0.,0.333233134534162,-0.94284446121751));
#55582=DIRECTION('center_axis',(0.,0.333233134534162,-0.94284446121751));
#55583=DIRECTION('ref_axis',(0.,-0.94284446121751,-0.333233134534162));
#55584=DIRECTION('center_axis',(0.,-0.333233134534162,0.94284446121751));
#55585=DIRECTION('ref_axis',(0.,-0.94284446121751,-0.333233134534162));
#55586=DIRECTION('center_axis',(0.,0.333233134534162,-0.94284446121751));
#55587=DIRECTION('ref_axis',(0.,0.94284446121751,0.333233134534162));
#55588=DIRECTION('',(0.,-0.333233134534162,0.94284446121751));
#55589=DIRECTION('center_axis',(0.,0.333233134534159,-0.942844461217511));
#55590=DIRECTION('ref_axis',(0.,-0.942844461217511,-0.333233134534159));
#55591=DIRECTION('center_axis',(0.,-0.333233134534162,0.94284446121751));
#55592=DIRECTION('ref_axis',(0.,-0.94284446121751,-0.333233134534162));
#55593=DIRECTION('center_axis',(0.,0.333233134534159,-0.942844461217511));
#55594=DIRECTION('ref_axis',(0.,-0.942844461217511,-0.333233134534159));
#55595=DIRECTION('',(0.,0.333233134534162,-0.94284446121751));
#55596=DIRECTION('center_axis',(0.,0.333233134534162,-0.94284446121751));
#55597=DIRECTION('ref_axis',(0.,-0.94284446121751,-0.333233134534162));
#55598=DIRECTION('center_axis',(0.,-0.333233134534162,0.94284446121751));
#55599=DIRECTION('ref_axis',(0.,-0.94284446121751,-0.333233134534162));
#55600=DIRECTION('center_axis',(0.,0.333233134534162,-0.94284446121751));
#55601=DIRECTION('ref_axis',(0.,0.94284446121751,0.333233134534162));
#55602=DIRECTION('',(0.,-0.333233134534162,0.94284446121751));
#55603=DIRECTION('center_axis',(0.,0.333233134534159,-0.942844461217511));
#55604=DIRECTION('ref_axis',(0.,-0.942844461217511,-0.333233134534159));
#55605=DIRECTION('center_axis',(0.,-0.333233134534162,0.94284446121751));
#55606=DIRECTION('ref_axis',(0.,-0.94284446121751,-0.333233134534161));
#55607=DIRECTION('center_axis',(0.,0.333233134534159,-0.942844461217511));
#55608=DIRECTION('ref_axis',(0.,-0.942844461217511,-0.333233134534159));
#55609=DIRECTION('',(0.,0.333233134534162,-0.94284446121751));
#55610=DIRECTION('center_axis',(0.,0.333233134534162,-0.94284446121751));
#55611=DIRECTION('ref_axis',(0.,-0.94284446121751,-0.333233134534162));
#55612=DIRECTION('center_axis',(0.,-0.333233134534162,0.94284446121751));
#55613=DIRECTION('ref_axis',(0.,-0.94284446121751,-0.333233134534162));
#55614=DIRECTION('center_axis',(0.,0.333233134534162,-0.94284446121751));
#55615=DIRECTION('ref_axis',(0.,0.94284446121751,0.333233134534162));
#55616=DIRECTION('',(0.,-0.333233134534162,0.94284446121751));
#55617=DIRECTION('center_axis',(0.,0.333233134534159,-0.942844461217511));
#55618=DIRECTION('ref_axis',(0.,-0.942844461217511,-0.333233134534159));
#55619=DIRECTION('center_axis',(0.,-0.333233134534162,0.94284446121751));
#55620=DIRECTION('ref_axis',(0.,-0.94284446121751,-0.333233134534162));
#55621=DIRECTION('center_axis',(0.,0.333233134534159,-0.942844461217511));
#55622=DIRECTION('ref_axis',(0.,-0.942844461217511,-0.333233134534159));
#55623=DIRECTION('',(0.,0.333233134534162,-0.94284446121751));
#55624=DIRECTION('center_axis',(0.,0.333233134534162,-0.94284446121751));
#55625=DIRECTION('ref_axis',(0.,-0.94284446121751,-0.333233134534162));
#55626=DIRECTION('center_axis',(0.,-0.333233134534162,0.94284446121751));
#55627=DIRECTION('ref_axis',(0.,-0.94284446121751,-0.333233134534162));
#55628=DIRECTION('center_axis',(0.,0.333233134534162,-0.94284446121751));
#55629=DIRECTION('ref_axis',(0.,0.94284446121751,0.333233134534162));
#55630=DIRECTION('',(0.,-0.333233134534162,0.94284446121751));
#55631=DIRECTION('center_axis',(0.,0.333233134534159,-0.942844461217511));
#55632=DIRECTION('ref_axis',(0.,-0.942844461217511,-0.333233134534159));
#55633=DIRECTION('center_axis',(0.,-0.333233134534162,0.94284446121751));
#55634=DIRECTION('ref_axis',(0.,-0.94284446121751,-0.333233134534162));
#55635=DIRECTION('center_axis',(0.,0.333233134534159,-0.942844461217511));
#55636=DIRECTION('ref_axis',(0.,-0.942844461217511,-0.333233134534159));
#55637=DIRECTION('',(0.,0.333233134534162,-0.94284446121751));
#55638=DIRECTION('center_axis',(0.,0.333233134534162,-0.94284446121751));
#55639=DIRECTION('ref_axis',(0.,-0.94284446121751,-0.333233134534162));
#55640=DIRECTION('center_axis',(0.,-0.333233134534162,0.94284446121751));
#55641=DIRECTION('ref_axis',(0.,-0.94284446121751,-0.333233134534162));
#55642=DIRECTION('center_axis',(0.,0.333233134534162,-0.94284446121751));
#55643=DIRECTION('ref_axis',(0.,0.94284446121751,0.333233134534162));
#55644=DIRECTION('',(0.,-0.333233134534162,0.94284446121751));
#55645=DIRECTION('center_axis',(0.,0.333233134534159,-0.942844461217511));
#55646=DIRECTION('ref_axis',(0.,-0.942844461217511,-0.333233134534159));
#55647=DIRECTION('center_axis',(0.,-0.333233134534162,0.94284446121751));
#55648=DIRECTION('ref_axis',(0.,-0.94284446121751,-0.333233134534162));
#55649=DIRECTION('center_axis',(0.,0.333233134534159,-0.942844461217511));
#55650=DIRECTION('ref_axis',(0.,-0.942844461217511,-0.333233134534159));
#55651=DIRECTION('',(0.,0.333233134534162,-0.94284446121751));
#55652=DIRECTION('center_axis',(0.,0.333233134534162,-0.94284446121751));
#55653=DIRECTION('ref_axis',(0.,-0.94284446121751,-0.333233134534162));
#55654=DIRECTION('center_axis',(0.,-0.333233134534162,0.94284446121751));
#55655=DIRECTION('ref_axis',(0.,-0.94284446121751,-0.333233134534162));
#55656=DIRECTION('center_axis',(0.,0.333233134534162,-0.94284446121751));
#55657=DIRECTION('ref_axis',(0.,0.94284446121751,0.333233134534162));
#55658=DIRECTION('',(0.,-0.333233134534162,0.94284446121751));
#55659=DIRECTION('center_axis',(0.,0.333233134534159,-0.942844461217511));
#55660=DIRECTION('ref_axis',(0.,-0.942844461217511,-0.333233134534159));
#55661=DIRECTION('center_axis',(0.,-0.333233134534162,0.94284446121751));
#55662=DIRECTION('ref_axis',(0.,-0.94284446121751,-0.333233134534162));
#55663=DIRECTION('center_axis',(0.,0.333233134534159,-0.942844461217511));
#55664=DIRECTION('ref_axis',(0.,-0.942844461217511,-0.333233134534159));
#55665=DIRECTION('',(0.,0.333233134534162,-0.94284446121751));
#55666=DIRECTION('center_axis',(0.,0.333233134534162,-0.94284446121751));
#55667=DIRECTION('ref_axis',(0.,-0.94284446121751,-0.333233134534162));
#55668=DIRECTION('center_axis',(0.,-0.333233134534162,0.94284446121751));
#55669=DIRECTION('ref_axis',(0.,-0.94284446121751,-0.333233134534162));
#55670=DIRECTION('center_axis',(0.,0.333233134534162,-0.94284446121751));
#55671=DIRECTION('ref_axis',(0.,0.94284446121751,0.333233134534162));
#55672=DIRECTION('',(0.,-0.333233134534162,0.94284446121751));
#55673=DIRECTION('center_axis',(0.,0.333233134534159,-0.942844461217511));
#55674=DIRECTION('ref_axis',(0.,-0.942844461217511,-0.333233134534159));
#55675=DIRECTION('center_axis',(0.,-0.333233134534162,0.94284446121751));
#55676=DIRECTION('ref_axis',(0.,-0.94284446121751,-0.333233134534162));
#55677=DIRECTION('center_axis',(0.,0.333233134534159,-0.942844461217511));
#55678=DIRECTION('ref_axis',(0.,-0.942844461217511,-0.333233134534159));
#55679=DIRECTION('',(0.,0.333233134534162,-0.94284446121751));
#55680=DIRECTION('center_axis',(0.,-0.333233134534162,0.94284446121751));
#55681=DIRECTION('ref_axis',(0.,-0.94284446121751,-0.333233134534162));
#55682=DIRECTION('center_axis',(0.,-0.333233134534162,0.94284446121751));
#55683=DIRECTION('ref_axis',(0.,-0.94284446121751,-0.333233134534162));
#55684=DIRECTION('center_axis',(0.,0.333233134534162,-0.94284446121751));
#55685=DIRECTION('ref_axis',(0.,0.94284446121751,0.333233134534162));
#55686=DIRECTION('',(0.,-0.333233134534162,0.94284446121751));
#55687=DIRECTION('center_axis',(0.,0.333233134534159,-0.942844461217511));
#55688=DIRECTION('ref_axis',(0.,-0.942844461217511,-0.333233134534159));
#55689=DIRECTION('center_axis',(0.,-0.333233134534162,0.94284446121751));
#55690=DIRECTION('ref_axis',(0.,-0.94284446121751,-0.333233134534162));
#55691=DIRECTION('center_axis',(0.,0.333233134534159,-0.942844461217511));
#55692=DIRECTION('ref_axis',(0.,-0.942844461217511,-0.333233134534159));
#55693=DIRECTION('',(0.,0.333233134534162,-0.94284446121751));
#55694=DIRECTION('center_axis',(0.,0.333233134534162,-0.94284446121751));
#55695=DIRECTION('ref_axis',(0.,-0.94284446121751,-0.333233134534162));
#55696=DIRECTION('center_axis',(0.,-0.333233134534162,0.94284446121751));
#55697=DIRECTION('ref_axis',(0.,-0.94284446121751,-0.333233134534162));
#55698=DIRECTION('center_axis',(0.,0.333233134534162,-0.94284446121751));
#55699=DIRECTION('ref_axis',(0.,0.94284446121751,0.333233134534162));
#55700=DIRECTION('',(0.,-0.333233134534162,0.94284446121751));
#55701=DIRECTION('center_axis',(0.,0.333233134534159,-0.942844461217511));
#55702=DIRECTION('ref_axis',(0.,-0.942844461217511,-0.333233134534159));
#55703=DIRECTION('center_axis',(0.,-0.333233134534162,0.94284446121751));
#55704=DIRECTION('ref_axis',(0.,-0.94284446121751,-0.333233134534162));
#55705=DIRECTION('center_axis',(0.,0.333233134534159,-0.942844461217511));
#55706=DIRECTION('ref_axis',(0.,-0.942844461217511,-0.333233134534159));
#55707=DIRECTION('',(0.,0.333233134534162,-0.94284446121751));
#55708=DIRECTION('center_axis',(0.,0.333233134534162,-0.94284446121751));
#55709=DIRECTION('ref_axis',(0.,-0.94284446121751,-0.333233134534162));
#55710=DIRECTION('center_axis',(0.,-0.333233134534162,0.94284446121751));
#55711=DIRECTION('ref_axis',(0.,-0.94284446121751,-0.333233134534162));
#55712=DIRECTION('center_axis',(0.,0.333233134534162,-0.94284446121751));
#55713=DIRECTION('ref_axis',(0.,0.94284446121751,0.333233134534162));
#55714=DIRECTION('',(0.,-0.333233134534162,0.94284446121751));
#55715=DIRECTION('center_axis',(0.,0.333233134534159,-0.942844461217511));
#55716=DIRECTION('ref_axis',(0.,-0.942844461217511,-0.333233134534159));
#55717=DIRECTION('center_axis',(0.,-0.333233134534162,0.94284446121751));
#55718=DIRECTION('ref_axis',(0.,-0.94284446121751,-0.333233134534162));
#55719=DIRECTION('center_axis',(0.,0.333233134534159,-0.942844461217511));
#55720=DIRECTION('ref_axis',(0.,-0.942844461217511,-0.333233134534159));
#55721=DIRECTION('',(0.,0.333233134534162,-0.94284446121751));
#55722=DIRECTION('center_axis',(0.,0.333233134534162,-0.94284446121751));
#55723=DIRECTION('ref_axis',(0.,-0.94284446121751,-0.333233134534162));
#55724=DIRECTION('center_axis',(0.,-0.333233134534162,0.94284446121751));
#55725=DIRECTION('ref_axis',(0.,-0.94284446121751,-0.333233134534162));
#55726=DIRECTION('center_axis',(0.,0.333233134534162,-0.94284446121751));
#55727=DIRECTION('ref_axis',(0.,0.94284446121751,0.333233134534162));
#55728=DIRECTION('',(0.,-0.333233134534162,0.94284446121751));
#55729=DIRECTION('center_axis',(0.,0.333233134534159,-0.942844461217511));
#55730=DIRECTION('ref_axis',(0.,-0.942844461217511,-0.333233134534159));
#55731=DIRECTION('center_axis',(0.,-0.333233134534162,0.94284446121751));
#55732=DIRECTION('ref_axis',(0.,-0.94284446121751,-0.333233134534162));
#55733=DIRECTION('center_axis',(0.,0.333233134534159,-0.942844461217511));
#55734=DIRECTION('ref_axis',(0.,-0.942844461217511,-0.333233134534159));
#55735=DIRECTION('',(0.,0.333233134534162,-0.94284446121751));
#55736=DIRECTION('center_axis',(0.,0.333233134534162,-0.94284446121751));
#55737=DIRECTION('ref_axis',(0.,-0.94284446121751,-0.333233134534162));
#55738=DIRECTION('center_axis',(0.,-0.333233134534162,0.94284446121751));
#55739=DIRECTION('ref_axis',(0.,-0.94284446121751,-0.333233134534162));
#55740=DIRECTION('center_axis',(0.,0.333233134534162,-0.94284446121751));
#55741=DIRECTION('ref_axis',(0.,0.94284446121751,0.333233134534162));
#55742=DIRECTION('',(0.,-0.333233134534162,0.94284446121751));
#55743=DIRECTION('center_axis',(0.,0.333233134534159,-0.942844461217511));
#55744=DIRECTION('ref_axis',(0.,-0.942844461217511,-0.333233134534159));
#55745=DIRECTION('center_axis',(0.,-0.333233134534162,0.94284446121751));
#55746=DIRECTION('ref_axis',(0.,-0.94284446121751,-0.333233134534162));
#55747=DIRECTION('center_axis',(0.,0.333233134534159,-0.942844461217511));
#55748=DIRECTION('ref_axis',(0.,-0.942844461217511,-0.333233134534159));
#55749=DIRECTION('',(0.,0.333233134534162,-0.94284446121751));
#55750=DIRECTION('center_axis',(0.,0.333233134534162,-0.94284446121751));
#55751=DIRECTION('ref_axis',(0.,-0.94284446121751,-0.333233134534162));
#55752=DIRECTION('center_axis',(0.,-0.333233134534162,0.94284446121751));
#55753=DIRECTION('ref_axis',(0.,-0.94284446121751,-0.333233134534162));
#55754=DIRECTION('center_axis',(0.,0.333233134534162,-0.94284446121751));
#55755=DIRECTION('ref_axis',(0.,0.94284446121751,0.333233134534162));
#55756=DIRECTION('',(0.,-0.333233134534162,0.94284446121751));
#55757=DIRECTION('center_axis',(0.,0.333233134534159,-0.942844461217511));
#55758=DIRECTION('ref_axis',(0.,-0.942844461217511,-0.333233134534159));
#55759=DIRECTION('center_axis',(0.,-0.333233134534162,0.94284446121751));
#55760=DIRECTION('ref_axis',(0.,-0.94284446121751,-0.333233134534162));
#55761=DIRECTION('center_axis',(0.,0.333233134534159,-0.942844461217511));
#55762=DIRECTION('ref_axis',(0.,-0.942844461217511,-0.333233134534159));
#55763=DIRECTION('',(0.,0.333233134534161,-0.94284446121751));
#55764=DIRECTION('center_axis',(0.,0.333233134534162,-0.94284446121751));
#55765=DIRECTION('ref_axis',(0.,-0.94284446121751,-0.333233134534162));
#55766=DIRECTION('center_axis',(0.,-0.333233134534162,0.94284446121751));
#55767=DIRECTION('ref_axis',(0.,-0.94284446121751,-0.333233134534162));
#55768=DIRECTION('center_axis',(0.,0.333233134534162,-0.94284446121751));
#55769=DIRECTION('ref_axis',(0.,0.94284446121751,0.333233134534162));
#55770=DIRECTION('',(0.,-0.333233134534162,0.94284446121751));
#55771=DIRECTION('center_axis',(0.,0.333233134534159,-0.942844461217511));
#55772=DIRECTION('ref_axis',(0.,-0.942844461217511,-0.333233134534159));
#55773=DIRECTION('center_axis',(0.,-0.333233134534162,0.94284446121751));
#55774=DIRECTION('ref_axis',(0.,-0.94284446121751,-0.333233134534162));
#55775=DIRECTION('center_axis',(0.,0.333233134534159,-0.942844461217511));
#55776=DIRECTION('ref_axis',(0.,-0.942844461217511,-0.333233134534159));
#55777=DIRECTION('',(0.,0.333233134534162,-0.94284446121751));
#55778=DIRECTION('center_axis',(0.,0.333233134534162,-0.94284446121751));
#55779=DIRECTION('ref_axis',(0.,-0.94284446121751,-0.333233134534162));
#55780=DIRECTION('center_axis',(0.,-0.333233134534162,0.94284446121751));
#55781=DIRECTION('ref_axis',(0.,-0.94284446121751,-0.333233134534162));
#55782=DIRECTION('center_axis',(0.,0.333233134534162,-0.94284446121751));
#55783=DIRECTION('ref_axis',(0.,0.94284446121751,0.333233134534162));
#55784=DIRECTION('',(0.,-0.333233134534162,0.94284446121751));
#55785=DIRECTION('center_axis',(0.,0.333233134534159,-0.942844461217511));
#55786=DIRECTION('ref_axis',(0.,-0.942844461217511,-0.333233134534159));
#55787=DIRECTION('center_axis',(0.,-0.333233134534162,0.94284446121751));
#55788=DIRECTION('ref_axis',(0.,-0.94284446121751,-0.333233134534162));
#55789=DIRECTION('center_axis',(0.,0.333233134534159,-0.942844461217511));
#55790=DIRECTION('ref_axis',(0.,-0.942844461217511,-0.333233134534159));
#55791=DIRECTION('',(0.,0.333233134534162,-0.94284446121751));
#55792=DIRECTION('center_axis',(0.,0.333233134534162,-0.94284446121751));
#55793=DIRECTION('ref_axis',(0.,-0.94284446121751,-0.333233134534162));
#55794=DIRECTION('center_axis',(0.,-0.333233134534162,0.94284446121751));
#55795=DIRECTION('ref_axis',(0.,-0.94284446121751,-0.333233134534162));
#55796=DIRECTION('center_axis',(0.,0.333233134534162,-0.94284446121751));
#55797=DIRECTION('ref_axis',(0.,0.94284446121751,0.333233134534162));
#55798=DIRECTION('',(0.,-0.333233134534162,0.94284446121751));
#55799=DIRECTION('center_axis',(0.,0.333233134534159,-0.942844461217511));
#55800=DIRECTION('ref_axis',(0.,-0.942844461217511,-0.333233134534159));
#55801=DIRECTION('center_axis',(0.,-0.333233134534162,0.94284446121751));
#55802=DIRECTION('ref_axis',(0.,-0.94284446121751,-0.333233134534162));
#55803=DIRECTION('center_axis',(0.,0.333233134534159,-0.942844461217511));
#55804=DIRECTION('ref_axis',(0.,-0.942844461217511,-0.333233134534159));
#55805=DIRECTION('',(0.,0.333233134534162,-0.94284446121751));
#55806=DIRECTION('center_axis',(0.,-0.333233134534162,0.94284446121751));
#55807=DIRECTION('ref_axis',(0.,-0.94284446121751,-0.333233134534162));
#55808=DIRECTION('center_axis',(0.,-0.333233134534162,0.94284446121751));
#55809=DIRECTION('ref_axis',(0.,-0.94284446121751,-0.333233134534162));
#55810=DIRECTION('center_axis',(0.,0.333233134534162,-0.94284446121751));
#55811=DIRECTION('ref_axis',(0.,0.94284446121751,0.333233134534162));
#55812=DIRECTION('',(0.,-0.333233134534162,0.94284446121751));
#55813=DIRECTION('center_axis',(0.,0.333233134534159,-0.942844461217511));
#55814=DIRECTION('ref_axis',(0.,-0.942844461217511,-0.333233134534159));
#55815=DIRECTION('center_axis',(0.,-0.333233134534162,0.94284446121751));
#55816=DIRECTION('ref_axis',(0.,-0.94284446121751,-0.333233134534161));
#55817=DIRECTION('center_axis',(0.,0.333233134534159,-0.942844461217511));
#55818=DIRECTION('ref_axis',(0.,-0.942844461217511,-0.333233134534159));
#55819=DIRECTION('',(0.,0.333233134534162,-0.94284446121751));
#55820=DIRECTION('center_axis',(0.,0.333233134534162,-0.94284446121751));
#55821=DIRECTION('ref_axis',(0.,-0.94284446121751,-0.333233134534162));
#55822=DIRECTION('center_axis',(0.,-0.333233134534162,0.94284446121751));
#55823=DIRECTION('ref_axis',(0.,-0.94284446121751,-0.333233134534162));
#55824=DIRECTION('center_axis',(0.,0.333233134534162,-0.94284446121751));
#55825=DIRECTION('ref_axis',(0.,0.94284446121751,0.333233134534162));
#55826=DIRECTION('',(0.,-0.333233134534162,0.94284446121751));
#55827=DIRECTION('center_axis',(0.,0.333233134534159,-0.942844461217511));
#55828=DIRECTION('ref_axis',(0.,-0.942844461217511,-0.333233134534159));
#55829=DIRECTION('center_axis',(0.,-0.333233134534162,0.94284446121751));
#55830=DIRECTION('ref_axis',(0.,-0.94284446121751,-0.333233134534162));
#55831=DIRECTION('center_axis',(0.,0.333233134534159,-0.942844461217511));
#55832=DIRECTION('ref_axis',(0.,-0.942844461217511,-0.333233134534159));
#55833=DIRECTION('',(0.,0.333233134534162,-0.94284446121751));
#55834=DIRECTION('center_axis',(0.,0.333233134534162,-0.94284446121751));
#55835=DIRECTION('ref_axis',(0.,-0.94284446121751,-0.333233134534162));
#55836=DIRECTION('center_axis',(0.,-0.333233134534162,0.94284446121751));
#55837=DIRECTION('ref_axis',(0.,-0.94284446121751,-0.333233134534162));
#55838=DIRECTION('center_axis',(0.,0.333233134534162,-0.94284446121751));
#55839=DIRECTION('ref_axis',(0.,0.94284446121751,0.333233134534162));
#55840=DIRECTION('',(0.,-0.333233134534162,0.94284446121751));
#55841=DIRECTION('center_axis',(0.,0.333233134534159,-0.942844461217511));
#55842=DIRECTION('ref_axis',(0.,-0.942844461217511,-0.333233134534159));
#55843=DIRECTION('center_axis',(0.,-0.333233134534162,0.94284446121751));
#55844=DIRECTION('ref_axis',(0.,-0.94284446121751,-0.333233134534162));
#55845=DIRECTION('center_axis',(0.,0.333233134534159,-0.942844461217511));
#55846=DIRECTION('ref_axis',(0.,-0.942844461217511,-0.333233134534159));
#55847=DIRECTION('',(0.,0.333233134534162,-0.94284446121751));
#55848=DIRECTION('center_axis',(0.,0.333233134534162,-0.94284446121751));
#55849=DIRECTION('ref_axis',(0.,-0.94284446121751,-0.333233134534162));
#55850=DIRECTION('center_axis',(0.,-0.333233134534162,0.94284446121751));
#55851=DIRECTION('ref_axis',(0.,-0.94284446121751,-0.333233134534162));
#55852=DIRECTION('center_axis',(0.,0.333233134534162,-0.94284446121751));
#55853=DIRECTION('ref_axis',(0.,0.94284446121751,0.333233134534162));
#55854=DIRECTION('',(0.,-0.333233134534162,0.94284446121751));
#55855=DIRECTION('center_axis',(0.,0.333233134534159,-0.942844461217511));
#55856=DIRECTION('ref_axis',(0.,-0.942844461217511,-0.333233134534159));
#55857=DIRECTION('center_axis',(0.,-0.333233134534162,0.94284446121751));
#55858=DIRECTION('ref_axis',(0.,-0.94284446121751,-0.333233134534162));
#55859=DIRECTION('center_axis',(0.,0.333233134534159,-0.942844461217511));
#55860=DIRECTION('ref_axis',(0.,-0.942844461217511,-0.333233134534159));
#55861=DIRECTION('',(0.,0.333233134534162,-0.94284446121751));
#55862=DIRECTION('center_axis',(0.,0.333233134534162,-0.94284446121751));
#55863=DIRECTION('ref_axis',(0.,-0.94284446121751,-0.333233134534162));
#55864=DIRECTION('center_axis',(0.,-0.333233134534162,0.94284446121751));
#55865=DIRECTION('ref_axis',(0.,-0.94284446121751,-0.333233134534162));
#55866=DIRECTION('center_axis',(0.,0.333233134534162,-0.94284446121751));
#55867=DIRECTION('ref_axis',(0.,0.94284446121751,0.333233134534162));
#55868=DIRECTION('',(0.,-0.333233134534162,0.94284446121751));
#55869=DIRECTION('center_axis',(0.,0.333233134534159,-0.942844461217511));
#55870=DIRECTION('ref_axis',(0.,-0.942844461217511,-0.333233134534159));
#55871=DIRECTION('center_axis',(0.,-0.333233134534162,0.94284446121751));
#55872=DIRECTION('ref_axis',(0.,-0.94284446121751,-0.333233134534162));
#55873=DIRECTION('center_axis',(0.,0.333233134534159,-0.942844461217511));
#55874=DIRECTION('ref_axis',(0.,-0.942844461217511,-0.333233134534159));
#55875=DIRECTION('',(0.,0.333233134534162,-0.94284446121751));
#55876=DIRECTION('center_axis',(0.,0.333233134534162,-0.94284446121751));
#55877=DIRECTION('ref_axis',(0.,-0.94284446121751,-0.333233134534162));
#55878=DIRECTION('center_axis',(0.,-0.333233134534162,0.94284446121751));
#55879=DIRECTION('ref_axis',(0.,-0.94284446121751,-0.333233134534161));
#55880=DIRECTION('center_axis',(0.,0.333233134534162,-0.94284446121751));
#55881=DIRECTION('ref_axis',(0.,0.94284446121751,0.333233134534162));
#55882=DIRECTION('',(0.,-0.333233134534162,0.94284446121751));
#55883=DIRECTION('center_axis',(0.,0.333233134534159,-0.942844461217511));
#55884=DIRECTION('ref_axis',(0.,-0.942844461217511,-0.333233134534159));
#55885=DIRECTION('center_axis',(0.,-0.333233134534162,0.94284446121751));
#55886=DIRECTION('ref_axis',(0.,-0.94284446121751,-0.333233134534162));
#55887=DIRECTION('center_axis',(0.,0.333233134534159,-0.942844461217511));
#55888=DIRECTION('ref_axis',(0.,-0.942844461217511,-0.333233134534159));
#55889=DIRECTION('',(0.,0.333233134534162,-0.94284446121751));
#55890=DIRECTION('center_axis',(0.,0.333233134534162,-0.94284446121751));
#55891=DIRECTION('ref_axis',(0.,-0.94284446121751,-0.333233134534162));
#55892=DIRECTION('center_axis',(0.,-0.333233134534162,0.94284446121751));
#55893=DIRECTION('ref_axis',(0.,-0.94284446121751,-0.333233134534162));
#55894=DIRECTION('center_axis',(0.,0.333233134534162,-0.94284446121751));
#55895=DIRECTION('ref_axis',(0.,0.94284446121751,0.333233134534162));
#55896=DIRECTION('',(0.,-0.333233134534162,0.94284446121751));
#55897=DIRECTION('center_axis',(0.,0.333233134534159,-0.942844461217511));
#55898=DIRECTION('ref_axis',(0.,-0.942844461217511,-0.333233134534159));
#55899=DIRECTION('center_axis',(0.,-0.333233134534162,0.94284446121751));
#55900=DIRECTION('ref_axis',(0.,-0.94284446121751,-0.333233134534162));
#55901=DIRECTION('center_axis',(0.,0.333233134534159,-0.942844461217511));
#55902=DIRECTION('ref_axis',(0.,-0.942844461217511,-0.333233134534159));
#55903=DIRECTION('',(0.,0.333233134534162,-0.94284446121751));
#55904=DIRECTION('center_axis',(0.,0.333233134534162,-0.94284446121751));
#55905=DIRECTION('ref_axis',(0.,-0.94284446121751,-0.333233134534162));
#55906=DIRECTION('center_axis',(0.,-0.333233134534162,0.94284446121751));
#55907=DIRECTION('ref_axis',(0.,-0.94284446121751,-0.333233134534162));
#55908=DIRECTION('center_axis',(0.,0.333233134534162,-0.94284446121751));
#55909=DIRECTION('ref_axis',(0.,0.94284446121751,0.333233134534162));
#55910=DIRECTION('',(0.,-0.333233134534162,0.94284446121751));
#55911=DIRECTION('center_axis',(0.,0.333233134534159,-0.942844461217511));
#55912=DIRECTION('ref_axis',(0.,-0.942844461217511,-0.333233134534159));
#55913=DIRECTION('center_axis',(0.,-0.333233134534162,0.94284446121751));
#55914=DIRECTION('ref_axis',(0.,-0.94284446121751,-0.333233134534162));
#55915=DIRECTION('center_axis',(0.,0.333233134534159,-0.942844461217511));
#55916=DIRECTION('ref_axis',(0.,-0.942844461217511,-0.333233134534159));
#55917=DIRECTION('',(0.,0.333233134534162,-0.94284446121751));
#55918=DIRECTION('center_axis',(0.,0.333233134534162,-0.94284446121751));
#55919=DIRECTION('ref_axis',(0.,-0.94284446121751,-0.333233134534162));
#55920=DIRECTION('center_axis',(0.,-0.333233134534162,0.94284446121751));
#55921=DIRECTION('ref_axis',(0.,-0.94284446121751,-0.333233134534162));
#55922=DIRECTION('center_axis',(0.,0.333233134534162,-0.94284446121751));
#55923=DIRECTION('ref_axis',(0.,0.94284446121751,0.333233134534162));
#55924=DIRECTION('',(0.,-0.333233134534162,0.94284446121751));
#55925=DIRECTION('center_axis',(0.,0.333233134534159,-0.942844461217511));
#55926=DIRECTION('ref_axis',(0.,-0.942844461217511,-0.333233134534159));
#55927=DIRECTION('center_axis',(0.,-0.333233134534162,0.94284446121751));
#55928=DIRECTION('ref_axis',(0.,-0.94284446121751,-0.333233134534162));
#55929=DIRECTION('center_axis',(0.,0.333233134534159,-0.942844461217511));
#55930=DIRECTION('ref_axis',(0.,-0.942844461217511,-0.333233134534159));
#55931=DIRECTION('',(0.,0.333233134534162,-0.94284446121751));
#55932=DIRECTION('center_axis',(0.,-0.333233134534162,0.94284446121751));
#55933=DIRECTION('ref_axis',(0.,-0.94284446121751,-0.333233134534162));
#55934=DIRECTION('center_axis',(0.,-0.333233134534162,0.94284446121751));
#55935=DIRECTION('ref_axis',(0.,-0.94284446121751,-0.333233134534162));
#55936=DIRECTION('center_axis',(0.,0.333233134534162,-0.94284446121751));
#55937=DIRECTION('ref_axis',(0.,0.94284446121751,0.333233134534162));
#55938=DIRECTION('',(0.,-0.333233134534162,0.94284446121751));
#55939=DIRECTION('center_axis',(0.,0.333233134534159,-0.942844461217511));
#55940=DIRECTION('ref_axis',(0.,-0.942844461217511,-0.333233134534159));
#55941=DIRECTION('center_axis',(0.,0.333233134534162,-0.94284446121751));
#55942=DIRECTION('ref_axis',(0.,0.94284446121751,0.333233134534162));
#55943=DIRECTION('center_axis',(-0.816874943384427,0.543798202596429,0.192350829796967));
#55944=DIRECTION('ref_axis',(-0.137012003453352,0.140999089472445,-0.980483027735636));
#55945=DIRECTION('center_axis',(0.,-0.333233134534162,0.94284446121751));
#55946=DIRECTION('ref_axis',(0.,-0.94284446121751,-0.333233134534162));
#55947=DIRECTION('center_axis',(0.,-0.333233134534162,0.94284446121751));
#55948=DIRECTION('ref_axis',(0.,-0.94284446121751,-0.333233134534162));
#55949=DIRECTION('center_axis',(0.,-0.333233134534162,0.94284446121751));
#55950=DIRECTION('ref_axis',(0.,-0.94284446121751,-0.333233134534162));
#55951=DIRECTION('center_axis',(0.,-0.333233134534162,0.94284446121751));
#55952=DIRECTION('ref_axis',(0.,-0.94284446121751,-0.333233134534162));
#55953=DIRECTION('center_axis',(0.,-0.333233134534162,0.94284446121751));
#55954=DIRECTION('ref_axis',(0.,-0.94284446121751,-0.333233134534162));
#55955=DIRECTION('center_axis',(0.,-0.333233134534162,0.94284446121751));
#55956=DIRECTION('ref_axis',(0.,-0.94284446121751,-0.333233134534162));
#55957=DIRECTION('center_axis',(0.,-0.333233134534162,0.94284446121751));
#55958=DIRECTION('ref_axis',(0.,-0.94284446121751,-0.333233134534162));
#55959=DIRECTION('center_axis',(0.,-0.333233134534162,0.94284446121751));
#55960=DIRECTION('ref_axis',(0.,-0.94284446121751,-0.333233134534162));
#55961=DIRECTION('center_axis',(0.,-0.333233134534162,0.94284446121751));
#55962=DIRECTION('ref_axis',(0.,-0.94284446121751,-0.333233134534162));
#55963=DIRECTION('center_axis',(0.,-0.333233134534162,0.94284446121751));
#55964=DIRECTION('ref_axis',(0.,-0.94284446121751,-0.333233134534162));
#55965=DIRECTION('center_axis',(0.,-0.333233134534162,0.94284446121751));
#55966=DIRECTION('ref_axis',(0.,-0.94284446121751,-0.333233134534162));
#55967=DIRECTION('center_axis',(0.,-0.333233134534162,0.94284446121751));
#55968=DIRECTION('ref_axis',(0.,-0.94284446121751,-0.333233134534162));
#55969=DIRECTION('center_axis',(0.,-0.333233134534162,0.94284446121751));
#55970=DIRECTION('ref_axis',(0.,-0.94284446121751,-0.333233134534162));
#55971=DIRECTION('center_axis',(0.,-0.333233134534162,0.94284446121751));
#55972=DIRECTION('ref_axis',(0.,-0.94284446121751,-0.333233134534162));
#55973=DIRECTION('center_axis',(0.,-0.333233134534162,0.94284446121751));
#55974=DIRECTION('ref_axis',(0.,-0.94284446121751,-0.333233134534162));
#55975=DIRECTION('center_axis',(0.,-0.333233134534162,0.94284446121751));
#55976=DIRECTION('ref_axis',(0.,-0.94284446121751,-0.333233134534162));
#55977=DIRECTION('center_axis',(0.,-0.333233134534162,0.94284446121751));
#55978=DIRECTION('ref_axis',(0.,-0.94284446121751,-0.333233134534162));
#55979=DIRECTION('center_axis',(0.,-0.333233134534162,0.94284446121751));
#55980=DIRECTION('ref_axis',(0.,-0.94284446121751,-0.333233134534162));
#55981=DIRECTION('center_axis',(0.,-0.333233134534162,0.94284446121751));
#55982=DIRECTION('ref_axis',(0.,-0.94284446121751,-0.333233134534162));
#55983=DIRECTION('center_axis',(0.,-0.333233134534162,0.94284446121751));
#55984=DIRECTION('ref_axis',(0.,-0.94284446121751,-0.333233134534162));
#55985=DIRECTION('center_axis',(0.,-0.333233134534162,0.94284446121751));
#55986=DIRECTION('ref_axis',(0.,-0.94284446121751,-0.333233134534162));
#55987=DIRECTION('center_axis',(0.,-0.333233134534162,0.94284446121751));
#55988=DIRECTION('ref_axis',(0.,-0.94284446121751,-0.333233134534162));
#55989=DIRECTION('center_axis',(0.,-0.333233134534162,0.94284446121751));
#55990=DIRECTION('ref_axis',(0.,-0.94284446121751,-0.333233134534162));
#55991=DIRECTION('center_axis',(0.,-0.333233134534162,0.94284446121751));
#55992=DIRECTION('ref_axis',(0.,-0.94284446121751,-0.333233134534162));
#55993=DIRECTION('center_axis',(0.,-0.333233134534162,0.94284446121751));
#55994=DIRECTION('ref_axis',(0.,-0.94284446121751,-0.333233134534162));
#55995=DIRECTION('center_axis',(0.816885842678963,0.543832096794536,0.192208664026204));
#55996=DIRECTION('ref_axis',(-1.43377373465901E-14,0.33323313453417,-0.942844461217507));
#55997=DIRECTION('center_axis',(0.,0.333233134534162,-0.94284446121751));
#55998=DIRECTION('ref_axis',(0.,0.94284446121751,0.333233134534162));
#55999=DIRECTION('center_axis',(0.,-0.333233134534162,0.94284446121751));
#56000=DIRECTION('ref_axis',(0.,0.94284446121751,0.333233134534162));
#56001=DIRECTION('center_axis',(-0.809731323701899,-0.553327332132966,-0.195356205252313));
#56002=DIRECTION('ref_axis',(0.000159129308641561,-0.333124458135407,0.942882850660598));
#56003=DIRECTION('center_axis',(0.809731322759568,-0.553327335018826,-0.195356200984262));
#56004=DIRECTION('ref_axis',(-0.58680078359079,-0.763450698364046,-0.269829337813154));
#56005=DIRECTION('center_axis',(0.,-0.333233134534242,0.942844461217482));
#56006=DIRECTION('ref_axis',(0.,-0.942844461217482,-0.333233134534242));
#56007=DIRECTION('center_axis',(0.,0.333233134534242,-0.942844461217482));
#56008=DIRECTION('ref_axis',(0.,-0.942844461217482,-0.333233134534242));
#56009=DIRECTION('',(-1.18291797137864E-16,0.824470733586849,0.565904593954461));
#56010=DIRECTION('center_axis',(0.,-0.333233134534162,0.94284446121751));
#56011=DIRECTION('ref_axis',(0.,0.94284446121751,0.333233134534162));
#56012=DIRECTION('center_axis',(0.,0.333233134534242,-0.942844461217482));
#56013=DIRECTION('ref_axis',(0.,-0.942844461217482,-0.333233134534242));
#56014=DIRECTION('center_axis',(0.,-0.333233134534162,0.94284446121751));
#56015=DIRECTION('ref_axis',(0.,-0.94284446121751,-0.333233134534163));
#56016=DIRECTION('center_axis',(-1.,0.,0.));
#56017=DIRECTION('ref_axis',(0.,0.94284446121751,0.333233134534162));
#56018=DIRECTION('center_axis',(0.,0.333233134534162,-0.94284446121751));
#56019=DIRECTION('ref_axis',(0.,-0.94284446121751,-0.333233134534162));
#56020=DIRECTION('center_axis',(0.,0.333233134534202,-0.942844461217496));
#56021=DIRECTION('ref_axis',(0.,0.942844461217497,0.333233134534199));
#56022=DIRECTION('center_axis',(-1.,0.,0.));
#56023=DIRECTION('ref_axis',(0.,-0.942844461217496,-0.333233134534202));
#56024=DIRECTION('center_axis',(0.,-0.333233134534202,0.942844461217496));
#56025=DIRECTION('ref_axis',(0.,0.942844461217496,0.333233134534202));
#56026=DIRECTION('center_axis',(0.,-0.333233134534202,0.942844461217496));
#56027=DIRECTION('ref_axis',(0.,0.942844461217496,0.333233134534202));
#56028=DIRECTION('center_axis',(0.,0.333233134534162,-0.94284446121751));
#56029=DIRECTION('ref_axis',(0.,0.94284446121751,0.333233134534161));
#56030=DIRECTION('center_axis',(0.,0.333233134534162,-0.94284446121751));
#56031=DIRECTION('ref_axis',(0.,0.94284446121751,0.333233134534162));
#56032=DIRECTION('center_axis',(0.,0.333233134534162,-0.94284446121751));
#56033=DIRECTION('ref_axis',(0.,0.94284446121751,0.333233134534162));
#56034=DIRECTION('center_axis',(0.,-1.,0.));
#56035=DIRECTION('ref_axis',(0.,0.,-1.));
#56036=DIRECTION('center_axis',(0.,1.,0.));
#56037=DIRECTION('ref_axis',(0.,0.,-1.));
#56038=DIRECTION('center_axis',(0.747684665568337,0.,0.664053944249987));
#56039=DIRECTION('ref_axis',(0.664053944249987,0.,-0.747684665568336));
#56040=DIRECTION('center_axis',(0.,-1.,0.));
#56041=DIRECTION('ref_axis',(0.,0.,-1.));
#56042=DIRECTION('center_axis',(0.747684665568331,0.,-0.664053944249993));
#56043=DIRECTION('ref_axis',(-0.664053944249993,0.,-0.747684665568331));
#56044=DIRECTION('center_axis',(0.,0.,1.));
#56045=DIRECTION('ref_axis',(1.,0.,0.));
#56046=DIRECTION('center_axis',(0.,0.,1.));
#56047=DIRECTION('ref_axis',(1.,0.,0.));
#56048=DIRECTION('center_axis',(0.,0.,1.));
#56049=DIRECTION('ref_axis',(1.,0.,0.));
#56050=DIRECTION('',(0.,0.,-1.));
#56051=DIRECTION('center_axis',(0.,0.,1.));
#56052=DIRECTION('ref_axis',(1.,0.,0.));
#56053=DIRECTION('',(0.,0.,1.));
#56054=DIRECTION('center_axis',(0.,0.333233134534162,-0.94284446121751));
#56055=DIRECTION('ref_axis',(0.,0.94284446121751,0.333233134534162));
#56056=DIRECTION('center_axis',(0.762076920749875,-0.61044884773581,-0.215849417785665));
#56057=DIRECTION('ref_axis',(-0.113718860840941,-0.454371624364075,0.883523880640354));
#56058=DIRECTION('center_axis',(0.,-0.333233134534162,0.94284446121751));
#56059=DIRECTION('ref_axis',(0.,-0.94284446121751,-0.333233134534162));
#56060=DIRECTION('center_axis',(0.,0.33323313453416,-0.942844461217511));
#56061=DIRECTION('ref_axis',(0.,0.942844461217511,0.333233134534161));
#56062=DIRECTION('',(0.,-0.333233134534162,0.94284446121751));
#56063=DIRECTION('center_axis',(0.,0.33323313453416,-0.942844461217511));
#56064=DIRECTION('ref_axis',(0.,0.942844461217511,0.333233134534161));
#56065=DIRECTION('center_axis',(0.,0.33323313453416,-0.942844461217511));
#56066=DIRECTION('ref_axis',(0.,0.942844461217512,0.333233134534158));
#56067=DIRECTION('center_axis',(-1.,0.,0.));
#56068=DIRECTION('ref_axis',(0.,-0.94284446121751,-0.333233134534163));
#56069=DIRECTION('center_axis',(0.,-0.33323313453416,0.942844461217511));
#56070=DIRECTION('ref_axis',(0.,0.942844461217511,0.33323313453416));
#56071=DIRECTION('center_axis',(0.,-0.333233134534162,0.94284446121751));
#56072=DIRECTION('ref_axis',(0.,-0.94284446121751,-0.333233134534162));
#56073=DIRECTION('center_axis',(0.,0.333233134534162,-0.94284446121751));
#56074=DIRECTION('ref_axis',(0.,0.94284446121751,0.333233134534162));
#56075=DIRECTION('',(0.,-0.333233134534162,0.94284446121751));
#56076=DIRECTION('center_axis',(0.,-0.333233134534162,0.94284446121751));
#56077=DIRECTION('ref_axis',(0.,-0.94284446121751,-0.333233134534162));
#56078=DIRECTION('',(0.,0.333233134534162,-0.94284446121751));
#56079=DIRECTION('center_axis',(0.,0.333233134534162,-0.94284446121751));
#56080=DIRECTION('ref_axis',(0.,0.94284446121751,0.333233134534162));
#56081=DIRECTION('center_axis',(0.,1.,0.));
#56082=DIRECTION('ref_axis',(1.,0.,0.));
#56083=DIRECTION('center_axis',(1.,0.,0.));
#56084=DIRECTION('ref_axis',(0.,0.0958457525203355,-0.995396198367168));
#56085=DIRECTION('',(0.,0.0958457525203355,-0.995396198367168));
#56086=DIRECTION('',(0.,-0.999992762491362,0.00380459786244685));
#56087=DIRECTION('',(0.,0.0958457525203355,-0.995396198367168));
#56088=DIRECTION('',(0.,0.995396198367168,0.0958457525203355));
#56089=DIRECTION('center_axis',(0.,0.0958457525203355,-0.995396198367168));
#56090=DIRECTION('ref_axis',(-1.,0.,0.));
#56091=DIRECTION('center_axis',(0.,0.0958457525203355,-0.995396198367168));
#56092=DIRECTION('ref_axis',(1.,-1.34077497793431E-14,-1.29101946472523E-15));
#56093=DIRECTION('',(0.,0.0958457525203355,-0.995396198367168));
#56094=DIRECTION('center_axis',(0.,-0.0958457525203355,0.995396198367168));
#56095=DIRECTION('ref_axis',(1.,0.,0.));
#56096=DIRECTION('center_axis',(0.,0.995396198367168,0.0958457525203355));
#56097=DIRECTION('ref_axis',(0.,-0.0958457525203355,0.995396198367168));
#56098=DIRECTION('center_axis',(0.,-0.0958457525203355,0.995396198367168));
#56099=DIRECTION('ref_axis',(-1.,-1.38980017783282E-14,-1.33822536308449E-15));
#56100=DIRECTION('center_axis',(0.,0.0958457525203355,-0.995396198367168));
#56101=DIRECTION('ref_axis',(-1.,0.,0.));
#56102=DIRECTION('',(0.,0.0958457525203355,-0.995396198367168));
#56103=DIRECTION('center_axis',(0.,-0.0479781285213995,0.998848386484948));
#56104=DIRECTION('ref_axis',(-1.81973168778901E-14,-0.998848386484948,-0.0479781285213995));
#56105=DIRECTION('',(0.,0.0958457525203355,-0.995396198367168));
#56106=DIRECTION('center_axis',(0.,0.0958457525203355,-0.995396198367168));
#56107=DIRECTION('ref_axis',(1.,1.34077497793431E-14,1.29101946472523E-15));
#56108=DIRECTION('',(0.,0.0958457525203355,-0.995396198367168));
#56109=DIRECTION('center_axis',(0.,0.0958457525203355,-0.995396198367168));
#56110=DIRECTION('ref_axis',(-1.,0.,0.));
#56111=DIRECTION('center_axis',(0.,0.0958457525203355,-0.995396198367168));
#56112=DIRECTION('ref_axis',(1.,2.68154995586863E-14,2.58203892945045E-15));
#56113=DIRECTION('center_axis',(-1.,0.,0.));
#56114=DIRECTION('ref_axis',(0.,-0.0958457525203355,0.995396198367168));
#56115=DIRECTION('',(0.,0.999992762491366,-0.00380459786137058));
#56116=DIRECTION('',(0.,-0.995396198367168,-0.0958457525203355));
#56117=DIRECTION('center_axis',(0.,-0.0958457525203355,0.995396198367168));
#56118=DIRECTION('ref_axis',(1.,0.,0.));
#56119=DIRECTION('',(0.,-0.995396198367168,-0.0958457525203355));
#56120=DIRECTION('center_axis',(0.,-0.0958457525203355,0.995396198367168));
#56121=DIRECTION('ref_axis',(1.,0.,0.));
#56122=DIRECTION('',(0.,0.995396198367168,0.0958457525203355));
#56123=DIRECTION('center_axis',(0.,-0.0958457525203355,0.995396198367168));
#56124=DIRECTION('ref_axis',(1.,0.,0.));
#56125=DIRECTION('center_axis',(0.70710678118655,-0.0677731815550566,0.703851401832732));
#56126=DIRECTION('ref_axis',(-8.71684762352402E-19,-0.995396198367168,-0.0958457525203355));
#56127=DIRECTION('',(0.707106781186545,0.0677731815550571,-0.703851401832737));
#56128=DIRECTION('',(0.,-0.995396198367168,-0.0958457525203355));
#56129=DIRECTION('',(-0.707106781186545,-0.0677731815550571,0.703851401832737));
#56130=DIRECTION('',(0.,0.995396198367168,0.0958457525203355));
#56131=DIRECTION('center_axis',(0.,0.0958457525203355,-0.995396198367168));
#56132=DIRECTION('ref_axis',(-1.,0.,0.));
#56133=DIRECTION('',(-0.707106781186545,0.0677731815550571,-0.703851401832737));
#56134=DIRECTION('center_axis',(0.,0.0958457525203355,-0.995396198367168));
#56135=DIRECTION('ref_axis',(1.,0.,0.));
#56136=DIRECTION('center_axis',(0.,-0.0958457525203355,0.995396198367168));
#56137=DIRECTION('ref_axis',(-1.,0.,0.));
#56138=DIRECTION('center_axis',(0.,0.0958457525203355,-0.995396198367168));
#56139=DIRECTION('ref_axis',(-1.,0.,0.));
#56140=DIRECTION('center_axis',(0.,0.0958457525203355,-0.995396198367168));
#56141=DIRECTION('ref_axis',(1.,0.,0.));
#56142=DIRECTION('',(0.707106781186545,-0.0677731815550571,0.703851401832737));
#56143=DIRECTION('center_axis',(0.,-0.0958457525203355,0.995396198367168));
#56144=DIRECTION('ref_axis',(-1.,0.,0.));
#56145=DIRECTION('center_axis',(-0.70710678118655,-0.0677731815550566,0.703851401832732));
#56146=DIRECTION('ref_axis',(-8.71684762352402E-19,0.995396198367168,0.0958457525203355));
#56147=DIRECTION('',(0.,0.995396198367168,0.0958457525203355));
#56148=DIRECTION('',(0.,-0.995396198367168,-0.0958457525203355));
#56149=DIRECTION('center_axis',(0.,-0.0958457525203355,0.995396198367168));
#56150=DIRECTION('ref_axis',(1.,0.,0.));
#56151=DIRECTION('center_axis',(0.,-0.995396198367168,-0.0958457525203355));
#56152=DIRECTION('ref_axis',(0.,0.0958457525203355,-0.995396198367168));
#56153=DIRECTION('center_axis',(0.,-0.995396198367168,-0.0958457525203355));
#56154=DIRECTION('ref_axis',(0.,0.0958457525203355,-0.995396198367168));
#56155=DIRECTION('center_axis',(0.,-0.995396198367168,-0.0958457525203355));
#56156=DIRECTION('ref_axis',(0.,0.0958457525203355,-0.995396198367168));
#56157=DIRECTION('center_axis',(0.,-0.995396198367168,-0.0958457525203355));
#56158=DIRECTION('ref_axis',(0.,0.0958457525203355,-0.995396198367168));
#56159=DIRECTION('center_axis',(0.,0.995396198367168,0.0958457525203355));
#56160=DIRECTION('ref_axis',(0.,-0.0958457525203355,0.995396198367168));
#56161=DIRECTION('center_axis',(0.,-0.995396198367168,-0.0958457525203355));
#56162=DIRECTION('ref_axis',(0.,0.0958457525203355,-0.995396198367168));
#56163=DIRECTION('center_axis',(0.,-0.0958457525203355,0.995396198367168));
#56164=DIRECTION('ref_axis',(1.,0.,0.));
#56165=DIRECTION('center_axis',(0.,-0.0958457525203355,0.995396198367168));
#56166=DIRECTION('ref_axis',(1.,0.,0.));
#56167=DIRECTION('center_axis',(0.,0.995396198367168,0.0958457525203355));
#56168=DIRECTION('ref_axis',(0.,-0.0958457525203355,0.995396198367168));
#56169=DIRECTION('center_axis',(0.,-0.995396198367168,-0.0958457525203355));
#56170=DIRECTION('ref_axis',(0.,0.0958457525203355,-0.995396198367168));
#56171=DIRECTION('center_axis',(0.,0.995396198367168,0.0958457525203355));
#56172=DIRECTION('ref_axis',(0.,-0.0958457525203355,0.995396198367168));
#56173=DIRECTION('center_axis',(0.,0.995396198367168,0.0958457525203355));
#56174=DIRECTION('ref_axis',(0.,-0.0958457525203355,0.995396198367168));
#56175=DIRECTION('center_axis',(0.,0.995396198367168,0.0958457525203355));
#56176=DIRECTION('ref_axis',(0.,-0.0958457525203355,0.995396198367168));
#56177=DIRECTION('center_axis',(0.,-0.0958457525203355,0.995396198367168));
#56178=DIRECTION('ref_axis',(1.,0.,0.));
#56179=DIRECTION('center_axis',(2.27199593986439E-14,0.999992816774261,
-0.00379030340206436));
#56180=DIRECTION('ref_axis',(0.999989540168118,1.7336051598704E-5,0.00457375707892275));
#56181=DIRECTION('center_axis',(0.,-0.993714552529049,-0.111943682680141));
#56182=DIRECTION('ref_axis',(0.,0.111943682680141,-0.993714552529049));
#56183=DIRECTION('center_axis',(0.,0.993714513001089,0.111944033565922));
#56184=DIRECTION('ref_axis',(0.,-0.111944033565922,0.993714513001089));
#56185=DIRECTION('center_axis',(-4.72985282513324E-19,-0.999992762691407,
0.00380454528272082));
#56186=DIRECTION('ref_axis',(1.,0.,-8.9883652947822E-12));
#56187=DIRECTION('center_axis',(1.05594678446211E-16,0.999992763056819,
-0.00380444923602132));
#56188=DIRECTION('ref_axis',(-7.13779962151542E-30,0.00380444923602132,
0.999992763056819));
#56189=DIRECTION('',(-3.137034099265E-5,0.999992710161712,-0.00381819844128151));
#56190=DIRECTION('center_axis',(-7.48214981472191E-6,0.999992732962714,
-0.00381234386965002));
#56191=DIRECTION('ref_axis',(0.396180495354598,0.00350335413362759,0.918165966266666));
#56192=DIRECTION('center_axis',(-2.39349104903811E-19,0.999992762286848,
-0.00380465161595737));
#56193=DIRECTION('ref_axis',(-1.,0.,4.51194621314849E-12));
#56194=DIRECTION('center_axis',(1.05594678446211E-16,-0.999992763056819,
0.00380444923602132));
#56195=DIRECTION('ref_axis',(-7.13779962151542E-30,-0.00380444923602132,
-0.999992763056819));
#56196=DIRECTION('',(-3.13703409353662E-5,-0.999992710161712,0.00381819844125435));
#56197=DIRECTION('center_axis',(0.,0.,-1.));
#56198=DIRECTION('ref_axis',(-1.,0.,0.));
#56199=DIRECTION('center_axis',(0.806909120659315,-0.558829829394105,-0.191329278408108));
#56200=DIRECTION('ref_axis',(-0.0849118339894143,-0.430294016492482,0.898686285540912));
#56201=DIRECTION('center_axis',(-0.835086390772497,0.517595659589867,0.186347667332585));
#56202=DIRECTION('ref_axis',(-0.526823571888351,-0.849974660859252,-1.43332569245731E-15));
#56203=DIRECTION('center_axis',(-0.835086381169178,-0.517595614917961,-0.186347834448014));
#56204=DIRECTION('ref_axis',(0.526823543416339,-0.849974678506515,9.57696623692639E-15));
#56205=DIRECTION('center_axis',(-0.806910218572417,-0.558828457766669,-0.191328654292922));
#56206=DIRECTION('ref_axis',(-0.590327175091889,0.751857820045504,0.293638629584822));
#56207=DIRECTION('center_axis',(-0.000872658099433895,0.999999542363192,
-0.0003920985191296));
#56208=DIRECTION('ref_axis',(0.999999619233104,0.000872658510876435,8.78244352734673E-7));
#56209=DIRECTION('center_axis',(0.747684665568336,3.91836177343196E-14,
-0.664053944249987));
#56210=DIRECTION('ref_axis',(-0.664053944249987,-4.89999445230472E-28,-0.747684665568336));
#56211=DIRECTION('center_axis',(0.,-1.,0.));
#56212=DIRECTION('ref_axis',(6.1857730524649E-16,0.,1.));
#56213=DIRECTION('center_axis',(0.747684665568342,2.64861897890156E-14,
0.664053944249981));
#56214=DIRECTION('ref_axis',(0.664053944249981,1.07359285114335E-28,-0.747684665568342));
#56215=DIRECTION('center_axis',(0.,-1.,0.));
#56216=DIRECTION('ref_axis',(0.,0.,-1.));
#56217=DIRECTION('center_axis',(0.,1.,0.));
#56218=DIRECTION('ref_axis',(0.,0.,1.));
#56219=DIRECTION('center_axis',(0.,0.,1.));
#56220=DIRECTION('ref_axis',(1.,0.,0.));
#56221=DIRECTION('center_axis',(0.000872658094508672,0.9999995423632,-0.000392098510262023));
#56222=DIRECTION('ref_axis',(-0.664054348043085,0.000872658504590579,0.747683797679344));
#56223=DIRECTION('center_axis',(-0.000872658095697528,0.999999542363198,
0.000392098510701838));
#56224=DIRECTION('ref_axis',(0.664054348059308,0.000872658505683059,-0.747683797664936));
#56225=DIRECTION('center_axis',(0.,0.,1.));
#56226=DIRECTION('ref_axis',(-0.708339837726479,-0.705871570676724,0.));
#56227=DIRECTION('center_axis',(-2.7852630342689E-14,-2.77555756158361E-14,
1.));
#56228=DIRECTION('ref_axis',(1.,-2.69380981579098E-30,2.7852630342689E-14));
#56229=DIRECTION('',(0.,0.,-1.));
#56230=DIRECTION('',(0.,0.,1.));
#56231=DIRECTION('center_axis',(0.000872658101303331,0.99999954236319,0.000392098519876546));
#56232=DIRECTION('ref_axis',(-0.999999619233102,0.000872658512739778,-8.78240000660092E-7));
#56233=DIRECTION('center_axis',(-0.781122637833718,-0.588690990414065,-0.208063313606701));
#56234=DIRECTION('ref_axis',(0.084909986182804,-0.430291959918125,0.898687444819529));
#56235=DIRECTION('center_axis',(0.,-0.333233134534162,0.94284446121751));
#56236=DIRECTION('ref_axis',(1.21997367885991E-7,0.942844461217503,0.333233134534159));
#56237=DIRECTION('center_axis',(0.,-0.333233134534161,0.942844461217511));
#56238=DIRECTION('ref_axis',(0.,-0.94284446121751,-0.333233134534161));
#56239=DIRECTION('center_axis',(0.00349620323913664,0.999992628662834,-0.00158719340524177));
#56240=DIRECTION('ref_axis',(-0.658393043656588,0.00349652845883053,0.752666177234869));
#56241=DIRECTION('center_axis',(0.00349064703388849,-0.999992652747851,
0.00158424543605274));
#56242=DIRECTION('ref_axis',(0.65839306424128,0.0034906514143529,0.75266618650746));
#56243=DIRECTION('',(0.,0.,1.));
#56244=DIRECTION('',(0.,0.,1.));
#56245=DIRECTION('center_axis',(6.57149350991999E-17,1.,0.));
#56246=DIRECTION('ref_axis',(1.,0.,0.));
#56247=DIRECTION('center_axis',(0.,0.333233134534161,-0.942844461217511));
#56248=DIRECTION('ref_axis',(0.,-0.94284446121751,-0.333233134534161));
#56249=DIRECTION('center_axis',(0.,-0.333233134534161,0.942844461217511));
#56250=DIRECTION('ref_axis',(-4.36200015704239E-7,0.942844461217421,0.33323313453413));
#56251=DIRECTION('center_axis',(-0.465249795635371,-0.834587947184017,-0.294967093209419));
#56252=DIRECTION('ref_axis',(0.885179432457581,-0.438657466759802,-0.15503870229703));
#56253=DIRECTION('center_axis',(0.0034906470338884,-0.999992652747851,-0.00158424543605272));
#56254=DIRECTION('ref_axis',(0.999993907657794,0.00349065141435304,8.88178419700162E-15));
#56255=DIRECTION('center_axis',(0.,-1.,0.));
#56256=DIRECTION('ref_axis',(2.09732571729144E-13,0.,-1.));
#56257=DIRECTION('center_axis',(0.00348618203660982,0.999992670981315,0.0015825670488381));
#56258=DIRECTION('ref_axis',(-0.999993923233682,0.00348618641343271,-7.06608105368013E-9));
#56259=DIRECTION('center_axis',(0.,-1.,0.));
#56260=DIRECTION('ref_axis',(0.,0.,-1.));
#56261=DIRECTION('center_axis',(-0.99999390765779,0.00349065141522374,0.));
#56262=DIRECTION('ref_axis',(-0.00349065141522374,-0.99999390765779,0.));
#56263=DIRECTION('center_axis',(0.99999390765779,0.00349065141522374,0.));
#56264=DIRECTION('ref_axis',(-0.00349065141522374,0.99999390765779,0.));
#56265=DIRECTION('center_axis',(0.,-1.,0.));
#56266=DIRECTION('ref_axis',(0.835314349256296,0.,0.549772623842377));
#56267=DIRECTION('center_axis',(-4.38167354516293E-13,-1.,-6.55088140642138E-13));
#56268=DIRECTION('ref_axis',(0.835314349256533,-5.8579526746184E-15,-0.549772623842016));
#56269=DIRECTION('center_axis',(0.,-1.,0.));
#56270=DIRECTION('ref_axis',(-7.6571373978539E-16,0.,1.));
#56271=DIRECTION('center_axis',(0.,-0.333233134534162,0.94284446121751));
#56272=DIRECTION('ref_axis',(0.,-0.94284446121751,-0.333233134534162));
#56273=DIRECTION('center_axis',(0.,0.333233134534162,-0.94284446121751));
#56274=DIRECTION('ref_axis',(0.,0.94284446121751,0.333233134534162));
#56275=DIRECTION('center_axis',(-4.48634137349537E-12,0.333233134518338,
-0.942844461223103));
#56276=DIRECTION('ref_axis',(0.26200914408981,0.909906558382195,0.321591765171923));
#56277=DIRECTION('center_axis',(1.18843000706592E-12,0.333233134529897,
-0.942844461219018));
#56278=DIRECTION('ref_axis',(-0.254118622727095,0.911893761488375,0.322294110001823));
#56279=DIRECTION('center_axis',(-1.,0.,0.));
#56280=DIRECTION('ref_axis',(0.,0.,1.));
#56281=DIRECTION('',(0.,0.,-1.));
#56282=DIRECTION('center_axis',(1.,0.,0.));
#56283=DIRECTION('ref_axis',(0.,0.,-1.));
#56284=DIRECTION('',(0.,0.,-1.));
#56285=DIRECTION('center_axis',(0.,0.,-1.));
#56286=DIRECTION('ref_axis',(-1.,0.,0.));
#56287=DIRECTION('center_axis',(0.,0.333233134534162,-0.94284446121751));
#56288=DIRECTION('ref_axis',(0.,0.94284446121751,0.333233134534162));
#56289=DIRECTION('center_axis',(0.,-0.333233134534159,0.942844461217511));
#56290=DIRECTION('ref_axis',(0.,-0.942844461217511,-0.333233134534159));
#56291=DIRECTION('center_axis',(0.,0.333233134534162,-0.94284446121751));
#56292=DIRECTION('ref_axis',(0.,0.94284446121751,0.333233134534162));
#56293=DIRECTION('center_axis',(0.,-0.333233134534159,0.942844461217511));
#56294=DIRECTION('ref_axis',(0.,-0.942844461217511,-0.333233134534159));
#56295=DIRECTION('center_axis',(0.,0.333233134534162,-0.94284446121751));
#56296=DIRECTION('ref_axis',(0.,0.94284446121751,0.333233134534162));
#56297=DIRECTION('center_axis',(0.,-0.333233134534159,0.942844461217511));
#56298=DIRECTION('ref_axis',(0.,-0.942844461217511,-0.333233134534159));
#56299=DIRECTION('center_axis',(0.,0.333233134534162,-0.94284446121751));
#56300=DIRECTION('ref_axis',(0.,0.94284446121751,0.333233134534162));
#56301=DIRECTION('center_axis',(0.,-0.333233134534159,0.942844461217511));
#56302=DIRECTION('ref_axis',(0.,-0.942844461217511,-0.333233134534159));
#56303=DIRECTION('center_axis',(0.,0.333233134534162,-0.94284446121751));
#56304=DIRECTION('ref_axis',(0.,0.94284446121751,0.333233134534162));
#56305=DIRECTION('center_axis',(0.,-0.333233134534159,0.942844461217511));
#56306=DIRECTION('ref_axis',(0.,-0.942844461217511,-0.333233134534159));
#56307=DIRECTION('center_axis',(0.,0.333233134534162,-0.94284446121751));
#56308=DIRECTION('ref_axis',(0.,0.94284446121751,0.333233134534162));
#56309=DIRECTION('center_axis',(0.,-0.333233134534159,0.942844461217511));
#56310=DIRECTION('ref_axis',(0.,-0.942844461217511,-0.333233134534159));
#56311=DIRECTION('center_axis',(0.,0.333233134534162,-0.94284446121751));
#56312=DIRECTION('ref_axis',(0.,0.94284446121751,0.333233134534162));
#56313=DIRECTION('center_axis',(0.,-0.333233134534159,0.942844461217511));
#56314=DIRECTION('ref_axis',(0.,-0.942844461217511,-0.333233134534159));
#56315=DIRECTION('center_axis',(0.,0.333233134534162,-0.94284446121751));
#56316=DIRECTION('ref_axis',(0.,0.94284446121751,0.333233134534162));
#56317=DIRECTION('center_axis',(0.,-0.333233134534159,0.942844461217511));
#56318=DIRECTION('ref_axis',(0.,-0.942844461217511,-0.333233134534159));
#56319=DIRECTION('center_axis',(0.,0.333233134534162,-0.94284446121751));
#56320=DIRECTION('ref_axis',(0.,0.94284446121751,0.333233134534162));
#56321=DIRECTION('center_axis',(0.,-0.333233134534159,0.942844461217511));
#56322=DIRECTION('ref_axis',(0.,-0.942844461217511,-0.333233134534159));
#56323=DIRECTION('center_axis',(0.,0.333233134534162,-0.94284446121751));
#56324=DIRECTION('ref_axis',(0.,0.94284446121751,0.333233134534162));
#56325=DIRECTION('center_axis',(0.,-0.333233134534159,0.942844461217511));
#56326=DIRECTION('ref_axis',(0.,-0.942844461217511,-0.333233134534159));
#56327=DIRECTION('center_axis',(0.,0.333233134534162,-0.94284446121751));
#56328=DIRECTION('ref_axis',(0.,0.94284446121751,0.333233134534162));
#56329=DIRECTION('center_axis',(0.,-0.333233134534159,0.942844461217511));
#56330=DIRECTION('ref_axis',(0.,-0.942844461217511,-0.333233134534159));
#56331=DIRECTION('center_axis',(0.,0.333233134534162,-0.94284446121751));
#56332=DIRECTION('ref_axis',(0.,0.94284446121751,0.333233134534162));
#56333=DIRECTION('center_axis',(0.,-0.333233134534159,0.942844461217511));
#56334=DIRECTION('ref_axis',(0.,-0.942844461217511,-0.333233134534159));
#56335=DIRECTION('center_axis',(0.,0.333233134534162,-0.94284446121751));
#56336=DIRECTION('ref_axis',(0.,0.94284446121751,0.333233134534162));
#56337=DIRECTION('center_axis',(0.,-0.333233134534159,0.942844461217511));
#56338=DIRECTION('ref_axis',(0.,-0.942844461217511,-0.333233134534159));
#56339=DIRECTION('center_axis',(0.,0.333233134534162,-0.94284446121751));
#56340=DIRECTION('ref_axis',(0.,0.94284446121751,0.333233134534162));
#56341=DIRECTION('center_axis',(0.,-0.333233134534159,0.942844461217511));
#56342=DIRECTION('ref_axis',(0.,-0.942844461217511,-0.333233134534159));
#56343=DIRECTION('center_axis',(0.,0.333233134534162,-0.94284446121751));
#56344=DIRECTION('ref_axis',(0.,0.94284446121751,0.333233134534162));
#56345=DIRECTION('center_axis',(0.,-0.333233134534159,0.942844461217511));
#56346=DIRECTION('ref_axis',(0.,-0.942844461217511,-0.333233134534159));
#56347=DIRECTION('center_axis',(0.,0.333233134534162,-0.94284446121751));
#56348=DIRECTION('ref_axis',(0.,0.94284446121751,0.333233134534162));
#56349=DIRECTION('center_axis',(0.,-0.333233134534159,0.942844461217511));
#56350=DIRECTION('ref_axis',(0.,-0.942844461217511,-0.333233134534159));
#56351=DIRECTION('center_axis',(0.,0.333233134534162,-0.94284446121751));
#56352=DIRECTION('ref_axis',(0.,0.94284446121751,0.333233134534162));
#56353=DIRECTION('center_axis',(0.,-0.333233134534159,0.942844461217511));
#56354=DIRECTION('ref_axis',(0.,-0.942844461217511,-0.333233134534159));
#56355=DIRECTION('center_axis',(0.,0.333233134534162,-0.94284446121751));
#56356=DIRECTION('ref_axis',(0.,0.94284446121751,0.333233134534162));
#56357=DIRECTION('center_axis',(0.,-0.333233134534159,0.942844461217511));
#56358=DIRECTION('ref_axis',(0.,-0.942844461217511,-0.333233134534159));
#56359=DIRECTION('center_axis',(0.,0.333233134534162,-0.94284446121751));
#56360=DIRECTION('ref_axis',(0.,0.94284446121751,0.333233134534162));
#56361=DIRECTION('center_axis',(0.,-0.333233134534159,0.942844461217511));
#56362=DIRECTION('ref_axis',(0.,-0.942844461217511,-0.333233134534159));
#56363=DIRECTION('center_axis',(0.,0.333233134534162,-0.94284446121751));
#56364=DIRECTION('ref_axis',(0.,0.94284446121751,0.333233134534162));
#56365=DIRECTION('center_axis',(0.,-0.333233134534159,0.942844461217511));
#56366=DIRECTION('ref_axis',(0.,-0.942844461217511,-0.333233134534159));
#56367=DIRECTION('center_axis',(0.,0.333233134534162,-0.94284446121751));
#56368=DIRECTION('ref_axis',(0.,0.94284446121751,0.333233134534162));
#56369=DIRECTION('center_axis',(0.,-0.333233134534159,0.942844461217511));
#56370=DIRECTION('ref_axis',(0.,-0.942844461217511,-0.333233134534159));
#56371=DIRECTION('center_axis',(0.,0.333233134534162,-0.94284446121751));
#56372=DIRECTION('ref_axis',(0.,0.94284446121751,0.333233134534162));
#56373=DIRECTION('center_axis',(0.,-0.333233134534159,0.942844461217511));
#56374=DIRECTION('ref_axis',(0.,-0.942844461217511,-0.333233134534159));
#56375=DIRECTION('center_axis',(0.,0.333233134534162,-0.94284446121751));
#56376=DIRECTION('ref_axis',(0.,0.94284446121751,0.333233134534162));
#56377=DIRECTION('center_axis',(0.,-0.333233134534159,0.942844461217511));
#56378=DIRECTION('ref_axis',(0.,-0.942844461217511,-0.333233134534159));
#56379=DIRECTION('center_axis',(0.,0.333233134534162,-0.94284446121751));
#56380=DIRECTION('ref_axis',(0.,0.94284446121751,0.333233134534162));
#56381=DIRECTION('center_axis',(0.,-0.333233134534159,0.942844461217511));
#56382=DIRECTION('ref_axis',(0.,-0.942844461217511,-0.333233134534159));
#56383=DIRECTION('center_axis',(0.,0.333233134534162,-0.94284446121751));
#56384=DIRECTION('ref_axis',(0.,0.94284446121751,0.333233134534162));
#56385=DIRECTION('center_axis',(0.,-0.333233134534159,0.942844461217511));
#56386=DIRECTION('ref_axis',(0.,-0.942844461217511,-0.333233134534159));
#56387=DIRECTION('center_axis',(0.,0.333233134534162,-0.94284446121751));
#56388=DIRECTION('ref_axis',(0.,0.94284446121751,0.333233134534162));
#56389=DIRECTION('center_axis',(0.,-0.333233134534159,0.942844461217511));
#56390=DIRECTION('ref_axis',(0.,-0.942844461217511,-0.333233134534159));
#56391=DIRECTION('center_axis',(0.,0.333233134534162,-0.94284446121751));
#56392=DIRECTION('ref_axis',(0.,0.94284446121751,0.333233134534162));
#56393=DIRECTION('center_axis',(0.,-0.333233134534159,0.942844461217511));
#56394=DIRECTION('ref_axis',(0.,-0.942844461217511,-0.333233134534159));
#56395=DIRECTION('center_axis',(0.,0.333233134534162,-0.94284446121751));
#56396=DIRECTION('ref_axis',(0.,0.94284446121751,0.333233134534162));
#56397=DIRECTION('center_axis',(0.,-0.333233134534159,0.942844461217511));
#56398=DIRECTION('ref_axis',(0.,-0.942844461217511,-0.333233134534159));
#56399=DIRECTION('center_axis',(0.,0.333233134534162,-0.94284446121751));
#56400=DIRECTION('ref_axis',(0.,0.94284446121751,0.333233134534162));
#56401=DIRECTION('center_axis',(0.,-0.333233134534159,0.942844461217511));
#56402=DIRECTION('ref_axis',(0.,-0.942844461217511,-0.333233134534159));
#56403=DIRECTION('center_axis',(0.,0.333233134534162,-0.94284446121751));
#56404=DIRECTION('ref_axis',(0.,0.94284446121751,0.333233134534162));
#56405=DIRECTION('center_axis',(0.,-0.333233134534159,0.942844461217511));
#56406=DIRECTION('ref_axis',(0.,-0.942844461217511,-0.333233134534159));
#56407=DIRECTION('center_axis',(0.,0.333233134534162,-0.94284446121751));
#56408=DIRECTION('ref_axis',(0.,0.94284446121751,0.333233134534162));
#56409=DIRECTION('center_axis',(0.,-0.333233134534159,0.942844461217511));
#56410=DIRECTION('ref_axis',(0.,-0.942844461217511,-0.333233134534159));
#56411=DIRECTION('center_axis',(0.,0.333233134534162,-0.94284446121751));
#56412=DIRECTION('ref_axis',(0.,0.94284446121751,0.333233134534162));
#56413=DIRECTION('center_axis',(0.,-0.333233134534159,0.942844461217511));
#56414=DIRECTION('ref_axis',(0.,-0.942844461217511,-0.333233134534159));
#56415=DIRECTION('center_axis',(0.,0.333233134534162,-0.94284446121751));
#56416=DIRECTION('ref_axis',(0.,0.94284446121751,0.333233134534162));
#56417=DIRECTION('center_axis',(0.,-0.333233134534159,0.942844461217511));
#56418=DIRECTION('ref_axis',(0.,-0.942844461217511,-0.333233134534159));
#56419=DIRECTION('center_axis',(0.,0.333233134534162,-0.94284446121751));
#56420=DIRECTION('ref_axis',(0.,0.94284446121751,0.333233134534162));
#56421=DIRECTION('center_axis',(0.,-0.333233134534159,0.942844461217511));
#56422=DIRECTION('ref_axis',(0.,-0.942844461217511,-0.333233134534159));
#56423=DIRECTION('center_axis',(0.,0.333233134534162,-0.94284446121751));
#56424=DIRECTION('ref_axis',(0.,0.94284446121751,0.333233134534162));
#56425=DIRECTION('center_axis',(0.,-0.333233134534159,0.942844461217511));
#56426=DIRECTION('ref_axis',(0.,-0.942844461217511,-0.333233134534159));
#56427=DIRECTION('center_axis',(0.,0.333233134534162,-0.94284446121751));
#56428=DIRECTION('ref_axis',(0.,0.94284446121751,0.333233134534162));
#56429=DIRECTION('center_axis',(0.,-0.333233134534159,0.942844461217511));
#56430=DIRECTION('ref_axis',(0.,-0.942844461217511,-0.333233134534159));
#56431=DIRECTION('center_axis',(0.,0.333233134534162,-0.94284446121751));
#56432=DIRECTION('ref_axis',(0.,0.94284446121751,0.333233134534162));
#56433=DIRECTION('center_axis',(0.,-0.333233134534159,0.942844461217511));
#56434=DIRECTION('ref_axis',(0.,-0.942844461217511,-0.333233134534159));
#56435=DIRECTION('center_axis',(0.,0.333233134534162,-0.94284446121751));
#56436=DIRECTION('ref_axis',(0.,0.94284446121751,0.333233134534162));
#56437=DIRECTION('center_axis',(0.,-0.333233134534159,0.942844461217511));
#56438=DIRECTION('ref_axis',(0.,-0.942844461217511,-0.333233134534159));
#56439=DIRECTION('center_axis',(0.,0.333233134534162,-0.94284446121751));
#56440=DIRECTION('ref_axis',(0.,0.94284446121751,0.333233134534162));
#56441=DIRECTION('center_axis',(0.,-0.333233134534159,0.942844461217511));
#56442=DIRECTION('ref_axis',(0.,-0.942844461217511,-0.333233134534159));
#56443=DIRECTION('center_axis',(0.,0.333233134534162,-0.94284446121751));
#56444=DIRECTION('ref_axis',(0.,0.94284446121751,0.333233134534162));
#56445=DIRECTION('center_axis',(0.,-0.333233134534159,0.942844461217511));
#56446=DIRECTION('ref_axis',(0.,-0.942844461217511,-0.333233134534159));
#56447=DIRECTION('center_axis',(0.,0.333233134534162,-0.94284446121751));
#56448=DIRECTION('ref_axis',(0.,0.94284446121751,0.333233134534162));
#56449=DIRECTION('center_axis',(0.,-0.333233134534159,0.942844461217511));
#56450=DIRECTION('ref_axis',(0.,-0.942844461217511,-0.333233134534159));
#56451=DIRECTION('center_axis',(0.,0.333233134534162,-0.94284446121751));
#56452=DIRECTION('ref_axis',(0.,0.94284446121751,0.333233134534162));
#56453=DIRECTION('center_axis',(0.,-0.333233134534159,0.942844461217511));
#56454=DIRECTION('ref_axis',(0.,-0.942844461217511,-0.333233134534159));
#56455=DIRECTION('center_axis',(0.,0.333233134534162,-0.94284446121751));
#56456=DIRECTION('ref_axis',(0.,0.94284446121751,0.333233134534162));
#56457=DIRECTION('center_axis',(0.,-0.333233134534159,0.942844461217511));
#56458=DIRECTION('ref_axis',(0.,-0.942844461217511,-0.333233134534159));
#56459=DIRECTION('center_axis',(0.,0.333233134534162,-0.94284446121751));
#56460=DIRECTION('ref_axis',(0.,0.94284446121751,0.333233134534162));
#56461=DIRECTION('center_axis',(0.,-0.333233134534159,0.942844461217511));
#56462=DIRECTION('ref_axis',(0.,-0.942844461217511,-0.333233134534159));
#56463=DIRECTION('center_axis',(0.,0.333233134534162,-0.94284446121751));
#56464=DIRECTION('ref_axis',(0.,0.94284446121751,0.333233134534162));
#56465=DIRECTION('center_axis',(0.,-0.333233134534159,0.942844461217511));
#56466=DIRECTION('ref_axis',(0.,-0.942844461217511,-0.333233134534159));
#56467=DIRECTION('center_axis',(0.,0.333233134534162,-0.94284446121751));
#56468=DIRECTION('ref_axis',(0.,0.94284446121751,0.333233134534162));
#56469=DIRECTION('center_axis',(0.,-0.333233134534159,0.942844461217511));
#56470=DIRECTION('ref_axis',(0.,-0.942844461217511,-0.333233134534159));
#56471=DIRECTION('center_axis',(0.,0.333233134534162,-0.94284446121751));
#56472=DIRECTION('ref_axis',(0.,0.94284446121751,0.333233134534162));
#56473=DIRECTION('center_axis',(0.,-0.333233134534159,0.942844461217511));
#56474=DIRECTION('ref_axis',(0.,-0.942844461217511,-0.333233134534159));
#56475=DIRECTION('center_axis',(0.,0.333233134534162,-0.94284446121751));
#56476=DIRECTION('ref_axis',(0.,0.94284446121751,0.333233134534162));
#56477=DIRECTION('center_axis',(0.,-0.333233134534159,0.942844461217511));
#56478=DIRECTION('ref_axis',(0.,-0.942844461217511,-0.333233134534159));
#56479=DIRECTION('center_axis',(0.,0.333233134534162,-0.94284446121751));
#56480=DIRECTION('ref_axis',(0.,0.94284446121751,0.333233134534162));
#56481=DIRECTION('center_axis',(0.,-0.333233134534159,0.942844461217511));
#56482=DIRECTION('ref_axis',(0.,-0.942844461217511,-0.333233134534159));
#56483=DIRECTION('center_axis',(0.,0.333233134534162,-0.94284446121751));
#56484=DIRECTION('ref_axis',(0.,0.94284446121751,0.333233134534162));
#56485=DIRECTION('center_axis',(0.,-0.333233134534159,0.942844461217511));
#56486=DIRECTION('ref_axis',(0.,-0.942844461217511,-0.333233134534159));
#56487=DIRECTION('center_axis',(0.,0.333233134534162,-0.94284446121751));
#56488=DIRECTION('ref_axis',(0.,0.94284446121751,0.333233134534162));
#56489=DIRECTION('center_axis',(0.,-0.333233134534159,0.942844461217511));
#56490=DIRECTION('ref_axis',(0.,-0.942844461217511,-0.333233134534159));
#56491=DIRECTION('center_axis',(0.,0.333233134534162,-0.94284446121751));
#56492=DIRECTION('ref_axis',(0.,0.94284446121751,0.333233134534162));
#56493=DIRECTION('center_axis',(0.,-0.333233134534159,0.942844461217511));
#56494=DIRECTION('ref_axis',(0.,-0.942844461217511,-0.333233134534159));
#56495=DIRECTION('center_axis',(0.,0.333233134534162,-0.94284446121751));
#56496=DIRECTION('ref_axis',(0.,0.94284446121751,0.333233134534162));
#56497=DIRECTION('center_axis',(0.,-0.333233134534159,0.942844461217511));
#56498=DIRECTION('ref_axis',(0.,-0.942844461217511,-0.333233134534159));
#56499=DIRECTION('center_axis',(0.,0.333233134534162,-0.94284446121751));
#56500=DIRECTION('ref_axis',(0.,0.94284446121751,0.333233134534162));
#56501=DIRECTION('center_axis',(0.,-0.333233134534159,0.942844461217511));
#56502=DIRECTION('ref_axis',(0.,-0.942844461217511,-0.333233134534159));
#56503=DIRECTION('center_axis',(0.,0.333233134534162,-0.94284446121751));
#56504=DIRECTION('ref_axis',(0.,0.94284446121751,0.333233134534162));
#56505=DIRECTION('center_axis',(0.,-0.333233134534159,0.942844461217511));
#56506=DIRECTION('ref_axis',(0.,-0.942844461217511,-0.333233134534159));
#56507=DIRECTION('center_axis',(0.,0.333233134534162,-0.94284446121751));
#56508=DIRECTION('ref_axis',(0.,0.94284446121751,0.333233134534162));
#56509=DIRECTION('center_axis',(0.,-0.333233134534159,0.942844461217511));
#56510=DIRECTION('ref_axis',(0.,-0.942844461217511,-0.333233134534159));
#56511=DIRECTION('center_axis',(0.,0.333233134534162,-0.94284446121751));
#56512=DIRECTION('ref_axis',(0.,0.94284446121751,0.333233134534162));
#56513=DIRECTION('center_axis',(0.,-0.333233134534159,0.942844461217511));
#56514=DIRECTION('ref_axis',(0.,-0.942844461217511,-0.333233134534159));
#56515=DIRECTION('center_axis',(0.,0.333233134534162,-0.94284446121751));
#56516=DIRECTION('ref_axis',(0.,0.94284446121751,0.333233134534162));
#56517=DIRECTION('center_axis',(0.,-0.333233134534159,0.942844461217511));
#56518=DIRECTION('ref_axis',(0.,-0.942844461217511,-0.333233134534159));
#56519=DIRECTION('center_axis',(0.,0.333233134534162,-0.94284446121751));
#56520=DIRECTION('ref_axis',(0.,0.94284446121751,0.333233134534162));
#56521=DIRECTION('center_axis',(0.,-0.333233134534159,0.942844461217511));
#56522=DIRECTION('ref_axis',(0.,-0.942844461217511,-0.333233134534159));
#56523=DIRECTION('center_axis',(0.,0.333233134534162,-0.94284446121751));
#56524=DIRECTION('ref_axis',(0.,0.94284446121751,0.333233134534162));
#56525=DIRECTION('center_axis',(0.,-0.333233134534159,0.942844461217511));
#56526=DIRECTION('ref_axis',(0.,-0.942844461217511,-0.333233134534159));
#56527=DIRECTION('center_axis',(0.,0.333233134534162,-0.94284446121751));
#56528=DIRECTION('ref_axis',(0.,0.94284446121751,0.333233134534162));
#56529=DIRECTION('center_axis',(0.,-0.333233134534159,0.942844461217511));
#56530=DIRECTION('ref_axis',(0.,-0.942844461217511,-0.333233134534159));
#56531=DIRECTION('center_axis',(0.,0.333233134534162,-0.94284446121751));
#56532=DIRECTION('ref_axis',(0.,0.94284446121751,0.333233134534162));
#56533=DIRECTION('center_axis',(0.,-0.333233134534159,0.942844461217511));
#56534=DIRECTION('ref_axis',(0.,-0.942844461217511,-0.333233134534159));
#56535=DIRECTION('center_axis',(0.,0.333233134534162,-0.94284446121751));
#56536=DIRECTION('ref_axis',(0.,0.94284446121751,0.333233134534162));
#56537=DIRECTION('center_axis',(0.,-0.333233134534159,0.942844461217511));
#56538=DIRECTION('ref_axis',(0.,-0.942844461217511,-0.333233134534159));
#56539=DIRECTION('center_axis',(0.,0.333233134534162,-0.94284446121751));
#56540=DIRECTION('ref_axis',(0.,0.94284446121751,0.333233134534162));
#56541=DIRECTION('center_axis',(0.,-0.333233134534159,0.942844461217511));
#56542=DIRECTION('ref_axis',(0.,-0.942844461217511,-0.333233134534159));
#56543=DIRECTION('center_axis',(0.,0.333233134534162,-0.94284446121751));
#56544=DIRECTION('ref_axis',(0.,0.94284446121751,0.333233134534162));
#56545=DIRECTION('center_axis',(0.,-0.333233134534159,0.942844461217511));
#56546=DIRECTION('ref_axis',(0.,-0.942844461217511,-0.333233134534159));
#56547=DIRECTION('center_axis',(0.,0.333233134534162,-0.94284446121751));
#56548=DIRECTION('ref_axis',(0.,0.94284446121751,0.333233134534162));
#56549=DIRECTION('center_axis',(0.,-0.333233134534159,0.942844461217511));
#56550=DIRECTION('ref_axis',(0.,-0.942844461217511,-0.333233134534159));
#56551=DIRECTION('center_axis',(0.,0.333233134534162,-0.94284446121751));
#56552=DIRECTION('ref_axis',(0.,0.94284446121751,0.333233134534162));
#56553=DIRECTION('center_axis',(0.,-0.333233134534159,0.942844461217511));
#56554=DIRECTION('ref_axis',(0.,-0.942844461217511,-0.333233134534159));
#56555=DIRECTION('center_axis',(0.,0.333233134534162,-0.94284446121751));
#56556=DIRECTION('ref_axis',(0.,0.94284446121751,0.333233134534162));
#56557=DIRECTION('center_axis',(0.,-0.333233134534159,0.942844461217511));
#56558=DIRECTION('ref_axis',(0.,-0.942844461217511,-0.333233134534159));
#56559=DIRECTION('center_axis',(0.,0.333233134534162,-0.94284446121751));
#56560=DIRECTION('ref_axis',(0.,0.94284446121751,0.333233134534162));
#56561=DIRECTION('center_axis',(0.,-0.333233134534159,0.942844461217511));
#56562=DIRECTION('ref_axis',(0.,-0.942844461217511,-0.333233134534159));
#56563=DIRECTION('center_axis',(0.,0.333233134534162,-0.94284446121751));
#56564=DIRECTION('ref_axis',(0.,0.94284446121751,0.333233134534162));
#56565=DIRECTION('center_axis',(0.,-0.333233134534159,0.942844461217511));
#56566=DIRECTION('ref_axis',(0.,-0.942844461217511,-0.333233134534159));
#56567=DIRECTION('center_axis',(0.,0.333233134534162,-0.94284446121751));
#56568=DIRECTION('ref_axis',(0.,0.94284446121751,0.333233134534162));
#56569=DIRECTION('center_axis',(0.,-0.333233134534159,0.942844461217511));
#56570=DIRECTION('ref_axis',(0.,-0.942844461217511,-0.333233134534159));
#56571=DIRECTION('center_axis',(0.,0.333233134534162,-0.94284446121751));
#56572=DIRECTION('ref_axis',(0.,0.94284446121751,0.333233134534162));
#56573=DIRECTION('center_axis',(0.,-0.333233134534159,0.942844461217511));
#56574=DIRECTION('ref_axis',(0.,-0.942844461217511,-0.333233134534159));
#56575=DIRECTION('center_axis',(0.,0.333233134534162,-0.94284446121751));
#56576=DIRECTION('ref_axis',(0.,0.94284446121751,0.333233134534162));
#56577=DIRECTION('center_axis',(0.,-0.333233134534159,0.942844461217511));
#56578=DIRECTION('ref_axis',(0.,-0.942844461217511,-0.333233134534159));
#56579=DIRECTION('center_axis',(0.,0.333233134534162,-0.94284446121751));
#56580=DIRECTION('ref_axis',(0.,0.94284446121751,0.333233134534162));
#56581=DIRECTION('center_axis',(0.,-0.333233134534159,0.942844461217511));
#56582=DIRECTION('ref_axis',(0.,-0.942844461217511,-0.333233134534159));
#56583=DIRECTION('center_axis',(0.,0.333233134534162,-0.94284446121751));
#56584=DIRECTION('ref_axis',(0.,0.94284446121751,0.333233134534162));
#56585=DIRECTION('center_axis',(0.,-0.333233134534159,0.942844461217511));
#56586=DIRECTION('ref_axis',(0.,-0.942844461217511,-0.333233134534159));
#56587=DIRECTION('center_axis',(0.,0.333233134534162,-0.94284446121751));
#56588=DIRECTION('ref_axis',(0.,0.94284446121751,0.333233134534162));
#56589=DIRECTION('center_axis',(0.,-0.333233134534159,0.942844461217511));
#56590=DIRECTION('ref_axis',(0.,-0.942844461217511,-0.333233134534159));
#56591=DIRECTION('center_axis',(0.,0.333233134534162,-0.94284446121751));
#56592=DIRECTION('ref_axis',(0.,0.94284446121751,0.333233134534162));
#56593=DIRECTION('center_axis',(0.,-0.333233134534159,0.942844461217511));
#56594=DIRECTION('ref_axis',(0.,-0.942844461217511,-0.333233134534159));
#56595=DIRECTION('center_axis',(0.,0.333233134534162,-0.94284446121751));
#56596=DIRECTION('ref_axis',(0.,0.94284446121751,0.333233134534162));
#56597=DIRECTION('center_axis',(0.,-0.333233134534159,0.942844461217511));
#56598=DIRECTION('ref_axis',(0.,-0.942844461217511,-0.333233134534159));
#56599=DIRECTION('center_axis',(0.,0.333233134534162,-0.94284446121751));
#56600=DIRECTION('ref_axis',(0.,0.94284446121751,0.333233134534162));
#56601=DIRECTION('center_axis',(0.,-0.333233134534159,0.942844461217511));
#56602=DIRECTION('ref_axis',(0.,-0.942844461217511,-0.333233134534159));
#56603=DIRECTION('center_axis',(0.,0.333233134534162,-0.94284446121751));
#56604=DIRECTION('ref_axis',(0.,0.94284446121751,0.333233134534162));
#56605=DIRECTION('center_axis',(0.,-0.333233134534159,0.942844461217511));
#56606=DIRECTION('ref_axis',(0.,-0.942844461217511,-0.333233134534159));
#56607=DIRECTION('center_axis',(0.,0.333233134534162,-0.94284446121751));
#56608=DIRECTION('ref_axis',(0.,0.94284446121751,0.333233134534162));
#56609=DIRECTION('center_axis',(0.,-0.333233134534159,0.942844461217511));
#56610=DIRECTION('ref_axis',(0.,-0.942844461217511,-0.333233134534159));
#56611=DIRECTION('center_axis',(0.,0.333233134534162,-0.94284446121751));
#56612=DIRECTION('ref_axis',(0.,0.94284446121751,0.333233134534162));
#56613=DIRECTION('center_axis',(0.,-0.333233134534159,0.942844461217511));
#56614=DIRECTION('ref_axis',(0.,-0.942844461217511,-0.333233134534159));
#56615=DIRECTION('center_axis',(0.,0.333233134534162,-0.94284446121751));
#56616=DIRECTION('ref_axis',(0.,0.94284446121751,0.333233134534162));
#56617=DIRECTION('center_axis',(0.,-0.333233134534159,0.942844461217511));
#56618=DIRECTION('ref_axis',(0.,-0.942844461217511,-0.333233134534159));
#56619=DIRECTION('center_axis',(0.,0.333233134534162,-0.94284446121751));
#56620=DIRECTION('ref_axis',(0.,0.94284446121751,0.333233134534162));
#56621=DIRECTION('center_axis',(0.,-0.333233134534159,0.942844461217511));
#56622=DIRECTION('ref_axis',(0.,-0.942844461217511,-0.333233134534159));
#56623=DIRECTION('center_axis',(0.,0.333233134534162,-0.94284446121751));
#56624=DIRECTION('ref_axis',(0.,0.94284446121751,0.333233134534162));
#56625=DIRECTION('center_axis',(0.,-0.333233134534159,0.942844461217511));
#56626=DIRECTION('ref_axis',(0.,-0.942844461217511,-0.333233134534159));
#56627=DIRECTION('center_axis',(0.,0.333233134534162,-0.94284446121751));
#56628=DIRECTION('ref_axis',(0.,0.94284446121751,0.333233134534162));
#56629=DIRECTION('center_axis',(0.,-0.333233134534159,0.942844461217511));
#56630=DIRECTION('ref_axis',(0.,-0.942844461217511,-0.333233134534159));
#56631=DIRECTION('center_axis',(0.,0.333233134534162,-0.94284446121751));
#56632=DIRECTION('ref_axis',(0.,0.94284446121751,0.333233134534162));
#56633=DIRECTION('center_axis',(0.,-0.333233134534159,0.942844461217511));
#56634=DIRECTION('ref_axis',(0.,-0.942844461217511,-0.333233134534159));
#56635=DIRECTION('center_axis',(0.,0.333233134534162,-0.94284446121751));
#56636=DIRECTION('ref_axis',(0.,0.94284446121751,0.333233134534162));
#56637=DIRECTION('center_axis',(0.,-0.333233134534159,0.942844461217511));
#56638=DIRECTION('ref_axis',(0.,-0.942844461217511,-0.333233134534159));
#56639=DIRECTION('center_axis',(0.,0.333233134534162,-0.94284446121751));
#56640=DIRECTION('ref_axis',(0.,0.94284446121751,0.333233134534162));
#56641=DIRECTION('center_axis',(0.,-0.333233134534159,0.942844461217511));
#56642=DIRECTION('ref_axis',(0.,-0.942844461217511,-0.333233134534159));
#56643=DIRECTION('center_axis',(0.,0.333233134534162,-0.94284446121751));
#56644=DIRECTION('ref_axis',(0.,0.94284446121751,0.333233134534162));
#56645=DIRECTION('center_axis',(0.,-0.333233134534159,0.942844461217511));
#56646=DIRECTION('ref_axis',(0.,-0.942844461217511,-0.333233134534159));
#56647=DIRECTION('center_axis',(0.,0.333233134534162,-0.94284446121751));
#56648=DIRECTION('ref_axis',(0.,0.94284446121751,0.333233134534162));
#56649=DIRECTION('center_axis',(0.,-0.333233134534159,0.942844461217511));
#56650=DIRECTION('ref_axis',(0.,-0.942844461217511,-0.333233134534159));
#56651=DIRECTION('center_axis',(0.,0.333233134534162,-0.94284446121751));
#56652=DIRECTION('ref_axis',(0.,0.94284446121751,0.333233134534162));
#56653=DIRECTION('center_axis',(0.,-0.333233134534159,0.942844461217511));
#56654=DIRECTION('ref_axis',(0.,-0.942844461217511,-0.333233134534159));
#56655=DIRECTION('center_axis',(0.,0.333233134534162,-0.94284446121751));
#56656=DIRECTION('ref_axis',(0.,0.94284446121751,0.333233134534162));
#56657=DIRECTION('center_axis',(0.,-0.333233134534159,0.942844461217511));
#56658=DIRECTION('ref_axis',(0.,-0.942844461217511,-0.333233134534159));
#56659=DIRECTION('center_axis',(0.,0.333233134534162,-0.94284446121751));
#56660=DIRECTION('ref_axis',(0.,0.94284446121751,0.333233134534162));
#56661=DIRECTION('center_axis',(0.,-0.333233134534159,0.942844461217511));
#56662=DIRECTION('ref_axis',(0.,-0.942844461217511,-0.333233134534159));
#56663=DIRECTION('center_axis',(0.,0.333233134534162,-0.94284446121751));
#56664=DIRECTION('ref_axis',(0.,0.94284446121751,0.333233134534162));
#56665=DIRECTION('center_axis',(0.,-0.333233134534159,0.942844461217511));
#56666=DIRECTION('ref_axis',(0.,-0.942844461217511,-0.333233134534159));
#56667=DIRECTION('center_axis',(0.,0.333233134534162,-0.94284446121751));
#56668=DIRECTION('ref_axis',(0.,0.94284446121751,0.333233134534162));
#56669=DIRECTION('center_axis',(0.,-0.333233134534159,0.942844461217511));
#56670=DIRECTION('ref_axis',(0.,-0.942844461217511,-0.333233134534159));
#56671=DIRECTION('center_axis',(0.,0.333233134534162,-0.94284446121751));
#56672=DIRECTION('ref_axis',(0.,0.94284446121751,0.333233134534162));
#56673=DIRECTION('center_axis',(0.,-0.333233134534159,0.942844461217511));
#56674=DIRECTION('ref_axis',(0.,-0.942844461217511,-0.333233134534159));
#56675=DIRECTION('center_axis',(0.,0.333233134534162,-0.94284446121751));
#56676=DIRECTION('ref_axis',(0.,0.94284446121751,0.333233134534162));
#56677=DIRECTION('center_axis',(0.,-0.333233134534159,0.942844461217511));
#56678=DIRECTION('ref_axis',(0.,-0.942844461217511,-0.333233134534159));
#56679=DIRECTION('center_axis',(0.,0.333233134534162,-0.94284446121751));
#56680=DIRECTION('ref_axis',(0.,0.94284446121751,0.333233134534162));
#56681=DIRECTION('center_axis',(0.,-0.333233134534159,0.942844461217511));
#56682=DIRECTION('ref_axis',(0.,-0.942844461217511,-0.333233134534159));
#56683=DIRECTION('center_axis',(0.,0.333233134534162,-0.94284446121751));
#56684=DIRECTION('ref_axis',(0.,0.94284446121751,0.333233134534162));
#56685=DIRECTION('center_axis',(0.,-0.333233134534159,0.942844461217511));
#56686=DIRECTION('ref_axis',(0.,-0.942844461217511,-0.333233134534159));
#56687=DIRECTION('center_axis',(0.,0.333233134534162,-0.94284446121751));
#56688=DIRECTION('ref_axis',(0.,0.94284446121751,0.333233134534162));
#56689=DIRECTION('center_axis',(0.,-0.333233134534159,0.942844461217511));
#56690=DIRECTION('ref_axis',(0.,-0.942844461217511,-0.333233134534159));
#56691=DIRECTION('center_axis',(0.,0.333233134534162,-0.94284446121751));
#56692=DIRECTION('ref_axis',(0.,0.94284446121751,0.333233134534162));
#56693=DIRECTION('center_axis',(0.,-0.333233134534159,0.942844461217511));
#56694=DIRECTION('ref_axis',(0.,-0.942844461217511,-0.333233134534159));
#56695=DIRECTION('center_axis',(0.,0.333233134534162,-0.94284446121751));
#56696=DIRECTION('ref_axis',(0.,0.94284446121751,0.333233134534162));
#56697=DIRECTION('center_axis',(0.,-0.333233134534159,0.942844461217511));
#56698=DIRECTION('ref_axis',(0.,-0.942844461217511,-0.333233134534159));
#56699=DIRECTION('center_axis',(0.,0.333233134534162,-0.94284446121751));
#56700=DIRECTION('ref_axis',(0.,0.94284446121751,0.333233134534162));
#56701=DIRECTION('center_axis',(0.,-0.333233134534159,0.942844461217511));
#56702=DIRECTION('ref_axis',(0.,-0.942844461217511,-0.333233134534159));
#56703=DIRECTION('center_axis',(0.,0.333233134534162,-0.94284446121751));
#56704=DIRECTION('ref_axis',(0.,0.94284446121751,0.333233134534162));
#56705=DIRECTION('center_axis',(0.,-0.333233134534159,0.942844461217511));
#56706=DIRECTION('ref_axis',(0.,-0.942844461217511,-0.333233134534159));
#56707=DIRECTION('center_axis',(0.,0.333233134534162,-0.94284446121751));
#56708=DIRECTION('ref_axis',(0.,0.94284446121751,0.333233134534162));
#56709=DIRECTION('center_axis',(0.,-0.333233134534159,0.942844461217511));
#56710=DIRECTION('ref_axis',(0.,-0.942844461217511,-0.333233134534159));
#56711=DIRECTION('center_axis',(0.,0.333233134534162,-0.94284446121751));
#56712=DIRECTION('ref_axis',(0.,0.94284446121751,0.333233134534162));
#56713=DIRECTION('center_axis',(0.,-0.333233134534159,0.942844461217511));
#56714=DIRECTION('ref_axis',(0.,-0.942844461217511,-0.333233134534159));
#56715=DIRECTION('center_axis',(0.,0.333233134534162,-0.94284446121751));
#56716=DIRECTION('ref_axis',(0.,0.94284446121751,0.333233134534162));
#56717=DIRECTION('center_axis',(0.,-0.333233134534159,0.942844461217511));
#56718=DIRECTION('ref_axis',(0.,-0.942844461217511,-0.333233134534159));
#56719=DIRECTION('center_axis',(0.,0.333233134534162,-0.94284446121751));
#56720=DIRECTION('ref_axis',(0.,0.94284446121751,0.333233134534162));
#56721=DIRECTION('center_axis',(0.,-0.333233134534159,0.942844461217511));
#56722=DIRECTION('ref_axis',(0.,-0.942844461217511,-0.333233134534159));
#56723=DIRECTION('center_axis',(0.,0.333233134534162,-0.94284446121751));
#56724=DIRECTION('ref_axis',(0.,0.94284446121751,0.333233134534162));
#56725=DIRECTION('center_axis',(0.,-0.333233134534159,0.942844461217511));
#56726=DIRECTION('ref_axis',(0.,-0.942844461217511,-0.333233134534159));
#56727=DIRECTION('center_axis',(0.,0.333233134534162,-0.94284446121751));
#56728=DIRECTION('ref_axis',(0.,0.94284446121751,0.333233134534162));
#56729=DIRECTION('center_axis',(0.,-0.333233134534159,0.942844461217511));
#56730=DIRECTION('ref_axis',(0.,-0.942844461217511,-0.333233134534159));
#56731=DIRECTION('center_axis',(0.,0.333233134534162,-0.94284446121751));
#56732=DIRECTION('ref_axis',(0.,0.94284446121751,0.333233134534162));
#56733=DIRECTION('center_axis',(0.,-0.333233134534159,0.942844461217511));
#56734=DIRECTION('ref_axis',(0.,-0.942844461217511,-0.333233134534159));
#56735=DIRECTION('center_axis',(0.,0.333233134534162,-0.94284446121751));
#56736=DIRECTION('ref_axis',(0.,0.94284446121751,0.333233134534162));
#56737=DIRECTION('center_axis',(0.,-0.333233134534159,0.942844461217511));
#56738=DIRECTION('ref_axis',(0.,-0.942844461217511,-0.333233134534159));
#56739=DIRECTION('center_axis',(0.,0.333233134534162,-0.94284446121751));
#56740=DIRECTION('ref_axis',(0.,0.94284446121751,0.333233134534162));
#56741=DIRECTION('center_axis',(0.,-0.333233134534159,0.942844461217511));
#56742=DIRECTION('ref_axis',(0.,-0.942844461217511,-0.333233134534159));
#56743=DIRECTION('center_axis',(0.,0.333233134534162,-0.94284446121751));
#56744=DIRECTION('ref_axis',(0.,0.94284446121751,0.333233134534162));
#56745=DIRECTION('center_axis',(0.,-0.333233134534159,0.942844461217511));
#56746=DIRECTION('ref_axis',(0.,-0.942844461217511,-0.333233134534159));
#56747=DIRECTION('center_axis',(0.,0.333233134534162,-0.94284446121751));
#56748=DIRECTION('ref_axis',(0.,0.94284446121751,0.333233134534162));
#56749=DIRECTION('center_axis',(0.,-0.333233134534159,0.942844461217511));
#56750=DIRECTION('ref_axis',(0.,-0.942844461217511,-0.333233134534159));
#56751=DIRECTION('center_axis',(0.,0.333233134534162,-0.94284446121751));
#56752=DIRECTION('ref_axis',(0.,0.94284446121751,0.333233134534162));
#56753=DIRECTION('center_axis',(0.,-0.333233134534159,0.942844461217511));
#56754=DIRECTION('ref_axis',(0.,-0.942844461217511,-0.333233134534159));
#56755=DIRECTION('center_axis',(0.,0.333233134534162,-0.94284446121751));
#56756=DIRECTION('ref_axis',(0.,0.94284446121751,0.333233134534162));
#56757=DIRECTION('center_axis',(0.,-0.333233134534159,0.942844461217511));
#56758=DIRECTION('ref_axis',(0.,-0.942844461217511,-0.333233134534159));
#56759=DIRECTION('center_axis',(0.,0.333233134534162,-0.94284446121751));
#56760=DIRECTION('ref_axis',(0.,0.94284446121751,0.333233134534162));
#56761=DIRECTION('center_axis',(0.,-0.333233134534159,0.942844461217511));
#56762=DIRECTION('ref_axis',(0.,-0.942844461217511,-0.333233134534159));
#56763=DIRECTION('center_axis',(0.,0.333233134534162,-0.94284446121751));
#56764=DIRECTION('ref_axis',(0.,0.94284446121751,0.333233134534162));
#56765=DIRECTION('center_axis',(0.,-0.333233134534159,0.942844461217511));
#56766=DIRECTION('ref_axis',(0.,-0.942844461217511,-0.333233134534159));
#56767=DIRECTION('center_axis',(0.,0.333233134534162,-0.94284446121751));
#56768=DIRECTION('ref_axis',(0.,0.94284446121751,0.333233134534162));
#56769=DIRECTION('center_axis',(0.,-0.333233134534159,0.942844461217511));
#56770=DIRECTION('ref_axis',(0.,-0.942844461217511,-0.333233134534159));
#56771=DIRECTION('center_axis',(0.,0.333233134534162,-0.94284446121751));
#56772=DIRECTION('ref_axis',(0.,0.94284446121751,0.333233134534162));
#56773=DIRECTION('center_axis',(0.,-0.333233134534159,0.942844461217511));
#56774=DIRECTION('ref_axis',(0.,-0.942844461217511,-0.333233134534159));
#56775=DIRECTION('center_axis',(0.,0.333233134534162,-0.94284446121751));
#56776=DIRECTION('ref_axis',(0.,0.94284446121751,0.333233134534162));
#56777=DIRECTION('center_axis',(0.,-0.333233134534159,0.942844461217511));
#56778=DIRECTION('ref_axis',(0.,-0.942844461217511,-0.333233134534159));
#56779=DIRECTION('center_axis',(0.,0.333233134534162,-0.94284446121751));
#56780=DIRECTION('ref_axis',(0.,0.94284446121751,0.333233134534162));
#56781=DIRECTION('center_axis',(0.,-0.333233134534159,0.942844461217511));
#56782=DIRECTION('ref_axis',(0.,-0.942844461217511,-0.333233134534159));
#56783=DIRECTION('center_axis',(0.,0.333233134534162,-0.94284446121751));
#56784=DIRECTION('ref_axis',(0.,0.94284446121751,0.333233134534162));
#56785=DIRECTION('center_axis',(0.,-0.333233134534159,0.942844461217511));
#56786=DIRECTION('ref_axis',(0.,-0.942844461217511,-0.333233134534159));
#56787=DIRECTION('center_axis',(0.,0.333233134534162,-0.94284446121751));
#56788=DIRECTION('ref_axis',(0.,0.94284446121751,0.333233134534162));
#56789=DIRECTION('center_axis',(0.,-0.333233134534159,0.942844461217511));
#56790=DIRECTION('ref_axis',(0.,-0.942844461217511,-0.333233134534159));
#56791=DIRECTION('center_axis',(0.,0.333233134534162,-0.94284446121751));
#56792=DIRECTION('ref_axis',(0.,0.94284446121751,0.333233134534162));
#56793=DIRECTION('center_axis',(0.,-0.333233134534159,0.942844461217511));
#56794=DIRECTION('ref_axis',(0.,-0.942844461217511,-0.333233134534159));
#56795=DIRECTION('center_axis',(0.,0.333233134534162,-0.94284446121751));
#56796=DIRECTION('ref_axis',(0.,0.94284446121751,0.333233134534162));
#56797=DIRECTION('center_axis',(0.,-0.333233134534159,0.942844461217511));
#56798=DIRECTION('ref_axis',(0.,-0.942844461217511,-0.333233134534159));
#56799=DIRECTION('center_axis',(0.,0.333233134534162,-0.94284446121751));
#56800=DIRECTION('ref_axis',(0.,0.94284446121751,0.333233134534162));
#56801=DIRECTION('center_axis',(0.,-0.333233134534159,0.942844461217511));
#56802=DIRECTION('ref_axis',(0.,-0.942844461217511,-0.333233134534159));
#56803=DIRECTION('center_axis',(0.,0.333233134534162,-0.94284446121751));
#56804=DIRECTION('ref_axis',(0.,0.94284446121751,0.333233134534162));
#56805=DIRECTION('center_axis',(0.,-0.333233134534159,0.942844461217511));
#56806=DIRECTION('ref_axis',(0.,-0.942844461217511,-0.333233134534159));
#56807=DIRECTION('center_axis',(0.,0.333233134534162,-0.94284446121751));
#56808=DIRECTION('ref_axis',(0.,0.94284446121751,0.333233134534162));
#56809=DIRECTION('center_axis',(0.,-0.333233134534159,0.942844461217511));
#56810=DIRECTION('ref_axis',(0.,-0.942844461217511,-0.333233134534159));
#56811=DIRECTION('center_axis',(0.,0.333233134534162,-0.94284446121751));
#56812=DIRECTION('ref_axis',(0.,0.94284446121751,0.333233134534162));
#56813=DIRECTION('center_axis',(0.,-0.333233134534159,0.942844461217511));
#56814=DIRECTION('ref_axis',(0.,-0.942844461217511,-0.333233134534159));
#56815=DIRECTION('center_axis',(0.,0.333233134534162,-0.94284446121751));
#56816=DIRECTION('ref_axis',(0.,0.94284446121751,0.333233134534162));
#56817=DIRECTION('center_axis',(0.,-0.333233134534159,0.942844461217511));
#56818=DIRECTION('ref_axis',(0.,-0.942844461217511,-0.333233134534159));
#56819=DIRECTION('center_axis',(0.,0.333233134534162,-0.94284446121751));
#56820=DIRECTION('ref_axis',(0.,0.94284446121751,0.333233134534162));
#56821=DIRECTION('center_axis',(0.,-0.333233134534159,0.942844461217511));
#56822=DIRECTION('ref_axis',(0.,-0.942844461217511,-0.333233134534159));
#56823=DIRECTION('center_axis',(0.,0.333233134534162,-0.94284446121751));
#56824=DIRECTION('ref_axis',(0.,0.94284446121751,0.333233134534162));
#56825=DIRECTION('center_axis',(0.,-0.333233134534159,0.942844461217511));
#56826=DIRECTION('ref_axis',(0.,-0.942844461217511,-0.333233134534159));
#56827=DIRECTION('center_axis',(0.,0.333233134534162,-0.94284446121751));
#56828=DIRECTION('ref_axis',(0.,0.94284446121751,0.333233134534162));
#56829=DIRECTION('center_axis',(0.,-0.333233134534159,0.942844461217511));
#56830=DIRECTION('ref_axis',(0.,-0.942844461217511,-0.333233134534159));
#56831=DIRECTION('center_axis',(0.,0.333233134534162,-0.94284446121751));
#56832=DIRECTION('ref_axis',(0.,0.94284446121751,0.333233134534162));
#56833=DIRECTION('center_axis',(0.,-0.333233134534159,0.942844461217511));
#56834=DIRECTION('ref_axis',(0.,-0.942844461217511,-0.333233134534159));
#56835=DIRECTION('center_axis',(0.,0.333233134534162,-0.94284446121751));
#56836=DIRECTION('ref_axis',(0.,0.94284446121751,0.333233134534162));
#56837=DIRECTION('center_axis',(0.,-0.333233134534159,0.942844461217511));
#56838=DIRECTION('ref_axis',(0.,-0.942844461217511,-0.333233134534159));
#56839=DIRECTION('center_axis',(0.,0.333233134534162,-0.94284446121751));
#56840=DIRECTION('ref_axis',(0.,0.94284446121751,0.333233134534162));
#56841=DIRECTION('center_axis',(0.,-0.333233134534159,0.942844461217511));
#56842=DIRECTION('ref_axis',(0.,-0.942844461217511,-0.333233134534159));
#56843=DIRECTION('center_axis',(0.,0.333233134534162,-0.94284446121751));
#56844=DIRECTION('ref_axis',(0.,0.94284446121751,0.333233134534162));
#56845=DIRECTION('center_axis',(0.,-0.333233134534159,0.942844461217511));
#56846=DIRECTION('ref_axis',(0.,-0.942844461217511,-0.333233134534159));
#56847=DIRECTION('center_axis',(0.,0.333233134534162,-0.94284446121751));
#56848=DIRECTION('ref_axis',(0.,0.94284446121751,0.333233134534162));
#56849=DIRECTION('center_axis',(0.,-0.333233134534159,0.942844461217511));
#56850=DIRECTION('ref_axis',(0.,-0.942844461217511,-0.333233134534159));
#56851=DIRECTION('center_axis',(0.,0.333233134534162,-0.94284446121751));
#56852=DIRECTION('ref_axis',(0.,0.94284446121751,0.333233134534162));
#56853=DIRECTION('center_axis',(0.,-0.333233134534159,0.942844461217511));
#56854=DIRECTION('ref_axis',(0.,-0.942844461217511,-0.333233134534159));
#56855=DIRECTION('center_axis',(0.,0.333233134534162,-0.94284446121751));
#56856=DIRECTION('ref_axis',(0.,0.94284446121751,0.333233134534162));
#56857=DIRECTION('center_axis',(0.,-0.333233134534159,0.942844461217511));
#56858=DIRECTION('ref_axis',(0.,-0.942844461217511,-0.333233134534159));
#56859=DIRECTION('center_axis',(0.,0.333233134534162,-0.94284446121751));
#56860=DIRECTION('ref_axis',(0.,0.94284446121751,0.333233134534162));
#56861=DIRECTION('center_axis',(0.,-0.333233134534159,0.942844461217511));
#56862=DIRECTION('ref_axis',(0.,-0.942844461217511,-0.333233134534159));
#56863=DIRECTION('center_axis',(0.,0.333233134534162,-0.94284446121751));
#56864=DIRECTION('ref_axis',(0.,0.94284446121751,0.333233134534162));
#56865=DIRECTION('center_axis',(0.,-0.333233134534159,0.942844461217511));
#56866=DIRECTION('ref_axis',(0.,-0.942844461217511,-0.333233134534159));
#56867=DIRECTION('center_axis',(0.,0.333233134534162,-0.94284446121751));
#56868=DIRECTION('ref_axis',(0.,0.94284446121751,0.333233134534162));
#56869=DIRECTION('center_axis',(0.,-0.333233134534159,0.942844461217511));
#56870=DIRECTION('ref_axis',(0.,-0.942844461217511,-0.333233134534159));
#56871=DIRECTION('center_axis',(0.,0.333233134534162,-0.94284446121751));
#56872=DIRECTION('ref_axis',(0.,0.94284446121751,0.333233134534162));
#56873=DIRECTION('center_axis',(0.,-0.333233134534159,0.942844461217511));
#56874=DIRECTION('ref_axis',(0.,-0.942844461217511,-0.333233134534159));
#56875=DIRECTION('center_axis',(0.,0.333233134534162,-0.94284446121751));
#56876=DIRECTION('ref_axis',(0.,0.94284446121751,0.333233134534162));
#56877=DIRECTION('center_axis',(0.,-0.333233134534159,0.942844461217511));
#56878=DIRECTION('ref_axis',(0.,-0.942844461217511,-0.333233134534159));
#56879=DIRECTION('center_axis',(0.,0.333233134534162,-0.94284446121751));
#56880=DIRECTION('ref_axis',(0.,0.94284446121751,0.333233134534162));
#56881=DIRECTION('center_axis',(0.,-0.333233134534159,0.942844461217511));
#56882=DIRECTION('ref_axis',(0.,-0.942844461217511,-0.333233134534159));
#56883=DIRECTION('center_axis',(0.,0.333233134534162,-0.94284446121751));
#56884=DIRECTION('ref_axis',(0.,0.94284446121751,0.333233134534162));
#56885=DIRECTION('center_axis',(0.,-0.333233134534159,0.942844461217511));
#56886=DIRECTION('ref_axis',(0.,-0.942844461217511,-0.333233134534159));
#56887=DIRECTION('center_axis',(0.,0.333233134534162,-0.94284446121751));
#56888=DIRECTION('ref_axis',(0.,0.94284446121751,0.333233134534162));
#56889=DIRECTION('center_axis',(0.,-0.333233134534159,0.942844461217511));
#56890=DIRECTION('ref_axis',(0.,-0.942844461217511,-0.333233134534159));
#56891=DIRECTION('center_axis',(0.,0.333233134534162,-0.94284446121751));
#56892=DIRECTION('ref_axis',(0.,0.94284446121751,0.333233134534162));
#56893=DIRECTION('center_axis',(0.,-0.333233134534159,0.942844461217511));
#56894=DIRECTION('ref_axis',(0.,-0.942844461217511,-0.333233134534159));
#56895=DIRECTION('center_axis',(0.,0.333233134534162,-0.94284446121751));
#56896=DIRECTION('ref_axis',(0.,0.94284446121751,0.333233134534162));
#56897=DIRECTION('center_axis',(0.,-0.333233134534159,0.942844461217511));
#56898=DIRECTION('ref_axis',(0.,-0.942844461217511,-0.333233134534159));
#56899=DIRECTION('center_axis',(0.,0.333233134534162,-0.94284446121751));
#56900=DIRECTION('ref_axis',(0.,0.94284446121751,0.333233134534162));
#56901=DIRECTION('center_axis',(0.,-0.333233134534159,0.942844461217511));
#56902=DIRECTION('ref_axis',(0.,-0.942844461217511,-0.333233134534159));
#56903=DIRECTION('center_axis',(0.,0.333233134534162,-0.94284446121751));
#56904=DIRECTION('ref_axis',(0.,0.94284446121751,0.333233134534162));
#56905=DIRECTION('center_axis',(0.,-0.333233134534159,0.942844461217511));
#56906=DIRECTION('ref_axis',(0.,-0.942844461217511,-0.333233134534159));
#56907=DIRECTION('center_axis',(0.,0.333233134534162,-0.94284446121751));
#56908=DIRECTION('ref_axis',(0.,0.94284446121751,0.333233134534162));
#56909=DIRECTION('center_axis',(0.,-0.333233134534159,0.942844461217511));
#56910=DIRECTION('ref_axis',(0.,-0.942844461217511,-0.333233134534159));
#56911=DIRECTION('center_axis',(0.,0.333233134534162,-0.94284446121751));
#56912=DIRECTION('ref_axis',(0.,0.94284446121751,0.333233134534162));
#56913=DIRECTION('center_axis',(0.,-0.333233134534159,0.942844461217511));
#56914=DIRECTION('ref_axis',(0.,-0.942844461217511,-0.333233134534159));
#56915=DIRECTION('center_axis',(0.,0.333233134534162,-0.94284446121751));
#56916=DIRECTION('ref_axis',(0.,0.94284446121751,0.333233134534162));
#56917=DIRECTION('center_axis',(0.,-0.333233134534159,0.942844461217511));
#56918=DIRECTION('ref_axis',(0.,-0.942844461217511,-0.333233134534159));
#56919=DIRECTION('center_axis',(0.,0.333233134534162,-0.94284446121751));
#56920=DIRECTION('ref_axis',(0.,0.94284446121751,0.333233134534162));
#56921=DIRECTION('center_axis',(0.,-0.333233134534159,0.942844461217511));
#56922=DIRECTION('ref_axis',(0.,-0.942844461217511,-0.333233134534159));
#56923=DIRECTION('center_axis',(0.,0.333233134534162,-0.94284446121751));
#56924=DIRECTION('ref_axis',(0.,0.94284446121751,0.333233134534162));
#56925=DIRECTION('center_axis',(0.,-0.333233134534159,0.942844461217511));
#56926=DIRECTION('ref_axis',(0.,-0.942844461217511,-0.333233134534159));
#56927=DIRECTION('center_axis',(0.,0.333233134534162,-0.94284446121751));
#56928=DIRECTION('ref_axis',(0.,0.94284446121751,0.333233134534162));
#56929=DIRECTION('center_axis',(0.,-0.333233134534159,0.942844461217511));
#56930=DIRECTION('ref_axis',(0.,-0.942844461217511,-0.333233134534159));
#56931=DIRECTION('center_axis',(0.,0.333233134534162,-0.94284446121751));
#56932=DIRECTION('ref_axis',(0.,0.94284446121751,0.333233134534162));
#56933=DIRECTION('center_axis',(0.,-0.333233134534159,0.942844461217511));
#56934=DIRECTION('ref_axis',(0.,-0.942844461217511,-0.333233134534159));
#56935=DIRECTION('center_axis',(0.,0.333233134534162,-0.94284446121751));
#56936=DIRECTION('ref_axis',(0.,0.94284446121751,0.333233134534162));
#56937=DIRECTION('center_axis',(0.,-0.333233134534159,0.942844461217511));
#56938=DIRECTION('ref_axis',(0.,-0.942844461217511,-0.333233134534159));
#56939=DIRECTION('center_axis',(0.,0.333233134534162,-0.94284446121751));
#56940=DIRECTION('ref_axis',(0.,0.94284446121751,0.333233134534162));
#56941=DIRECTION('center_axis',(0.,-0.333233134534159,0.942844461217511));
#56942=DIRECTION('ref_axis',(0.,-0.942844461217511,-0.333233134534159));
#56943=DIRECTION('center_axis',(0.,0.333233134534162,-0.94284446121751));
#56944=DIRECTION('ref_axis',(0.,0.94284446121751,0.333233134534162));
#56945=DIRECTION('center_axis',(0.,-0.333233134534159,0.942844461217511));
#56946=DIRECTION('ref_axis',(0.,-0.942844461217511,-0.333233134534159));
#56947=DIRECTION('center_axis',(0.,0.333233134534162,-0.94284446121751));
#56948=DIRECTION('ref_axis',(0.,0.94284446121751,0.333233134534162));
#56949=DIRECTION('center_axis',(0.,-0.333233134534159,0.942844461217511));
#56950=DIRECTION('ref_axis',(0.,-0.942844461217511,-0.333233134534159));
#56951=DIRECTION('center_axis',(0.,0.333233134534162,-0.94284446121751));
#56952=DIRECTION('ref_axis',(0.,0.94284446121751,0.333233134534162));
#56953=DIRECTION('center_axis',(0.,-0.333233134534159,0.942844461217511));
#56954=DIRECTION('ref_axis',(0.,-0.942844461217511,-0.333233134534159));
#56955=DIRECTION('center_axis',(0.,0.333233134534162,-0.94284446121751));
#56956=DIRECTION('ref_axis',(0.,0.94284446121751,0.333233134534162));
#56957=DIRECTION('center_axis',(0.,-0.333233134534159,0.942844461217511));
#56958=DIRECTION('ref_axis',(0.,-0.942844461217511,-0.333233134534159));
#56959=DIRECTION('center_axis',(0.,0.333233134534162,-0.94284446121751));
#56960=DIRECTION('ref_axis',(0.,0.94284446121751,0.333233134534162));
#56961=DIRECTION('center_axis',(0.,-0.333233134534159,0.942844461217511));
#56962=DIRECTION('ref_axis',(0.,-0.942844461217511,-0.333233134534159));
#56963=DIRECTION('center_axis',(0.,0.333233134534162,-0.94284446121751));
#56964=DIRECTION('ref_axis',(0.,0.94284446121751,0.333233134534162));
#56965=DIRECTION('center_axis',(0.,-0.333233134534159,0.942844461217511));
#56966=DIRECTION('ref_axis',(0.,-0.942844461217511,-0.333233134534159));
#56967=DIRECTION('center_axis',(0.,0.333233134534162,-0.94284446121751));
#56968=DIRECTION('ref_axis',(0.,0.94284446121751,0.333233134534162));
#56969=DIRECTION('center_axis',(0.,-0.333233134534159,0.942844461217511));
#56970=DIRECTION('ref_axis',(0.,-0.942844461217511,-0.333233134534159));
#56971=DIRECTION('center_axis',(0.,0.333233134534162,-0.94284446121751));
#56972=DIRECTION('ref_axis',(0.,0.94284446121751,0.333233134534162));
#56973=DIRECTION('center_axis',(0.,-0.333233134534159,0.942844461217511));
#56974=DIRECTION('ref_axis',(0.,-0.942844461217511,-0.333233134534159));
#56975=DIRECTION('center_axis',(0.,0.333233134534162,-0.94284446121751));
#56976=DIRECTION('ref_axis',(0.,0.94284446121751,0.333233134534162));
#56977=DIRECTION('center_axis',(0.,-0.333233134534159,0.942844461217511));
#56978=DIRECTION('ref_axis',(0.,-0.942844461217511,-0.333233134534159));
#56979=DIRECTION('center_axis',(0.,0.333233134534162,-0.94284446121751));
#56980=DIRECTION('ref_axis',(0.,0.94284446121751,0.333233134534162));
#56981=DIRECTION('center_axis',(0.,-0.333233134534159,0.942844461217511));
#56982=DIRECTION('ref_axis',(0.,-0.942844461217511,-0.333233134534159));
#56983=DIRECTION('center_axis',(0.,0.333233134534162,-0.94284446121751));
#56984=DIRECTION('ref_axis',(0.,0.94284446121751,0.333233134534162));
#56985=DIRECTION('center_axis',(0.,-0.333233134534159,0.942844461217511));
#56986=DIRECTION('ref_axis',(0.,-0.942844461217511,-0.333233134534159));
#56987=DIRECTION('center_axis',(0.,0.333233134534162,-0.94284446121751));
#56988=DIRECTION('ref_axis',(0.,0.94284446121751,0.333233134534162));
#56989=DIRECTION('center_axis',(0.,-0.333233134534159,0.942844461217511));
#56990=DIRECTION('ref_axis',(0.,-0.942844461217511,-0.333233134534159));
#56991=DIRECTION('center_axis',(0.,0.333233134534162,-0.94284446121751));
#56992=DIRECTION('ref_axis',(0.,0.94284446121751,0.333233134534162));
#56993=DIRECTION('center_axis',(0.,-0.333233134534159,0.942844461217511));
#56994=DIRECTION('ref_axis',(0.,-0.942844461217511,-0.333233134534159));
#56995=DIRECTION('center_axis',(0.,0.333233134534162,-0.94284446121751));
#56996=DIRECTION('ref_axis',(0.,0.94284446121751,0.333233134534162));
#56997=DIRECTION('center_axis',(0.,-0.333233134534159,0.942844461217511));
#56998=DIRECTION('ref_axis',(0.,-0.942844461217511,-0.333233134534159));
#56999=DIRECTION('center_axis',(0.,0.333233134534162,-0.94284446121751));
#57000=DIRECTION('ref_axis',(0.,0.94284446121751,0.333233134534162));
#57001=DIRECTION('center_axis',(0.,-0.333233134534159,0.942844461217511));
#57002=DIRECTION('ref_axis',(0.,-0.942844461217511,-0.333233134534159));
#57003=DIRECTION('center_axis',(0.,0.333233134534162,-0.94284446121751));
#57004=DIRECTION('ref_axis',(0.,0.94284446121751,0.333233134534162));
#57005=DIRECTION('center_axis',(0.,-0.333233134534159,0.942844461217511));
#57006=DIRECTION('ref_axis',(0.,-0.942844461217511,-0.333233134534159));
#57007=DIRECTION('center_axis',(0.,0.333233134534162,-0.94284446121751));
#57008=DIRECTION('ref_axis',(0.,0.94284446121751,0.333233134534162));
#57009=DIRECTION('center_axis',(0.,-0.333233134534159,0.942844461217511));
#57010=DIRECTION('ref_axis',(0.,-0.942844461217511,-0.333233134534159));
#57011=DIRECTION('center_axis',(0.,0.333233134534162,-0.94284446121751));
#57012=DIRECTION('ref_axis',(0.,0.94284446121751,0.333233134534162));
#57013=DIRECTION('center_axis',(0.,-0.333233134534159,0.942844461217511));
#57014=DIRECTION('ref_axis',(0.,-0.942844461217511,-0.333233134534159));
#57015=DIRECTION('center_axis',(0.,0.333233134534162,-0.94284446121751));
#57016=DIRECTION('ref_axis',(0.,0.94284446121751,0.333233134534162));
#57017=DIRECTION('center_axis',(0.,-0.333233134534159,0.942844461217511));
#57018=DIRECTION('ref_axis',(0.,-0.942844461217511,-0.333233134534159));
#57019=DIRECTION('center_axis',(0.,0.333233134534162,-0.94284446121751));
#57020=DIRECTION('ref_axis',(0.,0.94284446121751,0.333233134534162));
#57021=DIRECTION('center_axis',(0.,-0.333233134534159,0.942844461217511));
#57022=DIRECTION('ref_axis',(0.,-0.942844461217511,-0.333233134534159));
#57023=DIRECTION('center_axis',(0.,0.333233134534162,-0.94284446121751));
#57024=DIRECTION('ref_axis',(0.,0.94284446121751,0.333233134534162));
#57025=DIRECTION('center_axis',(0.,-0.333233134534159,0.942844461217511));
#57026=DIRECTION('ref_axis',(0.,-0.942844461217511,-0.333233134534159));
#57027=DIRECTION('center_axis',(0.,0.333233134534162,-0.94284446121751));
#57028=DIRECTION('ref_axis',(0.,0.94284446121751,0.333233134534162));
#57029=DIRECTION('center_axis',(0.,-0.333233134534159,0.942844461217511));
#57030=DIRECTION('ref_axis',(0.,-0.942844461217511,-0.333233134534159));
#57031=DIRECTION('center_axis',(0.,0.333233134534162,-0.94284446121751));
#57032=DIRECTION('ref_axis',(0.,0.94284446121751,0.333233134534162));
#57033=DIRECTION('center_axis',(0.,-0.333233134534159,0.942844461217511));
#57034=DIRECTION('ref_axis',(0.,-0.942844461217511,-0.333233134534159));
#57035=DIRECTION('center_axis',(0.,0.333233134534162,-0.94284446121751));
#57036=DIRECTION('ref_axis',(0.,0.94284446121751,0.333233134534162));
#57037=DIRECTION('center_axis',(0.,-0.333233134534159,0.942844461217511));
#57038=DIRECTION('ref_axis',(0.,-0.942844461217511,-0.333233134534159));
#57039=DIRECTION('center_axis',(0.,0.333233134534162,-0.94284446121751));
#57040=DIRECTION('ref_axis',(0.,0.94284446121751,0.333233134534162));
#57041=DIRECTION('center_axis',(0.,-0.333233134534159,0.942844461217511));
#57042=DIRECTION('ref_axis',(0.,-0.942844461217511,-0.333233134534159));
#57043=DIRECTION('center_axis',(0.,0.333233134534162,-0.94284446121751));
#57044=DIRECTION('ref_axis',(0.,0.94284446121751,0.333233134534162));
#57045=DIRECTION('center_axis',(0.,-0.333233134534159,0.942844461217511));
#57046=DIRECTION('ref_axis',(0.,-0.942844461217511,-0.333233134534159));
#57047=DIRECTION('center_axis',(0.,0.333233134534162,-0.94284446121751));
#57048=DIRECTION('ref_axis',(0.,0.94284446121751,0.333233134534162));
#57049=DIRECTION('center_axis',(0.,-0.333233134534159,0.942844461217511));
#57050=DIRECTION('ref_axis',(0.,-0.942844461217511,-0.333233134534159));
#57051=DIRECTION('center_axis',(0.,0.333233134534162,-0.94284446121751));
#57052=DIRECTION('ref_axis',(0.,0.94284446121751,0.333233134534162));
#57053=DIRECTION('center_axis',(0.,-0.333233134534159,0.942844461217511));
#57054=DIRECTION('ref_axis',(0.,-0.942844461217511,-0.333233134534159));
#57055=DIRECTION('center_axis',(0.,0.333233134534162,-0.94284446121751));
#57056=DIRECTION('ref_axis',(0.,0.94284446121751,0.333233134534162));
#57057=DIRECTION('center_axis',(0.,-0.333233134534159,0.942844461217511));
#57058=DIRECTION('ref_axis',(0.,-0.942844461217511,-0.333233134534159));
#57059=DIRECTION('center_axis',(0.,0.333233134534162,-0.94284446121751));
#57060=DIRECTION('ref_axis',(0.,0.94284446121751,0.333233134534162));
#57061=DIRECTION('center_axis',(0.,-0.333233134534159,0.942844461217511));
#57062=DIRECTION('ref_axis',(0.,-0.942844461217511,-0.333233134534159));
#57063=DIRECTION('center_axis',(0.,0.333233134534162,-0.94284446121751));
#57064=DIRECTION('ref_axis',(0.,0.94284446121751,0.333233134534162));
#57065=DIRECTION('center_axis',(0.,-0.333233134534159,0.942844461217511));
#57066=DIRECTION('ref_axis',(0.,-0.942844461217511,-0.333233134534159));
#57067=DIRECTION('center_axis',(0.,0.333233134534162,-0.94284446121751));
#57068=DIRECTION('ref_axis',(0.,0.94284446121751,0.333233134534162));
#57069=DIRECTION('center_axis',(0.,-0.333233134534159,0.942844461217511));
#57070=DIRECTION('ref_axis',(0.,-0.942844461217511,-0.333233134534159));
#57071=DIRECTION('center_axis',(0.,0.333233134534162,-0.94284446121751));
#57072=DIRECTION('ref_axis',(0.,0.94284446121751,0.333233134534162));
#57073=DIRECTION('center_axis',(0.,-0.333233134534159,0.942844461217511));
#57074=DIRECTION('ref_axis',(0.,-0.942844461217511,-0.333233134534159));
#57075=DIRECTION('center_axis',(0.,0.333233134534162,-0.94284446121751));
#57076=DIRECTION('ref_axis',(0.,0.94284446121751,0.333233134534162));
#57077=DIRECTION('center_axis',(0.,-0.333233134534159,0.942844461217511));
#57078=DIRECTION('ref_axis',(0.,-0.942844461217511,-0.333233134534159));
#57079=DIRECTION('center_axis',(0.,0.333233134534162,-0.94284446121751));
#57080=DIRECTION('ref_axis',(0.,0.94284446121751,0.333233134534162));
#57081=DIRECTION('center_axis',(0.,-0.333233134534159,0.942844461217511));
#57082=DIRECTION('ref_axis',(0.,-0.942844461217511,-0.333233134534159));
#57083=DIRECTION('center_axis',(0.,0.333233134534162,-0.94284446121751));
#57084=DIRECTION('ref_axis',(0.,0.94284446121751,0.333233134534162));
#57085=DIRECTION('center_axis',(0.,-0.333233134534159,0.942844461217511));
#57086=DIRECTION('ref_axis',(0.,-0.942844461217511,-0.333233134534159));
#57087=DIRECTION('center_axis',(0.,0.333233134534162,-0.94284446121751));
#57088=DIRECTION('ref_axis',(0.,0.94284446121751,0.333233134534162));
#57089=DIRECTION('center_axis',(0.,-0.333233134534159,0.942844461217511));
#57090=DIRECTION('ref_axis',(0.,-0.942844461217511,-0.333233134534159));
#57091=DIRECTION('center_axis',(0.,0.333233134534162,-0.94284446121751));
#57092=DIRECTION('ref_axis',(0.,0.94284446121751,0.333233134534162));
#57093=DIRECTION('center_axis',(0.,-0.333233134534159,0.942844461217511));
#57094=DIRECTION('ref_axis',(0.,-0.942844461217511,-0.333233134534159));
#57095=DIRECTION('center_axis',(0.,0.333233134534162,-0.94284446121751));
#57096=DIRECTION('ref_axis',(0.,0.94284446121751,0.333233134534162));
#57097=DIRECTION('center_axis',(0.,-0.333233134534159,0.942844461217511));
#57098=DIRECTION('ref_axis',(0.,-0.942844461217511,-0.333233134534159));
#57099=DIRECTION('center_axis',(0.,0.333233134534162,-0.94284446121751));
#57100=DIRECTION('ref_axis',(0.,0.94284446121751,0.333233134534162));
#57101=DIRECTION('center_axis',(0.,-0.333233134534159,0.942844461217511));
#57102=DIRECTION('ref_axis',(0.,-0.942844461217511,-0.333233134534159));
#57103=DIRECTION('center_axis',(0.,0.333233134534162,-0.94284446121751));
#57104=DIRECTION('ref_axis',(0.,0.94284446121751,0.333233134534162));
#57105=DIRECTION('center_axis',(0.,-0.333233134534159,0.942844461217511));
#57106=DIRECTION('ref_axis',(0.,-0.942844461217511,-0.333233134534159));
#57107=DIRECTION('center_axis',(0.,0.333233134534162,-0.94284446121751));
#57108=DIRECTION('ref_axis',(0.,0.94284446121751,0.333233134534162));
#57109=DIRECTION('center_axis',(0.,-0.333233134534159,0.942844461217511));
#57110=DIRECTION('ref_axis',(0.,-0.942844461217511,-0.333233134534159));
#57111=DIRECTION('center_axis',(0.,0.333233134534162,-0.94284446121751));
#57112=DIRECTION('ref_axis',(0.,0.94284446121751,0.333233134534162));
#57113=DIRECTION('center_axis',(0.,-0.333233134534159,0.942844461217511));
#57114=DIRECTION('ref_axis',(0.,-0.942844461217511,-0.333233134534159));
#57115=DIRECTION('center_axis',(0.,0.333233134534162,-0.94284446121751));
#57116=DIRECTION('ref_axis',(0.,0.94284446121751,0.333233134534162));
#57117=DIRECTION('center_axis',(0.,-0.333233134534159,0.942844461217511));
#57118=DIRECTION('ref_axis',(0.,-0.942844461217511,-0.333233134534159));
#57119=DIRECTION('center_axis',(0.,0.333233134534162,-0.94284446121751));
#57120=DIRECTION('ref_axis',(0.,0.94284446121751,0.333233134534162));
#57121=DIRECTION('center_axis',(0.,-0.333233134534159,0.942844461217511));
#57122=DIRECTION('ref_axis',(0.,-0.942844461217511,-0.333233134534159));
#57123=DIRECTION('center_axis',(0.,0.333233134534162,-0.94284446121751));
#57124=DIRECTION('ref_axis',(0.,0.94284446121751,0.333233134534162));
#57125=DIRECTION('center_axis',(0.,-0.333233134534159,0.942844461217511));
#57126=DIRECTION('ref_axis',(0.,-0.942844461217511,-0.333233134534159));
#57127=DIRECTION('center_axis',(0.,0.333233134534162,-0.94284446121751));
#57128=DIRECTION('ref_axis',(0.,0.94284446121751,0.333233134534162));
#57129=DIRECTION('center_axis',(0.,-0.333233134534159,0.942844461217511));
#57130=DIRECTION('ref_axis',(0.,-0.942844461217511,-0.333233134534159));
#57131=DIRECTION('center_axis',(0.,0.333233134534162,-0.94284446121751));
#57132=DIRECTION('ref_axis',(0.,0.94284446121751,0.333233134534162));
#57133=DIRECTION('center_axis',(0.,-0.333233134534159,0.942844461217511));
#57134=DIRECTION('ref_axis',(0.,-0.942844461217511,-0.333233134534159));
#57135=DIRECTION('center_axis',(0.,0.333233134534162,-0.94284446121751));
#57136=DIRECTION('ref_axis',(0.,0.94284446121751,0.333233134534162));
#57137=DIRECTION('center_axis',(0.,-0.333233134534159,0.942844461217511));
#57138=DIRECTION('ref_axis',(0.,-0.942844461217511,-0.333233134534159));
#57139=DIRECTION('center_axis',(0.,0.333233134534162,-0.94284446121751));
#57140=DIRECTION('ref_axis',(0.,0.94284446121751,0.333233134534162));
#57141=DIRECTION('center_axis',(0.,-0.333233134534159,0.942844461217511));
#57142=DIRECTION('ref_axis',(0.,-0.942844461217511,-0.333233134534159));
#57143=DIRECTION('center_axis',(0.,0.333233134534162,-0.94284446121751));
#57144=DIRECTION('ref_axis',(0.,0.94284446121751,0.333233134534162));
#57145=DIRECTION('center_axis',(0.,-0.333233134534159,0.942844461217511));
#57146=DIRECTION('ref_axis',(0.,-0.942844461217511,-0.333233134534159));
#57147=DIRECTION('center_axis',(0.,0.333233134534162,-0.94284446121751));
#57148=DIRECTION('ref_axis',(0.,0.94284446121751,0.333233134534162));
#57149=DIRECTION('center_axis',(0.,-0.333233134534159,0.942844461217511));
#57150=DIRECTION('ref_axis',(0.,-0.942844461217511,-0.333233134534159));
#57151=DIRECTION('center_axis',(0.,0.333233134534162,-0.94284446121751));
#57152=DIRECTION('ref_axis',(0.,0.94284446121751,0.333233134534162));
#57153=DIRECTION('center_axis',(0.,-0.333233134534159,0.942844461217511));
#57154=DIRECTION('ref_axis',(0.,-0.942844461217511,-0.333233134534159));
#57155=DIRECTION('center_axis',(0.,0.333233134534162,-0.94284446121751));
#57156=DIRECTION('ref_axis',(0.,0.94284446121751,0.333233134534162));
#57157=DIRECTION('center_axis',(0.,-0.333233134534159,0.942844461217511));
#57158=DIRECTION('ref_axis',(0.,-0.942844461217511,-0.333233134534159));
#57159=DIRECTION('center_axis',(0.,0.333233134534162,-0.94284446121751));
#57160=DIRECTION('ref_axis',(0.,0.94284446121751,0.333233134534162));
#57161=DIRECTION('center_axis',(0.,-0.333233134534159,0.942844461217511));
#57162=DIRECTION('ref_axis',(0.,-0.942844461217511,-0.333233134534159));
#57163=DIRECTION('center_axis',(0.,0.333233134534162,-0.94284446121751));
#57164=DIRECTION('ref_axis',(0.,0.94284446121751,0.333233134534162));
#57165=DIRECTION('center_axis',(0.,-0.333233134534159,0.942844461217511));
#57166=DIRECTION('ref_axis',(0.,-0.942844461217511,-0.333233134534159));
#57167=DIRECTION('center_axis',(0.,0.333233134534162,-0.94284446121751));
#57168=DIRECTION('ref_axis',(0.,0.94284446121751,0.333233134534162));
#57169=DIRECTION('center_axis',(0.,-0.333233134534159,0.942844461217511));
#57170=DIRECTION('ref_axis',(0.,-0.942844461217511,-0.333233134534159));
#57171=DIRECTION('center_axis',(0.,0.333233134534162,-0.94284446121751));
#57172=DIRECTION('ref_axis',(0.,0.94284446121751,0.333233134534162));
#57173=DIRECTION('center_axis',(0.,-0.333233134534159,0.942844461217511));
#57174=DIRECTION('ref_axis',(0.,-0.942844461217511,-0.333233134534159));
#57175=DIRECTION('center_axis',(0.,0.333233134534162,-0.94284446121751));
#57176=DIRECTION('ref_axis',(0.,0.94284446121751,0.333233134534162));
#57177=DIRECTION('center_axis',(0.,-0.333233134534159,0.942844461217511));
#57178=DIRECTION('ref_axis',(0.,-0.942844461217511,-0.333233134534159));
#57179=DIRECTION('center_axis',(0.,0.333233134534162,-0.94284446121751));
#57180=DIRECTION('ref_axis',(0.,0.94284446121751,0.333233134534162));
#57181=DIRECTION('center_axis',(0.,-0.333233134534159,0.942844461217511));
#57182=DIRECTION('ref_axis',(0.,-0.942844461217511,-0.333233134534159));
#57183=DIRECTION('center_axis',(0.,0.333233134534162,-0.94284446121751));
#57184=DIRECTION('ref_axis',(0.,0.94284446121751,0.333233134534162));
#57185=DIRECTION('center_axis',(0.,-0.333233134534159,0.942844461217511));
#57186=DIRECTION('ref_axis',(0.,-0.942844461217511,-0.333233134534159));
#57187=DIRECTION('center_axis',(0.,0.333233134534162,-0.94284446121751));
#57188=DIRECTION('ref_axis',(0.,0.94284446121751,0.333233134534162));
#57189=DIRECTION('center_axis',(0.,-0.333233134534159,0.942844461217511));
#57190=DIRECTION('ref_axis',(0.,-0.942844461217511,-0.333233134534159));
#57191=DIRECTION('center_axis',(0.,0.333233134534162,-0.94284446121751));
#57192=DIRECTION('ref_axis',(0.,0.94284446121751,0.333233134534162));
#57193=DIRECTION('center_axis',(0.,-0.333233134534159,0.942844461217511));
#57194=DIRECTION('ref_axis',(0.,-0.942844461217511,-0.333233134534159));
#57195=DIRECTION('center_axis',(0.,0.333233134534162,-0.94284446121751));
#57196=DIRECTION('ref_axis',(0.,0.94284446121751,0.333233134534162));
#57197=DIRECTION('center_axis',(0.,-0.333233134534159,0.942844461217511));
#57198=DIRECTION('ref_axis',(0.,-0.942844461217511,-0.333233134534159));
#57199=DIRECTION('center_axis',(0.,0.333233134534162,-0.94284446121751));
#57200=DIRECTION('ref_axis',(0.,0.94284446121751,0.333233134534162));
#57201=DIRECTION('center_axis',(0.,-0.333233134534159,0.942844461217511));
#57202=DIRECTION('ref_axis',(0.,-0.942844461217511,-0.333233134534159));
#57203=DIRECTION('center_axis',(0.,0.333233134534162,-0.94284446121751));
#57204=DIRECTION('ref_axis',(0.,0.94284446121751,0.333233134534162));
#57205=DIRECTION('center_axis',(0.,-0.333233134534159,0.942844461217511));
#57206=DIRECTION('ref_axis',(0.,-0.942844461217511,-0.333233134534159));
#57207=DIRECTION('center_axis',(0.,0.333233134534162,-0.94284446121751));
#57208=DIRECTION('ref_axis',(0.,0.94284446121751,0.333233134534162));
#57209=DIRECTION('center_axis',(0.,-0.333233134534159,0.942844461217511));
#57210=DIRECTION('ref_axis',(0.,-0.942844461217511,-0.333233134534159));
#57211=DIRECTION('center_axis',(0.,0.333233134534162,-0.94284446121751));
#57212=DIRECTION('ref_axis',(0.,0.94284446121751,0.333233134534162));
#57213=DIRECTION('center_axis',(0.,-0.333233134534159,0.942844461217511));
#57214=DIRECTION('ref_axis',(0.,-0.942844461217511,-0.333233134534159));
#57215=DIRECTION('center_axis',(0.,0.333233134534162,-0.94284446121751));
#57216=DIRECTION('ref_axis',(0.,0.94284446121751,0.333233134534162));
#57217=DIRECTION('center_axis',(0.,-0.333233134534159,0.942844461217511));
#57218=DIRECTION('ref_axis',(0.,-0.942844461217511,-0.333233134534159));
#57219=DIRECTION('center_axis',(0.,0.333233134534162,-0.94284446121751));
#57220=DIRECTION('ref_axis',(0.,0.94284446121751,0.333233134534162));
#57221=DIRECTION('center_axis',(0.,-0.333233134534159,0.942844461217511));
#57222=DIRECTION('ref_axis',(0.,-0.942844461217511,-0.333233134534159));
#57223=DIRECTION('center_axis',(0.,0.333233134534162,-0.94284446121751));
#57224=DIRECTION('ref_axis',(0.,0.94284446121751,0.333233134534162));
#57225=DIRECTION('center_axis',(0.,-0.333233134534159,0.942844461217511));
#57226=DIRECTION('ref_axis',(0.,-0.942844461217511,-0.333233134534159));
#57227=DIRECTION('center_axis',(0.,0.333233134534162,-0.94284446121751));
#57228=DIRECTION('ref_axis',(0.,0.94284446121751,0.333233134534162));
#57229=DIRECTION('center_axis',(0.,-0.333233134534159,0.942844461217511));
#57230=DIRECTION('ref_axis',(0.,-0.942844461217511,-0.333233134534159));
#57231=DIRECTION('center_axis',(0.,0.333233134534162,-0.94284446121751));
#57232=DIRECTION('ref_axis',(0.,0.94284446121751,0.333233134534162));
#57233=DIRECTION('center_axis',(0.,-0.333233134534159,0.942844461217511));
#57234=DIRECTION('ref_axis',(0.,-0.942844461217511,-0.333233134534159));
#57235=DIRECTION('center_axis',(0.,0.333233134534162,-0.94284446121751));
#57236=DIRECTION('ref_axis',(0.,0.94284446121751,0.333233134534162));
#57237=DIRECTION('center_axis',(0.,-0.333233134534159,0.942844461217511));
#57238=DIRECTION('ref_axis',(0.,-0.942844461217511,-0.333233134534159));
#57239=DIRECTION('center_axis',(0.,0.333233134534162,-0.94284446121751));
#57240=DIRECTION('ref_axis',(0.,0.94284446121751,0.333233134534162));
#57241=DIRECTION('center_axis',(0.,-0.333233134534159,0.942844461217511));
#57242=DIRECTION('ref_axis',(0.,-0.942844461217511,-0.333233134534159));
#57243=DIRECTION('center_axis',(0.,0.333233134534162,-0.94284446121751));
#57244=DIRECTION('ref_axis',(0.,0.94284446121751,0.333233134534162));
#57245=DIRECTION('center_axis',(0.,-0.333233134534159,0.942844461217511));
#57246=DIRECTION('ref_axis',(0.,-0.942844461217511,-0.333233134534159));
#57247=DIRECTION('center_axis',(0.,0.333233134534162,-0.94284446121751));
#57248=DIRECTION('ref_axis',(0.,0.94284446121751,0.333233134534162));
#57249=DIRECTION('center_axis',(0.,-0.333233134534159,0.942844461217511));
#57250=DIRECTION('ref_axis',(0.,-0.942844461217511,-0.333233134534159));
#57251=DIRECTION('center_axis',(0.,0.333233134534162,-0.94284446121751));
#57252=DIRECTION('ref_axis',(0.,0.94284446121751,0.333233134534162));
#57253=DIRECTION('center_axis',(0.,-0.333233134534159,0.942844461217511));
#57254=DIRECTION('ref_axis',(0.,-0.942844461217511,-0.333233134534159));
#57255=DIRECTION('center_axis',(0.,0.333233134534162,-0.94284446121751));
#57256=DIRECTION('ref_axis',(0.,0.94284446121751,0.333233134534162));
#57257=DIRECTION('center_axis',(0.,-0.333233134534159,0.942844461217511));
#57258=DIRECTION('ref_axis',(0.,-0.942844461217511,-0.333233134534159));
#57259=DIRECTION('center_axis',(0.,0.333233134534162,-0.94284446121751));
#57260=DIRECTION('ref_axis',(0.,0.94284446121751,0.333233134534162));
#57261=DIRECTION('center_axis',(0.,-0.333233134534159,0.942844461217511));
#57262=DIRECTION('ref_axis',(0.,-0.942844461217511,-0.333233134534159));
#57263=DIRECTION('center_axis',(0.,0.333233134534162,-0.94284446121751));
#57264=DIRECTION('ref_axis',(0.,0.94284446121751,0.333233134534162));
#57265=DIRECTION('center_axis',(0.,-0.333233134534159,0.942844461217511));
#57266=DIRECTION('ref_axis',(0.,-0.942844461217511,-0.333233134534159));
#57267=DIRECTION('center_axis',(0.,0.333233134534162,-0.94284446121751));
#57268=DIRECTION('ref_axis',(0.,0.94284446121751,0.333233134534162));
#57269=DIRECTION('center_axis',(0.,-0.333233134534159,0.942844461217511));
#57270=DIRECTION('ref_axis',(0.,-0.942844461217511,-0.333233134534159));
#57271=DIRECTION('center_axis',(0.,0.333233134534162,-0.94284446121751));
#57272=DIRECTION('ref_axis',(0.,0.94284446121751,0.333233134534162));
#57273=DIRECTION('center_axis',(0.,-0.333233134534159,0.942844461217511));
#57274=DIRECTION('ref_axis',(0.,-0.942844461217511,-0.333233134534159));
#57275=DIRECTION('center_axis',(0.,0.333233134534162,-0.94284446121751));
#57276=DIRECTION('ref_axis',(0.,0.94284446121751,0.333233134534162));
#57277=DIRECTION('center_axis',(0.,-0.333233134534159,0.942844461217511));
#57278=DIRECTION('ref_axis',(0.,-0.942844461217511,-0.333233134534159));
#57279=DIRECTION('center_axis',(0.,0.333233134534162,-0.94284446121751));
#57280=DIRECTION('ref_axis',(0.,0.94284446121751,0.333233134534162));
#57281=DIRECTION('center_axis',(0.,-0.333233134534159,0.942844461217511));
#57282=DIRECTION('ref_axis',(0.,-0.942844461217511,-0.333233134534159));
#57283=DIRECTION('center_axis',(0.,0.333233134534162,-0.94284446121751));
#57284=DIRECTION('ref_axis',(0.,0.94284446121751,0.333233134534162));
#57285=DIRECTION('center_axis',(0.,-0.333233134534159,0.942844461217511));
#57286=DIRECTION('ref_axis',(0.,-0.942844461217511,-0.333233134534159));
#57287=DIRECTION('center_axis',(0.,0.333233134534162,-0.94284446121751));
#57288=DIRECTION('ref_axis',(0.,0.94284446121751,0.333233134534162));
#57289=DIRECTION('center_axis',(0.,-0.333233134534159,0.942844461217511));
#57290=DIRECTION('ref_axis',(0.,-0.942844461217511,-0.333233134534159));
#57291=DIRECTION('center_axis',(0.,0.333233134534162,-0.94284446121751));
#57292=DIRECTION('ref_axis',(0.,0.94284446121751,0.333233134534162));
#57293=DIRECTION('center_axis',(0.,-0.333233134534159,0.942844461217511));
#57294=DIRECTION('ref_axis',(0.,-0.942844461217511,-0.333233134534159));
#57295=DIRECTION('center_axis',(0.,0.333233134534162,-0.94284446121751));
#57296=DIRECTION('ref_axis',(0.,0.94284446121751,0.333233134534162));
#57297=DIRECTION('center_axis',(0.,-0.333233134534159,0.942844461217511));
#57298=DIRECTION('ref_axis',(0.,-0.942844461217511,-0.333233134534159));
#57299=DIRECTION('center_axis',(0.,0.333233134534162,-0.94284446121751));
#57300=DIRECTION('ref_axis',(0.,0.94284446121751,0.333233134534162));
#57301=DIRECTION('center_axis',(0.,-0.333233134534159,0.942844461217511));
#57302=DIRECTION('ref_axis',(0.,-0.942844461217511,-0.333233134534159));
#57303=DIRECTION('center_axis',(0.,0.333233134534162,-0.94284446121751));
#57304=DIRECTION('ref_axis',(0.,0.94284446121751,0.333233134534162));
#57305=DIRECTION('center_axis',(0.,-0.333233134534159,0.942844461217511));
#57306=DIRECTION('ref_axis',(0.,-0.942844461217511,-0.333233134534159));
#57307=DIRECTION('center_axis',(0.,0.333233134534162,-0.94284446121751));
#57308=DIRECTION('ref_axis',(0.,0.94284446121751,0.333233134534162));
#57309=DIRECTION('center_axis',(0.,-0.333233134534159,0.942844461217511));
#57310=DIRECTION('ref_axis',(0.,-0.942844461217511,-0.333233134534159));
#57311=DIRECTION('center_axis',(0.,0.333233134534162,-0.94284446121751));
#57312=DIRECTION('ref_axis',(0.,0.94284446121751,0.333233134534162));
#57313=DIRECTION('center_axis',(0.,-0.333233134534159,0.942844461217511));
#57314=DIRECTION('ref_axis',(0.,-0.942844461217511,-0.333233134534159));
#57315=DIRECTION('center_axis',(0.,0.333233134534162,-0.94284446121751));
#57316=DIRECTION('ref_axis',(0.,0.94284446121751,0.333233134534162));
#57317=DIRECTION('center_axis',(0.,-0.333233134534159,0.942844461217511));
#57318=DIRECTION('ref_axis',(0.,-0.942844461217511,-0.333233134534159));
#57319=DIRECTION('center_axis',(0.,0.333233134534162,-0.94284446121751));
#57320=DIRECTION('ref_axis',(0.,0.94284446121751,0.333233134534162));
#57321=DIRECTION('center_axis',(0.,0.333233134534162,-0.94284446121751));
#57322=DIRECTION('ref_axis',(0.,0.94284446121751,0.333233134534162));
#57323=DIRECTION('center_axis',(0.,0.333233134534162,-0.94284446121751));
#57324=DIRECTION('ref_axis',(0.,0.94284446121751,0.333233134534162));
#57325=DIRECTION('center_axis',(0.,0.333233134534162,-0.94284446121751));
#57326=DIRECTION('ref_axis',(0.,0.94284446121751,0.333233134534162));
#57327=DIRECTION('center_axis',(0.,0.333233134534162,-0.94284446121751));
#57328=DIRECTION('ref_axis',(0.,0.94284446121751,0.333233134534162));
#57329=DIRECTION('center_axis',(0.,0.333233134534162,-0.94284446121751));
#57330=DIRECTION('ref_axis',(0.,0.94284446121751,0.333233134534162));
#57331=DIRECTION('center_axis',(0.,0.333233134534162,-0.94284446121751));
#57332=DIRECTION('ref_axis',(0.,0.94284446121751,0.333233134534162));
#57333=DIRECTION('center_axis',(0.,0.333233134534162,-0.94284446121751));
#57334=DIRECTION('ref_axis',(0.,0.94284446121751,0.333233134534162));
#57335=DIRECTION('center_axis',(0.,0.333233134534162,-0.94284446121751));
#57336=DIRECTION('ref_axis',(0.,0.94284446121751,0.333233134534162));
#57337=DIRECTION('center_axis',(0.,0.333233134534162,-0.94284446121751));
#57338=DIRECTION('ref_axis',(0.,0.94284446121751,0.333233134534162));
#57339=DIRECTION('center_axis',(0.,0.333233134534162,-0.94284446121751));
#57340=DIRECTION('ref_axis',(0.,0.94284446121751,0.333233134534162));
#57341=DIRECTION('center_axis',(0.,0.333233134534162,-0.94284446121751));
#57342=DIRECTION('ref_axis',(0.,0.94284446121751,0.333233134534162));
#57343=DIRECTION('center_axis',(0.,0.333233134534162,-0.94284446121751));
#57344=DIRECTION('ref_axis',(0.,0.94284446121751,0.333233134534162));
#57345=DIRECTION('center_axis',(0.,0.333233134534162,-0.94284446121751));
#57346=DIRECTION('ref_axis',(0.,0.94284446121751,0.333233134534162));
#57347=DIRECTION('center_axis',(0.,0.333233134534162,-0.94284446121751));
#57348=DIRECTION('ref_axis',(0.,0.94284446121751,0.333233134534162));
#57349=DIRECTION('center_axis',(0.,-0.333233134534159,0.942844461217511));
#57350=DIRECTION('ref_axis',(0.,-0.942844461217511,-0.333233134534159));
#57351=DIRECTION('center_axis',(0.,0.333233134534162,-0.94284446121751));
#57352=DIRECTION('ref_axis',(0.,0.94284446121751,0.333233134534162));
#57353=DIRECTION('center_axis',(0.,0.333233134534162,-0.94284446121751));
#57354=DIRECTION('ref_axis',(0.,0.94284446121751,0.333233134534162));
#57355=DIRECTION('center_axis',(0.,0.333233134534162,-0.94284446121751));
#57356=DIRECTION('ref_axis',(0.,0.94284446121751,0.333233134534162));
#57357=DIRECTION('center_axis',(0.,-0.333233134534159,0.942844461217511));
#57358=DIRECTION('ref_axis',(0.,-0.942844461217511,-0.333233134534159));
#57359=DIRECTION('center_axis',(0.,0.333233134534162,-0.94284446121751));
#57360=DIRECTION('ref_axis',(0.,0.94284446121751,0.333233134534162));
#57361=DIRECTION('center_axis',(0.,0.333233134534162,-0.94284446121751));
#57362=DIRECTION('ref_axis',(0.,0.94284446121751,0.333233134534162));
#57363=DIRECTION('center_axis',(0.,0.333233134534162,-0.94284446121751));
#57364=DIRECTION('ref_axis',(0.,0.94284446121751,0.333233134534162));
#57365=DIRECTION('center_axis',(0.,-0.333233134534159,0.942844461217511));
#57366=DIRECTION('ref_axis',(0.,-0.942844461217511,-0.333233134534159));
#57367=DIRECTION('center_axis',(0.,0.333233134534162,-0.94284446121751));
#57368=DIRECTION('ref_axis',(0.,0.94284446121751,0.333233134534162));
#57369=DIRECTION('center_axis',(0.,-0.333233134534159,0.942844461217511));
#57370=DIRECTION('ref_axis',(0.,-0.942844461217511,-0.333233134534159));
#57371=DIRECTION('center_axis',(0.,0.333233134534162,-0.94284446121751));
#57372=DIRECTION('ref_axis',(0.,0.94284446121751,0.333233134534162));
#57373=DIRECTION('center_axis',(0.,0.333233134534162,-0.94284446121751));
#57374=DIRECTION('ref_axis',(0.,0.94284446121751,0.333233134534162));
#57375=DIRECTION('center_axis',(0.,0.333233134534162,-0.94284446121751));
#57376=DIRECTION('ref_axis',(0.,0.94284446121751,0.333233134534162));
#57377=DIRECTION('center_axis',(0.,-0.333233134534159,0.942844461217511));
#57378=DIRECTION('ref_axis',(0.,-0.942844461217511,-0.333233134534159));
#57379=DIRECTION('center_axis',(0.,0.333233134534162,-0.94284446121751));
#57380=DIRECTION('ref_axis',(0.,0.94284446121751,0.333233134534162));
#57381=DIRECTION('center_axis',(0.,-0.333233134534159,0.942844461217511));
#57382=DIRECTION('ref_axis',(0.,-0.942844461217511,-0.333233134534159));
#57383=DIRECTION('center_axis',(0.,0.333233134534162,-0.94284446121751));
#57384=DIRECTION('ref_axis',(0.,0.94284446121751,0.333233134534162));
#57385=DIRECTION('center_axis',(0.,0.333233134534162,-0.94284446121751));
#57386=DIRECTION('ref_axis',(0.,0.94284446121751,0.333233134534162));
#57387=DIRECTION('center_axis',(0.,0.333233134534162,-0.94284446121751));
#57388=DIRECTION('ref_axis',(0.,0.94284446121751,0.333233134534162));
#57389=DIRECTION('center_axis',(0.,0.333233134534162,-0.94284446121751));
#57390=DIRECTION('ref_axis',(0.,0.94284446121751,0.333233134534162));
#57391=DIRECTION('center_axis',(0.,0.333233134534162,-0.94284446121751));
#57392=DIRECTION('ref_axis',(0.,0.94284446121751,0.333233134534162));
#57393=DIRECTION('center_axis',(0.,0.333233134534162,-0.94284446121751));
#57394=DIRECTION('ref_axis',(0.,0.94284446121751,0.333233134534162));
#57395=DIRECTION('center_axis',(0.,0.333233134534162,-0.94284446121751));
#57396=DIRECTION('ref_axis',(0.,0.94284446121751,0.333233134534162));
#57397=DIRECTION('center_axis',(0.,0.333233134534162,-0.94284446121751));
#57398=DIRECTION('ref_axis',(0.,0.94284446121751,0.333233134534162));
#57399=DIRECTION('center_axis',(0.,0.333233134534162,-0.94284446121751));
#57400=DIRECTION('ref_axis',(0.,0.94284446121751,0.333233134534162));
#57401=DIRECTION('center_axis',(0.,0.333233134534162,-0.94284446121751));
#57402=DIRECTION('ref_axis',(0.,0.94284446121751,0.333233134534162));
#57403=DIRECTION('center_axis',(0.,0.333233134534162,-0.94284446121751));
#57404=DIRECTION('ref_axis',(0.,0.94284446121751,0.333233134534162));
#57405=DIRECTION('center_axis',(0.,0.333233134534162,-0.94284446121751));
#57406=DIRECTION('ref_axis',(0.,0.94284446121751,0.333233134534162));
#57407=DIRECTION('center_axis',(0.,0.333233134534162,-0.94284446121751));
#57408=DIRECTION('ref_axis',(0.,0.94284446121751,0.333233134534162));
#57409=DIRECTION('center_axis',(0.,0.333233134534162,-0.94284446121751));
#57410=DIRECTION('ref_axis',(0.,0.94284446121751,0.333233134534162));
#57411=DIRECTION('center_axis',(0.,0.333233134534162,-0.94284446121751));
#57412=DIRECTION('ref_axis',(0.,0.94284446121751,0.333233134534162));
#57413=DIRECTION('center_axis',(0.,0.333233134534162,-0.94284446121751));
#57414=DIRECTION('ref_axis',(0.,0.94284446121751,0.333233134534162));
#57415=DIRECTION('center_axis',(0.,0.333233134534162,-0.94284446121751));
#57416=DIRECTION('ref_axis',(0.,0.94284446121751,0.333233134534162));
#57417=DIRECTION('center_axis',(0.,0.333233134534162,-0.94284446121751));
#57418=DIRECTION('ref_axis',(0.,0.94284446121751,0.333233134534162));
#57419=DIRECTION('center_axis',(0.,0.333233134534162,-0.94284446121751));
#57420=DIRECTION('ref_axis',(0.,0.94284446121751,0.333233134534162));
#57421=DIRECTION('center_axis',(0.,0.333233134534162,-0.94284446121751));
#57422=DIRECTION('ref_axis',(0.,0.94284446121751,0.333233134534162));
#57423=DIRECTION('center_axis',(0.,0.333233134534162,-0.94284446121751));
#57424=DIRECTION('ref_axis',(0.,0.94284446121751,0.333233134534162));
#57425=DIRECTION('center_axis',(0.,0.333233134534162,-0.94284446121751));
#57426=DIRECTION('ref_axis',(0.,0.94284446121751,0.333233134534162));
#57427=DIRECTION('center_axis',(0.,0.333233134534162,-0.94284446121751));
#57428=DIRECTION('ref_axis',(0.,0.94284446121751,0.333233134534162));
#57429=DIRECTION('center_axis',(0.,0.333233134534162,-0.94284446121751));
#57430=DIRECTION('ref_axis',(0.,0.94284446121751,0.333233134534162));
#57431=DIRECTION('center_axis',(0.,0.333233134534162,-0.94284446121751));
#57432=DIRECTION('ref_axis',(0.,0.94284446121751,0.333233134534162));
#57433=DIRECTION('center_axis',(0.,0.333233134534162,-0.94284446121751));
#57434=DIRECTION('ref_axis',(0.,0.94284446121751,0.333233134534162));
#57435=DIRECTION('center_axis',(0.,0.333233134534162,-0.94284446121751));
#57436=DIRECTION('ref_axis',(0.,0.94284446121751,0.333233134534162));
#57437=DIRECTION('center_axis',(0.,0.333233134534162,-0.94284446121751));
#57438=DIRECTION('ref_axis',(0.,0.94284446121751,0.333233134534162));
#57439=DIRECTION('center_axis',(0.,0.333233134534162,-0.94284446121751));
#57440=DIRECTION('ref_axis',(0.,0.94284446121751,0.333233134534162));
#57441=DIRECTION('center_axis',(0.,0.333233134534162,-0.94284446121751));
#57442=DIRECTION('ref_axis',(0.,0.94284446121751,0.333233134534162));
#57443=DIRECTION('center_axis',(0.,0.333233134534162,-0.94284446121751));
#57444=DIRECTION('ref_axis',(0.,0.94284446121751,0.333233134534162));
#57445=DIRECTION('center_axis',(0.,0.333233134534162,-0.94284446121751));
#57446=DIRECTION('ref_axis',(0.,0.94284446121751,0.333233134534162));
#57447=DIRECTION('center_axis',(0.,0.333233134534162,-0.94284446121751));
#57448=DIRECTION('ref_axis',(0.,0.94284446121751,0.333233134534162));
#57449=DIRECTION('center_axis',(0.,0.333233134534162,-0.94284446121751));
#57450=DIRECTION('ref_axis',(0.,0.94284446121751,0.333233134534162));
#57451=DIRECTION('center_axis',(0.,0.333233134534162,-0.94284446121751));
#57452=DIRECTION('ref_axis',(0.,0.94284446121751,0.333233134534162));
#57453=DIRECTION('center_axis',(0.,0.333233134534162,-0.94284446121751));
#57454=DIRECTION('ref_axis',(0.,0.94284446121751,0.333233134534162));
#57455=DIRECTION('center_axis',(0.,0.333233134534162,-0.94284446121751));
#57456=DIRECTION('ref_axis',(0.,0.94284446121751,0.333233134534162));
#57457=DIRECTION('center_axis',(0.,0.333233134534162,-0.94284446121751));
#57458=DIRECTION('ref_axis',(0.,0.94284446121751,0.333233134534162));
#57459=DIRECTION('center_axis',(0.,0.333233134534162,-0.94284446121751));
#57460=DIRECTION('ref_axis',(0.,0.94284446121751,0.333233134534162));
#57461=DIRECTION('center_axis',(0.,-0.333233134534159,0.942844461217511));
#57462=DIRECTION('ref_axis',(0.,-0.942844461217511,-0.333233134534159));
#57463=DIRECTION('center_axis',(0.,-0.333233134534162,0.94284446121751));
#57464=DIRECTION('ref_axis',(0.,-0.94284446121751,-0.333233134534162));
#57465=DIRECTION('center_axis',(0.,-0.333233134534159,0.942844461217511));
#57466=DIRECTION('ref_axis',(0.,-0.942844461217511,-0.333233134534159));
#57467=DIRECTION('center_axis',(0.,-0.333233134534162,0.94284446121751));
#57468=DIRECTION('ref_axis',(0.,-0.94284446121751,-0.333233134534162));
#57469=DIRECTION('center_axis',(0.,-0.333233134534159,0.942844461217511));
#57470=DIRECTION('ref_axis',(0.,-0.942844461217511,-0.333233134534159));
#57471=DIRECTION('center_axis',(0.,-0.333233134534162,0.94284446121751));
#57472=DIRECTION('ref_axis',(0.,-0.94284446121751,-0.333233134534162));
#57473=DIRECTION('center_axis',(0.,-0.333233134534159,0.942844461217511));
#57474=DIRECTION('ref_axis',(0.,-0.942844461217511,-0.333233134534159));
#57475=DIRECTION('center_axis',(0.,-0.333233134534162,0.94284446121751));
#57476=DIRECTION('ref_axis',(0.,-0.94284446121751,-0.333233134534162));
#57477=DIRECTION('center_axis',(0.,-0.333233134534159,0.942844461217511));
#57478=DIRECTION('ref_axis',(0.,-0.942844461217511,-0.333233134534159));
#57479=DIRECTION('center_axis',(0.,-0.333233134534162,0.94284446121751));
#57480=DIRECTION('ref_axis',(0.,-0.94284446121751,-0.333233134534162));
#57481=DIRECTION('center_axis',(0.,-0.333233134534159,0.942844461217511));
#57482=DIRECTION('ref_axis',(0.,-0.942844461217511,-0.333233134534159));
#57483=DIRECTION('center_axis',(0.,-0.333233134534162,0.94284446121751));
#57484=DIRECTION('ref_axis',(0.,-0.94284446121751,-0.333233134534162));
#65509=CARTESIAN_POINT('',(0.,0.,0.));
#65510=CARTESIAN_POINT('Origin',(52.8776183915471,752.330434448379,91.3216571729483));
#65511=CARTESIAN_POINT('',(44.574479425553,751.596144557082,91.2509530983505));
#65512=CARTESIAN_POINT('',(44.574479425553,744.926214295584,90.6087118617898));
#65513=CARTESIAN_POINT('',(44.574479425553,752.330434448379,91.3216571729483));
#65514=CARTESIAN_POINT('',(61.1807573575412,751.596144557082,91.2509530983505));
#65515=CARTESIAN_POINT('Origin',(52.8776183915471,751.59614455564,91.2509530980753));
#65516=CARTESIAN_POINT('',(61.1807573575412,744.926214295584,90.6087118617898));
#65517=CARTESIAN_POINT('',(61.1807573575412,752.330434448379,91.3216571729483));
#65518=CARTESIAN_POINT('',(52.8776183915471,744.926214295584,90.6087118617898));
#65519=CARTESIAN_POINT('Origin',(52.8776183915471,751.59614455564,90.6087118617898));
#65520=CARTESIAN_POINT('',(61.1807573575412,751.59614455564,90.6087118617898));
#65521=CARTESIAN_POINT('',(61.1807573575412,751.59614455564,90.6087118617898));
#65522=CARTESIAN_POINT('',(44.574479425553,751.59614455564,90.6087118617898));
#65523=CARTESIAN_POINT('Origin',(52.8776183915471,751.59614455564,90.6087118617898));
#65524=CARTESIAN_POINT('',(44.574479425553,751.59614455564,90.6087118617898));
#65525=CARTESIAN_POINT('Origin',(52.8776183915471,751.59614455564,112.60871186179));
#65526=CARTESIAN_POINT('',(44.574479425553,751.59614455564,112.60871186179));
#65527=CARTESIAN_POINT('',(61.1807573575412,751.59614455564,112.60871186179));
#65528=CARTESIAN_POINT('Origin',(61.1807573575412,751.59614455564,112.60871186179));
#65529=CARTESIAN_POINT('Origin',(44.574479425553,751.59614455564,112.60871186179));
#65530=CARTESIAN_POINT('Origin',(52.8776183915471,736.753459031024,105.895766550631));
#65531=CARTESIAN_POINT('',(61.1807573575412,737.487748923763,98.2698744426026));
#65532=CARTESIAN_POINT('',(61.1807573575412,738.225434976757,90.6087118617898));
#65533=CARTESIAN_POINT('',(61.1807573575412,736.753459031024,105.895766550631));
#65534=CARTESIAN_POINT('',(44.574479425553,737.487748923763,98.2698744426026));
#65535=CARTESIAN_POINT('Origin',(52.8776183915471,737.487748923763,98.2698744426026));
#65536=CARTESIAN_POINT('',(44.574479425553,738.225434976757,90.6087118617898));
#65537=CARTESIAN_POINT('',(44.574479425553,736.753459031024,105.895766550631));
#65538=CARTESIAN_POINT('Origin',(52.8776183915471,738.225434976757,90.6087118617898));
#65539=CARTESIAN_POINT('Origin',(44.574479425553,751.59614455564,112.60871186179));
#65540=CARTESIAN_POINT('',(44.574479425553,737.487748923763,90.6087118617898));
#65541=CARTESIAN_POINT('',(44.574479425553,737.487748923763,112.60871186179));
#65542=CARTESIAN_POINT('',(44.574479425553,751.59614455564,90.6087118617898));
#65543=CARTESIAN_POINT('Origin',(61.1807573575412,751.59614455564,112.60871186179));
#65544=CARTESIAN_POINT('',(61.1807573575412,737.487748923763,90.6087118617898));
#65545=CARTESIAN_POINT('',(61.1807573575412,737.487748923763,112.60871186179));
#65546=CARTESIAN_POINT('',(61.1807573575412,751.59614455564,90.6087118617898));
#65547=CARTESIAN_POINT('Origin',(52.8776183915471,751.59614455564,90.6087118617898));
#65548=CARTESIAN_POINT('Origin',(52.8776183915471,737.487748923763,90.6087118617898));
#65549=CARTESIAN_POINT('Origin',(52.8776183915471,737.487748923763,112.60871186179));
#65550=CARTESIAN_POINT('Origin',(18.9359428831647,828.055101296691,114.974210298));
#65551=CARTESIAN_POINT('',(18.9359428831647,825.603059199699,123.412429725824));
#65552=CARTESIAN_POINT('Origin',(18.9359428831647,825.131636969091,123.245813158557));
#65553=CARTESIAN_POINT('',(18.9359428831647,824.936592930631,125.298118648259));
#65554=CARTESIAN_POINT('',(18.9359428831647,828.5265235273,115.140826865267));
#65555=CARTESIAN_POINT('Origin',(18.9359428831647,824.465170700022,125.131502080992));
#65556=CARTESIAN_POINT('Origin',(18.9359428831647,828.055101296691,114.974210298));
#65557=CARTESIAN_POINT('',(18.9359428831647,826.174413048403,125.73560616057));
#65558=CARTESIAN_POINT('Origin',(18.9359428831647,824.465170700022,125.131502080992));
#65559=CARTESIAN_POINT('',(18.9359428831647,826.840879317471,123.849917238135));
#65560=CARTESIAN_POINT('',(18.9359428831647,829.764343645071,115.578314377579));
#65561=CARTESIAN_POINT('Origin',(18.9359428831647,825.131636969091,123.245813158557));
#65562=CARTESIAN_POINT('Origin',(37.0601473032809,800.968635034531,105.400936627455));
#65563=CARTESIAN_POINT('',(37.0601473032809,798.51659293754,113.839156055278));
#65564=CARTESIAN_POINT('Origin',(37.0601473032809,798.045170706931,113.672539488011));
#65565=CARTESIAN_POINT('',(37.0601473032809,797.850126668471,115.724844977713));
#65566=CARTESIAN_POINT('',(37.0601473032809,801.44005726514,105.567553194722));
#65567=CARTESIAN_POINT('Origin',(37.0601473032809,797.378704437862,115.558228410446));
#65568=CARTESIAN_POINT('Origin',(37.0601473032809,800.968635034531,105.400936627455));
#65569=CARTESIAN_POINT('',(37.0601473032809,799.087946786243,116.162332490025));
#65570=CARTESIAN_POINT('Origin',(37.0601473032809,797.378704437862,115.558228410446));
#65571=CARTESIAN_POINT('',(37.0601473032809,799.754413055311,114.276643567589));
#65572=CARTESIAN_POINT('',(37.0601473032809,802.677877382911,106.005040707033));
#65573=CARTESIAN_POINT('Origin',(37.0601473032809,798.045170706931,113.672539488011));
#65574=CARTESIAN_POINT('Origin',(71.0018228116636,802.224308791869,105.844734220082));
#65575=CARTESIAN_POINT('',(71.0018228116636,799.772266694878,114.282953647905));
#65576=CARTESIAN_POINT('Origin',(71.0018228116636,799.300844464269,114.116337080638));
#65577=CARTESIAN_POINT('',(71.0018228116636,799.105800425809,116.16864257034));
#65578=CARTESIAN_POINT('',(71.0018228116636,802.695731022478,106.011350787349));
#65579=CARTESIAN_POINT('Origin',(71.0018228116636,798.634378195201,116.002026003073));
#65580=CARTESIAN_POINT('Origin',(71.0018228116636,802.224308791869,105.844734220082));
#65581=CARTESIAN_POINT('',(71.0018228116636,800.343620543581,116.606130082651));
#65582=CARTESIAN_POINT('Origin',(71.0018228116636,798.634378195201,116.002026003073));
#65583=CARTESIAN_POINT('',(71.0018228116636,801.010086812649,114.720441160216));
#65584=CARTESIAN_POINT('',(71.0018228116636,803.933551140249,106.44883829966));
#65585=CARTESIAN_POINT('Origin',(71.0018228116636,799.300844464269,114.116337080638));
#65586=CARTESIAN_POINT('Origin',(86.81929389993,830.566448811367,115.861805483254));
#65587=CARTESIAN_POINT('',(86.81929389993,828.114406714375,124.300024911078));
#65588=CARTESIAN_POINT('Origin',(86.81929389993,827.642984483766,124.13340834381));
#65589=CARTESIAN_POINT('',(86.81929389993,827.447940445307,126.185713833513));
#65590=CARTESIAN_POINT('',(86.81929389993,831.037871041975,116.028422050521));
#65591=CARTESIAN_POINT('Origin',(86.81929389993,826.976518214698,126.019097266246));
#65592=CARTESIAN_POINT('Origin',(86.81929389993,830.566448811367,115.861805483254));
#65593=CARTESIAN_POINT('',(86.81929389993,828.685760563078,126.623201345824));
#65594=CARTESIAN_POINT('Origin',(86.81929389993,826.976518214698,126.019097266246));
#65595=CARTESIAN_POINT('',(86.81929389993,829.352226832147,124.737512423389));
#65596=CARTESIAN_POINT('',(86.81929389993,832.275691159747,116.465909562833));
#65597=CARTESIAN_POINT('Origin',(86.81929389993,827.642984483766,124.13340834381));
#65598=CARTESIAN_POINT('Origin',(68.6950894798137,857.652915073526,125.4350791538));
#65599=CARTESIAN_POINT('',(68.6950894798137,855.200872976535,133.873298581623));
#65600=CARTESIAN_POINT('Origin',(68.6950894798137,854.729450745926,133.706682014356));
#65601=CARTESIAN_POINT('',(68.6950894798137,854.534406707466,135.758987504058));
#65602=CARTESIAN_POINT('',(68.6950894798137,858.124337304135,125.601695721067));
#65603=CARTESIAN_POINT('Origin',(68.6950894798137,854.062984476858,135.592370936791));
#65604=CARTESIAN_POINT('Origin',(68.6950894798137,857.652915073526,125.4350791538));
#65605=CARTESIAN_POINT('',(68.6950894798137,855.772226825238,136.196475016369));
#65606=CARTESIAN_POINT('Origin',(68.6950894798137,854.062984476858,135.592370936791));
#65607=CARTESIAN_POINT('',(68.6950894798137,856.438693094306,134.310786093934));
#65608=CARTESIAN_POINT('',(68.6950894798137,859.362157421907,126.039183233378));
#65609=CARTESIAN_POINT('Origin',(68.6950894798137,854.729450745926,133.706682014356));
#65610=CARTESIAN_POINT('Origin',(34.7534139714311,856.397241316188,124.991281561173));
#65611=CARTESIAN_POINT('',(34.7534139714311,853.945199219197,133.429500988996));
#65612=CARTESIAN_POINT('Origin',(34.7534139714311,853.473776988588,133.262884421729));
#65613=CARTESIAN_POINT('',(34.7534139714311,853.278732950129,135.315189911431));
#65614=CARTESIAN_POINT('',(34.7534139714311,856.868663546797,125.15789812844));
#65615=CARTESIAN_POINT('Origin',(34.7534139714311,852.80731071952,135.148573344164));
#65616=CARTESIAN_POINT('Origin',(34.7534139714311,856.397241316188,124.991281561173));
#65617=CARTESIAN_POINT('',(34.7534139714311,854.5165530679,135.752677423742));
#65618=CARTESIAN_POINT('Origin',(34.7534139714311,852.80731071952,135.148573344164));
#65619=CARTESIAN_POINT('',(34.7534139714311,855.183019336969,133.866988501307));
#65620=CARTESIAN_POINT('',(34.7534139714311,858.106483664569,125.595385640751));
#65621=CARTESIAN_POINT('Origin',(34.7534139714311,853.473776988588,133.262884421729));
#65622=CARTESIAN_POINT('Origin',(-1.20267165682036,833.015540270651,116.727397272047));
#65623=CARTESIAN_POINT('',(-1.20267165682034,828.334694790224,127.12619746849));
#65624=CARTESIAN_POINT('',(-1.20267165689381,830.114166174335,127.781606968093));
#65625=CARTESIAN_POINT('Ctrl Pts',(-1.20267165682036,828.334694790224,127.12619746849));
#65626=CARTESIAN_POINT('Ctrl Pts',(-1.3291142188831,828.327437388836,127.146731443034));
#65627=CARTESIAN_POINT('Ctrl Pts',(-1.45430614477952,828.343822635535,127.176277230326));
#65628=CARTESIAN_POINT('Ctrl Pts',(-1.68514549780207,828.421280943045,127.249050764508));
#65629=CARTESIAN_POINT('Ctrl Pts',(-1.78913151791979,828.480813166934,127.291365400256));
#65630=CARTESIAN_POINT('Ctrl Pts',(-1.96268735299014,828.63467591294,127.382585424871));
#65631=CARTESIAN_POINT('Ctrl Pts',(-2.03128818522246,828.726948767031,127.430517553467));
#65632=CARTESIAN_POINT('Ctrl Pts',(-2.12497808078248,828.93287659233,127.525644047322));
#65633=CARTESIAN_POINT('Ctrl Pts',(-2.14960818542247,829.044222386194,127.571881210666));
#65634=CARTESIAN_POINT('Ctrl Pts',(-2.15183078840391,829.273431394245,127.657118282923));
#65635=CARTESIAN_POINT('Ctrl Pts',(-2.12918070135601,829.388843907327,127.695159946446));
#65636=CARTESIAN_POINT('Ctrl Pts',(-2.03824460180004,829.609963821869,127.758397540592));
#65637=CARTESIAN_POINT('Ctrl Pts',(-1.97014853040882,829.713054774199,127.782671606508));
#65638=CARTESIAN_POINT('Ctrl Pts',(-1.79626212620278,829.892523762626,127.814159147211));
#65639=CARTESIAN_POINT('Ctrl Pts',(-1.69155932791356,829.966552839317,127.82074104684));
#65640=CARTESIAN_POINT('Ctrl Pts',(-1.45854118760016,830.074434502816,127.815266376305));
#65641=CARTESIAN_POINT('Ctrl Pts',(-1.33197961484755,830.106424544809,127.80289079258));
#65642=CARTESIAN_POINT('Ctrl Pts',(-1.2041959927763,830.114076056837,127.781858267725));
#65643=CARTESIAN_POINT('Ctrl Pts',(-1.20368786395239,830.114106482911,127.781774632343));
#65644=CARTESIAN_POINT('Ctrl Pts',(-1.20317975185534,830.11413652206,127.781690865762));
#65645=CARTESIAN_POINT('Ctrl Pts',(-1.20267165696724,830.114166174335,127.781606968093));
#65646=CARTESIAN_POINT('',(-1.20267165682039,830.786433008964,125.879506018928));
#65647=CARTESIAN_POINT('',(-1.20267165682036,833.90943644327,117.043330425183));
#65648=CARTESIAN_POINT('Ctrl Pts',(-2.14826343637025,829.917241856529,125.699848416551));
#65649=CARTESIAN_POINT('Ctrl Pts',(-2.13968331783687,830.028581984869,125.739199785193));
#65650=CARTESIAN_POINT('Ctrl Pts',(-2.10906597586262,830.138399269345,125.774665152322));
#65651=CARTESIAN_POINT('Ctrl Pts',(-2.00423449611768,830.349368657819,125.835950927927));
#65652=CARTESIAN_POINT('Ctrl Pts',(-1.92876920194896,830.447515187103,125.860493869567));
#65653=CARTESIAN_POINT('Ctrl Pts',(-1.74517237638948,830.610903128901,125.89303488207));
#65654=CARTESIAN_POINT('Ctrl Pts',(-1.6393470870339,830.675148515068,125.901011837026));
#65655=CARTESIAN_POINT('Ctrl Pts',(-1.40805851153518,830.764006551829,125.900183193205));
#65656=CARTESIAN_POINT('Ctrl Pts',(-1.28442099189681,830.787154608998,125.891119405913));
#65657=CARTESIAN_POINT('Ctrl Pts',(-1.03549471494797,830.787627832663,125.856694388783));
#65658=CARTESIAN_POINT('Ctrl Pts',(-0.912507313011831,830.764379738259,
125.831453139541));
#65659=CARTESIAN_POINT('Ctrl Pts',(-0.685066390374408,830.673330581152,
125.767818087782));
#65660=CARTESIAN_POINT('Ctrl Pts',(-0.582847405174743,830.606301586927,
125.73000134134));
#65661=CARTESIAN_POINT('Ctrl Pts',(-0.417444637388589,830.440518446962,
125.648255064278));
#65662=CARTESIAN_POINT('Ctrl Pts',(-0.354334495380809,830.344757667241,
125.605401289678));
#65663=CARTESIAN_POINT('Ctrl Pts',(-0.272235940190863,830.137680511632,
125.519746988106));
#65664=CARTESIAN_POINT('Ctrl Pts',(-0.252596354959246,830.028841515062,
125.477755754259));
#65665=CARTESIAN_POINT('Ctrl Pts',(-0.256908479385002,829.807553875916,
125.397939782603));
#65666=CARTESIAN_POINT('Ctrl Pts',(-0.281063582749534,829.697120774919,
125.360871691001));
#65667=CARTESIAN_POINT('Ctrl Pts',(-0.371978455736119,829.48586098202,125.295656791375));
#65668=CARTESIAN_POINT('Ctrl Pts',(-0.438971591876693,829.387393335529,
125.268401313436));
#65669=CARTESIAN_POINT('Ctrl Pts',(-0.611791129636721,829.213469532326,
125.227497034506));
#65670=CARTESIAN_POINT('Ctrl Pts',(-0.71768204207598,829.141291221418,125.215068563833));
#65671=CARTESIAN_POINT('Ctrl Pts',(-0.94855904425708,829.040221526745,125.209010221274));
#65672=CARTESIAN_POINT('Ctrl Pts',(-1.07088004178212,829.01133993113,125.215023726535));
#65673=CARTESIAN_POINT('Ctrl Pts',(-1.31977016635572,828.998589587703,125.244637629106));
#65674=CARTESIAN_POINT('Ctrl Pts',(-1.44406179396237,829.015467658869,125.268205976454));
#65675=CARTESIAN_POINT('Ctrl Pts',(-1.67726982621071,829.094269915464,125.330137787643));
#65676=CARTESIAN_POINT('Ctrl Pts',(-1.78383407157677,829.15585890019,125.368044484481));
#65677=CARTESIAN_POINT('Ctrl Pts',(-1.9537147677774,829.307840573972,125.448382754829));
#65678=CARTESIAN_POINT('Ctrl Pts',(-2.01902459780627,829.393366107762,125.489290147882));
#65679=CARTESIAN_POINT('Ctrl Pts',(-2.1155257471177,829.588730151941,125.574991781173));
#65680=CARTESIAN_POINT('Ctrl Pts',(-2.14392988243959,829.697750196142,125.619071567142));
#65681=CARTESIAN_POINT('Ctrl Pts',(-2.1514912867446,829.845633941601,125.674194438292));
#65682=CARTESIAN_POINT('Ctrl Pts',(-2.15102207108058,829.881444362415,125.687196370892));
#65683=CARTESIAN_POINT('Ctrl Pts',(-2.14826343637024,829.917241856529,125.699848416551));
#65684=CARTESIAN_POINT('Ctrl Pts',(-1.20267165696725,830.114166174335,127.781606968093));
#65685=CARTESIAN_POINT('Ctrl Pts',(-1.08075513521124,830.121281188299,127.761475862289));
#65686=CARTESIAN_POINT('Ctrl Pts',(-0.959826602679901,830.106116474443,
127.733812530951));
#65687=CARTESIAN_POINT('Ctrl Pts',(-0.730868912708148,830.031822843933,
127.665555151892));
#65688=CARTESIAN_POINT('Ctrl Pts',(-0.625279805937704,829.97244057417,127.625319322289));
#65689=CARTESIAN_POINT('Ctrl Pts',(-0.447392920247649,829.816861543733,
127.537684702249));
#65690=CARTESIAN_POINT('Ctrl Pts',(-0.376667260732679,829.722425613006,
127.49118481603));
#65691=CARTESIAN_POINT('Ctrl Pts',(-0.280809829819228,829.512612223396,
127.39829819797));
#65692=CARTESIAN_POINT('Ctrl Pts',(-0.255751495196176,829.399818558959,
127.352855356984));
#65693=CARTESIAN_POINT('Ctrl Pts',(-0.253491139094301,829.167773722023,
127.267415838435));
#65694=CARTESIAN_POINT('Ctrl Pts',(-0.276786155720067,829.05091066254,127.228372802782));
#65695=CARTESIAN_POINT('Ctrl Pts',(-0.369939352279435,828.828729024651,
127.162251511837));
#65696=CARTESIAN_POINT('Ctrl Pts',(-0.439293744486302,828.725907820965,
127.136015715078));
#65697=CARTESIAN_POINT('Ctrl Pts',(-0.614808006592645,828.549194309779,
127.100810464247));
#65698=CARTESIAN_POINT('Ctrl Pts',(-0.719259927691373,828.477181737511,
127.09225800998));
#65699=CARTESIAN_POINT('Ctrl Pts',(-0.950157935397135,828.373046628809,
127.094515945668));
#65700=CARTESIAN_POINT('Ctrl Pts',(-1.07459576691847,828.342365977433,127.105523095909));
#65701=CARTESIAN_POINT('Ctrl Pts',(-1.20096012459087,828.33479410665,127.125919940975));
#65702=CARTESIAN_POINT('Ctrl Pts',(-1.20181591927738,828.33474390684,127.126058498727));
#65703=CARTESIAN_POINT('Ctrl Pts',(-1.20267165682035,828.334694790224,127.12619746849));
#65704=CARTESIAN_POINT('Origin',(-1.20267165682036,833.015540270651,116.727397272047));
#65705=CARTESIAN_POINT('',(-1.20267165682036,831.352123639145,122.934292515535));
#65706=CARTESIAN_POINT('Origin',(-1.20267165682036,830.880701408536,122.767675948268));
#65707=CARTESIAN_POINT('',(-1.2026716568203,829.69401966521,127.625705181122));
#65708=CARTESIAN_POINT('',(-1.20267165682036,833.48696250126,116.894013839314));
#65709=CARTESIAN_POINT('Ctrl Pts',(-1.20298789650297,828.755542369383,127.280115959316));
#65710=CARTESIAN_POINT('Ctrl Pts',(-1.26887122471697,828.751787433989,127.290865160166));
#65711=CARTESIAN_POINT('Ctrl Pts',(-1.33412418331166,828.760243626981,127.306140151335));
#65712=CARTESIAN_POINT('Ctrl Pts',(-1.45539836846876,828.800520225111,127.343823147789));
#65713=CARTESIAN_POINT('Ctrl Pts',(-1.51042491793021,828.831820515841,127.365848130137));
#65714=CARTESIAN_POINT('Ctrl Pts',(-1.60243301003513,828.912928606751,127.413422591274));
#65715=CARTESIAN_POINT('Ctrl Pts',(-1.63886413982435,828.961661140245,127.438463863894));
#65716=CARTESIAN_POINT('Ctrl Pts',(-1.68873358792721,829.070474044544,127.488316661981));
#65717=CARTESIAN_POINT('Ctrl Pts',(-1.7019139603871,829.129337809819,127.51262594284));
#65718=CARTESIAN_POINT('Ctrl Pts',(-1.70336818240946,829.250386378696,127.557595635152));
#65719=CARTESIAN_POINT('Ctrl Pts',(-1.69154803172257,829.311287908161,127.577763325018));
#65720=CARTESIAN_POINT('Ctrl Pts',(-1.64384832228144,829.427807146915,127.611468761738));
#65721=CARTESIAN_POINT('Ctrl Pts',(-1.60811863359135,829.482076408695,127.624540058091));
#65722=CARTESIAN_POINT('Ctrl Pts',(-1.51662342963629,829.576768936407,127.641807379075));
#65723=CARTESIAN_POINT('Ctrl Pts',(-1.46137405383466,829.61589349437,127.64562967002));
#65724=CARTESIAN_POINT('Ctrl Pts',(-1.3387017035892,829.672759375328,127.643299679692));
#65725=CARTESIAN_POINT('Ctrl Pts',(-1.27227880068162,829.689651767026,127.637030621277));
#65726=CARTESIAN_POINT('Ctrl Pts',(-1.13852642382636,829.698056300692,127.615272519426));
#65727=CARTESIAN_POINT('Ctrl Pts',(-1.07240032751607,829.689653389529,127.600037251621));
#65728=CARTESIAN_POINT('Ctrl Pts',(-0.949560991481654,829.648697322975,
127.562662456503));
#65729=CARTESIAN_POINT('Ctrl Pts',(-0.893904099793958,829.616719276534,
127.540922137783));
#65730=CARTESIAN_POINT('Ctrl Pts',(-0.801489156487562,829.534118127831,
127.494118858639));
#65731=CARTESIAN_POINT('Ctrl Pts',(-0.765173137461864,829.484772996318,
127.469596522221));
#65732=CARTESIAN_POINT('Ctrl Pts',(-0.715749284920526,829.374827607324,
127.420534890526));
#65733=CARTESIAN_POINT('Ctrl Pts',(-0.702925728831747,829.315445699046,
127.396489634076));
#65734=CARTESIAN_POINT('Ctrl Pts',(-0.702425039945017,829.193907478153,
127.351746728171));
#65735=CARTESIAN_POINT('Ctrl Pts',(-0.714756156375707,829.133015743589,
127.33151451947));
#65736=CARTESIAN_POINT('Ctrl Pts',(-0.763581488527736,829.016671918521,
127.2972799177));
#65737=CARTESIAN_POINT('Ctrl Pts',(-0.799999909523447,828.962580079425,
127.283766673945));
#65738=CARTESIAN_POINT('Ctrl Pts',(-0.892604933571247,828.868976250883,
127.26570534795));
#65739=CARTESIAN_POINT('Ctrl Pts',(-0.948103826096839,828.830643552855,
127.261474926263));
#65740=CARTESIAN_POINT('Ctrl Pts',(-1.07061270446102,828.775475790961,127.263227961856));
#65741=CARTESIAN_POINT('Ctrl Pts',(-1.13652913761774,828.759330100707,127.269272874018));
#65742=CARTESIAN_POINT('Ctrl Pts',(-1.20298789650297,828.755542369383,127.280115959316));
#65743=CARTESIAN_POINT('Origin',(6.55478737542994,847.253007595304,121.759399961329));
#65744=CARTESIAN_POINT('',(6.55478737542992,842.677000252971,131.641535184651));
#65745=CARTESIAN_POINT('',(6.55478737542993,844.584249391867,132.375487632912));
#65746=CARTESIAN_POINT('Ctrl Pts',(6.55478737542991,842.677000252971,131.641535184651));
#65747=CARTESIAN_POINT('Ctrl Pts',(6.55303790676142,842.676966746103,131.641629988445));
#65748=CARTESIAN_POINT('Ctrl Pts',(6.5512882317057,842.676937403425,131.641726498407));
#65749=CARTESIAN_POINT('Ctrl Pts',(6.41373413291095,842.674958404046,131.649447180971));
#65750=CARTESIAN_POINT('Ctrl Pts',(6.2794941213037,842.698132529524,131.66722321588));
#65751=CARTESIAN_POINT('Ctrl Pts',(6.03154658372636,842.791160631172,131.720813774759));
#65752=CARTESIAN_POINT('Ctrl Pts',(5.91994139510763,842.859481708406,131.755862738239));
#65753=CARTESIAN_POINT('Ctrl Pts',(5.73273525877527,843.032411930828,131.838382174141));
#65754=CARTESIAN_POINT('Ctrl Pts',(5.6587689273465,843.135292902605,131.88502954403));
#65755=CARTESIAN_POINT('Ctrl Pts',(5.55849985454393,843.362329295746,131.983106345019));
#65756=CARTESIAN_POINT('Ctrl Pts',(5.53294178186754,843.484253043593,132.033574133132));
#65757=CARTESIAN_POINT('Ctrl Pts',(5.53382741502631,843.731867371789,132.131263306231));
#65758=CARTESIAN_POINT('Ctrl Pts',(5.5602262917009,843.85513724034,132.177522209149));
#65759=CARTESIAN_POINT('Ctrl Pts',(5.66228992565744,844.087427841061,132.259627098616));
#65760=CARTESIAN_POINT('Ctrl Pts',(5.73714625520192,844.194049471479,132.294601117337));
#65761=CARTESIAN_POINT('Ctrl Pts',(5.92629383071629,844.376164218133,132.348689178051));
#65762=CARTESIAN_POINT('Ctrl Pts',(6.03893300012467,844.449643022453,132.367175469941));
#65763=CARTESIAN_POINT('Ctrl Pts',(6.28711596896352,844.552556231306,132.385476700563));
#65764=CARTESIAN_POINT('Ctrl Pts',(6.4203220368891,844.580860808567,132.3850752359));
#65765=CARTESIAN_POINT('Ctrl Pts',(6.5547873754299,844.584249391867,132.375487632912));
#65766=CARTESIAN_POINT('',(6.55478737646738,845.225288746624,130.561741212106));
#65767=CARTESIAN_POINT('',(6.55478737542994,848.216036735547,122.099767044397));
#65768=CARTESIAN_POINT('Ctrl Pts',(5.60999635886,844.61143003858,130.398176720001));
#65769=CARTESIAN_POINT('Ctrl Pts',(5.66060421325564,844.727579351653,130.439227817251));
#65770=CARTESIAN_POINT('Ctrl Pts',(5.73480526396349,844.833978699371,130.474516036691));
#65771=CARTESIAN_POINT('Ctrl Pts',(5.92197687730667,845.015281112435,130.529742818498));
#65772=CARTESIAN_POINT('Ctrl Pts',(6.03312264845888,845.088412618786,130.549147387708));
#65773=CARTESIAN_POINT('Ctrl Pts',(6.27847082239455,845.191632644705,130.569776359054));
#65774=CARTESIAN_POINT('Ctrl Pts',(6.41041618741639,845.220536970346,130.570730292764));
#65775=CARTESIAN_POINT('Ctrl Pts',(6.67790868490085,845.229442389718,130.554113051095));
#65776=CARTESIAN_POINT('Ctrl Pts',(6.81092204572145,845.209142652417,130.536625508053));
#65777=CARTESIAN_POINT('Ctrl Pts',(7.05983328010717,845.121243103356,130.485463008613));
#65778=CARTESIAN_POINT('Ctrl Pts',(7.17333222258342,845.054432865275,130.452260839241));
#65779=CARTESIAN_POINT('Ctrl Pts',(7.36432235367931,844.883570080731,130.37466281296));
#65780=CARTESIAN_POINT('Ctrl Pts',(7.44032470527312,844.781503834337,130.331108901728));
#65781=CARTESIAN_POINT('Ctrl Pts',(7.5462596693881,844.553385257458,130.238079676163));
#65782=CARTESIAN_POINT('Ctrl Pts',(7.57454430994381,844.429302892799,130.18944702958));
#65783=CARTESIAN_POINT('Ctrl Pts',(7.57770914177435,844.176793165481,130.093710651757));
#65784=CARTESIAN_POINT('Ctrl Pts',(7.55247229926116,844.050879973687,130.047557195243));
#65785=CARTESIAN_POINT('Ctrl Pts',(7.45175414255303,843.815798288611,129.964375202193));
#65786=CARTESIAN_POINT('Ctrl Pts',(7.37775872910222,843.70877597874,129.928074640688));
#65787=CARTESIAN_POINT('Ctrl Pts',(7.19052260488021,843.526789513878,129.869935499952));
#65788=CARTESIAN_POINT('Ctrl Pts',(7.0791397409318,843.453575009385,129.848659915797));
#65789=CARTESIAN_POINT('Ctrl Pts',(6.83389387739383,843.350924365173,129.824455764558));
#65790=CARTESIAN_POINT('Ctrl Pts',(6.70247479869712,843.322328360243,129.821707600764));
#65791=CARTESIAN_POINT('Ctrl Pts',(6.43533783189951,843.313366162955,129.835543150273));
#65792=CARTESIAN_POINT('Ctrl Pts',(6.30218241860372,843.333492045012,129.852161243939));
#65793=CARTESIAN_POINT('Ctrl Pts',(6.05154626048353,843.421068675173,129.903245440815));
#65794=CARTESIAN_POINT('Ctrl Pts',(5.93672077240539,843.48822147147,129.937421063615));
#65795=CARTESIAN_POINT('Ctrl Pts',(5.74402223653652,843.65999995787,130.01814503857));
#65796=CARTESIAN_POINT('Ctrl Pts',(5.66759854594246,843.762573828124,130.063778460294));
#65797=CARTESIAN_POINT('Ctrl Pts',(5.56246946534555,843.990325593362,130.160418011578));
#65798=CARTESIAN_POINT('Ctrl Pts',(5.53472239572821,844.113274934977,130.210474525316));
#65799=CARTESIAN_POINT('Ctrl Pts',(5.53277376714332,844.30146602845,130.283852718444));
#65800=CARTESIAN_POINT('Ctrl Pts',(5.53884227970387,844.364603779265,130.307934207726));
#65801=CARTESIAN_POINT('Ctrl Pts',(5.56440372553955,844.489907018077,130.354616535628));
#65802=CARTESIAN_POINT('Ctrl Pts',(5.5839832628442,844.55172777953,130.377075921576));
#65803=CARTESIAN_POINT('Ctrl Pts',(5.60999635885999,844.61143003858,130.398176720001));
#65804=CARTESIAN_POINT('Ctrl Pts',(6.5547873754299,844.584249391867,132.375487632912));
#65805=CARTESIAN_POINT('Ctrl Pts',(6.55480622813589,844.584249866963,132.375486288682));
#65806=CARTESIAN_POINT('Ctrl Pts',(6.55482508086662,844.58425034157,132.375484944272));
#65807=CARTESIAN_POINT('Ctrl Pts',(6.55484393362206,844.584250815686,132.375483599682));
#65808=CARTESIAN_POINT('Ctrl Pts',(6.68623894655647,844.587555190458,132.366112421274));
#65809=CARTESIAN_POINT('Ctrl Pts',(6.81642370072574,844.567003761885,132.348152635533));
#65810=CARTESIAN_POINT('Ctrl Pts',(7.06398759568666,844.478908057817,132.296499199516));
#65811=CARTESIAN_POINT('Ctrl Pts',(7.17839446645992,844.410728578013,132.262825655811));
#65812=CARTESIAN_POINT('Ctrl Pts',(7.37002394334276,844.23639007631,132.18469173527));
#65813=CARTESIAN_POINT('Ctrl Pts',(7.44575283668634,844.132356427329,132.141104935307));
#65814=CARTESIAN_POINT('Ctrl Pts',(7.54923081147987,843.901799809453,132.048801961113));
#65815=CARTESIAN_POINT('Ctrl Pts',(7.57598548488475,843.777573322673,132.000982234916));
#65816=CARTESIAN_POINT('Ctrl Pts',(7.57640419121021,843.525170126346,131.906562051835));
#65817=CARTESIAN_POINT('Ctrl Pts',(7.54985107163003,843.39949110052,131.860890489685));
#65818=CARTESIAN_POINT('Ctrl Pts',(7.44627657764221,843.1643784139,131.777803202536));
#65819=CARTESIAN_POINT('Ctrl Pts',(7.37028164579431,843.057273335293,131.741210390762));
#65820=CARTESIAN_POINT('Ctrl Pts',(7.17909431489495,842.876627618429,131.682596366717));
#65821=CARTESIAN_POINT('Ctrl Pts',(7.06594289073692,842.804729314389,131.661109320234));
#65822=CARTESIAN_POINT('Ctrl Pts',(6.81873561039477,842.705983821545,131.636976560333));
#65823=CARTESIAN_POINT('Ctrl Pts',(6.68735363927127,842.679539241202,131.634351412262));
#65824=CARTESIAN_POINT('Ctrl Pts',(6.55478737542991,842.677000252971,131.641535184651));
#65825=CARTESIAN_POINT('Origin',(6.55478737542994,847.253007595304,121.759399961329));
#65826=CARTESIAN_POINT('',(6.55478737542994,845.589590963798,127.966295204818));
#65827=CARTESIAN_POINT('Origin',(6.55478737542994,845.118168733189,127.799678637551));
#65828=CARTESIAN_POINT('',(6.55478737543003,844.09812975394,132.186211518965));
#65829=CARTESIAN_POINT('',(6.55478737542994,847.724429825913,121.926016528596));
#65830=CARTESIAN_POINT('Ctrl Pts',(6.55481851312468,843.164473852138,131.826980425391));
#65831=CARTESIAN_POINT('Ctrl Pts',(6.49382472049681,843.163209185906,131.830547252986));
#65832=CARTESIAN_POINT('Ctrl Pts',(6.43336250093996,843.172340323356,131.838191491812));
#65833=CARTESIAN_POINT('Ctrl Pts',(6.31517108154337,843.211873723551,131.861776761809));
#65834=CARTESIAN_POINT('Ctrl Pts',(6.25911871175114,843.24345373982,131.878076868745));
#65835=CARTESIAN_POINT('Ctrl Pts',(6.16392510454186,843.325110848359,131.916860147554));
#65836=CARTESIAN_POINT('Ctrl Pts',(6.12563808773415,843.37436783186,131.938957654843));
#65837=CARTESIAN_POINT('Ctrl Pts',(6.07204655748402,843.484148214731,131.98587934228));
#65838=CARTESIAN_POINT('Ctrl Pts',(6.05717241963223,843.54358604734,132.010242691029));
#65839=CARTESIAN_POINT('Ctrl Pts',(6.05293317978062,843.665034674381,132.057919717385));
#65840=CARTESIAN_POINT('Ctrl Pts',(6.06357636693077,843.725858898406,132.080767224076));
#65841=CARTESIAN_POINT('Ctrl Pts',(6.10927807047822,843.841077253218,132.121902922219));
#65842=CARTESIAN_POINT('Ctrl Pts',(6.14393797108856,843.894313107552,132.139772164867));
#65843=CARTESIAN_POINT('Ctrl Pts',(6.23305703868034,843.986063403245,132.168160912873));
#65844=CARTESIAN_POINT('Ctrl Pts',(6.28671435890372,844.023605589203,132.178370566321));
#65845=CARTESIAN_POINT('Ctrl Pts',(6.40605752914277,844.077640466166,132.189790697383));
#65846=CARTESIAN_POINT('Ctrl Pts',(6.47061868105095,844.093540264309,132.190865731911));
#65847=CARTESIAN_POINT('Ctrl Pts',(6.60263192308899,844.10124280269,132.183755074975));
#65848=CARTESIAN_POINT('Ctrl Pts',(6.66881976307734,844.092705764824,132.175541289738));
#65849=CARTESIAN_POINT('Ctrl Pts',(6.79335192706539,844.05171026747,132.150834900201));
#65850=CARTESIAN_POINT('Ctrl Pts',(6.85043847313586,844.019558982461,132.134552843621));
#65851=CARTESIAN_POINT('Ctrl Pts',(6.94696815080633,843.93604369985,132.096143876332));
#65852=CARTESIAN_POINT('Ctrl Pts',(6.98555744226268,843.885615368059,132.074427178142));
#65853=CARTESIAN_POINT('Ctrl Pts',(7.03907629503223,843.773133595323,132.028241411814));
#65854=CARTESIAN_POINT('Ctrl Pts',(7.05349101350017,843.712215014848,132.004231698388));
#65855=CARTESIAN_POINT('Ctrl Pts',(7.05591879218544,843.588034847224,131.95694833136));
#65856=CARTESIAN_POINT('Ctrl Pts',(7.04386252616135,843.526023081629,131.934149518317));
#65857=CARTESIAN_POINT('Ctrl Pts',(6.99459986187663,843.409564880055,131.892876156114));
#65858=CARTESIAN_POINT('Ctrl Pts',(6.95788872341961,843.356295342004,131.874818710348));
#65859=CARTESIAN_POINT('Ctrl Pts',(6.86471312661731,843.265977604734,131.846072563347));
#65860=CARTESIAN_POINT('Ctrl Pts',(6.80921918804558,843.229809044465,131.835663634095));
#65861=CARTESIAN_POINT('Ctrl Pts',(6.68682008321809,843.179487726841,131.824116116221));
#65862=CARTESIAN_POINT('Ctrl Pts',(6.62113381468758,843.165848856363,131.823102403754));
#65863=CARTESIAN_POINT('Ctrl Pts',(6.55481851312468,843.164473852138,131.826980425391));
#65864=CARTESIAN_POINT('Origin',(0.796070088965373,843.535854240486,120.445632192709));
#65865=CARTESIAN_POINT('',(0.796070088965328,838.864125149569,130.818638623573));
#65866=CARTESIAN_POINT('',(0.796070088870976,840.620830057273,131.538463224669));
#65867=CARTESIAN_POINT('Ctrl Pts',(0.796070088965304,838.864125149569,130.818638623573));
#65868=CARTESIAN_POINT('Ctrl Pts',(0.794827698097562,838.864057778329,130.818829242672));
#65869=CARTESIAN_POINT('Ctrl Pts',(0.793585218870054,838.863992651324,130.81902084043));
#65870=CARTESIAN_POINT('Ctrl Pts',(0.665663372755533,838.857518991375,130.838846563929));
#65871=CARTESIAN_POINT('Ctrl Pts',(0.540503522400223,838.874558326616,130.868296531431));
#65872=CARTESIAN_POINT('Ctrl Pts',(0.3092728956842,838.95277065554,130.942868566291));
#65873=CARTESIAN_POINT('Ctrl Pts',(0.205004865688482,839.012754838599,130.987154596652));
#65874=CARTESIAN_POINT('Ctrl Pts',(0.0315660344768318,839.167045965043,
131.083967170336));
#65875=CARTESIAN_POINT('Ctrl Pts',(-0.0366671735241947,839.259396874592,
131.135483488003));
#65876=CARTESIAN_POINT('Ctrl Pts',(-0.128592083149956,839.464373004797,
131.238526591522));
#65877=CARTESIAN_POINT('Ctrl Pts',(-0.152136571347762,839.574692592277,
131.289052191409));
#65878=CARTESIAN_POINT('Ctrl Pts',(-0.151891702170995,839.800490232602,
131.38283457539));
#65879=CARTESIAN_POINT('Ctrl Pts',(-0.128294067025386,839.913586090429,
131.425133728983));
#65880=CARTESIAN_POINT('Ctrl Pts',(-0.0360050571459805,840.129586582997,
131.496426943252));
#65881=CARTESIAN_POINT('Ctrl Pts',(0.0322173588675454,840.229979376594,
131.524472423262));
#65882=CARTESIAN_POINT('Ctrl Pts',(0.205944640509112,840.404927795732,131.562614261849));
#65883=CARTESIAN_POINT('Ctrl Pts',(0.310325571819949,840.477066589318,131.571943694023));
#65884=CARTESIAN_POINT('Ctrl Pts',(0.542115274605274,840.582108231562,131.570482146171));
#65885=CARTESIAN_POINT('Ctrl Pts',(0.667674821467832,840.613202212936,131.559325066392));
#65886=CARTESIAN_POINT('Ctrl Pts',(0.794285400310592,840.620725573823,131.538753807651));
#65887=CARTESIAN_POINT('Ctrl Pts',(0.794880322885515,840.620760924875,131.538657146642));
#65888=CARTESIAN_POINT('Ctrl Pts',(0.795475219297333,840.620795752662,131.538560285583));
#65889=CARTESIAN_POINT('Ctrl Pts',(0.796070088776574,840.620830057273,131.538463224669));
#65890=CARTESIAN_POINT('',(0.796070088965362,841.298123280429,129.622140692799));
#65891=CARTESIAN_POINT('',(0.796070088965373,844.429750413105,120.761565345845));
#65892=CARTESIAN_POINT('Ctrl Pts',(-0.114573768475245,840.621503109177,
129.483096530971));
#65893=CARTESIAN_POINT('Ctrl Pts',(-0.0816289370406585,840.72872824179,
129.520993520889));
#65894=CARTESIAN_POINT('Ctrl Pts',(-0.0276962030890162,840.830166871951,
129.553497588084));
#65895=CARTESIAN_POINT('Ctrl Pts',(0.12044651238664,841.016067290245,129.605923141397));
#65896=CARTESIAN_POINT('Ctrl Pts',(0.215202624761209,841.097345397984,129.624504212106));
#65897=CARTESIAN_POINT('Ctrl Pts',(0.429070634791453,841.221345788405,129.643124331242));
#65898=CARTESIAN_POINT('Ctrl Pts',(0.545729974921351,841.263543627242,129.643308936973));
#65899=CARTESIAN_POINT('Ctrl Pts',(0.789325626678496,841.305342087345,129.625847846461));
#65900=CARTESIAN_POINT('Ctrl Pts',(0.914171079203174,841.303866240822,129.608081138434));
#65901=CARTESIAN_POINT('Ctrl Pts',(1.15536541434991,841.255770008622,129.556490032213));
#65902=CARTESIAN_POINT('Ctrl Pts',(1.26935916895088,841.209037805329,129.522948704284));
#65903=CARTESIAN_POINT('Ctrl Pts',(1.46957291102217,841.075609376976,129.444335384128));
#65904=CARTESIAN_POINT('Ctrl Pts',(1.55379852050348,840.990104292807,129.399988562346));
#65905=CARTESIAN_POINT('Ctrl Pts',(1.67742500701556,840.795679236415,129.308119262895));
#65906=CARTESIAN_POINT('Ctrl Pts',(1.71741516907379,840.689701531423,129.261654481206));
#65907=CARTESIAN_POINT('Ctrl Pts',(1.75119228074715,840.471141451104,129.171941725508));
#65908=CARTESIAN_POINT('Ctrl Pts',(1.74615787971708,840.360855125383,129.129438956567));
#65909=CARTESIAN_POINT('Ctrl Pts',(1.69303143168079,840.145259473354,129.051634725752));
#65910=CARTESIAN_POINT('Ctrl Pts',(1.64518796173878,840.041961211094,129.017088327572));
#65911=CARTESIAN_POINT('Ctrl Pts',(1.51032859251117,839.8530749561,128.959780993269));
#65912=CARTESIAN_POINT('Ctrl Pts',(1.42360862026976,839.76983980922,128.937909196098));
#65913=CARTESIAN_POINT('Ctrl Pts',(1.21763762780869,839.633452990763,128.910271757672));
#65914=CARTESIAN_POINT('Ctrl Pts',(1.09905060553251,839.583519757645,128.905705450172));
#65915=CARTESIAN_POINT('Ctrl Pts',(0.852986550115753,839.529713465236,128.916351593169));
#65916=CARTESIAN_POINT('Ctrl Pts',(0.728093581363388,839.525330018705,128.931023573232));
#65917=CARTESIAN_POINT('Ctrl Pts',(0.484194615840542,839.561413569164,128.977897026239));
#65918=CARTESIAN_POINT('Ctrl Pts',(0.367560526885127,839.602166643071,129.009903607386));
#65919=CARTESIAN_POINT('Ctrl Pts',(0.159186954517308,839.724728288124,129.087301467092));
#65920=CARTESIAN_POINT('Ctrl Pts',(0.0696508749860938,839.805750216171,
129.13207642363));
#65921=CARTESIAN_POINT('Ctrl Pts',(-0.0611587166226164,839.987529379187,
129.222946134897));
#65922=CARTESIAN_POINT('Ctrl Pts',(-0.105441748260835,840.08391523088,129.267691931765));
#65923=CARTESIAN_POINT('Ctrl Pts',(-0.155599545862111,840.293812728813,
129.358530179364));
#65924=CARTESIAN_POINT('Ctrl Pts',(-0.158957976707979,840.40598034632,129.40372242424));
#65925=CARTESIAN_POINT('Ctrl Pts',(-0.133545652799168,840.552095120162,
129.458220080966));
#65926=CARTESIAN_POINT('Ctrl Pts',(-0.125166017890976,840.587028646908,
129.470912089532));
#65927=CARTESIAN_POINT('Ctrl Pts',(-0.114573768475226,840.621503109177,
129.483096530971));
#65928=CARTESIAN_POINT('Ctrl Pts',(0.796070088776549,840.620830057273,131.538463224669));
#65929=CARTESIAN_POINT('Ctrl Pts',(0.919117110633732,840.627925866344,131.518386456895));
#65930=CARTESIAN_POINT('Ctrl Pts',(1.04101449669179,840.612631456257,131.489773246558));
#65931=CARTESIAN_POINT('Ctrl Pts',(1.27106987721238,840.538183828132,131.418089116851));
#65932=CARTESIAN_POINT('Ctrl Pts',(1.37685998985184,840.478851109327,131.375388976825));
#65933=CARTESIAN_POINT('Ctrl Pts',(1.55418389755524,840.32403888529,131.282026824372));
#65934=CARTESIAN_POINT('Ctrl Pts',(1.62438039829403,840.230422130879,131.232331969497));
#65935=CARTESIAN_POINT('Ctrl Pts',(1.71997755586114,840.020721214871,131.13168195422));
#65936=CARTESIAN_POINT('Ctrl Pts',(1.74451008525223,839.906844836805,131.081747906321));
#65937=CARTESIAN_POINT('Ctrl Pts',(1.7437990867947,839.676499988517,130.98891715077));
#65938=CARTESIAN_POINT('Ctrl Pts',(1.71963538228123,839.562495315449,130.946831551189));
#65939=CARTESIAN_POINT('Ctrl Pts',(1.62521025709541,839.344576997806,130.874096289475));
#65940=CARTESIAN_POINT('Ctrl Pts',(1.55492888472768,839.243292762205,130.844512251832));
#65941=CARTESIAN_POINT('Ctrl Pts',(1.37774643215128,839.069982346398,130.803354915119));
#65942=CARTESIAN_POINT('Ctrl Pts',(1.27270211381144,838.999772092652,130.792226269154));
#65943=CARTESIAN_POINT('Ctrl Pts',(1.04253480033382,838.899769675012,130.790398083267));
#65944=CARTESIAN_POINT('Ctrl Pts',(0.919739196074592,838.870831365168,130.799664165218));
#65945=CARTESIAN_POINT('Ctrl Pts',(0.796070088965291,838.864125149569,130.818638623573));
#65946=CARTESIAN_POINT('Origin',(0.796070088965373,843.535854240486,120.445632192709));
#65947=CARTESIAN_POINT('',(0.796070088965373,841.87243760898,126.652527436197));
#65948=CARTESIAN_POINT('Origin',(0.796070088965373,841.401015378371,126.48591086893));
#65949=CARTESIAN_POINT('',(0.796070088965553,840.20622826248,131.366873312312));
#65950=CARTESIAN_POINT('',(0.796070088965373,844.007276471095,120.612248759976));
#65951=CARTESIAN_POINT('Ctrl Pts',(0.795562167795383,839.279741102276,130.987359868053));
#65952=CARTESIAN_POINT('Ctrl Pts',(0.731430348524241,839.276273003913,130.997367951997));
#65953=CARTESIAN_POINT('Ctrl Pts',(0.667960761387491,839.284234123323,131.012060478403));
#65954=CARTESIAN_POINT('Ctrl Pts',(0.546370658361078,839.322949872229,131.050091378513));
#65955=CARTESIAN_POINT('Ctrl Pts',(0.489756979218874,839.35443841009,131.073469241664));
#65956=CARTESIAN_POINT('Ctrl Pts',(0.396272683050392,839.435786511789,131.124336462737));
#65957=CARTESIAN_POINT('Ctrl Pts',(0.35962563070478,839.484265194161,131.151205415196));
#65958=CARTESIAN_POINT('Ctrl Pts',(0.3097598849944,839.592204362186,131.205143643489));
#65959=CARTESIAN_POINT('Ctrl Pts',(0.296659653429387,839.650449381564,131.231684608902));
#65960=CARTESIAN_POINT('Ctrl Pts',(0.295522146159853,839.769777315234,131.281163845474));
#65961=CARTESIAN_POINT('Ctrl Pts',(0.307379297042506,839.829607500631,131.303603261328));
#65962=CARTESIAN_POINT('Ctrl Pts',(0.354957946136456,839.943866973982,131.341673658187));
#65963=CARTESIAN_POINT('Ctrl Pts',(0.390394184750389,839.997002029084,131.356825299141));
#65964=CARTESIAN_POINT('Ctrl Pts',(0.48098165965852,840.089715368037,131.377829139342));
#65965=CARTESIAN_POINT('Ctrl Pts',(0.535518517417103,840.128053538018,131.383290349174));
#65966=CARTESIAN_POINT('Ctrl Pts',(0.657493684472937,840.184536999717,131.383631985095));
#65967=CARTESIAN_POINT('Ctrl Pts',(0.724034462236347,840.201509191044,131.378206313534));
#65968=CARTESIAN_POINT('Ctrl Pts',(0.858253621700997,840.210342346372,131.357106463382));
#65969=CARTESIAN_POINT('Ctrl Pts',(0.924704672466089,840.202192909004,131.341655540851));
#65970=CARTESIAN_POINT('Ctrl Pts',(1.04807337406688,840.161926284063,131.30296106932));
#65971=CARTESIAN_POINT('Ctrl Pts',(1.10395853967236,840.130363981493,131.280127550429));
#65972=CARTESIAN_POINT('Ctrl Pts',(1.19756615135367,840.048035258523,131.230056322029));
#65973=CARTESIAN_POINT('Ctrl Pts',(1.23453049148622,839.99819766724,131.203326248251));
#65974=CARTESIAN_POINT('Ctrl Pts',(1.28378485237463,839.888055818276,131.149983504672));
#65975=CARTESIAN_POINT('Ctrl Pts',(1.29625187582928,839.829164649058,131.123908659801));
#65976=CARTESIAN_POINT('Ctrl Pts',(1.29588526796899,839.709016475608,131.075132935204));
#65977=CARTESIAN_POINT('Ctrl Pts',(1.28318542618251,839.649007168727,131.052914243734));
#65978=CARTESIAN_POINT('Ctrl Pts',(1.23397083316012,839.535181990415,131.015043182221));
#65979=CARTESIAN_POINT('Ctrl Pts',(1.19784873878774,839.482592971347,130.99982322664));
#65980=CARTESIAN_POINT('Ctrl Pts',(1.10569639300086,839.390903804502,130.978341912658));
#65981=CARTESIAN_POINT('Ctrl Pts',(1.05014519878274,839.353176332159,130.972561536973));
#65982=CARTESIAN_POINT('Ctrl Pts',(0.927639293927917,839.299054603199,130.971861820969));
#65983=CARTESIAN_POINT('Ctrl Pts',(0.861843163686722,839.283325423069,130.977016394591));
#65984=CARTESIAN_POINT('Ctrl Pts',(0.795562167795383,839.279741102276,130.987359868053));
#65985=CARTESIAN_POINT('Origin',(11.5235903376672,855.941516570216,124.830213016114));
#65986=CARTESIAN_POINT('',(11.5235903376672,851.368643130532,134.703481225781));
#65987=CARTESIAN_POINT('',(11.5235903376673,853.266588565377,135.463757424364));
#65988=CARTESIAN_POINT('Ctrl Pts',(11.5235903376672,851.368643130532,134.703481225781));
#65989=CARTESIAN_POINT('Ctrl Pts',(11.5205021226678,851.368593808959,134.703620775445));
#65990=CARTESIAN_POINT('Ctrl Pts',(11.5174132752579,851.36855744311,134.703765698308));
#65991=CARTESIAN_POINT('Ctrl Pts',(11.3794022374267,851.367512362552,134.710480119367));
#65992=CARTESIAN_POINT('Ctrl Pts',(11.246127730073,851.391242846567,134.72719324216));
#65993=CARTESIAN_POINT('Ctrl Pts',(10.9990624023133,851.484833008573,134.779260202327));
#65994=CARTESIAN_POINT('Ctrl Pts',(10.8875292827729,851.55347968161,134.813990765133));
#65995=CARTESIAN_POINT('Ctrl Pts',(10.7003910944404,851.726799524684,134.896941108057));
#65996=CARTESIAN_POINT('Ctrl Pts',(10.626505033589,851.829800131095,134.944355825167));
#65997=CARTESIAN_POINT('Ctrl Pts',(10.5266345429849,852.056594180815,135.044993714505));
#65998=CARTESIAN_POINT('Ctrl Pts',(10.5013771736133,852.178179672887,135.097235730556));
#65999=CARTESIAN_POINT('Ctrl Pts',(10.503023411694,852.424395424166,135.199054871647));
#66000=CARTESIAN_POINT('Ctrl Pts',(10.5297458928562,852.546658827902,135.247651124626));
#66001=CARTESIAN_POINT('Ctrl Pts',(10.6322545121574,852.776515752824,135.33451099905));
#66002=CARTESIAN_POINT('Ctrl Pts',(10.7071100086572,852.881800419343,135.371887362115));
#66003=CARTESIAN_POINT('Ctrl Pts',(10.896054365022,853.061541060369,135.43039791291));
#66004=CARTESIAN_POINT('Ctrl Pts',(11.0084685942409,853.134002248043,135.450851545521));
#66005=CARTESIAN_POINT('Ctrl Pts',(11.2562712869861,853.23551591681,135.472220334527));
#66006=CARTESIAN_POINT('Ctrl Pts',(11.3893185237754,853.263374010964,135.472852632822));
#66007=CARTESIAN_POINT('Ctrl Pts',(11.5235903376673,853.266588565377,135.463757424364));
#66008=CARTESIAN_POINT('',(11.5235903391071,853.90899332006,133.646147763011));
#66009=CARTESIAN_POINT('',(11.5235903376672,856.904545710459,125.170580099181));
#66010=CARTESIAN_POINT('Ctrl Pts',(10.680142013218,853.477148071031,133.531621451738));
#66011=CARTESIAN_POINT('Ctrl Pts',(10.7552566727792,853.580838666919,133.568269216784));
#66012=CARTESIAN_POINT('Ctrl Pts',(10.8511384208992,853.670383328694,133.597600419919));
#66013=CARTESIAN_POINT('Ctrl Pts',(11.0735865855287,853.811093672709,133.638480591057));
#66014=CARTESIAN_POINT('Ctrl Pts',(11.1979838140956,853.86088358712,133.649635451893));
#66015=CARTESIAN_POINT('Ctrl Pts',(11.4596338352218,853.913861640245,133.652507210074));
#66016=CARTESIAN_POINT('Ctrl Pts',(11.5944280372036,853.916332889399,133.644118800169));
#66017=CARTESIAN_POINT('Ctrl Pts',(11.8566696033935,853.872743280832,133.608948039412));
#66018=CARTESIAN_POINT('Ctrl Pts',(11.9815853878325,853.826883552933,133.582426730849));
#66019=CARTESIAN_POINT('Ctrl Pts',(12.2042818130555,853.692249125062,133.514746543923));
#66020=CARTESIAN_POINT('Ctrl Pts',(12.2999034801377,853.604715673213,133.474220089617));
#66021=CARTESIAN_POINT('Ctrl Pts',(12.4478498336772,853.40026531813,133.384751079444));
#66022=CARTESIAN_POINT('Ctrl Pts',(12.4991659215438,853.285582203206,133.336737939971));
#66023=CARTESIAN_POINT('Ctrl Pts',(12.55162288623,853.0417674699,133.238161161633));
#66024=CARTESIAN_POINT('Ctrl Pts',(12.5515963550512,852.9148848129,133.188538796986));
#66025=CARTESIAN_POINT('Ctrl Pts',(12.4985600437562,852.667317196894,133.094549128521));
#66026=CARTESIAN_POINT('Ctrl Pts',(12.445994474123,852.549113986541,133.051120640321));
#66027=CARTESIAN_POINT('Ctrl Pts',(12.2956314640741,852.338913678305,132.97673256773));
#66028=CARTESIAN_POINT('Ctrl Pts',(12.1997586031175,852.248724795663,132.94638150898));
#66029=CARTESIAN_POINT('Ctrl Pts',(11.9769114666055,852.107376329575,132.902605212033));
#66030=CARTESIAN_POINT('Ctrl Pts',(11.8521364266482,852.057564352149,132.889600872787));
#66031=CARTESIAN_POINT('Ctrl Pts',(11.5904503957502,852.005149110542,132.883151612586));
#66032=CARTESIAN_POINT('Ctrl Pts',(11.4561071093275,852.002889344376,132.889711566681));
#66033=CARTESIAN_POINT('Ctrl Pts',(11.1940094503849,852.046372682254,132.922083142856));
#66034=CARTESIAN_POINT('Ctrl Pts',(11.0688603989777,852.092095747919,132.947748147312));
#66035=CARTESIAN_POINT('Ctrl Pts',(10.8444080174315,852.226752201474,133.01547194676));
#66036=CARTESIAN_POINT('Ctrl Pts',(10.7476233879218,852.314874914181,133.057059047555));
#66037=CARTESIAN_POINT('Ctrl Pts',(10.5984020412124,852.520536616746,133.14975849757));
#66038=CARTESIAN_POINT('Ctrl Pts',(10.5469174051594,852.635785811548,133.19987180787));
#66039=CARTESIAN_POINT('Ctrl Pts',(10.4954269424383,852.879058095224,133.301996835519));
#66040=CARTESIAN_POINT('Ctrl Pts',(10.4958558425417,853.00471458401,133.353010146666));
#66041=CARTESIAN_POINT('Ctrl Pts',(10.5359244585833,853.189128103142,133.425053217205));
#66042=CARTESIAN_POINT('Ctrl Pts',(10.5559055903532,853.249684413758,133.448222338175));
#66043=CARTESIAN_POINT('Ctrl Pts',(10.6087057436789,853.367222257402,133.492160112676));
#66044=CARTESIAN_POINT('Ctrl Pts',(10.6415321002965,853.423849754811,133.512784023393));
#66045=CARTESIAN_POINT('Ctrl Pts',(10.680142013218,853.477148071031,133.531621451738));
#66046=CARTESIAN_POINT('Ctrl Pts',(11.5235903376673,853.266588565377,135.463757424364));
#66047=CARTESIAN_POINT('Ctrl Pts',(11.5236943901661,853.266591056462,135.46375037613));
#66048=CARTESIAN_POINT('Ctrl Pts',(11.5237984434004,853.266593532747,135.463743322055));
#66049=CARTESIAN_POINT('Ctrl Pts',(11.5239024973665,853.266595994231,135.463736262138));
#66050=CARTESIAN_POINT('Ctrl Pts',(11.6551425361477,853.269700588689,135.454831808873));
#66051=CARTESIAN_POINT('Ctrl Pts',(11.7851296518499,853.249200036743,135.436812128387));
#66052=CARTESIAN_POINT('Ctrl Pts',(12.0334729099227,853.161290212145,135.383955763739));
#66053=CARTESIAN_POINT('Ctrl Pts',(12.1486654966744,853.092808126151,135.348975051315));
#66054=CARTESIAN_POINT('Ctrl Pts',(12.3408496401843,852.917885897015,135.26778523619));
#66055=CARTESIAN_POINT('Ctrl Pts',(12.4164867427695,852.813713385906,135.222532568282));
#66056=CARTESIAN_POINT('Ctrl Pts',(12.5190707641202,852.583469542574,135.127118673292));
#66057=CARTESIAN_POINT('Ctrl Pts',(12.5452809191628,852.459794537162,135.077909345789));
#66058=CARTESIAN_POINT('Ctrl Pts',(12.5447108915423,852.208730494133,134.980949860915));
#66059=CARTESIAN_POINT('Ctrl Pts',(12.5177773471651,852.083827409251,134.934148102748));
#66060=CARTESIAN_POINT('Ctrl Pts',(12.4135224748329,851.849957798997,134.848759380441));
#66061=CARTESIAN_POINT('Ctrl Pts',(12.3370911785135,851.743365151998,134.811036680661));
#66062=CARTESIAN_POINT('Ctrl Pts',(12.1449200415364,851.563846763306,134.750115378063));
#66063=CARTESIAN_POINT('Ctrl Pts',(12.0311862886986,851.492601493932,134.727487315331));
#66064=CARTESIAN_POINT('Ctrl Pts',(11.7845957909319,851.396167511552,134.701317415303));
#66065=CARTESIAN_POINT('Ctrl Pts',(11.6546626058585,851.370736472623,134.697558357399));
#66066=CARTESIAN_POINT('Ctrl Pts',(11.5235903376672,851.368643130532,134.703481225781));
#66067=CARTESIAN_POINT('Origin',(11.5235903376672,855.941516570216,124.830213016114));
#66068=CARTESIAN_POINT('',(11.5235903376672,854.27809993871,131.037108259602));
#66069=CARTESIAN_POINT('Origin',(11.5235903376672,853.806677708101,130.870491692335));
#66070=CARTESIAN_POINT('',(11.5235903376671,852.783421454099,135.266127479096));
#66071=CARTESIAN_POINT('',(11.5235903376672,856.412938800825,124.996829583381));
#66072=CARTESIAN_POINT('Ctrl Pts',(11.5234307913646,851.854317302887,134.894017809227));
#66073=CARTESIAN_POINT('Ctrl Pts',(11.4620605953806,851.8532288306,134.897156281172));
#66074=CARTESIAN_POINT('Ctrl Pts',(11.4012425456016,851.862628695986,134.904523912193));
#66075=CARTESIAN_POINT('Ctrl Pts',(11.2827884647596,851.902731625166,134.927852321044));
#66076=CARTESIAN_POINT('Ctrl Pts',(11.2268079678992,851.934490807818,134.944155309179));
#66077=CARTESIAN_POINT('Ctrl Pts',(11.1317720398537,852.016366574967,134.983364582381));
#66078=CARTESIAN_POINT('Ctrl Pts',(11.0935952813509,852.065685262024,135.005889850397));
#66079=CARTESIAN_POINT('Ctrl Pts',(11.0403322118733,852.175381959815,135.054046308876));
#66080=CARTESIAN_POINT('Ctrl Pts',(11.0256691663884,852.234683649601,135.079207243204));
#66081=CARTESIAN_POINT('Ctrl Pts',(11.0219278432404,852.355573996643,135.128693372122));
#66082=CARTESIAN_POINT('Ctrl Pts',(11.0328118469896,852.415992694243,135.15254086669));
#66083=CARTESIAN_POINT('Ctrl Pts',(11.0789341059454,852.530195117028,135.195700871793));
#66084=CARTESIAN_POINT('Ctrl Pts',(11.1137266837724,852.582852009129,135.214584939382));
#66085=CARTESIAN_POINT('Ctrl Pts',(11.2030012436641,852.673469967185,135.244856780591));
#66086=CARTESIAN_POINT('Ctrl Pts',(11.2566637199698,852.710476923002,135.255917874418));
#66087=CARTESIAN_POINT('Ctrl Pts',(11.3759898352345,852.763637145866,135.268732408905));
#66088=CARTESIAN_POINT('Ctrl Pts',(11.4405267510195,852.779181193359,135.270325149122));
#66089=CARTESIAN_POINT('Ctrl Pts',(11.5718381732654,852.786333960206,135.263867260214));
#66090=CARTESIAN_POINT('Ctrl Pts',(11.6373514964259,852.777824259386,135.255863124021));
#66091=CARTESIAN_POINT('Ctrl Pts',(11.7615714398395,852.73722955077,135.231158375251));
#66092=CARTESIAN_POINT('Ctrl Pts',(11.8189055150791,852.705119303221,135.214548792635));
#66093=CARTESIAN_POINT('Ctrl Pts',(11.9157287467566,852.621732954991,135.175170316205));
#66094=CARTESIAN_POINT('Ctrl Pts',(11.9543928728251,852.571416662468,135.152832569033));
#66095=CARTESIAN_POINT('Ctrl Pts',(12.0079060009128,852.459321242942,135.105288065939));
#66096=CARTESIAN_POINT('Ctrl Pts',(12.0223015627294,852.398693476501,135.08055888157));
#66097=CARTESIAN_POINT('Ctrl Pts',(12.0247151338561,852.275147512267,135.031782572753));
#66098=CARTESIAN_POINT('Ctrl Pts',(12.0126797276385,852.213469882361,135.008222185968));
#66099=CARTESIAN_POINT('Ctrl Pts',(11.9634580546866,852.097571840821,134.965378255875));
#66100=CARTESIAN_POINT('Ctrl Pts',(11.9267343509588,852.044534466716,134.946531893362));
#66101=CARTESIAN_POINT('Ctrl Pts',(11.8334642424212,851.954654908216,134.916244729229));
#66102=CARTESIAN_POINT('Ctrl Pts',(11.7778816295094,851.91870038575,134.905102603088));
#66103=CARTESIAN_POINT('Ctrl Pts',(11.6553877837247,851.868885618794,134.8922340432));
#66104=CARTESIAN_POINT('Ctrl Pts',(11.5897214869269,851.855493045995,134.890627702924));
#66105=CARTESIAN_POINT('Ctrl Pts',(11.5234307913646,851.854317302887,134.894017809227));
#66106=CARTESIAN_POINT('Origin',(5.07102541057036,853.43446399037,123.944135806152));
#66107=CARTESIAN_POINT('',(5.07102541057036,848.771152051143,134.293326883657));
#66108=CARTESIAN_POINT('',(5.07102541052708,850.506278886623,135.074204134598));
#66109=CARTESIAN_POINT('Ctrl Pts',(5.07102541057036,848.771152051143,134.293326883657));
#66110=CARTESIAN_POINT('Ctrl Pts',(5.0699582962581,848.771099914276,134.293474398867));
#66111=CARTESIAN_POINT('Ctrl Pts',(5.06889111868239,848.7710494163,134.293622683548));
#66112=CARTESIAN_POINT('Ctrl Pts',(4.94165327412791,848.765224438062,134.311393163062));
#66113=CARTESIAN_POINT('Ctrl Pts',(4.81710114981319,848.782464983614,134.33943824526));
#66114=CARTESIAN_POINT('Ctrl Pts',(4.58394097750445,848.860926766562,134.41368984665));
#66115=CARTESIAN_POINT('Ctrl Pts',(4.47773994242997,848.922069921972,134.459475719585));
#66116=CARTESIAN_POINT('Ctrl Pts',(4.30295154857553,849.07816947996,134.56079191155));
#66117=CARTESIAN_POINT('Ctrl Pts',(4.23491862264972,849.170822301041,134.615145628139));
#66118=CARTESIAN_POINT('Ctrl Pts',(4.14429105857174,849.375464639912,134.72504769072));
#66119=CARTESIAN_POINT('Ctrl Pts',(4.12168011923636,849.48521408266,134.77955337809));
#66120=CARTESIAN_POINT('Ctrl Pts',(4.12429471942459,849.70841290292,134.881590968212));
#66121=CARTESIAN_POINT('Ctrl Pts',(4.14893812838373,849.819580954806,134.928171807675));
#66122=CARTESIAN_POINT('Ctrl Pts',(4.24291571131902,850.03073743613,135.007798329004));
#66123=CARTESIAN_POINT('Ctrl Pts',(4.31142571246568,850.128392921735,135.039921708603));
#66124=CARTESIAN_POINT('Ctrl Pts',(4.48513736682712,850.298206835272,135.085630847371));
#66125=CARTESIAN_POINT('Ctrl Pts',(4.58907400449951,850.368022432266,135.098381587636));
#66126=CARTESIAN_POINT('Ctrl Pts',(4.81954792508221,850.469430147485,135.102577107638));
#66127=CARTESIAN_POINT('Ctrl Pts',(4.94413173609949,850.499233941933,135.093579592117));
#66128=CARTESIAN_POINT('Ctrl Pts',(5.06962996552313,850.506202346397,135.074417614505));
#66129=CARTESIAN_POINT('Ctrl Pts',(5.07009513240186,850.506228175216,135.074346589461));
#66130=CARTESIAN_POINT('Ctrl Pts',(5.07056028084347,850.506253688607,135.074275429459));
#66131=CARTESIAN_POINT('Ctrl Pts',(5.0710254104838,850.506278886623,135.074204134598));
#66132=CARTESIAN_POINT('',(5.07102541057036,851.188478953102,133.143998259299));
#66133=CARTESIAN_POINT('',(5.07102541057036,854.328360162989,124.260068959288));
#66134=CARTESIAN_POINT('Ctrl Pts',(4.23512898156332,850.693189667638,133.042771344765));
#66135=CARTESIAN_POINT('Ctrl Pts',(4.29099867867875,850.791613551705,133.07755767565));
#66136=CARTESIAN_POINT('Ctrl Pts',(4.36588968533656,850.88028614259,133.105549792614));
#66137=CARTESIAN_POINT('Ctrl Pts',(4.55086908900839,851.033175176208,133.146308005615));
#66138=CARTESIAN_POINT('Ctrl Pts',(4.66077472278794,851.094171929925,133.157720959576));
#66139=CARTESIAN_POINT('Ctrl Pts',(4.89556685899703,851.17371147003,133.160627109839));
#66140=CARTESIAN_POINT('Ctrl Pts',(5.01796167694315,851.192219771856,133.152439031636));
#66141=CARTESIAN_POINT('Ctrl Pts',(5.26321810607648,851.185574483663,133.11785628134));
#66142=CARTESIAN_POINT('Ctrl Pts',(5.38381514613692,851.159776035689,133.091493142985));
#66143=CARTESIAN_POINT('Ctrl Pts',(5.60673618965806,851.065687386839,133.023646760527));
#66144=CARTESIAN_POINT('Ctrl Pts',(5.70675422284467,850.997747268953,132.982609837993));
#66145=CARTESIAN_POINT('Ctrl Pts',(5.87099048308924,850.828202958375,132.891231943048));
#66146=CARTESIAN_POINT('Ctrl Pts',(5.93354165355819,850.728152743558,132.841744379948));
#66147=CARTESIAN_POINT('Ctrl Pts',(6.00998878810946,850.51390100233,132.742867659224));
#66148=CARTESIAN_POINT('Ctrl Pts',(6.02511120824281,850.402461808752,132.694472602674));
#66149=CARTESIAN_POINT('Ctrl Pts',(6.009090654539,850.182142107766,132.604137937494));
#66150=CARTESIAN_POINT('Ctrl Pts',(5.97960229472973,850.075276882214,132.562844301108));
#66151=CARTESIAN_POINT('Ctrl Pts',(5.87998340379096,849.874817826804,132.490389855698));
#66152=CARTESIAN_POINT('Ctrl Pts',(5.81054255648633,849.783142082205,132.459951248518));
#66153=CARTESIAN_POINT('Ctrl Pts',(5.63763269257999,849.624754818309,132.413423289628));
#66154=CARTESIAN_POINT('Ctrl Pts',(5.53497596315341,849.560286324222,132.398184262539));
#66155=CARTESIAN_POINT('Ctrl Pts',(5.30485543671926,849.467114843493,132.385820586694));
#66156=CARTESIAN_POINT('Ctrl Pts',(5.17875512652277,849.441429377766,132.389824260633));
#66157=CARTESIAN_POINT('Ctrl Pts',(4.9282581978398,849.43683076242,132.417862061688));
#66158=CARTESIAN_POINT('Ctrl Pts',(4.8062516798978,849.456914301006,132.441181502153));
#66159=CARTESIAN_POINT('Ctrl Pts',(4.57800342857582,849.53978619875,132.504591540214));
#66160=CARTESIAN_POINT('Ctrl Pts',(4.47412434763127,849.602391454363,132.544321421763));
#66161=CARTESIAN_POINT('Ctrl Pts',(4.2996921601432,849.762887981157,132.635126752235));
#66162=CARTESIAN_POINT('Ctrl Pts',(4.23109740276462,849.859580192221,132.685440117008));
#66163=CARTESIAN_POINT('Ctrl Pts',(4.14507592259544,850.062846652263,132.783904166084));
#66164=CARTESIAN_POINT('Ctrl Pts',(4.12375507032402,850.165733648502,132.830947687406));
#66165=CARTESIAN_POINT('Ctrl Pts',(4.1221327608723,850.380762396911,132.923599492544));
#66166=CARTESIAN_POINT('Ctrl Pts',(4.14396681404573,850.491099136668,132.968144643274));
#66167=CARTESIAN_POINT('Ctrl Pts',(4.20124222567194,850.629019808441,133.019746227074));
#66168=CARTESIAN_POINT('Ctrl Pts',(4.21716604956892,850.661544936641,133.031587026104));
#66169=CARTESIAN_POINT('Ctrl Pts',(4.23512898156325,850.693189667638,133.042771344765));
#66170=CARTESIAN_POINT('Ctrl Pts',(5.07102541048378,850.506278886623,135.074204134598));
#66171=CARTESIAN_POINT('Ctrl Pts',(5.19423078066677,850.512953436295,135.055319271343));
#66172=CARTESIAN_POINT('Ctrl Pts',(5.31611901355964,850.497498731957,135.026985023423));
#66173=CARTESIAN_POINT('Ctrl Pts',(5.54705036221113,850.423151972727,134.953923209424));
#66174=CARTESIAN_POINT('Ctrl Pts',(5.65355205997801,850.363656200473,134.90939339752));
#66175=CARTESIAN_POINT('Ctrl Pts',(5.83121312845475,850.209017353198,134.811222468209));
#66176=CARTESIAN_POINT('Ctrl Pts',(5.90123008407851,850.115815905014,134.75861491801));
#66177=CARTESIAN_POINT('Ctrl Pts',(5.99585789558844,849.90787126927,134.651654591827));
#66178=CARTESIAN_POINT('Ctrl Pts',(6.01988600047576,849.795357887299,134.598362087097));
#66179=CARTESIAN_POINT('Ctrl Pts',(6.01831170401472,849.567711146755,134.498395590651));
#66180=CARTESIAN_POINT('Ctrl Pts',(5.99371779675477,849.454975907878,134.452607245757));
#66181=CARTESIAN_POINT('Ctrl Pts',(5.89885078072835,849.241046241887,134.372903188918));
#66182=CARTESIAN_POINT('Ctrl Pts',(5.82913869410888,849.1422252107,134.339941444606));
#66183=CARTESIAN_POINT('Ctrl Pts',(5.65278354333737,848.972221136584,134.291760233714));
#66184=CARTESIAN_POINT('Ctrl Pts',(5.54766206537191,848.903127388101,134.277239294612));
#66185=CARTESIAN_POINT('Ctrl Pts',(5.31736144834189,848.805210438417,134.269484061337));
#66186=CARTESIAN_POINT('Ctrl Pts',(5.19461728992305,848.777190479516,134.276241851719));
#66187=CARTESIAN_POINT('Ctrl Pts',(5.07102541057036,848.771152051143,134.293326883657));
#66188=CARTESIAN_POINT('Origin',(5.07102541057036,853.43446399037,123.944135806152));
#66189=CARTESIAN_POINT('',(5.07102541057036,851.771047358864,130.15103104964));
#66190=CARTESIAN_POINT('Origin',(5.07102541057036,851.299625128255,129.984414482373));
#66191=CARTESIAN_POINT('',(5.07102541057048,850.097096174575,134.887281556846));
#66192=CARTESIAN_POINT('',(5.07102541057036,853.905886220979,124.110752373419));
#66193=CARTESIAN_POINT('Ctrl Pts',(5.0706266353229,849.181994456725,134.475554028475));
#66194=CARTESIAN_POINT('Ctrl Pts',(5.00538071894428,849.178772050676,134.484827609953));
#66195=CARTESIAN_POINT('Ctrl Pts',(4.94089660084872,849.187245813263,134.49932329689));
#66196=CARTESIAN_POINT('Ctrl Pts',(4.81872050007149,849.226996978315,134.537709047521));
#66197=CARTESIAN_POINT('Ctrl Pts',(4.76242595381707,849.258633076072,134.561535719969));
#66198=CARTESIAN_POINT('Ctrl Pts',(4.66924894253178,849.340049433716,134.614327125243));
#66199=CARTESIAN_POINT('Ctrl Pts',(4.63273407721486,849.388658790337,134.642690753026));
#66200=CARTESIAN_POINT('Ctrl Pts',(4.58357471445859,849.496406215602,134.700180626491));
#66201=CARTESIAN_POINT('Ctrl Pts',(4.570969969903,849.5543586624,134.728755879377));
#66202=CARTESIAN_POINT('Ctrl Pts',(4.57108058031632,849.672413088542,134.782444381829));
#66203=CARTESIAN_POINT('Ctrl Pts',(4.58350979218662,849.731306290975,134.807055202564));
#66204=CARTESIAN_POINT('Ctrl Pts',(4.63206290571102,849.843190482258,134.849348000012));
#66205=CARTESIAN_POINT('Ctrl Pts',(4.6677306976392,849.89497121084,134.866559374063));
#66206=CARTESIAN_POINT('Ctrl Pts',(4.7584701484939,849.985054915219,134.891392852513));
#66207=CARTESIAN_POINT('Ctrl Pts',(4.81284882588072,850.022167910333,134.898598615293));
#66208=CARTESIAN_POINT('Ctrl Pts',(4.93389009301996,850.076473238899,134.901886229569));
#66209=CARTESIAN_POINT('Ctrl Pts',(4.99954868223937,850.092655060561,134.897692010075));
#66210=CARTESIAN_POINT('Ctrl Pts',(5.13320829335458,850.101006435591,134.878245413705));
#66211=CARTESIAN_POINT('Ctrl Pts',(5.19995559405832,850.092681927241,134.862994352188));
#66212=CARTESIAN_POINT('Ctrl Pts',(5.32383274316292,850.052242247041,134.823711597774));
#66213=CARTESIAN_POINT('Ctrl Pts',(5.37990540190694,850.020624931118,134.800083176872));
#66214=CARTESIAN_POINT('Ctrl Pts',(5.47351575204461,849.938512202664,134.747726210205));
#66215=CARTESIAN_POINT('Ctrl Pts',(5.51036094006763,849.888945988342,134.71952470307));
#66216=CARTESIAN_POINT('Ctrl Pts',(5.55928135851067,849.779525665693,134.662740083004));
#66217=CARTESIAN_POINT('Ctrl Pts',(5.57152417748079,849.721020436217,134.634723276507));
#66218=CARTESIAN_POINT('Ctrl Pts',(5.57050061265669,849.602042816117,134.581957801238));
#66219=CARTESIAN_POINT('Ctrl Pts',(5.5574911359873,849.542792490688,134.557707958326));
#66220=CARTESIAN_POINT('Ctrl Pts',(5.50772101855733,849.430814536929,134.515872560121));
#66221=CARTESIAN_POINT('Ctrl Pts',(5.47148092102027,849.379252328022,134.498721208165));
#66222=CARTESIAN_POINT('Ctrl Pts',(5.37954247592785,849.289859054838,134.473632059099));
#66223=CARTESIAN_POINT('Ctrl Pts',(5.3244836160405,849.253247527649,134.466136803691));
#66224=CARTESIAN_POINT('Ctrl Pts',(5.20257928156474,849.200519585333,134.462286635868));
#66225=CARTESIAN_POINT('Ctrl Pts',(5.13683475959023,849.185264384898,134.466143685743));
#66226=CARTESIAN_POINT('Ctrl Pts',(5.0706266353229,849.181994456725,134.475554028475));
#66227=CARTESIAN_POINT('Origin',(18.2997627645019,863.466134352395,127.489667542144));
#66228=CARTESIAN_POINT('',(18.2997627645018,858.895801196787,137.355748312979));
#66229=CARTESIAN_POINT('',(18.2997627644989,860.785555989654,138.139198981994));
#66230=CARTESIAN_POINT('Ctrl Pts',(18.2997627645018,858.895801196787,137.355748312979));
#66231=CARTESIAN_POINT('Ctrl Pts',(18.2983068136417,858.895782959237,137.355799914008));
#66232=CARTESIAN_POINT('Ctrl Pts',(18.2968507168663,858.895767600436,137.355852711893));
#66233=CARTESIAN_POINT('Ctrl Pts',(18.1608616249801,858.89460231778,137.360895047597));
#66234=CARTESIAN_POINT('Ctrl Pts',(18.0278281919414,858.918050978786,137.37601610752));
#66235=CARTESIAN_POINT('Ctrl Pts',(17.7786029347692,859.011612283662,137.425711003125));
#66236=CARTESIAN_POINT('Ctrl Pts',(17.6651217807427,859.081309034422,137.460017191673));
#66237=CARTESIAN_POINT('Ctrl Pts',(17.4764533886176,859.256319335015,137.542854104322));
#66238=CARTESIAN_POINT('Ctrl Pts',(17.4025240193924,859.359427527541,137.590376644922));
#66239=CARTESIAN_POINT('Ctrl Pts',(17.3026195959521,859.586115931001,137.692365692213));
#66240=CARTESIAN_POINT('Ctrl Pts',(17.277421515798,859.707516946354,137.745845666951));
#66241=CARTESIAN_POINT('Ctrl Pts',(17.2793359665033,859.952765012574,137.851018357706));
#66242=CARTESIAN_POINT('Ctrl Pts',(17.3061982152061,860.074293963003,137.901713187695));
#66243=CARTESIAN_POINT('Ctrl Pts',(17.4088728257215,860.302144253813,137.993172112431));
#66244=CARTESIAN_POINT('Ctrl Pts',(17.4836394713146,860.406259319673,138.033042761101));
#66245=CARTESIAN_POINT('Ctrl Pts',(17.672197256176,860.58372504773,138.096468904178));
#66246=CARTESIAN_POINT('Ctrl Pts',(17.7842656183664,860.655152976418,138.119312482594));
#66247=CARTESIAN_POINT('Ctrl Pts',(18.0316171493468,860.755226628336,138.144865426948));
#66248=CARTESIAN_POINT('Ctrl Pts',(18.1645680107954,860.782589038475,138.147197677704));
#66249=CARTESIAN_POINT('Ctrl Pts',(18.2987622212797,860.785534481657,138.139258365774));
#66250=CARTESIAN_POINT('Ctrl Pts',(18.2990957438871,860.785541802181,138.139238633626));
#66251=CARTESIAN_POINT('Ctrl Pts',(18.2994292583314,860.785548971507,138.139218839026));
#66252=CARTESIAN_POINT('Ctrl Pts',(18.299762764496,860.785555989654,138.139198981994));
#66253=CARTESIAN_POINT('',(18.2997627661012,861.429330672107,136.317713269084));
#66254=CARTESIAN_POINT('',(18.2997627645019,864.429163492638,127.830034625211));
#66255=CARTESIAN_POINT('Ctrl Pts',(17.594519871266,861.155236423289,136.24531767004));
#66256=CARTESIAN_POINT('Ctrl Pts',(17.6908584649292,861.241936525388,136.275960419694));
#66257=CARTESIAN_POINT('Ctrl Pts',(17.804230417976,861.310744784423,136.297962676467));
#66258=CARTESIAN_POINT('Ctrl Pts',(18.0522330816735,861.404834888075,136.322365677225));
#66259=CARTESIAN_POINT('Ctrl Pts',(18.1844450118424,861.429195618522,136.324533004031));
#66260=CARTESIAN_POINT('Ctrl Pts',(18.4509615187008,861.429833981708,136.308906144829));
#66261=CARTESIAN_POINT('Ctrl Pts',(18.5827134042018,861.405891327604,136.291182167775));
#66262=CARTESIAN_POINT('Ctrl Pts',(18.8282428242795,861.311983164994,136.238227127449));
#66263=CARTESIAN_POINT('Ctrl Pts',(18.9396016131448,861.242709348448,136.203430487723));
#66264=CARTESIAN_POINT('Ctrl Pts',(19.1263503268062,861.067500157729,136.121409806725));
#66265=CARTESIAN_POINT('Ctrl Pts',(19.1999155927994,860.963200797497,136.074957713108));
#66266=CARTESIAN_POINT('Ctrl Pts',(19.2983522032081,860.734334643123,135.976859333337));
#66267=CARTESIAN_POINT('Ctrl Pts',(19.3227392680653,860.612149576957,135.92619475046));
#66268=CARTESIAN_POINT('Ctrl Pts',(19.3194256122495,860.363464891823,135.825896766366));
#66269=CARTESIAN_POINT('Ctrl Pts',(19.2910890688764,860.239392928892,135.777267796106));
#66270=CARTESIAN_POINT('Ctrl Pts',(19.1841695557557,860.007676446591,135.688880454628));
#66271=CARTESIAN_POINT('Ctrl Pts',(19.1065726266327,859.902371942357,135.65001080561));
#66272=CARTESIAN_POINT('Ctrl Pts',(18.9131363483052,859.726241093662,135.587664032789));
#66273=CARTESIAN_POINT('Ctrl Pts',(18.7995761439172,859.656806388201,135.564648202491));
#66274=CARTESIAN_POINT('Ctrl Pts',(18.5508574843179,859.562188652378,135.537388126793));
#66275=CARTESIAN_POINT('Ctrl Pts',(18.4181435363346,859.537893047305,135.533402136904));
#66276=CARTESIAN_POINT('Ctrl Pts',(18.1514542733364,859.537838183702,135.545458805947));
#66277=CARTESIAN_POINT('Ctrl Pts',(18.0200582254551,859.561912374016,135.561326071294));
#66278=CARTESIAN_POINT('Ctrl Pts',(17.7744547997471,859.655707338899,135.61147947879));
#66279=CARTESIAN_POINT('Ctrl Pts',(17.6627817243068,859.724898754097,135.645438992041));
#66280=CARTESIAN_POINT('Ctrl Pts',(17.4743227654491,859.900473460484,135.727624686544));
#66281=CARTESIAN_POINT('Ctrl Pts',(17.3998089472424,860.005571326227,135.775211380791));
#66282=CARTESIAN_POINT('Ctrl Pts',(17.3005864785872,860.235853052164,135.876612380104));
#66283=CARTESIAN_POINT('Ctrl Pts',(17.2762910227212,860.358611822648,135.929379828543));
#66284=CARTESIAN_POINT('Ctrl Pts',(17.2806895581755,860.606550772501,136.033154213921));
#66285=CARTESIAN_POINT('Ctrl Pts',(17.3092756830069,860.729331960926,136.083151296631));
#66286=CARTESIAN_POINT('Ctrl Pts',(17.3896103528833,860.901813882126,136.150977336745));
#66287=CARTESIAN_POINT('Ctrl Pts',(17.4226308325239,860.957117894915,136.172290117947));
#66288=CARTESIAN_POINT('Ctrl Pts',(17.5003620732768,861.06172047604,136.211656132999));
#66289=CARTESIAN_POINT('Ctrl Pts',(17.5450005799048,861.110671442074,136.229566897785));
#66290=CARTESIAN_POINT('Ctrl Pts',(17.5945198712659,861.155236423289,136.24531767004));
#66291=CARTESIAN_POINT('Ctrl Pts',(18.299762764496,860.785555989654,138.139198981994));
#66292=CARTESIAN_POINT('Ctrl Pts',(18.4310515283573,860.788318768667,138.131382019577));
#66293=CARTESIAN_POINT('Ctrl Pts',(18.5610575008464,860.767652691017,138.11389506776));
#66294=CARTESIAN_POINT('Ctrl Pts',(18.8072939520139,860.680553108331,138.061531489626));
#66295=CARTESIAN_POINT('Ctrl Pts',(18.9207645229621,860.613820608303,138.026744860966));
#66296=CARTESIAN_POINT('Ctrl Pts',(19.1134734904683,860.441564281237,137.944467023966));
#66297=CARTESIAN_POINT('Ctrl Pts',(19.1903967296927,860.337278540976,137.897641488792));
#66298=CARTESIAN_POINT('Ctrl Pts',(19.2944244219691,860.107094203539,137.798995600584));
#66299=CARTESIAN_POINT('Ctrl Pts',(19.3211066916547,859.983737438504,137.748200676581));
#66300=CARTESIAN_POINT('Ctrl Pts',(19.3212349898297,859.733815019667,137.648372605662));
#66301=CARTESIAN_POINT('Ctrl Pts',(19.2948235226952,859.609730037168,137.600301655224));
#66302=CARTESIAN_POINT('Ctrl Pts',(19.1918492603882,859.377156910803,137.512381797694));
#66303=CARTESIAN_POINT('Ctrl Pts',(19.116165062299,859.27102093137,137.47341188137));
#66304=CARTESIAN_POINT('Ctrl Pts',(18.9252420327866,859.091752276658,137.409732445018));
#66305=CARTESIAN_POINT('Ctrl Pts',(18.8118777132635,859.020399903431,137.385654923748));
#66306=CARTESIAN_POINT('Ctrl Pts',(18.5641974706985,858.923091316913,137.356286466893));
#66307=CARTESIAN_POINT('Ctrl Pts',(18.4325874854965,858.897464987428,137.351040810548));
#66308=CARTESIAN_POINT('Ctrl Pts',(18.2997627645018,858.895801196787,137.355748312979));
#66309=CARTESIAN_POINT('Origin',(18.2997627645019,863.466134352395,127.489667542144));
#66310=CARTESIAN_POINT('',(18.2997627645019,861.802717720889,133.696562785632));
#66311=CARTESIAN_POINT('Origin',(18.2997627645019,861.33129549028,133.529946218365));
#66312=CARTESIAN_POINT('',(18.299762764502,860.305153003216,137.933748266442));
#66313=CARTESIAN_POINT('',(18.2997627645019,863.937556583004,127.656284109411));
#66314=CARTESIAN_POINT('Ctrl Pts',(18.29939398446,859.38006602879,137.550272793039));
#66315=CARTESIAN_POINT('Ctrl Pts',(18.2379737606721,859.379200950101,137.55285637696));
#66316=CARTESIAN_POINT('Ctrl Pts',(18.1771136100427,859.38881406725,137.55975239348));
#66317=CARTESIAN_POINT('Ctrl Pts',(18.0575828896044,859.429646471273,137.582550689604));
#66318=CARTESIAN_POINT('Ctrl Pts',(18.00076816786,859.462274904145,137.598964230339));
#66319=CARTESIAN_POINT('Ctrl Pts',(17.9055516740868,859.545601002131,137.63864787193));
#66320=CARTESIAN_POINT('Ctrl Pts',(17.8677591905645,859.595188064968,137.661418479812));
#66321=CARTESIAN_POINT('Ctrl Pts',(17.8153741855982,859.705128586251,137.710432519616));
#66322=CARTESIAN_POINT('Ctrl Pts',(17.8012093834401,859.764415303675,137.736201186751));
#66323=CARTESIAN_POINT('Ctrl Pts',(17.7985313307441,859.884894677905,137.787164297783));
#66324=CARTESIAN_POINT('Ctrl Pts',(17.809949935042,859.944934259786,137.811871862339));
#66325=CARTESIAN_POINT('Ctrl Pts',(17.8570605234403,860.058029050945,137.856847222995));
#66326=CARTESIAN_POINT('Ctrl Pts',(17.8922619245073,860.109992517185,137.8766799161));
#66327=CARTESIAN_POINT('Ctrl Pts',(17.9821682557319,860.199082414306,137.908779616291));
#66328=CARTESIAN_POINT('Ctrl Pts',(18.0360273313281,860.235287778738,137.920708924167));
#66329=CARTESIAN_POINT('Ctrl Pts',(18.1555962784103,860.286929139148,137.93502439619));
#66330=CARTESIAN_POINT('Ctrl Pts',(18.2201700895372,860.301758691313,137.937228091227));
#66331=CARTESIAN_POINT('Ctrl Pts',(18.3514611526987,860.307659280882,137.931613387731));
#66332=CARTESIAN_POINT('Ctrl Pts',(18.4169046345712,860.298592812182,137.923820301848));
#66333=CARTESIAN_POINT('Ctrl Pts',(18.5397083677385,860.257453422974,137.899351328351));
#66334=CARTESIAN_POINT('Ctrl Pts',(18.595890064477,860.22576078684,137.882907870571));
#66335=CARTESIAN_POINT('Ctrl Pts',(18.6921251876924,860.14308502739,137.843265089781));
#66336=CARTESIAN_POINT('Ctrl Pts',(18.7309491520631,860.092609833795,137.820351574453));
#66337=CARTESIAN_POINT('Ctrl Pts',(18.7844040045152,859.980416734138,137.771490547314));
#66338=CARTESIAN_POINT('Ctrl Pts',(18.7986717946644,859.91988779825,137.746045105218));
#66339=CARTESIAN_POINT('Ctrl Pts',(18.8007306858124,859.796863325834,137.695837304615));
#66340=CARTESIAN_POINT('Ctrl Pts',(18.7885708633062,859.735601727313,137.671569735768));
#66341=CARTESIAN_POINT('Ctrl Pts',(18.7392248793321,859.620606992745,137.627292543392));
#66342=CARTESIAN_POINT('Ctrl Pts',(18.702523066407,859.568034582268,137.60772658718));
#66343=CARTESIAN_POINT('Ctrl Pts',(18.6093398118923,859.478950383452,137.575958450104));
#66344=CARTESIAN_POINT('Ctrl Pts',(18.5537944644497,859.443337588619,137.564076699109));
#66345=CARTESIAN_POINT('Ctrl Pts',(18.431346935512,859.394122374484,137.549769252772));
#66346=CARTESIAN_POINT('Ctrl Pts',(18.3656820900001,859.380999669599,137.547484446252));
#66347=CARTESIAN_POINT('Ctrl Pts',(18.29939398446,859.38006602879,137.550272793039));
#66348=CARTESIAN_POINT('Origin',(11.4353582469288,862.278752775433,127.070006716785));
#66349=CARTESIAN_POINT('',(11.4353582469287,857.622828056485,137.398296512269));
#66350=CARTESIAN_POINT('',(11.4353582469181,859.338553021224,138.234069103648));
#66351=CARTESIAN_POINT('Ctrl Pts',(11.4353582469287,857.622828056485,137.398296512269));
#66352=CARTESIAN_POINT('Ctrl Pts',(11.4320865847077,857.62269184695,137.398681901332));
#66353=CARTESIAN_POINT('Ctrl Pts',(11.4288143447741,857.622570916339,137.39907488024));
#66354=CARTESIAN_POINT('Ctrl Pts',(11.3000083658543,857.618413477821,137.414840308951));
#66355=CARTESIAN_POINT('Ctrl Pts',(11.1763214765735,857.636941059338,137.441069094707));
#66356=CARTESIAN_POINT('Ctrl Pts',(10.9451375843786,857.716774500484,137.512851098856));
#66357=CARTESIAN_POINT('Ctrl Pts',(10.8400642756321,857.777921112359,137.557999546846));
#66358=CARTESIAN_POINT('Ctrl Pts',(10.6656844460716,857.933799732246,137.660417061792));
#66359=CARTESIAN_POINT('Ctrl Pts',(10.5975262436369,858.026820199112,137.716661029169));
#66360=CARTESIAN_POINT('Ctrl Pts',(10.5072882989536,858.231586562797,137.831998211912));
#66361=CARTESIAN_POINT('Ctrl Pts',(10.4852163453759,858.341202487111,137.890013046486));
#66362=CARTESIAN_POINT('Ctrl Pts',(10.4895943608974,858.562777705946,137.999770984508));
#66363=CARTESIAN_POINT('Ctrl Pts',(10.5151728975665,858.672574961164,138.050559385957));
#66364=CARTESIAN_POINT('Ctrl Pts',(10.6108366295515,858.879630696045,138.138605941696));
#66365=CARTESIAN_POINT('Ctrl Pts',(10.6797107821902,858.974788226131,138.175003641196));
#66366=CARTESIAN_POINT('Ctrl Pts',(10.853433514803,859.139375609029,138.228935249572));
#66367=CARTESIAN_POINT('Ctrl Pts',(10.9567842004717,859.206682240259,138.24565223094));
#66368=CARTESIAN_POINT('Ctrl Pts',(11.1859684721632,859.304118626678,138.256987142537));
#66369=CARTESIAN_POINT('Ctrl Pts',(11.309772514178,859.332426008226,138.251037788143));
#66370=CARTESIAN_POINT('Ctrl Pts',(11.434431606882,859.338508219923,138.234194504867));
#66371=CARTESIAN_POINT('Ctrl Pts',(11.4347404960019,859.338523290858,138.234152769388));
#66372=CARTESIAN_POINT('Ctrl Pts',(11.4350493760453,859.338538224605,138.234110968965));
#66373=CARTESIAN_POINT('Ctrl Pts',(11.4353582469074,859.338553021224,138.234069103648));
#66374=CARTESIAN_POINT('',(11.4353582469288,860.025278981789,136.291057736552));
#66375=CARTESIAN_POINT('',(11.4353582469288,863.172648948052,127.385939869922));
#66376=CARTESIAN_POINT('Ctrl Pts',(10.7107419313788,859.692120499991,136.223297987356));
#66377=CARTESIAN_POINT('Ctrl Pts',(10.7870947203183,859.777441539487,136.253453329623));
#66378=CARTESIAN_POINT('Ctrl Pts',(10.879670903324,859.849518643311,136.275580039938));
#66379=CARTESIAN_POINT('Ctrl Pts',(11.0934025076228,859.962896633673,136.302373713363));
#66380=CARTESIAN_POINT('Ctrl Pts',(11.2136542592252,860.001085493384,136.305725585857));
#66381=CARTESIAN_POINT('Ctrl Pts',(11.4591089786043,860.03303403674,136.291811467588));
#66382=CARTESIAN_POINT('Ctrl Pts',(11.5818900335077,860.027246158317,136.275036297202));
#66383=CARTESIAN_POINT('Ctrl Pts',(11.8180883571915,859.972890174448,136.223590972723));
#66384=CARTESIAN_POINT('Ctrl Pts',(11.9291663154482,859.924133441659,136.189113599701));
#66385=CARTESIAN_POINT('Ctrl Pts',(12.1240713480493,859.788639504677,136.106633187435));
#66386=CARTESIAN_POINT('Ctrl Pts',(12.2057423918307,859.702694554128,136.05923274783));
#66387=CARTESIAN_POINT('Ctrl Pts',(12.3268232575814,859.504876187704,135.957861844871));
#66388=CARTESIAN_POINT('Ctrl Pts',(12.3649662027356,859.394847493541,135.904847549541));
#66389=CARTESIAN_POINT('Ctrl Pts',(12.3908928787125,859.170450820332,135.802385266591));
#66390=CARTESIAN_POINT('Ctrl Pts',(12.3804866345953,859.058544268114,135.753825029685));
#66391=CARTESIAN_POINT('Ctrl Pts',(12.3153685905864,858.84626515437,135.666332180096));
#66392=CARTESIAN_POINT('Ctrl Pts',(12.2627150548227,858.747539939813,135.62791549902));
#66393=CARTESIAN_POINT('Ctrl Pts',(12.1209575445399,858.571000548618,135.563915072285));
#66394=CARTESIAN_POINT('Ctrl Pts',(12.0329542181142,858.494927040812,135.538990823503));
#66395=CARTESIAN_POINT('Ctrl Pts',(11.8295508502949,858.373831268946,135.505642939685));
#66396=CARTESIAN_POINT('Ctrl Pts',(11.7154439553601,858.330843388052,135.497995888114));
#66397=CARTESIAN_POINT('Ctrl Pts',(11.4712312662008,858.284676880409,135.50224536021));
#66398=CARTESIAN_POINT('Ctrl Pts',(11.3431288567371,858.284182127883,135.515152284544));
#66399=CARTESIAN_POINT('Ctrl Pts',(11.0991469725864,858.328584852785,135.560508817244));
#66400=CARTESIAN_POINT('Ctrl Pts',(10.9853591757403,858.372034887868,135.592086768196));
#66401=CARTESIAN_POINT('Ctrl Pts',(10.7827371824602,858.497604711005,135.670587697811));
#66402=CARTESIAN_POINT('Ctrl Pts',(10.6961531238308,858.579084282088,135.716988401076));
#66403=CARTESIAN_POINT('Ctrl Pts',(10.5632858448346,858.77003324754,135.818556653753));
#66404=CARTESIAN_POINT('Ctrl Pts',(10.5186303296598,858.877948214756,135.872836520283));
#66405=CARTESIAN_POINT('Ctrl Pts',(10.4811565123898,859.093452681628,135.975625895056));
#66406=CARTESIAN_POINT('Ctrl Pts',(10.4837296630386,859.198197517844,136.023326039887));
#66407=CARTESIAN_POINT('Ctrl Pts',(10.530713744444,859.408731053183,136.114389084627));
#66408=CARTESIAN_POINT('Ctrl Pts',(10.5767860287417,859.512338482279,136.156555869277));
#66409=CARTESIAN_POINT('Ctrl Pts',(10.6634213177592,859.635998043111,136.203117093934));
#66410=CARTESIAN_POINT('Ctrl Pts',(10.6861933831297,859.664688526859,136.213602599867));
#66411=CARTESIAN_POINT('Ctrl Pts',(10.7107419313789,859.692120499991,136.223297987356));
#66412=CARTESIAN_POINT('Ctrl Pts',(11.4353582469074,859.338553021224,138.234069103648));
#66413=CARTESIAN_POINT('Ctrl Pts',(11.5585407700079,859.344454144118,138.217372561631));
#66414=CARTESIAN_POINT('Ctrl Pts',(11.6802640064212,859.328543777274,138.190361913439));
#66415=CARTESIAN_POINT('Ctrl Pts',(11.9117504582451,859.253850445023,138.117998610973));
#66416=CARTESIAN_POINT('Ctrl Pts',(12.0187722078778,859.194107831381,138.072641106697));
#66417=CARTESIAN_POINT('Ctrl Pts',(12.1968995691043,859.039470178997,137.97125906028));
#66418=CARTESIAN_POINT('Ctrl Pts',(12.2669116858857,858.946467335536,137.916298138233));
#66419=CARTESIAN_POINT('Ctrl Pts',(12.3609585691097,858.739753194833,137.803809423437));
#66420=CARTESIAN_POINT('Ctrl Pts',(12.3846034703439,858.628243661073,137.747373198729));
#66421=CARTESIAN_POINT('Ctrl Pts',(12.3821982225962,858.400942981135,137.639665883526));
#66422=CARTESIAN_POINT('Ctrl Pts',(12.356324383801,858.287491813633,137.589466738589));
#66423=CARTESIAN_POINT('Ctrl Pts',(12.2587335578108,858.076308145489,137.50262605921));
#66424=CARTESIAN_POINT('Ctrl Pts',(12.1890262960479,857.9804447875,137.466591781897));
#66425=CARTESIAN_POINT('Ctrl Pts',(12.012377014696,857.814748789332,137.411662720805));
#66426=CARTESIAN_POINT('Ctrl Pts',(11.9065264991529,857.747340837536,137.393769477282));
#66427=CARTESIAN_POINT('Ctrl Pts',(11.6772701963114,857.653954703855,137.380147881689));
#66428=CARTESIAN_POINT('Ctrl Pts',(11.556711719808,857.627880381267,137.384001545942));
#66429=CARTESIAN_POINT('Ctrl Pts',(11.4353582469287,857.622828056485,137.398296512269));
#66430=CARTESIAN_POINT('Origin',(11.4353582469288,862.278752775433,127.070006716785));
#66431=CARTESIAN_POINT('',(11.4353582469288,860.615336143927,133.276901960274));
#66432=CARTESIAN_POINT('Origin',(11.4353582469288,860.143913913318,133.110285393007));
#66433=CARTESIAN_POINT('',(11.4353582469292,858.934374098609,138.032988884704));
#66434=CARTESIAN_POINT('',(11.4353582469288,862.750175006042,127.236623284052));
#66435=CARTESIAN_POINT('Ctrl Pts',(11.4353409859824,858.029527342834,137.592245655571));
#66436=CARTESIAN_POINT('Ctrl Pts',(11.3714258466797,858.026771612524,137.600049295908));
#66437=CARTESIAN_POINT('Ctrl Pts',(11.3082664140231,858.035126649353,137.613183561539));
#66438=CARTESIAN_POINT('Ctrl Pts',(11.187192726061,858.073771395391,137.649568773904));
#66439=CARTESIAN_POINT('Ctrl Pts',(11.1308368061775,858.104791595968,137.672961899672));
#66440=CARTESIAN_POINT('Ctrl Pts',(11.0357617041929,858.185728686537,137.726636532982));
#66441=CARTESIAN_POINT('Ctrl Pts',(10.9980144608311,858.23503256091,137.756475064446));
#66442=CARTESIAN_POINT('Ctrl Pts',(10.9479256982084,858.343459450832,137.817334264073));
#66443=CARTESIAN_POINT('Ctrl Pts',(10.9352247351614,858.401245751621,137.847742836107));
#66444=CARTESIAN_POINT('Ctrl Pts',(10.9354916676171,858.518457696539,137.905498570289));
#66445=CARTESIAN_POINT('Ctrl Pts',(10.9480429333104,858.57672717557,137.932335231537));
#66446=CARTESIAN_POINT('Ctrl Pts',(10.9968288283811,858.686824604485,137.979127287851));
#66447=CARTESIAN_POINT('Ctrl Pts',(11.0324265036371,858.737547494408,137.998634075903));
#66448=CARTESIAN_POINT('Ctrl Pts',(11.1227658162271,858.825449110991,138.02792509068));
#66449=CARTESIAN_POINT('Ctrl Pts',(11.1766999687752,858.861548400801,138.037302469546));
#66450=CARTESIAN_POINT('Ctrl Pts',(11.2966265781814,858.914238670561,138.04457552041));
#66451=CARTESIAN_POINT('Ctrl Pts',(11.3615468796824,858.92990608801,138.042186163842));
#66452=CARTESIAN_POINT('Ctrl Pts',(11.4946528743705,858.938074061457,138.025654200299));
#66453=CARTESIAN_POINT('Ctrl Pts',(11.5615376947085,858.929791724399,138.011335589564));
#66454=CARTESIAN_POINT('Ctrl Pts',(11.6859232148725,858.889705148093,137.972878399885));
#66455=CARTESIAN_POINT('Ctrl Pts',(11.7423076352131,858.858319303421,137.949115413728));
#66456=CARTESIAN_POINT('Ctrl Pts',(11.8365300611981,858.776912540008,137.895577954623));
#66457=CARTESIAN_POINT('Ctrl Pts',(11.8736705998395,858.727769568308,137.866330839782));
#66458=CARTESIAN_POINT('Ctrl Pts',(11.9236019175578,858.618365478065,137.80622892357));
#66459=CARTESIAN_POINT('Ctrl Pts',(11.9361091204556,858.559230654604,137.775954595012));
#66460=CARTESIAN_POINT('Ctrl Pts',(11.9345598686111,858.440209979897,137.718936907514));
#66461=CARTESIAN_POINT('Ctrl Pts',(11.9212542753335,858.381556985196,137.692672767461));
#66462=CARTESIAN_POINT('Ctrl Pts',(11.8708786532403,858.271201026943,137.646825173002));
#66463=CARTESIAN_POINT('Ctrl Pts',(11.8344621486659,858.220592602821,137.627672546176));
#66464=CARTESIAN_POINT('Ctrl Pts',(11.7427775851303,858.133644866505,137.598827304036));
#66465=CARTESIAN_POINT('Ctrl Pts',(11.6883829066964,858.098287087514,137.589483483378));
#66466=CARTESIAN_POINT('Ctrl Pts',(11.5672638486872,858.047104506123,137.581955024154));
#66467=CARTESIAN_POINT('Ctrl Pts',(11.5015422870096,858.032381642046,137.584162889129));
#66468=CARTESIAN_POINT('Ctrl Pts',(11.4353409859824,858.029527342834,137.592245655571));
#66469=CARTESIAN_POINT('Origin',(26.5871534051988,869.497999037637,129.621532615152));
#66470=CARTESIAN_POINT('',(26.5871534051988,864.929584227576,139.482185650009));
#66471=CARTESIAN_POINT('',(26.5871534051999,866.812688940616,140.284451947729));
#66472=CARTESIAN_POINT('Ctrl Pts',(26.5871534051988,864.929584227576,139.482185650009));
#66473=CARTESIAN_POINT('Ctrl Pts',(26.5841573362241,864.929557222217,139.482262058535));
#66474=CARTESIAN_POINT('Ctrl Pts',(26.5811606574118,864.929542413547,139.482343517111));
#66475=CARTESIAN_POINT('Ctrl Pts',(26.4438450892314,864.929423400893,139.486307239835));
#66476=CARTESIAN_POINT('Ctrl Pts',(26.3111245569331,864.953832371642,139.500264749134));
#66477=CARTESIAN_POINT('Ctrl Pts',(26.0634220090255,865.048778496406,139.547580931716));
#66478=CARTESIAN_POINT('Ctrl Pts',(25.9509992542654,865.118604517996,139.580585753559));
#66479=CARTESIAN_POINT('Ctrl Pts',(25.7631707179859,865.293761695947,139.661567534247));
#66480=CARTESIAN_POINT('Ctrl Pts',(25.6893391335263,865.397164211242,139.708667886131));
#66481=CARTESIAN_POINT('Ctrl Pts',(25.5895898042354,865.624238507318,139.810905030994));
#66482=CARTESIAN_POINT('Ctrl Pts',(25.5645603817579,865.745751975618,139.865063001591));
#66483=CARTESIAN_POINT('Ctrl Pts',(25.5670106198202,865.990684247581,139.972625649828));
#66484=CARTESIAN_POINT('Ctrl Pts',(25.5942373034062,866.111810289127,140.025014472418));
#66485=CARTESIAN_POINT('Ctrl Pts',(25.6976267215419,866.338078488702,140.12047049549));
#66486=CARTESIAN_POINT('Ctrl Pts',(25.772631528245,866.441115147401,140.16264348319));
#66487=CARTESIAN_POINT('Ctrl Pts',(25.9613232969961,866.616044266393,140.230828193134));
#66488=CARTESIAN_POINT('Ctrl Pts',(26.0731963745589,866.686155071173,140.256132466736));
#66489=CARTESIAN_POINT('Ctrl Pts',(26.3199956490675,866.78393271988,140.286298227696));
#66490=CARTESIAN_POINT('Ctrl Pts',(26.452566411568,866.810359909426,140.2907382711));
#66491=CARTESIAN_POINT('Ctrl Pts',(26.5863839149178,866.812675889115,140.284488005616));
#66492=CARTESIAN_POINT('Ctrl Pts',(26.5866404166808,866.812680328392,140.284476025089));
#66493=CARTESIAN_POINT('Ctrl Pts',(26.5868969134595,866.812684678889,140.284464005791));
#66494=CARTESIAN_POINT('Ctrl Pts',(26.587153405201,866.812688940616,140.284451947729));
#66495=CARTESIAN_POINT('',(26.587153406672,867.457684615548,138.459511578372));
#66496=CARTESIAN_POINT('',(26.5871534051988,870.46102817788,129.96189969822));
#66497=CARTESIAN_POINT('Ctrl Pts',(26.0509384417415,867.310125790805,138.420663828409));
#66498=CARTESIAN_POINT('Ctrl Pts',(26.1642905106799,867.376046188621,138.443962327469));
#66499=CARTESIAN_POINT('Ctrl Pts',(26.2901977702864,867.421142608424,138.457584017948));
#66500=CARTESIAN_POINT('Ctrl Pts',(26.5529160266006,867.464621828609,138.464099420027));
#66501=CARTESIAN_POINT('Ctrl Pts',(26.6871643626009,867.462577160429,138.456934185508));
#66502=CARTESIAN_POINT('Ctrl Pts',(26.946899304951,867.411065612132,138.422875783052));
#66503=CARTESIAN_POINT('Ctrl Pts',(27.0698506843585,867.361882642322,138.396231024401));
#66504=CARTESIAN_POINT('Ctrl Pts',(27.2879371444874,867.222031561834,138.327038202379));
#66505=CARTESIAN_POINT('Ctrl Pts',(27.3808720243468,867.132512866614,138.285086337527));
#66506=CARTESIAN_POINT('Ctrl Pts',(27.5235112115396,866.924662340849,138.191529104276));
#66507=CARTESIAN_POINT('Ctrl Pts',(27.5718049213144,866.808287128267,138.140808995843));
#66508=CARTESIAN_POINT('Ctrl Pts',(27.616429636366,866.565244033439,138.037700005626));
#66509=CARTESIAN_POINT('Ctrl Pts',(27.6128218464575,866.440999804584,137.986307644981));
#66510=CARTESIAN_POINT('Ctrl Pts',(27.5538823927995,866.198484212482,137.888190027101));
#66511=CARTESIAN_POINT('Ctrl Pts',(27.4984742801511,866.082711089212,137.842494147576));
#66512=CARTESIAN_POINT('Ctrl Pts',(27.342344460985,865.877061992407,137.763319902144));
#66513=CARTESIAN_POINT('Ctrl Pts',(27.2431075305264,865.78928118362,137.730643720026));
#66514=CARTESIAN_POINT('Ctrl Pts',(27.0150520774923,865.654918878296,137.683059363707));
#66515=CARTESIAN_POINT('Ctrl Pts',(26.8887676555259,865.609252042839,137.668443902873));
#66516=CARTESIAN_POINT('Ctrl Pts',(26.6250476717488,865.565415411623,137.659131587765));
#66517=CARTESIAN_POINT('Ctrl Pts',(26.4901950520978,865.567634836273,137.66451690654));
#66518=CARTESIAN_POINT('Ctrl Pts',(26.2301581575115,865.619776926303,137.695021745125));
#66519=CARTESIAN_POINT('Ctrl Pts',(26.1074519859725,865.669031870551,137.719788740923));
#66520=CARTESIAN_POINT('Ctrl Pts',(25.8890768417382,865.808805694758,137.786192633038));
#66521=CARTESIAN_POINT('Ctrl Pts',(25.7957603915284,865.898310945924,137.827331743256));
#66522=CARTESIAN_POINT('Ctrl Pts',(25.6515314161874,866.106854010585,137.921169571086));
#66523=CARTESIAN_POINT('Ctrl Pts',(25.6025450206964,866.224190370345,137.973081763217));
#66524=CARTESIAN_POINT('Ctrl Pts',(25.5576579280982,866.468752913701,138.079530086611));
#66525=CARTESIAN_POINT('Ctrl Pts',(25.5616134804233,866.593527306509,138.133009924179));
#66526=CARTESIAN_POINT('Ctrl Pts',(25.6217087769471,866.835075114573,138.234525463799));
#66527=CARTESIAN_POINT('Ctrl Pts',(25.67720277568,866.949524219527,138.281577706287));
#66528=CARTESIAN_POINT('Ctrl Pts',(25.7942924888293,867.10244198729,138.342489112607));
#66529=CARTESIAN_POINT('Ctrl Pts',(25.8389091629305,867.150052395241,138.36108271354));
#66530=CARTESIAN_POINT('Ctrl Pts',(25.9381742628927,867.237115179535,138.394249570918));
#66531=CARTESIAN_POINT('Ctrl Pts',(25.9926740025924,867.276241848119,138.408688096572));
#66532=CARTESIAN_POINT('Ctrl Pts',(26.0509384417415,867.310125790805,138.420663828409));
#66533=CARTESIAN_POINT('Ctrl Pts',(26.587153405201,866.812688940616,140.284451947729));
#66534=CARTESIAN_POINT('Ctrl Pts',(26.7193793732077,866.814885935223,140.27823580659));
#66535=CARTESIAN_POINT('Ctrl Pts',(26.8502664503425,866.793494538863,140.261714995427));
#66536=CARTESIAN_POINT('Ctrl Pts',(27.0971885346626,866.705014039761,140.210141054699));
#66537=CARTESIAN_POINT('Ctrl Pts',(27.2105273651152,866.637908000364,140.175251086928));
#66538=CARTESIAN_POINT('Ctrl Pts',(27.4023994581216,866.465679384199,140.092020876916));
#66539=CARTESIAN_POINT('Ctrl Pts',(27.4787882987761,866.361916724528,140.044388992606));
#66540=CARTESIAN_POINT('Ctrl Pts',(27.5824289901366,866.132397663624,139.943336242273));
#66541=CARTESIAN_POINT('Ctrl Pts',(27.6089075312998,866.008996721649,139.890929576514));
#66542=CARTESIAN_POINT('Ctrl Pts',(27.6082114386975,865.759642775383,139.788074798368));
#66543=CARTESIAN_POINT('Ctrl Pts',(27.5814117467065,865.636169556493,139.738611745961));
#66544=CARTESIAN_POINT('Ctrl Pts',(27.477752251191,865.404971889854,139.648097208982));
#66545=CARTESIAN_POINT('Ctrl Pts',(27.4018173881855,865.299576554605,139.607941662044));
#66546=CARTESIAN_POINT('Ctrl Pts',(27.2102770903413,865.121570406777,139.541879144639));
#66547=CARTESIAN_POINT('Ctrl Pts',(27.0964598713859,865.050824388365,139.516659824231));
#66548=CARTESIAN_POINT('Ctrl Pts',(26.849268718363,864.955513020048,139.48520463439));
#66549=CARTESIAN_POINT('Ctrl Pts',(26.7188000123769,864.930770837042,139.478828276305));
#66550=CARTESIAN_POINT('Ctrl Pts',(26.5871534051988,864.929584227576,139.482185650009));
#66551=CARTESIAN_POINT('Origin',(26.5871534051988,869.497999037637,129.621532615152));
#66552=CARTESIAN_POINT('',(26.5871534051988,867.834582406131,135.828427858641));
#66553=CARTESIAN_POINT('Origin',(26.5871534051988,867.363160175522,135.661811291374));
#66554=CARTESIAN_POINT('',(26.5871534051989,866.334637698876,140.072347243623));
#66555=CARTESIAN_POINT('',(26.5871534051988,869.969421268246,129.788149182419));
#66556=CARTESIAN_POINT('Ctrl Pts',(26.5868406553291,865.412824171668,139.679609816816));
#66557=CARTESIAN_POINT('Ctrl Pts',(26.5255998020287,865.412183595571,139.681537205492));
#66558=CARTESIAN_POINT('Ctrl Pts',(26.4649104955618,865.421941243081,139.68780579045));
#66559=CARTESIAN_POINT('Ctrl Pts',(26.3457464565317,865.462873629541,139.709418190761));
#66560=CARTESIAN_POINT('Ctrl Pts',(26.2891055273704,865.495411593307,139.725285602752));
#66561=CARTESIAN_POINT('Ctrl Pts',(26.1937997484409,865.578522678673,139.764274150391));
#66562=CARTESIAN_POINT('Ctrl Pts',(26.1558424859167,865.628074988295,139.786932714436));
#66563=CARTESIAN_POINT('Ctrl Pts',(26.103082090476,865.737925353352,139.836204427724));
#66564=CARTESIAN_POINT('Ctrl Pts',(26.0887497271715,865.79717062609,139.862344963465));
#66565=CARTESIAN_POINT('Ctrl Pts',(26.0858142209995,865.917447595876,139.914486375135));
#66566=CARTESIAN_POINT('Ctrl Pts',(26.0971464162827,865.977336585021,139.939991349396));
#66567=CARTESIAN_POINT('Ctrl Pts',(26.1441282561774,866.089926265049,139.986829514137));
#66568=CARTESIAN_POINT('Ctrl Pts',(26.1792517930982,866.141567010159,140.007721422777));
#66569=CARTESIAN_POINT('Ctrl Pts',(26.2689503584317,866.229912144945,140.042023720481));
#66570=CARTESIAN_POINT('Ctrl Pts',(26.3226466874476,866.265743802293,140.055092849982));
#66571=CARTESIAN_POINT('Ctrl Pts',(26.441881427653,866.316758842355,140.071590853784));
#66572=CARTESIAN_POINT('Ctrl Pts',(26.5062738764259,866.331359924575,140.074821826206));
#66573=CARTESIAN_POINT('Ctrl Pts',(26.6373461264923,866.337029436076,140.070966439477));
#66574=CARTESIAN_POINT('Ctrl Pts',(26.7027421471079,866.327940656787,140.063877351223));
#66575=CARTESIAN_POINT('Ctrl Pts',(26.8256441219465,866.286918105112,140.04037031043));
#66576=CARTESIAN_POINT('Ctrl Pts',(26.881946610192,866.255328764845,140.024162420287));
#66577=CARTESIAN_POINT('Ctrl Pts',(26.9786069339817,866.172867767899,139.984500598062));
#66578=CARTESIAN_POINT('Ctrl Pts',(27.0176803150346,866.122451804828,139.96130813766));
#66579=CARTESIAN_POINT('Ctrl Pts',(27.0715216886377,866.010441767537,139.911553817448));
#66580=CARTESIAN_POINT('Ctrl Pts',(27.085940382297,865.950035340394,139.88550652597));
#66581=CARTESIAN_POINT('Ctrl Pts',(27.0882151259211,865.827369124149,139.83393799764));
#66582=CARTESIAN_POINT('Ctrl Pts',(27.0761576373045,865.766335361574,139.808922668868));
#66583=CARTESIAN_POINT('Ctrl Pts',(27.0269873600959,865.651790351316,139.763061341531));
#66584=CARTESIAN_POINT('Ctrl Pts',(26.9903600724254,865.599432603596,139.742672719495));
#66585=CARTESIAN_POINT('Ctrl Pts',(26.8972212757687,865.510709914048,139.709218650094));
#66586=CARTESIAN_POINT('Ctrl Pts',(26.8416271124669,865.475260573725,139.696497506621));
#66587=CARTESIAN_POINT('Ctrl Pts',(26.7190165790861,865.426428105236,139.68057103062));
#66588=CARTESIAN_POINT('Ctrl Pts',(26.6532462147938,865.413518770318,139.677519883112));
#66589=CARTESIAN_POINT('Ctrl Pts',(26.5868406553291,865.412824171668,139.679609816816));
#66590=CARTESIAN_POINT('Origin',(19.6109167136347,869.682182736162,129.686629366222));
#66591=CARTESIAN_POINT('',(19.6109167136347,865.032343784683,139.997700189292));
#66592=CARTESIAN_POINT('',(19.6109167136317,866.731743347019,140.879663611168));
#66593=CARTESIAN_POINT('Ctrl Pts',(19.6109167136347,865.032343784683,139.997700189293));
#66594=CARTESIAN_POINT('Ctrl Pts',(19.6079091554838,865.032244744606,139.997980411688));
#66595=CARTESIAN_POINT('Ctrl Pts',(19.6049010676707,865.032158534803,139.998267278442));
#66596=CARTESIAN_POINT('Ctrl Pts',(19.4766452794723,865.029030963697,140.010779980277));
#66597=CARTESIAN_POINT('Ctrl Pts',(19.3532338372231,865.048294548138,140.034265423507));
#66598=CARTESIAN_POINT('Ctrl Pts',(19.1229869647607,865.128765153076,140.101570012603));
#66599=CARTESIAN_POINT('Ctrl Pts',(19.0185497725543,865.189582551132,140.144935981));
#66600=CARTESIAN_POINT('Ctrl Pts',(18.8426550411811,865.345508921656,140.246549461264));
#66601=CARTESIAN_POINT('Ctrl Pts',(18.7732964870958,865.439673391445,140.304075495621));
#66602=CARTESIAN_POINT('Ctrl Pts',(18.6822541059607,865.645813434001,140.423536535197));
#66603=CARTESIAN_POINT('Ctrl Pts',(18.6603346908435,865.755588806299,140.484316542825));
#66604=CARTESIAN_POINT('Ctrl Pts',(18.6657293960687,865.976428794269,140.600814327004));
#66605=CARTESIAN_POINT('Ctrl Pts',(18.6920611528413,866.085448363961,140.655550665007));
#66606=CARTESIAN_POINT('Ctrl Pts',(18.7893203169287,866.289454747597,140.751818413044));
#66607=CARTESIAN_POINT('Ctrl Pts',(18.8587059789424,866.382580844235,140.792546559396));
#66608=CARTESIAN_POINT('Ctrl Pts',(19.0327570890426,866.542331936136,140.855025819383));
#66609=CARTESIAN_POINT('Ctrl Pts',(19.1356492734084,866.607153791863,140.876043211764));
#66610=CARTESIAN_POINT('Ctrl Pts',(19.3634697244148,866.700199832375,140.895524818092));
#66611=CARTESIAN_POINT('Ctrl Pts',(19.486253519577,866.726755317152,140.893386472135));
#66612=CARTESIAN_POINT('Ctrl Pts',(19.6099239036713,866.731704083989,140.879773141484));
#66613=CARTESIAN_POINT('Ctrl Pts',(19.6102548515049,866.731717327124,140.879736711563));
#66614=CARTESIAN_POINT('Ctrl Pts',(19.6105857882002,866.731730414779,140.879700201439));
#66615=CARTESIAN_POINT('Ctrl Pts',(19.6109167136287,866.731743347019,140.879663611168));
#66616=CARTESIAN_POINT('',(19.6109167136152,867.422358230611,138.925648987921));
#66617=CARTESIAN_POINT('',(19.6109167136347,870.576078908781,130.002562519359));
#66618=CARTESIAN_POINT('Ctrl Pts',(19.0292497216265,867.224999147202,138.885672182601));
#66619=CARTESIAN_POINT('Ctrl Pts',(19.1227486191325,867.293488403287,138.909878603093));
#66620=CARTESIAN_POINT('Ctrl Pts',(19.2289639550593,867.345865874679,138.925042796753));
#66621=CARTESIAN_POINT('Ctrl Pts',(19.4621066632783,867.414959985394,138.936185048728));
#66622=CARTESIAN_POINT('Ctrl Pts',(19.5874489541267,867.428811225524,138.930935182979));
#66623=CARTESIAN_POINT('Ctrl Pts',(19.8328387076159,867.412118580623,138.899829622964));
#66624=CARTESIAN_POINT('Ctrl Pts',(19.950639878208,867.382489738374,138.874628249283));
#66625=CARTESIAN_POINT('Ctrl Pts',(20.1674570962931,867.283241297794,138.807316411628));
#66626=CARTESIAN_POINT('Ctrl Pts',(20.2641613329589,867.21389398404,138.765561630593));
#66627=CARTESIAN_POINT('Ctrl Pts',(20.422532069456,867.04339149722,138.67070801227));
#66628=CARTESIAN_POINT('Ctrl Pts',(20.4822867073186,866.943431693524,138.618354249358));
#66629=CARTESIAN_POINT('Ctrl Pts',(20.5549203637325,866.726416809543,138.510198647565));
#66630=CARTESIAN_POINT('Ctrl Pts',(20.566988053838,866.611412394766,138.455425764211));
#66631=CARTESIAN_POINT('Ctrl Pts',(20.5412611510902,866.38699592464,138.352956484362));
#66632=CARTESIAN_POINT('Ctrl Pts',(20.505781045525,866.279636569542,138.306003380776));
#66633=CARTESIAN_POINT('Ctrl Pts',(20.3944114822048,866.084846838703,138.224691870873));
#66634=CARTESIAN_POINT('Ctrl Pts',(20.3208939826588,865.998624788428,138.19069423111));
#66635=CARTESIAN_POINT('Ctrl Pts',(20.1431933364602,865.853742724939,138.137882575139));
#66636=CARTESIAN_POINT('Ctrl Pts',(20.0404736985657,865.796569280442,138.11963824823));
#66637=CARTESIAN_POINT('Ctrl Pts',(19.8154665300435,865.717927684392,138.101295106619));
#66638=CARTESIAN_POINT('Ctrl Pts',(19.6948964884546,865.698195571221,138.101867430239));
#66639=CARTESIAN_POINT('Ctrl Pts',(19.4472649029493,865.70076932914,138.123343361353));
#66640=CARTESIAN_POINT('Ctrl Pts',(19.3227590842156,865.72530728058,138.145097690271));
#66641=CARTESIAN_POINT('Ctrl Pts',(19.0959554236896,865.816363415214,138.206943116528));
#66642=CARTESIAN_POINT('Ctrl Pts',(18.9953594206764,865.881058230151,138.246029691516));
#66643=CARTESIAN_POINT('Ctrl Pts',(18.827219238832,866.043369452561,138.33751627481));
#66644=CARTESIAN_POINT('Ctrl Pts',(18.7617143413566,866.139920574725,138.389243774185));
#66645=CARTESIAN_POINT('Ctrl Pts',(18.6762189085124,866.352508618056,138.498460009162));
#66646=CARTESIAN_POINT('Ctrl Pts',(18.6574542958356,866.466708326262,138.554961115806));
#66647=CARTESIAN_POINT('Ctrl Pts',(18.6701659270992,866.684666650145,138.658617766676));
#66648=CARTESIAN_POINT('Ctrl Pts',(18.6965206216375,866.786544825246,138.705304736474));
#66649=CARTESIAN_POINT('Ctrl Pts',(18.7900576640883,866.983153146354,138.791446139332));
#66650=CARTESIAN_POINT('Ctrl Pts',(18.8583545996072,867.07542693504,138.829607231979));
#66651=CARTESIAN_POINT('Ctrl Pts',(18.9705633881621,867.179381655039,138.869204099155));
#66652=CARTESIAN_POINT('Ctrl Pts',(18.9991884464773,867.202978840793,138.877889461241));
#66653=CARTESIAN_POINT('Ctrl Pts',(19.0292497216264,867.224999147202,138.885672182601));
#66654=CARTESIAN_POINT('Ctrl Pts',(19.6109167136287,866.731743347019,140.879663611168));
#66655=CARTESIAN_POINT('Ctrl Pts',(19.7350453890134,866.736594173375,140.865938761243));
#66656=CARTESIAN_POINT('Ctrl Pts',(19.8575890635283,866.719582206182,140.840940708518));
#66657=CARTESIAN_POINT('Ctrl Pts',(20.0901695612099,866.642879318333,140.770738181999));
#66658=CARTESIAN_POINT('Ctrl Pts',(20.1973571074338,866.582323959062,140.725481789898));
#66659=CARTESIAN_POINT('Ctrl Pts',(20.3754174637689,866.426657499236,140.622508788399));
#66660=CARTESIAN_POINT('Ctrl Pts',(20.4451444074523,866.333349007783,140.565863304855));
#66661=CARTESIAN_POINT('Ctrl Pts',(20.5380041418204,866.127030987397,140.448960690095));
#66662=CARTESIAN_POINT('Ctrl Pts',(20.5608936512099,866.016174028422,140.389818557589));
#66663=CARTESIAN_POINT('Ctrl Pts',(20.5568757972104,865.791108459228,140.27612392233));
#66664=CARTESIAN_POINT('Ctrl Pts',(20.5302903942735,865.679142892364,140.222655234495));
#66665=CARTESIAN_POINT('Ctrl Pts',(20.431342672214,865.471046158108,140.128893158474));
#66666=CARTESIAN_POINT('Ctrl Pts',(20.3609340088257,865.376737859219,140.089285391298));
#66667=CARTESIAN_POINT('Ctrl Pts',(20.1849676314699,865.216411830746,140.027945043353));
#66668=CARTESIAN_POINT('Ctrl Pts',(20.081302657797,865.151979964545,140.006799493586));
#66669=CARTESIAN_POINT('Ctrl Pts',(19.8541102059258,865.061508501907,139.985891334474));
#66670=CARTESIAN_POINT('Ctrl Pts',(19.7329498924299,865.036362385392,139.986330025201));
#66671=CARTESIAN_POINT('Ctrl Pts',(19.6109167136347,865.032343784683,139.997700189293));
#66672=CARTESIAN_POINT('Origin',(19.6109167136347,869.682182736162,129.686629366222));
#66673=CARTESIAN_POINT('',(19.6109167136347,868.018766104656,135.89352460971));
#66674=CARTESIAN_POINT('Origin',(19.6109167136347,867.547343874047,135.726908042443));
#66675=CARTESIAN_POINT('',(19.610916713635,866.331868113397,140.666406603934));
#66676=CARTESIAN_POINT('',(19.6109167136347,870.153604966771,129.853245933489));
#66677=CARTESIAN_POINT('Ctrl Pts',(19.6105158575642,865.435626868842,140.201315561332));
#66678=CARTESIAN_POINT('Ctrl Pts',(19.5445607754985,865.433403241226,140.207765736195));
#66679=CARTESIAN_POINT('Ctrl Pts',(19.4794591273816,865.442910966889,140.220171218638));
#66680=CARTESIAN_POINT('Ctrl Pts',(19.3574081226334,865.484197021565,140.255701685095));
#66681=CARTESIAN_POINT('Ctrl Pts',(19.3017731489761,865.515910048717,140.278645727799));
#66682=CARTESIAN_POINT('Ctrl Pts',(19.2081734914731,865.597527739722,140.332138008657));
#66683=CARTESIAN_POINT('Ctrl Pts',(19.171200496397,865.64683527457,140.362261189116));
#66684=CARTESIAN_POINT('Ctrl Pts',(19.1221696357718,865.755215094921,140.42482899266));
#66685=CARTESIAN_POINT('Ctrl Pts',(19.1100598110342,865.813135045759,140.456671002359));
#66686=CARTESIAN_POINT('Ctrl Pts',(19.1118515839942,865.929940662849,140.517783623131));
#66687=CARTESIAN_POINT('Ctrl Pts',(19.1252751719824,865.987726201218,140.546529918869));
#66688=CARTESIAN_POINT('Ctrl Pts',(19.1758037643967,866.09600162304,140.597229592055));
#66689=CARTESIAN_POINT('Ctrl Pts',(19.2121130439346,866.145496203584,140.618755424259));
#66690=CARTESIAN_POINT('Ctrl Pts',(19.3034447035421,866.230415067544,140.651972355631));
#66691=CARTESIAN_POINT('Ctrl Pts',(19.3575214778058,866.26491290037,140.663293686408));
#66692=CARTESIAN_POINT('Ctrl Pts',(19.4773038659371,866.314517498044,140.674213215849));
#66693=CARTESIAN_POINT('Ctrl Pts',(19.5418730777901,866.328797056902,140.673521190791));
#66694=CARTESIAN_POINT('Ctrl Pts',(19.6736152354049,866.334683065614,140.659959493424));
#66695=CARTESIAN_POINT('Ctrl Pts',(19.7394529565544,866.325710171844,140.64695922555));
#66696=CARTESIAN_POINT('Ctrl Pts',(19.8629345980097,866.284947722344,140.610242714423));
#66697=CARTESIAN_POINT('Ctrl Pts',(19.9192622420866,866.253198558701,140.586718168127));
#66698=CARTESIAN_POINT('Ctrl Pts',(20.0132730793094,866.171458568217,140.532754359423));
#66699=CARTESIAN_POINT('Ctrl Pts',(20.0502301346248,866.122304978792,140.502838248092));
#66700=CARTESIAN_POINT('Ctrl Pts',(20.0996784957012,866.013357514328,140.440711734639));
#66701=CARTESIAN_POINT('Ctrl Pts',(20.1119106306503,865.954641076045,140.409084347246));
#66702=CARTESIAN_POINT('Ctrl Pts',(20.1098221531946,865.836541728484,140.348768299185));
#66703=CARTESIAN_POINT('Ctrl Pts',(20.0961522190309,865.778328520145,140.320595559343));
#66704=CARTESIAN_POINT('Ctrl Pts',(20.0449647107109,865.669355314645,140.270849586179));
#66705=CARTESIAN_POINT('Ctrl Pts',(20.0082152325769,865.619618008665,140.249706310016));
#66706=CARTESIAN_POINT('Ctrl Pts',(19.9160806668646,865.534755094891,140.21696815546));
#66707=CARTESIAN_POINT('Ctrl Pts',(19.8616751765707,865.500496340684,140.205702364501));
#66708=CARTESIAN_POINT('Ctrl Pts',(19.7411182416906,865.451592425235,140.194505652039));
#66709=CARTESIAN_POINT('Ctrl Pts',(19.6760599579182,865.437836640507,140.194905579033));
#66710=CARTESIAN_POINT('Ctrl Pts',(19.6105158575642,865.435626868842,140.201315561332));
#66711=CARTESIAN_POINT('Origin',(36.023563521447,873.7734891951,131.132635501626));
#66712=CARTESIAN_POINT('',(36.0235635214469,869.206369897989,140.989623033016));
#66713=CARTESIAN_POINT('',(36.023563521447,871.084717611128,141.805348709603));
#66714=CARTESIAN_POINT('Ctrl Pts',(36.0235635214469,869.206369897989,140.989623033016));
#66715=CARTESIAN_POINT('Ctrl Pts',(36.0214735898105,869.206358310681,140.989655817959));
#66716=CARTESIAN_POINT('Ctrl Pts',(36.0193833524411,869.206352662864,140.989691046781));
#66717=CARTESIAN_POINT('Ctrl Pts',(35.882617727463,869.206372074219,140.992155845574));
#66718=CARTESIAN_POINT('Ctrl Pts',(35.749463090655,869.231065880043,141.004676089211));
#66719=CARTESIAN_POINT('Ctrl Pts',(35.5018229049838,869.326523954077,141.049072545613));
#66720=CARTESIAN_POINT('Ctrl Pts',(35.3897375564408,869.396230800334,141.080483069051));
#66721=CARTESIAN_POINT('Ctrl Pts',(35.2007289639281,869.572090641614,141.159163642578));
#66722=CARTESIAN_POINT('Ctrl Pts',(35.1259807189736,869.676783296143,141.205790862873));
#66723=CARTESIAN_POINT('Ctrl Pts',(35.0257778864496,869.90557827225,141.307681298877));
#66724=CARTESIAN_POINT('Ctrl Pts',(35.0008332545979,870.027310359311,141.361887441756));
#66725=CARTESIAN_POINT('Ctrl Pts',(35.0035814081167,870.272368126865,141.470698389129));
#66726=CARTESIAN_POINT('Ctrl Pts',(35.031104524426,870.393401514357,141.524273249009));
#66727=CARTESIAN_POINT('Ctrl Pts',(35.135198376659,870.618759041376,141.62296180998));
#66728=CARTESIAN_POINT('Ctrl Pts',(35.2105584998169,870.721042028848,141.667170482921));
#66729=CARTESIAN_POINT('Ctrl Pts',(35.3996779064446,870.893807170752,141.739826611328));
#66730=CARTESIAN_POINT('Ctrl Pts',(35.5115271934762,870.962665330356,141.767583474772));
#66731=CARTESIAN_POINT('Ctrl Pts',(35.7579249443527,871.057941141116,141.802619551707));
#66732=CARTESIAN_POINT('Ctrl Pts',(35.8900792569755,871.083250324898,141.809472095662));
#66733=CARTESIAN_POINT('Ctrl Pts',(36.0234917745249,871.084716824771,141.805350926948));
#66734=CARTESIAN_POINT('Ctrl Pts',(36.023515690209,871.084717087657,141.805350188182));
#66735=CARTESIAN_POINT('Ctrl Pts',(36.0235396058497,871.084717349776,141.805349449067));
#66736=CARTESIAN_POINT('Ctrl Pts',(36.023563521447,871.084717611128,141.805348709603));
#66737=CARTESIAN_POINT('',(36.0235635225402,871.730643764381,139.977775659879));
#66738=CARTESIAN_POINT('',(36.023563521447,874.736518335342,131.473002584693));
#66739=CARTESIAN_POINT('Ctrl Pts',(35.6798116547162,871.672817973783,139.962586861254));
#66740=CARTESIAN_POINT('Ctrl Pts',(35.8052231695942,871.71507762961,139.977522853514));
#66741=CARTESIAN_POINT('Ctrl Pts',(35.9381629843462,871.734523094844,139.982078628726));
#66742=CARTESIAN_POINT('Ctrl Pts',(36.2041147848115,871.725612726923,139.970077777723));
#66743=CARTESIAN_POINT('Ctrl Pts',(36.3345322301639,871.697340488082,139.9536428323));
#66744=CARTESIAN_POINT('Ctrl Pts',(36.5761339446808,871.596148008136,139.902025507603));
#66745=CARTESIAN_POINT('Ctrl Pts',(36.6849112527287,871.524001433083,139.867264633866));
#66746=CARTESIAN_POINT('Ctrl Pts',(36.8660233281058,871.34459099685,139.784090197));
#66747=CARTESIAN_POINT('Ctrl Pts',(36.9364725987585,871.238881431279,139.736415930733));
#66748=CARTESIAN_POINT('Ctrl Pts',(37.0287682425443,871.007749581237,139.63463028974));
#66749=CARTESIAN_POINT('Ctrl Pts',(37.0496797292442,870.884516345032,139.581486323711));
#66750=CARTESIAN_POINT('Ctrl Pts',(37.0385422347577,870.638154768914,139.477204469923));
#66751=CARTESIAN_POINT('Ctrl Pts',(37.0070972678148,870.517384161214,139.427039804527));
#66752=CARTESIAN_POINT('Ctrl Pts',(36.8951079532623,870.291807088037,139.334908832364));
#66753=CARTESIAN_POINT('Ctrl Pts',(36.8150498717391,870.189458250906,139.293957549782));
#66754=CARTESIAN_POINT('Ctrl Pts',(36.6165333688192,870.018953521555,139.227204512949));
#66755=CARTESIAN_POINT('Ctrl Pts',(36.4999935670778,869.952555527962,139.202085741226));
#66756=CARTESIAN_POINT('Ctrl Pts',(36.2472860569667,869.86583536407,139.1713397297));
#66757=CARTESIAN_POINT('Ctrl Pts',(36.113796652642,869.845911321467,139.165822642891));
#66758=CARTESIAN_POINT('Ctrl Pts',(35.846601173448,869.854686791253,139.175105224452));
#66759=CARTESIAN_POINT('Ctrl Pts',(35.7155035887039,869.883261068966,139.189805240037));
#66760=CARTESIAN_POINT('Ctrl Pts',(35.4734839226148,869.985155430913,139.237894214928));
#66761=CARTESIAN_POINT('Ctrl Pts',(35.3648304759233,870.057337406772,139.270764399454));
#66762=CARTESIAN_POINT('Ctrl Pts',(35.1832276548471,870.236747825837,139.351177205328));
#66763=CARTESIAN_POINT('Ctrl Pts',(35.1123462065239,870.342524587299,139.398067217846));
#66764=CARTESIAN_POINT('Ctrl Pts',(35.0186507130101,870.574645240218,139.500238163134));
#66765=CARTESIAN_POINT('Ctrl Pts',(34.9973326807799,870.698948554061,139.554612712571));
#66766=CARTESIAN_POINT('Ctrl Pts',(35.0087427455771,870.946828568636,139.662233542543));
#66767=CARTESIAN_POINT('Ctrl Pts',(35.0407764294759,871.068036538043,139.714452885408));
#66768=CARTESIAN_POINT('Ctrl Pts',(35.1539420342416,871.292414719914,139.809900098182));
#66769=CARTESIAN_POINT('Ctrl Pts',(35.2339185528415,871.393439110319,139.852207592312));
#66770=CARTESIAN_POINT('Ctrl Pts',(35.3826459269411,871.520015216523,139.903808964145));
#66771=CARTESIAN_POINT('Ctrl Pts',(35.4369088327499,871.557826960076,139.918939385534));
#66772=CARTESIAN_POINT('Ctrl Pts',(35.5533694307271,871.623511986515,139.944550619951));
#66773=CARTESIAN_POINT('Ctrl Pts',(35.6153485033544,871.651095960516,139.954909566782));
#66774=CARTESIAN_POINT('Ctrl Pts',(35.6798116547161,871.672817973783,139.962586861254));
#66775=CARTESIAN_POINT('Ctrl Pts',(36.023563521447,871.084717611128,141.805348709603));
#66776=CARTESIAN_POINT('Ctrl Pts',(36.1535485828446,871.086138099153,141.801329603676));
#66777=CARTESIAN_POINT('Ctrl Pts',(36.2822520299091,871.064895525646,141.786978732021));
#66778=CARTESIAN_POINT('Ctrl Pts',(36.5277296351162,870.977781321758,141.738902417381));
#66779=CARTESIAN_POINT('Ctrl Pts',(36.6415087243966,870.911149537884,141.704969375112));
#66780=CARTESIAN_POINT('Ctrl Pts',(36.8346602266769,870.740029154615,141.622421346045));
#66781=CARTESIAN_POINT('Ctrl Pts',(36.9118265070258,870.636834245981,141.574480960796));
#66782=CARTESIAN_POINT('Ctrl Pts',(37.0173134081556,870.408051769617,141.471727260535));
#66783=CARTESIAN_POINT('Ctrl Pts',(37.0446601784414,870.284713024406,141.417925385765));
#66784=CARTESIAN_POINT('Ctrl Pts',(37.0452748520624,870.035789658795,141.312099019871));
#66785=CARTESIAN_POINT('Ctrl Pts',(37.0191063125277,869.912675413112,141.261085179727));
#66786=CARTESIAN_POINT('Ctrl Pts',(36.9166621004451,869.682160318425,141.167510971958));
#66787=CARTESIAN_POINT('Ctrl Pts',(36.8413893433617,869.577047198559,141.125859475705));
#66788=CARTESIAN_POINT('Ctrl Pts',(36.6508038094406,869.399038736796,141.056715830726));
#66789=CARTESIAN_POINT('Ctrl Pts',(36.5371750424065,869.328106314267,141.029977428978));
#66790=CARTESIAN_POINT('Ctrl Pts',(36.2887995441781,869.231998274348,140.995352221373));
#66791=CARTESIAN_POINT('Ctrl Pts',(36.1568030641379,869.207108624384,140.987532892458));
#66792=CARTESIAN_POINT('Ctrl Pts',(36.0235635214469,869.206369897989,140.989623033016));
#66793=CARTESIAN_POINT('Origin',(36.023563521447,873.7734891951,131.132635501626));
#66794=CARTESIAN_POINT('',(36.023563521447,872.110072563594,137.339530745114));
#66795=CARTESIAN_POINT('Origin',(36.023563521447,871.638650332985,137.172914177847));
#66796=CARTESIAN_POINT('',(36.0235635214471,870.608405405657,141.588323604301));
#66797=CARTESIAN_POINT('',(36.023563521447,874.244911425709,131.299252068893));
#66798=CARTESIAN_POINT('Ctrl Pts',(36.023552436116,869.688940292305,141.188941320012));
#66799=CARTESIAN_POINT('Ctrl Pts',(35.9633631698392,869.688520842301,141.190132109607));
#66800=CARTESIAN_POINT('Ctrl Pts',(35.9036857119017,869.698133963336,141.195550737741));
#66801=CARTESIAN_POINT('Ctrl Pts',(35.7853286796557,869.738381949188,141.215393646171));
#66802=CARTESIAN_POINT('Ctrl Pts',(35.7285620503972,869.770665463377,141.230488710799));
#66803=CARTESIAN_POINT('Ctrl Pts',(35.6320548273116,869.853831216061,141.268507782764));
#66804=CARTESIAN_POINT('Ctrl Pts',(35.5933235777732,869.903939954933,141.29108002934));
#66805=CARTESIAN_POINT('Ctrl Pts',(35.5398537319471,870.014490714732,141.340430302232));
#66806=CARTESIAN_POINT('Ctrl Pts',(35.5253419006028,870.073746821741,141.366684028314));
#66807=CARTESIAN_POINT('Ctrl Pts',(35.5220958115816,870.193996208895,141.41954015403));
#66808=CARTESIAN_POINT('Ctrl Pts',(35.5333326526035,870.253850853304,141.445640232718));
#66809=CARTESIAN_POINT('Ctrl Pts',(35.5802108352733,870.366178452406,141.494031816885));
#66810=CARTESIAN_POINT('Ctrl Pts',(35.6153125063336,870.417611126486,141.51587339165));
#66811=CARTESIAN_POINT('Ctrl Pts',(35.7049419116693,870.505339114735,141.55225255951));
#66812=CARTESIAN_POINT('Ctrl Pts',(35.7585566921889,870.540813238459,141.566448497113));
#66813=CARTESIAN_POINT('Ctrl Pts',(35.8775574317109,870.591104860492,141.585201642523));
#66814=CARTESIAN_POINT('Ctrl Pts',(35.9417806479005,870.605391865572,141.589557400257));
#66815=CARTESIAN_POINT('Ctrl Pts',(36.0725734574083,870.610611423961,141.587762685552));
#66816=CARTESIAN_POINT('Ctrl Pts',(36.1378527847367,870.601397690208,141.581589950046));
#66817=CARTESIAN_POINT('Ctrl Pts',(36.2607138445109,870.560312018696,141.559533663607));
#66818=CARTESIAN_POINT('Ctrl Pts',(36.3170688658126,870.528758849371,141.54383433519));
#66819=CARTESIAN_POINT('Ctrl Pts',(36.4140299847881,870.44644218463,141.504705130878));
#66820=CARTESIAN_POINT('Ctrl Pts',(36.4533051342435,870.396097725773,141.481509106258));
#66821=CARTESIAN_POINT('Ctrl Pts',(36.507536546622,870.284320328245,141.431333906446));
#66822=CARTESIAN_POINT('Ctrl Pts',(36.5221437683816,870.224067148803,141.404876273121));
#66823=CARTESIAN_POINT('Ctrl Pts',(36.5247797852127,870.101801258789,141.352231451907));
#66824=CARTESIAN_POINT('Ctrl Pts',(36.5129148662676,870.041000669466,141.326558385375));
#66825=CARTESIAN_POINT('Ctrl Pts',(36.4641227992931,869.926876460825,141.279211080816));
#66826=CARTESIAN_POINT('Ctrl Pts',(36.4276685530675,869.874698686033,141.258007904886));
#66827=CARTESIAN_POINT('Ctrl Pts',(36.3347189194866,869.786196540001,141.222815192883));
#66828=CARTESIAN_POINT('Ctrl Pts',(36.279101758849,869.750821435053,141.209201905681));
#66829=CARTESIAN_POINT('Ctrl Pts',(36.1562325648716,869.702171695576,141.191512996649));
#66830=CARTESIAN_POINT('Ctrl Pts',(36.0902224625366,869.689404905759,141.187622314505));
#66831=CARTESIAN_POINT('Ctrl Pts',(36.023552436116,869.688940292305,141.188941320012));
#66832=CARTESIAN_POINT('Origin',(29.240389675011,875.321188457674,131.679644788733));
#66833=CARTESIAN_POINT('',(29.240389675011,870.675924374847,141.977771552158));
#66834=CARTESIAN_POINT('',(29.2403896750132,872.362839858081,142.895057226278));
#66835=CARTESIAN_POINT('Ctrl Pts',(29.240389675011,870.675924374847,141.977771552158));
#66836=CARTESIAN_POINT('Ctrl Pts',(29.2367816845808,870.675840918628,141.978007681839));
#66837=CARTESIAN_POINT('Ctrl Pts',(29.2331728647531,870.675775848065,141.978253596864));
#66838=CARTESIAN_POINT('Ctrl Pts',(29.1043285666561,870.674110361653,141.987381376002));
#66839=CARTESIAN_POINT('Ctrl Pts',(28.9809421210146,870.694687261028,142.007848186233));
#66840=CARTESIAN_POINT('Ctrl Pts',(28.7509635165537,870.777401026941,142.070066517537));
#66841=CARTESIAN_POINT('Ctrl Pts',(28.6468282149897,870.839029892949,142.111371712144));
#66842=CARTESIAN_POINT('Ctrl Pts',(28.471506017528,870.995818703683,142.210241340407));
#66843=CARTESIAN_POINT('Ctrl Pts',(28.4024845445846,871.089971733926,142.26710605341));
#66844=CARTESIAN_POINT('Ctrl Pts',(28.3113570012837,871.296145178495,142.387593174257));
#66845=CARTESIAN_POINT('Ctrl Pts',(28.2895286618689,871.406165584795,142.450083449862));
#66846=CARTESIAN_POINT('Ctrl Pts',(28.2955935390807,871.62674069641,142.57167116704));
#66847=CARTESIAN_POINT('Ctrl Pts',(28.3225857931083,871.7353464104,142.629746646865));
#66848=CARTESIAN_POINT('Ctrl Pts',(28.4213904548344,871.937131752257,142.733463409759));
#66849=CARTESIAN_POINT('Ctrl Pts',(28.4914745110623,872.028660429407,142.778324187968));
#66850=CARTESIAN_POINT('Ctrl Pts',(28.6663561746253,872.184110305666,142.849229501281));
#66851=CARTESIAN_POINT('Ctrl Pts',(28.7691430256071,872.246568056492,142.874634279215));
#66852=CARTESIAN_POINT('Ctrl Pts',(28.9959552138475,872.3348806794,142.902694767692));
#66853=CARTESIAN_POINT('Ctrl Pts',(29.1176930263198,872.359391999469,142.904812541878));
#66854=CARTESIAN_POINT('Ctrl Pts',(29.2403896750154,872.362839858081,142.895057226278));
#66855=CARTESIAN_POINT('',(29.240389674993,873.056476967889,140.93249156488));
#66856=CARTESIAN_POINT('',(29.240389675011,876.215084630293,131.99557794187));
#66857=CARTESIAN_POINT('Ctrl Pts',(28.8270936452429,872.962602665625,140.91353540268));
#66858=CARTESIAN_POINT('Ctrl Pts',(28.9336523008359,873.011266829159,140.930734964666));
#66859=CARTESIAN_POINT('Ctrl Pts',(29.0488646698254,873.041701491219,140.938143827054));
#66860=CARTESIAN_POINT('Ctrl Pts',(29.2912290268742,873.063674303931,140.932631817926));
#66861=CARTESIAN_POINT('Ctrl Pts',(29.4161837973998,873.052721869669,140.918615494393));
#66862=CARTESIAN_POINT('Ctrl Pts',(29.6507838752602,872.988463698336,140.870698667918));
#66863=CARTESIAN_POINT('Ctrl Pts',(29.7584566851137,872.936491073207,140.837600245346));
#66864=CARTESIAN_POINT('Ctrl Pts',(29.946416844765,872.797130430654,140.756111398283));
#66865=CARTESIAN_POINT('Ctrl Pts',(30.0245209206595,872.710460146978,140.708234093541));
#66866=CARTESIAN_POINT('Ctrl Pts',(30.1394357999211,872.51287589023,140.603808861391));
#66867=CARTESIAN_POINT('Ctrl Pts',(30.1746624674555,872.403503729237,140.548128452935));
#66868=CARTESIAN_POINT('Ctrl Pts',(30.1956744752123,872.177208845924,140.436692985381));
#66869=CARTESIAN_POINT('Ctrl Pts',(30.1811394943046,872.06244893213,140.382006516948));
#66870=CARTESIAN_POINT('Ctrl Pts',(30.1048834019336,871.848138665372,140.28310911132));
#66871=CARTESIAN_POINT('Ctrl Pts',(30.0458800857863,871.750142328819,140.239465215294));
#66872=CARTESIAN_POINT('Ctrl Pts',(29.8931263874831,871.581526406594,140.167404414969));
#66873=CARTESIAN_POINT('Ctrl Pts',(29.8019579916615,871.511624225611,140.13917476921));
#66874=CARTESIAN_POINT('Ctrl Pts',(29.5960805804867,871.404753576186,140.099797633118));
#66875=CARTESIAN_POINT('Ctrl Pts',(29.4831339722014,871.368951998056,140.089106846918));
#66876=CARTESIAN_POINT('Ctrl Pts',(29.246356895948,871.336071810407,140.086937335411));
#66877=CARTESIAN_POINT('Ctrl Pts',(29.1245931970823,871.340354230845,140.095997207761));
#66878=CARTESIAN_POINT('Ctrl Pts',(28.8843654037844,871.391273363315,140.134560030048));
#66879=CARTESIAN_POINT('Ctrl Pts',(28.7688976775041,871.439591960204,140.164719243706));
#66880=CARTESIAN_POINT('Ctrl Pts',(28.5691846488931,871.57291459618,140.24150308166));
#66881=CARTESIAN_POINT('Ctrl Pts',(28.4861769677574,871.655803975503,140.28702023133));
#66882=CARTESIAN_POINT('Ctrl Pts',(28.3598671301212,871.847294295614,140.388819695051));
#66883=CARTESIAN_POINT('Ctrl Pts',(28.3183042721467,871.954455505366,140.444297158382));
#66884=CARTESIAN_POINT('Ctrl Pts',(28.2839172461224,872.178923534258,140.557712182225));
#66885=CARTESIAN_POINT('Ctrl Pts',(28.29186363956,872.294195294952,140.614592188492));
#66886=CARTESIAN_POINT('Ctrl Pts',(28.3542051600735,872.504716080702,140.71562016173));
#66887=CARTESIAN_POINT('Ctrl Pts',(28.4031895718858,872.599128380444,140.759668438562));
#66888=CARTESIAN_POINT('Ctrl Pts',(28.539191557786,872.772990084837,140.837770417423));
#66889=CARTESIAN_POINT('Ctrl Pts',(28.6267282407186,872.849821237841,140.870473560104));
#66890=CARTESIAN_POINT('Ctrl Pts',(28.7596064663182,872.929488583218,140.901486447305));
#66891=CARTESIAN_POINT('Ctrl Pts',(28.79283346517,872.946956418997,140.908005489718));
#66892=CARTESIAN_POINT('Ctrl Pts',(28.8270936452429,872.962602665625,140.91353540268));
#66893=CARTESIAN_POINT('Ctrl Pts',(29.2403896750154,872.362839858081,142.895057226278));
#66894=CARTESIAN_POINT('Ctrl Pts',(29.2405343880238,872.362843924614,142.895045720495));
#66895=CARTESIAN_POINT('Ctrl Pts',(29.2406791023676,872.362847961838,142.895034198211));
#66896=CARTESIAN_POINT('Ctrl Pts',(29.2408238180354,872.36285196975,142.895022659426));
#66897=CARTESIAN_POINT('Ctrl Pts',(29.3621682470146,872.36621261347,142.885347361435));
#66898=CARTESIAN_POINT('Ctrl Pts',(29.4819887080006,872.348905343143,142.864265901722));
#66899=CARTESIAN_POINT('Ctrl Pts',(29.711794366194,872.273420916633,142.800706501727));
#66900=CARTESIAN_POINT('Ctrl Pts',(29.8186582549862,872.213860059979,142.757787166795));
#66901=CARTESIAN_POINT('Ctrl Pts',(29.9990404951428,872.05967678094,142.656582416295));
#66902=CARTESIAN_POINT('Ctrl Pts',(30.0705564373936,871.96610060915,142.599073633974));
#66903=CARTESIAN_POINT('Ctrl Pts',(30.1660633553242,871.759492852032,142.478737404305));
#66904=CARTESIAN_POINT('Ctrl Pts',(30.1898706208027,871.648600351706,142.417069812452));
#66905=CARTESIAN_POINT('Ctrl Pts',(30.1869698340323,871.424544776654,142.297613225431));
#66906=CARTESIAN_POINT('Ctrl Pts',(30.1609292067764,871.313545347621,142.240903072839));
#66907=CARTESIAN_POINT('Ctrl Pts',(30.0621397778283,871.105762271853,142.139169867226));
#66908=CARTESIAN_POINT('Ctrl Pts',(29.9906321851297,871.011024473981,142.095109691605));
#66909=CARTESIAN_POINT('Ctrl Pts',(29.8127632268166,870.852368043617,142.025877871808));
#66910=CARTESIAN_POINT('Ctrl Pts',(29.7089787024167,870.789466448968,142.00102846387));
#66911=CARTESIAN_POINT('Ctrl Pts',(29.4822392208746,870.70236091131,141.972947166182));
#66912=CARTESIAN_POINT('Ctrl Pts',(29.3617843938213,870.678732349099,141.969826715056));
#66913=CARTESIAN_POINT('Ctrl Pts',(29.240389675011,870.675924374847,141.977771552158));
#66914=CARTESIAN_POINT('Origin',(29.240389675011,875.321188457674,131.679644788733));
#66915=CARTESIAN_POINT('',(29.240389675011,873.657771826168,137.886540032222));
#66916=CARTESIAN_POINT('Origin',(29.240389675011,873.186349595559,137.719923464954));
#66917=CARTESIAN_POINT('',(29.2403896750113,871.966311801343,142.672329770708));
#66918=CARTESIAN_POINT('',(29.240389675011,875.792610688283,131.846261356));
#66919=CARTESIAN_POINT('Ctrl Pts',(29.2406093312764,871.076684303001,142.188525563727));
#66920=CARTESIAN_POINT('Ctrl Pts',(29.1766503670039,871.075101410464,142.192919855086));
#66921=CARTESIAN_POINT('Ctrl Pts',(29.1134480527164,871.08447829764,142.203123919309));
#66922=CARTESIAN_POINT('Ctrl Pts',(28.992504095938,871.124714337439,142.234746280417));
#66923=CARTESIAN_POINT('Ctrl Pts',(28.9363839134385,871.156158888874,142.256354888854));
#66924=CARTESIAN_POINT('Ctrl Pts',(28.8415260359534,871.237140896149,142.308141310702));
#66925=CARTESIAN_POINT('Ctrl Pts',(28.8038531092525,871.286088118937,142.337914947352));
#66926=CARTESIAN_POINT('Ctrl Pts',(28.7526370196238,871.394946036471,142.40164596502));
#66927=CARTESIAN_POINT('Ctrl Pts',(28.7397121645,871.453939292401,142.435051348497));
#66928=CARTESIAN_POINT('Ctrl Pts',(28.7410976817578,871.571637431497,142.499533406106));
#66929=CARTESIAN_POINT('Ctrl Pts',(28.7544777193056,871.629248844171,142.530081070611));
#66930=CARTESIAN_POINT('Ctrl Pts',(28.8051004198344,871.736636062784,142.584812959593));
#66931=CARTESIAN_POINT('Ctrl Pts',(28.8414633996518,871.785510712384,142.608573729047));
#66932=CARTESIAN_POINT('Ctrl Pts',(28.9327524760998,871.868747444632,142.646374157118));
#66933=CARTESIAN_POINT('Ctrl Pts',(28.9866219900859,871.902337699474,142.660080304813));
#66934=CARTESIAN_POINT('Ctrl Pts',(29.1057819299297,871.950168605278,142.675695243178));
#66935=CARTESIAN_POINT('Ctrl Pts',(29.1698765851482,871.963718616303,142.677330612537));
#66936=CARTESIAN_POINT('Ctrl Pts',(29.3005806209985,871.968579870734,142.668091050424));
#66937=CARTESIAN_POINT('Ctrl Pts',(29.3658219558896,871.959429472694,142.657088724495));
#66938=CARTESIAN_POINT('Ctrl Pts',(29.4887925124197,871.918887670554,142.623647814261));
#66939=CARTESIAN_POINT('Ctrl Pts',(29.5451141946069,871.887439870253,142.601311981726));
#66940=CARTESIAN_POINT('Ctrl Pts',(29.6401652702456,871.806187156151,142.548411193144));
#66941=CARTESIAN_POINT('Ctrl Pts',(29.6778518120375,871.75696139772,142.518260725676));
#66942=CARTESIAN_POINT('Ctrl Pts',(29.7284548414666,871.648039823179,142.454728397488));
#66943=CARTESIAN_POINT('Ctrl Pts',(29.7411139006961,871.589404978822,142.421942267325));
#66944=CARTESIAN_POINT('Ctrl Pts',(29.7396085708653,871.470797147763,142.358169018261));
#66945=CARTESIAN_POINT('Ctrl Pts',(29.7257062079282,871.411960181392,142.327766482922));
#66946=CARTESIAN_POINT('Ctrl Pts',(29.6735692326996,871.303236472631,142.273898165055));
#66947=CARTESIAN_POINT('Ctrl Pts',(29.6365554302358,871.254201035098,142.250779342196));
#66948=CARTESIAN_POINT('Ctrl Pts',(29.5440060903363,871.171100939789,142.214056048446));
#66949=CARTESIAN_POINT('Ctrl Pts',(29.4895324840044,871.137798929603,142.200768706667));
#66950=CARTESIAN_POINT('Ctrl Pts',(29.3696130132614,871.091101375852,142.185672833383));
#66951=CARTESIAN_POINT('Ctrl Pts',(29.3053785337554,871.07828724777,142.184075605069));
#66952=CARTESIAN_POINT('Ctrl Pts',(29.2406093312764,871.076684303001,142.188525563727));
#66953=CARTESIAN_POINT('Origin',(46.1965767102463,876.105745388824,131.956933754349));
#66954=CARTESIAN_POINT('',(46.1965767102464,871.539310156617,141.811985803522));
#66955=CARTESIAN_POINT('',(46.1965767102472,873.415048332981,142.635094861413));
#66956=CARTESIAN_POINT('Ctrl Pts',(46.1965767102464,871.539310156617,141.811985803522));
#66957=CARTESIAN_POINT('Ctrl Pts',(46.1937144929431,871.539304011668,141.812003189942));
#66958=CARTESIAN_POINT('Ctrl Pts',(46.1908517067503,871.539309014205,141.812025139295));
#66959=CARTESIAN_POINT('Ctrl Pts',(46.0534999164937,871.540084360332,141.813297227722));
#66960=CARTESIAN_POINT('Ctrl Pts',(45.9205687407884,871.565458979681,141.82457740446));
#66961=CARTESIAN_POINT('Ctrl Pts',(45.6732533278176,871.662243775346,141.86636373246));
#66962=CARTESIAN_POINT('Ctrl Pts',(45.5612848662722,871.73264076831,141.896452617147));
#66963=CARTESIAN_POINT('Ctrl Pts',(45.3727302369807,871.909663678627,141.972570662421));
#66964=CARTESIAN_POINT('Ctrl Pts',(45.2982635416768,872.014754229373,142.017961410119));
#66965=CARTESIAN_POINT('Ctrl Pts',(45.1984532575828,872.244160547686,142.118029234544));
#66966=CARTESIAN_POINT('Ctrl Pts',(45.173694385883,872.366101220885,142.171669705127));
#66967=CARTESIAN_POINT('Ctrl Pts',(45.1767763349096,872.611297248011,142.280401900152));
#66968=CARTESIAN_POINT('Ctrl Pts',(45.2045270734912,872.732242899625,142.334460899895));
#66969=CARTESIAN_POINT('Ctrl Pts',(45.3090871620149,872.956892070233,142.435187370653));
#66970=CARTESIAN_POINT('Ctrl Pts',(45.3847033292099,873.058580649317,142.480934171599));
#66971=CARTESIAN_POINT('Ctrl Pts',(45.5741277010826,873.229568847835,142.557408367027));
#66972=CARTESIAN_POINT('Ctrl Pts',(45.6859935378586,873.297356096951,142.587446034274));
#66973=CARTESIAN_POINT('Ctrl Pts',(45.9319537470132,873.39026526088,142.627317120645));
#66974=CARTESIAN_POINT('Ctrl Pts',(46.0636192986767,873.414464480635,142.636746803833));
#66975=CARTESIAN_POINT('Ctrl Pts',(46.196576710248,873.415048332981,142.635094861413));
#66976=CARTESIAN_POINT('',(46.1965767107091,874.061504505576,140.806022183502));
#66977=CARTESIAN_POINT('',(46.1965767102463,877.068774529067,132.297300837416));
#66978=CARTESIAN_POINT('Ctrl Pts',(46.0603115463226,874.052642389307,140.803697333072));
#66979=CARTESIAN_POINT('Ctrl Pts',(46.1923014221479,874.069394353401,140.809618043999));
#66980=CARTESIAN_POINT('Ctrl Pts',(46.3264636842238,874.062370818533,140.804818778975));
#66981=CARTESIAN_POINT('Ctrl Pts',(46.5840256589845,874.00158183426,140.774482269596));
#66982=CARTESIAN_POINT('Ctrl Pts',(46.7049123455155,873.948406123414,140.749245594537));
#66983=CARTESIAN_POINT('Ctrl Pts',(46.9178216779398,873.802172986762,140.681709377771));
#66984=CARTESIAN_POINT('Ctrl Pts',(47.0076708242949,873.710343136668,140.639991768634));
#66985=CARTESIAN_POINT('Ctrl Pts',(47.1438930481538,873.499485840497,140.545702947435));
#66986=CARTESIAN_POINT('Ctrl Pts',(47.1887777384192,873.382347031621,140.493989199866));
#66987=CARTESIAN_POINT('Ctrl Pts',(47.2266960762805,873.138311373662,140.387642916544));
#66988=CARTESIAN_POINT('Ctrl Pts',(47.2193114075928,873.013737671103,140.334025184349));
#66989=CARTESIAN_POINT('Ctrl Pts',(47.1528984655208,872.775061106413,140.232459473628));
#66990=CARTESIAN_POINT('Ctrl Pts',(47.0949906174885,872.6631450898,140.185424320325));
#66991=CARTESIAN_POINT('Ctrl Pts',(46.9348459124716,872.464535666884,140.102824628238));
#66992=CARTESIAN_POINT('Ctrl Pts',(46.8336367843973,872.380149856647,140.068222087155));
#66993=CARTESIAN_POINT('Ctrl Pts',(46.6014097214899,872.25233049921,140.016555505051));
#66994=CARTESIAN_POINT('Ctrl Pts',(46.4726603970214,872.210239908928,140.00002779212));
#66995=CARTESIAN_POINT('Ctrl Pts',(46.2063453606493,872.174953294334,139.987460137214));
#66996=CARTESIAN_POINT('Ctrl Pts',(46.0714851014881,872.181621883862,139.991341786384));
#66997=CARTESIAN_POINT('Ctrl Pts',(45.8124918514646,872.242541049771,140.019053714481));
#66998=CARTESIAN_POINT('Ctrl Pts',(45.6908788951564,872.296158170341,140.042604718078));
#66999=CARTESIAN_POINT('Ctrl Pts',(45.4774538783132,872.443185709471,140.106645284904));
#67000=CARTESIAN_POINT('Ctrl Pts',(45.3876018334669,872.53503897332,140.1464679682));
#67001=CARTESIAN_POINT('Ctrl Pts',(45.2507082502561,872.746011413384,140.238035860224));
#67002=CARTESIAN_POINT('Ctrl Pts',(45.2053596632383,872.86330621639,140.288996738346));
#67003=CARTESIAN_POINT('Ctrl Pts',(45.1662925942187,873.108583233809,140.395817588004));
#67004=CARTESIAN_POINT('Ctrl Pts',(45.1735746255535,873.234277472475,140.450683737337));
#67005=CARTESIAN_POINT('Ctrl Pts',(45.2407831731627,873.474366622656,140.555551012221));
#67006=CARTESIAN_POINT('Ctrl Pts',(45.299494962934,873.586581992753,140.604592066219));
#67007=CARTESIAN_POINT('Ctrl Pts',(45.460784995985,873.783762459085,140.690426686063));
#67008=CARTESIAN_POINT('Ctrl Pts',(45.5617486768193,873.866856228305,140.726396891969));
#67009=CARTESIAN_POINT('Ctrl Pts',(45.735613611947,873.961464421838,140.766699721802));
#67010=CARTESIAN_POINT('Ctrl Pts',(45.7971512000974,873.987800690086,140.777774321936));
#67011=CARTESIAN_POINT('Ctrl Pts',(45.9257174091181,874.029204308247,140.794803685085));
#67012=CARTESIAN_POINT('Ctrl Pts',(45.9924670317909,874.044031661671,140.800654010574));
#67013=CARTESIAN_POINT('Ctrl Pts',(46.0603115463226,874.052642389307,140.803697333072));
#67014=CARTESIAN_POINT('Ctrl Pts',(46.196576710248,873.415048332981,142.635094861413));
#67015=CARTESIAN_POINT('Ctrl Pts',(46.1967585223272,873.415049131367,142.635092602471));
#67016=CARTESIAN_POINT('Ctrl Pts',(46.1969403368227,873.415049885594,142.635090322854));
#67017=CARTESIAN_POINT('Ctrl Pts',(46.1971221537155,873.415050595624,142.635088022543));
#67018=CARTESIAN_POINT('Ctrl Pts',(46.3293223641573,873.415566862643,142.633415452066));
#67019=CARTESIAN_POINT('Ctrl Pts',(46.4601815023246,873.392724222154,142.62082390506));
#67020=CARTESIAN_POINT('Ctrl Pts',(46.7070847335911,873.301991730621,142.575215625585));
#67021=CARTESIAN_POINT('Ctrl Pts',(46.8203476425693,873.234141395486,142.542275498948));
#67022=CARTESIAN_POINT('Ctrl Pts',(47.0113946314043,873.061914923075,142.461033399297));
#67023=CARTESIAN_POINT('Ctrl Pts',(47.0872875550886,872.95912834712,142.413501722372));
#67024=CARTESIAN_POINT('Ctrl Pts',(47.191388287791,872.731128706094,142.310358062614));
#67025=CARTESIAN_POINT('Ctrl Pts',(47.2182095430374,872.607945942266,142.255692675743));
#67026=CARTESIAN_POINT('Ctrl Pts',(47.2177581155975,872.358734507253,142.147233054814));
#67027=CARTESIAN_POINT('Ctrl Pts',(47.1906112853271,872.23515978004,142.094499346869));
#67028=CARTESIAN_POINT('Ctrl Pts',(47.0859676846827,872.005453148782,141.998084602508));
#67029=CARTESIAN_POINT('Ctrl Pts',(47.0099705478659,871.901433474046,141.955257327032));
#67030=CARTESIAN_POINT('Ctrl Pts',(46.8187821282926,871.72628129303,141.884120969343));
#67031=CARTESIAN_POINT('Ctrl Pts',(46.7054924529518,871.656871990556,141.856490742835));
#67032=CARTESIAN_POINT('Ctrl Pts',(46.4588710796671,871.563505879996,141.820029177464));
#67033=CARTESIAN_POINT('Ctrl Pts',(46.3283266687638,871.539593013127,141.81118549387));
#67034=CARTESIAN_POINT('Ctrl Pts',(46.1965767102464,871.539310156617,141.811985803522));
#67035=CARTESIAN_POINT('Origin',(46.1965767102463,876.105745388824,131.956933754349));
#67036=CARTESIAN_POINT('',(46.1965767102463,874.442328757318,138.163828997837));
#67037=CARTESIAN_POINT('Origin',(46.1965767102463,873.970906526709,137.99721243057));
#67038=CARTESIAN_POINT('',(46.1965767102465,872.9397096753,142.415315215679));
#67039=CARTESIAN_POINT('',(46.1965767102463,876.577167619433,132.123550321616));
#67040=CARTESIAN_POINT('Ctrl Pts',(46.1968411429053,872.021533786227,142.012285430459));
#67041=CARTESIAN_POINT('Ctrl Pts',(46.1348931452708,872.021333101247,142.012754929298));
#67042=CARTESIAN_POINT('Ctrl Pts',(46.0734881842045,872.031753178132,142.017723413552));
#67043=CARTESIAN_POINT('Ctrl Pts',(45.9539222363994,872.074169732284,142.036888757063));
#67044=CARTESIAN_POINT('Ctrl Pts',(45.8975019133049,872.107219689185,142.051526873118));
#67045=CARTESIAN_POINT('Ctrl Pts',(45.8018160037468,872.191770318541,142.088792446426));
#67046=CARTESIAN_POINT('Ctrl Pts',(45.7635893227472,872.242503045512,142.111085597979));
#67047=CARTESIAN_POINT('Ctrl Pts',(45.7113639353332,872.353896025228,142.160089161092));
#67048=CARTESIAN_POINT('Ctrl Pts',(45.6975489663079,872.413342437864,142.186266910223));
#67049=CARTESIAN_POINT('Ctrl Pts',(45.6957048070797,872.533595683546,142.239294927549));
#67050=CARTESIAN_POINT('Ctrl Pts',(45.707655214252,872.593263119955,142.265641318822));
#67051=CARTESIAN_POINT('Ctrl Pts',(45.755874856025,872.704797681698,142.314839509429));
#67052=CARTESIAN_POINT('Ctrl Pts',(45.7915983533186,872.75564184062,142.33723653254));
#67053=CARTESIAN_POINT('Ctrl Pts',(45.8822487270904,872.841827223409,142.374943231437));
#67054=CARTESIAN_POINT('Ctrl Pts',(45.93624673542,872.876389215919,142.389908920414));
#67055=CARTESIAN_POINT('Ctrl Pts',(46.0557121402089,872.924688941862,142.410281649844));
#67056=CARTESIAN_POINT('Ctrl Pts',(46.1200085400123,872.937943820786,142.415482566568));
#67057=CARTESIAN_POINT('Ctrl Pts',(46.2507038369816,872.941158942785,142.415287982749));
#67058=CARTESIAN_POINT('Ctrl Pts',(46.3158069054221,872.930997240269,142.409854411394));
#67059=CARTESIAN_POINT('Ctrl Pts',(46.4381591803029,872.888206354577,142.389003820392));
#67060=CARTESIAN_POINT('Ctrl Pts',(46.4941628674793,872.855898190198,142.373751151953));
#67061=CARTESIAN_POINT('Ctrl Pts',(46.5892921029457,872.773168953882,142.335537771323));
#67062=CARTESIAN_POINT('Ctrl Pts',(46.6274605851056,872.723506146392,142.312933083704));
#67063=CARTESIAN_POINT('Ctrl Pts',(46.680824830468,872.612808685136,142.263274783167));
#67064=CARTESIAN_POINT('Ctrl Pts',(46.6952693168326,872.552740939566,142.236664232516));
#67065=CARTESIAN_POINT('Ctrl Pts',(46.6977194079068,872.430496918115,142.18317264406));
#67066=CARTESIAN_POINT('Ctrl Pts',(46.6855983534884,872.369519818791,142.156818143097));
#67067=CARTESIAN_POINT('Ctrl Pts',(46.6361791776284,872.255686822419,142.108158336933));
#67068=CARTESIAN_POINT('Ctrl Pts',(46.5995270010882,872.203913057215,142.086307973218));
#67069=CARTESIAN_POINT('Ctrl Pts',(46.506493373721,872.116527594763,142.049839061974));
#67070=CARTESIAN_POINT('Ctrl Pts',(46.4510803079727,872.081760306271,142.035567122818));
#67071=CARTESIAN_POINT('Ctrl Pts',(46.3287961632862,872.034129605604,142.01644344205));
#67072=CARTESIAN_POINT('Ctrl Pts',(46.2631519379868,872.021748604802,142.011782866332));
#67073=CARTESIAN_POINT('Ctrl Pts',(46.1968411429053,872.021533786227,142.012285430459));
#67074=CARTESIAN_POINT('Origin',(39.9029229553071,878.949318330988,132.961948646806));
#67075=CARTESIAN_POINT('',(39.9029229553071,874.306969838757,143.251826085178));
#67076=CARTESIAN_POINT('',(39.9029229553089,875.985831224642,144.191899892559));
#67077=CARTESIAN_POINT('Ctrl Pts',(39.9029229553071,874.306969838757,143.251826085178));
#67078=CARTESIAN_POINT('Ctrl Pts',(39.9009534307544,874.30694501926,143.251896309062));
#67079=CARTESIAN_POINT('Ctrl Pts',(39.8989836282631,874.306925665399,143.251969485561));
#67080=CARTESIAN_POINT('Ctrl Pts',(39.7715568737462,874.306027659273,143.256893792742));
#67081=CARTESIAN_POINT('Ctrl Pts',(39.647744719753,874.327347554828,143.273607956868));
#67082=CARTESIAN_POINT('Ctrl Pts',(39.4173398036129,874.41140713584,143.329072565374));
#67083=CARTESIAN_POINT('Ctrl Pts',(39.3131699848017,874.473363560329,143.367310208833));
#67084=CARTESIAN_POINT('Ctrl Pts',(39.1377884732739,874.629965346088,143.461038823805));
#67085=CARTESIAN_POINT('Ctrl Pts',(39.0686354901211,874.723405963652,143.515797110725));
#67086=CARTESIAN_POINT('Ctrl Pts',(38.9751238774499,874.930005668183,143.635280747051));
#67087=CARTESIAN_POINT('Ctrl Pts',(38.9522966177509,875.041537208258,143.699046013975));
#67088=CARTESIAN_POINT('Ctrl Pts',(38.9577679347267,875.263774022378,143.824633567473));
#67089=CARTESIAN_POINT('Ctrl Pts',(38.984895821811,875.372543450952,143.885386157237));
#67090=CARTESIAN_POINT('Ctrl Pts',(39.0844870246255,875.573527435018,143.995719560666));
#67091=CARTESIAN_POINT('Ctrl Pts',(39.1551805947154,875.664229356601,144.044498187797));
#67092=CARTESIAN_POINT('Ctrl Pts',(39.3309860528678,875.816648737464,144.123676489077));
#67093=CARTESIAN_POINT('Ctrl Pts',(39.4338855056939,875.877241726121,144.153527221637));
#67094=CARTESIAN_POINT('Ctrl Pts',(39.6600704936404,875.961350771491,144.190529796745));
#67095=CARTESIAN_POINT('Ctrl Pts',(39.7809437428096,875.983935484909,144.197263668013));
#67096=CARTESIAN_POINT('Ctrl Pts',(39.9029229553107,875.985831224642,144.191899892559));
#67097=CARTESIAN_POINT('',(39.9029229553206,876.681439899921,142.223755915584));
#67098=CARTESIAN_POINT('',(39.9029229553071,879.843214503607,133.277881799942));
#67099=CARTESIAN_POINT('Ctrl Pts',(39.6760609074945,876.65417024943,142.218260294109));
#67100=CARTESIAN_POINT('Ctrl Pts',(39.7910221966015,876.680882462951,142.227701294197));
#67101=CARTESIAN_POINT('Ctrl Pts',(39.9101962652796,876.688090144837,142.226900955887));
#67102=CARTESIAN_POINT('Ctrl Pts',(40.1511897857589,876.662163668026,142.204459717129));
#67103=CARTESIAN_POINT('Ctrl Pts',(40.2702959128896,876.627025544152,142.181895352544));
#67104=CARTESIAN_POINT('Ctrl Pts',(40.4838531659849,876.518356349961,142.118282167906));
#67105=CARTESIAN_POINT('Ctrl Pts',(40.5766917966377,876.446513653426,142.078160989779));
#67106=CARTESIAN_POINT('Ctrl Pts',(40.7275801369447,876.273574159347,141.984804240418));
#67107=CARTESIAN_POINT('Ctrl Pts',(40.7836705291662,876.173605613701,141.932226879937));
#67108=CARTESIAN_POINT('Ctrl Pts',(40.8501072195456,875.958049970237,141.821449951645));
#67109=CARTESIAN_POINT('Ctrl Pts',(40.8592663423443,875.844279312972,141.764214965779));
#67110=CARTESIAN_POINT('Ctrl Pts',(40.8277383758783,875.619026529051,141.653147811411));
#67111=CARTESIAN_POINT('Ctrl Pts',(40.7872359723692,875.509720651974,141.600388984095));
#67112=CARTESIAN_POINT('Ctrl Pts',(40.663783447529,875.315200899285,141.508486215769));
#67113=CARTESIAN_POINT('Ctrl Pts',(40.5838356488444,875.230974193866,141.469708973292));
#67114=CARTESIAN_POINT('Ctrl Pts',(40.3963738851674,875.096072584928,141.409563952035));
#67115=CARTESIAN_POINT('Ctrl Pts',(40.2915390894419,875.045593721648,141.388199163957));
#67116=CARTESIAN_POINT('Ctrl Pts',(40.0664827440692,874.981427291455,141.363915143875));
#67117=CARTESIAN_POINT('Ctrl Pts',(39.9482454741537,874.968535329637,141.361321391245));
#67118=CARTESIAN_POINT('Ctrl Pts',(39.7100467845826,874.982723789839,141.375787532497));
#67119=CARTESIAN_POINT('Ctrl Pts',(39.5924110863674,875.010729959418,141.393232180506));
#67120=CARTESIAN_POINT('Ctrl Pts',(39.3700861925856,875.107486650575,141.447995546985));
#67121=CARTESIAN_POINT('Ctrl Pts',(39.2687030524731,875.177294506076,141.485749791744));
#67122=CARTESIAN_POINT('Ctrl Pts',(39.1048090734562,875.346649486077,141.575268679262));
#67123=CARTESIAN_POINT('Ctrl Pts',(39.0430175481789,875.44388802455,141.625857307291));
#67124=CARTESIAN_POINT('Ctrl Pts',(38.964058400758,875.655719874202,141.734846155825));
#67125=CARTESIAN_POINT('Ctrl Pts',(38.9482540786183,875.768565996308,141.792332859536));
#67126=CARTESIAN_POINT('Ctrl Pts',(38.9664783374583,875.994635706068,141.906313971592));
#67127=CARTESIAN_POINT('Ctrl Pts',(39.0007884414862,876.105719976912,141.961713977259));
#67128=CARTESIAN_POINT('Ctrl Pts',(39.1100352276555,876.299236885488,142.056732204963));
#67129=CARTESIAN_POINT('Ctrl Pts',(39.1795085028925,876.381910390205,142.09663159444));
#67130=CARTESIAN_POINT('Ctrl Pts',(39.352031492848,876.525198211704,142.163927728593));
#67131=CARTESIAN_POINT('Ctrl Pts',(39.4549821501028,876.58315265103,142.189959201952));
#67132=CARTESIAN_POINT('Ctrl Pts',(39.6027223966637,876.635011562805,142.211143647796));
#67133=CARTESIAN_POINT('Ctrl Pts',(39.6390991567632,876.645581878637,142.215224873276));
#67134=CARTESIAN_POINT('Ctrl Pts',(39.6760609074945,876.65417024943,142.218260294109));
#67135=CARTESIAN_POINT('Ctrl Pts',(39.9029229553107,875.985831224642,144.191899892559));
#67136=CARTESIAN_POINT('Ctrl Pts',(39.9030874038895,875.985833780419,144.191892661284));
#67137=CARTESIAN_POINT('Ctrl Pts',(39.9032518544797,875.985836298579,144.191885408044));
#67138=CARTESIAN_POINT('Ctrl Pts',(39.903416307065,875.98583877912,144.191878132838));
#67139=CARTESIAN_POINT('Ctrl Pts',(40.0251817976164,875.987675443772,144.186491358095));
#67140=CARTESIAN_POINT('Ctrl Pts',(40.1454673356734,875.968858913891,144.169170410953));
#67141=CARTESIAN_POINT('Ctrl Pts',(40.3747002237885,875.890893894539,144.112074599829));
#67142=CARTESIAN_POINT('Ctrl Pts',(40.4806317218925,875.830953575662,144.072022552572));
#67143=CARTESIAN_POINT('Ctrl Pts',(40.6609684533752,875.676257671763,143.974339399571));
#67144=CARTESIAN_POINT('Ctrl Pts',(40.7328104936842,875.582157529378,143.917245070734));
#67145=CARTESIAN_POINT('Ctrl Pts',(40.8287772622849,875.374989520591,143.795799754419));
#67146=CARTESIAN_POINT('Ctrl Pts',(40.852578328741,875.263981598242,143.732618331064));
#67147=CARTESIAN_POINT('Ctrl Pts',(40.8492990764597,875.040632595631,143.608970566394));
#67148=CARTESIAN_POINT('Ctrl Pts',(40.822962703033,874.930358621375,143.549594774218));
#67149=CARTESIAN_POINT('Ctrl Pts',(40.7236050577374,874.724818305239,143.441853751764));
#67150=CARTESIAN_POINT('Ctrl Pts',(40.6519180075985,874.631458998882,143.39445059914));
#67151=CARTESIAN_POINT('Ctrl Pts',(40.473614022833,874.475647779633,143.31810069937));
#67152=CARTESIAN_POINT('Ctrl Pts',(40.3695340826542,874.41417502236,143.28955402088));
#67153=CARTESIAN_POINT('Ctrl Pts',(40.1431929620499,874.330531654497,143.254288726939));
#67154=CARTESIAN_POINT('Ctrl Pts',(40.0235798236697,874.308490328937,143.247524034764));
#67155=CARTESIAN_POINT('Ctrl Pts',(39.9029229553071,874.306969838757,143.251826085178));
#67156=CARTESIAN_POINT('Origin',(39.9029229553071,878.949318330988,132.961948646806));
#67157=CARTESIAN_POINT('',(39.9029229553071,877.285901699482,139.168843890294));
#67158=CARTESIAN_POINT('Origin',(39.9029229553071,876.814479468873,139.002227323027));
#67159=CARTESIAN_POINT('',(39.9029229553073,875.591487946798,143.962990858787));
#67160=CARTESIAN_POINT('',(39.9029229553071,879.420740561597,133.128565214073));
#67161=CARTESIAN_POINT('Ctrl Pts',(39.9029125861287,874.706111633602,143.46715827259));
#67162=CARTESIAN_POINT('Ctrl Pts',(39.8394125814979,874.705266289056,143.469554028673));
#67163=CARTESIAN_POINT('Ctrl Pts',(39.776620906851,874.715175936815,143.477814522341));
#67164=CARTESIAN_POINT('Ctrl Pts',(39.6560352456007,874.756218438025,143.505866775024));
#67165=CARTESIAN_POINT('Ctrl Pts',(39.5999333149543,874.787994049393,143.525943440243));
#67166=CARTESIAN_POINT('Ctrl Pts',(39.5051137443104,874.86924503659,143.575310541464));
#67167=CARTESIAN_POINT('Ctrl Pts',(39.4674503889586,874.918056839898,143.604189947962));
#67168=CARTESIAN_POINT('Ctrl Pts',(39.4159003605091,875.026297036297,143.667051502762));
#67169=CARTESIAN_POINT('Ctrl Pts',(39.4026875151781,875.084826141436,143.700503306233));
#67170=CARTESIAN_POINT('Ctrl Pts',(39.4031600074572,875.202109358987,143.766523330033));
#67171=CARTESIAN_POINT('Ctrl Pts',(39.4163122704492,875.259821781453,143.798523025633));
#67172=CARTESIAN_POINT('Ctrl Pts',(39.466789581369,875.36696636881,143.856818331159));
#67173=CARTESIAN_POINT('Ctrl Pts',(39.5032188927284,875.415560110795,143.882675862872));
#67174=CARTESIAN_POINT('Ctrl Pts',(39.5946098126277,875.497644378116,143.924914833303));
#67175=CARTESIAN_POINT('Ctrl Pts',(39.6484193347918,875.530516057664,143.940997221764));
#67176=CARTESIAN_POINT('Ctrl Pts',(39.7671645023835,875.576691676965,143.961401618141));
#67177=CARTESIAN_POINT('Ctrl Pts',(39.8308435880341,875.589497549965,143.965501203725));
#67178=CARTESIAN_POINT('Ctrl Pts',(39.9606812981915,875.593175112385,143.961031974467));
#67179=CARTESIAN_POINT('Ctrl Pts',(40.0254550063193,875.583696188365,143.952334245958));
#67180=CARTESIAN_POINT('Ctrl Pts',(40.1479332230503,875.542958292175,143.922963072296));
#67181=CARTESIAN_POINT('Ctrl Pts',(40.2041732943436,875.511641195688,143.902335419013));
#67182=CARTESIAN_POINT('Ctrl Pts',(40.2998867208973,875.43074791286,143.851772613677));
#67183=CARTESIAN_POINT('Ctrl Pts',(40.3381061536731,875.381620484094,143.822161237435));
#67184=CARTESIAN_POINT('Ctrl Pts',(40.3898919840359,875.273017444946,143.758620287658));
#67185=CARTESIAN_POINT('Ctrl Pts',(40.4031198235907,875.214565922328,143.725282428387));
#67186=CARTESIAN_POINT('Ctrl Pts',(40.4027233846304,875.096514204187,143.659534746794));
#67187=CARTESIAN_POINT('Ctrl Pts',(40.3893338580669,875.037997724845,143.627713405857));
#67188=CARTESIAN_POINT('Ctrl Pts',(40.3375528663649,874.928767732513,143.569742176593));
#67189=CARTESIAN_POINT('Ctrl Pts',(40.299830830971,874.879075145497,143.544120454941));
#67190=CARTESIAN_POINT('Ctrl Pts',(40.2060206396531,874.796466898826,143.503003556349));
#67191=CARTESIAN_POINT('Ctrl Pts',(40.1514502513785,874.763924057369,143.487638595844));
#67192=CARTESIAN_POINT('Ctrl Pts',(40.031578849116,874.718958482736,143.468406330896));
#67193=CARTESIAN_POINT('Ctrl Pts',(39.9675407015733,874.706971996137,143.464719954647));
#67194=CARTESIAN_POINT('Ctrl Pts',(39.9029125861287,874.706111633602,143.46715827259));
#67195=CARTESIAN_POINT('Origin',(56.6615834797138,876.392836831737,132.058401584256));
#67196=CARTESIAN_POINT('',(56.6615834797139,871.826484696526,141.913218520128));
#67197=CARTESIAN_POINT('',(56.6615834797138,873.701900949848,142.737238421883));
#67198=CARTESIAN_POINT('Ctrl Pts',(56.6615834797139,871.826484696526,141.913218520128));
#67199=CARTESIAN_POINT('Ctrl Pts',(56.6609946908177,871.826485410375,141.913216500375));
#67200=CARTESIAN_POINT('Ctrl Pts',(56.6604058766319,871.826486596065,141.913214673391));
#67201=CARTESIAN_POINT('Ctrl Pts',(56.5249017417484,871.826868056857,141.912838616704));
#67202=CARTESIAN_POINT('Ctrl Pts',(56.3913631648341,871.85202727222,141.922567460365));
#67203=CARTESIAN_POINT('Ctrl Pts',(56.1429026589535,871.948751438092,141.961234954755));
#67204=CARTESIAN_POINT('Ctrl Pts',(56.0303721644293,872.019212471289,141.989744021337));
#67205=CARTESIAN_POINT('Ctrl Pts',(55.8412133365598,872.1960898603,142.062545795087));
#67206=CARTESIAN_POINT('Ctrl Pts',(55.7664566066399,872.300752572678,142.106137665102));
#67207=CARTESIAN_POINT('Ctrl Pts',(55.66455851989,872.531309682226,142.203863605437));
#67208=CARTESIAN_POINT('Ctrl Pts',(55.638908707713,872.655089391935,142.257131608936));
#67209=CARTESIAN_POINT('Ctrl Pts',(55.6415222063443,872.902456466717,142.365462442173));
#67210=CARTESIAN_POINT('Ctrl Pts',(55.6691223250622,873.023665489806,142.419460728698));
#67211=CARTESIAN_POINT('Ctrl Pts',(55.773569354643,873.248580449788,142.521253485098));
#67212=CARTESIAN_POINT('Ctrl Pts',(55.8493012069038,873.350237199982,142.568103286156));
#67213=CARTESIAN_POINT('Ctrl Pts',(56.0389867145052,873.520509358991,142.647720348297));
#67214=CARTESIAN_POINT('Ctrl Pts',(56.150978431199,873.58768400378,142.679790881428));
#67215=CARTESIAN_POINT('Ctrl Pts',(56.3970138101901,873.678948589189,142.724285393482));
#67216=CARTESIAN_POINT('Ctrl Pts',(56.5286286481765,873.702232170148,142.736301272505));
#67217=CARTESIAN_POINT('Ctrl Pts',(56.6615834797138,873.701900949848,142.737238421883));
#67218=CARTESIAN_POINT('',(56.6615834794499,874.348423453521,140.907978067888));
#67219=CARTESIAN_POINT('',(56.6615834797138,877.355865971979,132.398768667323));
#67220=CARTESIAN_POINT('Ctrl Pts',(56.7387604601335,874.345589290753,140.907234680149));
#67221=CARTESIAN_POINT('Ctrl Pts',(56.8715601059757,874.336101421898,140.903881346266));
#67222=CARTESIAN_POINT('Ctrl Pts',(57.0010812807415,874.30294766371,140.889846776181));
#67223=CARTESIAN_POINT('Ctrl Pts',(57.2389967355791,874.193058379317,140.84215655939));
#67224=CARTESIAN_POINT('Ctrl Pts',(57.3450693350082,874.11739169635,140.808970813782));
#67225=CARTESIAN_POINT('Ctrl Pts',(57.5199811258611,873.932726670759,140.72785146709));
#67226=CARTESIAN_POINT('Ctrl Pts',(57.5869752716837,873.825354129399,140.680640544959));
#67227=CARTESIAN_POINT('Ctrl Pts',(57.6723540791752,873.592536847775,140.578590321866));
#67228=CARTESIAN_POINT('Ctrl Pts',(57.6897125127079,873.469229935417,140.524696557824));
#67229=CARTESIAN_POINT('Ctrl Pts',(57.6715963313277,873.223231944225,140.41765671954));
#67230=CARTESIAN_POINT('Ctrl Pts',(57.6362382527093,873.10289391739,140.365536018464));
#67231=CARTESIAN_POINT('Ctrl Pts',(57.5174524273053,872.882569984974,140.270456748966));
#67232=CARTESIAN_POINT('Ctrl Pts',(57.4356125490153,872.78450254126,140.228316149903));
#67233=CARTESIAN_POINT('Ctrl Pts',(57.234311545603,872.62171128422,140.158375809575));
#67234=CARTESIAN_POINT('Ctrl Pts',(57.1163746955299,872.559042171161,140.131448684077));
#67235=CARTESIAN_POINT('Ctrl Pts',(56.8605865096311,872.479583634516,140.09687445237));
#67236=CARTESIAN_POINT('Ctrl Pts',(56.7252546257234,872.463662685499,140.089595976134));
#67237=CARTESIAN_POINT('Ctrl Pts',(56.4569713081032,872.481353135161,140.09575220826));
#67238=CARTESIAN_POINT('Ctrl Pts',(56.326634234563,872.514301970465,140.108922185502));
#67239=CARTESIAN_POINT('Ctrl Pts',(56.087162461522,872.624617497883,140.154092459123));
#67240=CARTESIAN_POINT('Ctrl Pts',(55.9803492034041,872.700870958704,140.185643911285));
#67241=CARTESIAN_POINT('Ctrl Pts',(55.804846533169,872.886440043867,140.263306364565));
#67242=CARTESIAN_POINT('Ctrl Pts',(55.7377228556858,872.993849122406,140.308626999117));
#67243=CARTESIAN_POINT('Ctrl Pts',(55.6515214168156,873.226929597842,140.408008618885));
#67244=CARTESIAN_POINT('Ctrl Pts',(55.6336876419626,873.350485579954,140.461182409555));
#67245=CARTESIAN_POINT('Ctrl Pts',(55.650956415818,873.597922741854,140.568766727364));
#67246=CARTESIAN_POINT('Ctrl Pts',(55.6865202510053,873.719371085996,140.622132233908));
#67247=CARTESIAN_POINT('Ctrl Pts',(55.806589945394,873.94090153433,140.72044023561));
#67248=CARTESIAN_POINT('Ctrl Pts',(55.8894138540945,874.039091148948,140.764524113048));
#67249=CARTESIAN_POINT('Ctrl Pts',(56.0917791670309,874.20023448107,140.837621990316));
#67250=CARTESIAN_POINT('Ctrl Pts',(56.2093174127696,874.261675376655,140.865939338036));
#67251=CARTESIAN_POINT('Ctrl Pts',(56.4007211769631,874.320086557591,140.893448918861));
#67252=CARTESIAN_POINT('Ctrl Pts',(56.4668439595631,874.333772072963,140.900052314879));
#67253=CARTESIAN_POINT('Ctrl Pts',(56.6018968193636,874.349051846478,140.907848627408));
#67254=CARTESIAN_POINT('Ctrl Pts',(56.6704997132709,874.350466178866,140.908958337422));
#67255=CARTESIAN_POINT('Ctrl Pts',(56.7387604601335,874.345589290753,140.907234680149));
#67256=CARTESIAN_POINT('Ctrl Pts',(56.6615834797139,873.701900949848,142.737238421883));
#67257=CARTESIAN_POINT('Ctrl Pts',(56.6615908286669,873.701900931541,142.737238473683));
#67258=CARTESIAN_POINT('Ctrl Pts',(56.6615981776241,873.701900913178,142.737238525457));
#67259=CARTESIAN_POINT('Ctrl Pts',(56.6616055265853,873.701900894726,142.73723857719));
#67260=CARTESIAN_POINT('Ctrl Pts',(56.7920552216792,873.701573353253,142.73815686803));
#67261=CARTESIAN_POINT('Ctrl Pts',(56.9212693873624,873.678518937705,142.728390846398));
#67262=CARTESIAN_POINT('Ctrl Pts',(57.1668593346475,873.588131091588,142.68812134135));
#67263=CARTESIAN_POINT('Ctrl Pts',(57.2802745242113,873.520412040137,142.657423550219));
#67264=CARTESIAN_POINT('Ctrl Pts',(57.4723085051569,873.348581722697,142.579476613341));
#67265=CARTESIAN_POINT('Ctrl Pts',(57.5489049042427,873.245991264003,142.532933896641));
#67266=CARTESIAN_POINT('Ctrl Pts',(57.6541627852097,873.019492886243,142.430970318421));
#67267=CARTESIAN_POINT('Ctrl Pts',(57.681832787815,872.897736939774,142.376533693577));
#67268=CARTESIAN_POINT('Ctrl Pts',(57.6840938909722,872.649461894248,142.266717717683));
#67269=CARTESIAN_POINT('Ctrl Pts',(57.6579766086863,872.52533699858,142.212418898586));
#67270=CARTESIAN_POINT('Ctrl Pts',(57.554839527277,872.294897300328,142.112675071343));
#67271=CARTESIAN_POINT('Ctrl Pts',(57.4794877508656,872.190634193339,142.068093323857));
#67272=CARTESIAN_POINT('Ctrl Pts',(57.2894177385193,872.015132848579,141.993539452835));
#67273=CARTESIAN_POINT('Ctrl Pts',(57.176705659342,871.945522323037,141.964236815098));
#67274=CARTESIAN_POINT('Ctrl Pts',(56.9286459505039,871.850676119467,141.924128858445));
#67275=CARTESIAN_POINT('Ctrl Pts',(56.7957714512608,871.826322006757,141.913678831938));
#67276=CARTESIAN_POINT('Ctrl Pts',(56.6615834797138,871.826484696526,141.913218520128));
#67277=CARTESIAN_POINT('Origin',(56.6615834797138,876.392836831737,132.058401584256));
#67278=CARTESIAN_POINT('',(56.6615834797138,874.72942020023,138.265296827744));
#67279=CARTESIAN_POINT('Origin',(56.6615834797138,874.257997969622,138.098680260477));
#67280=CARTESIAN_POINT('',(56.661583479714,873.226683339969,142.517116285449));
#67281=CARTESIAN_POINT('',(56.6615834797138,876.864259062345,132.225018151523));
#67282=CARTESIAN_POINT('Ctrl Pts',(56.6615880190493,872.308665685004,142.113638585422));
#67283=CARTESIAN_POINT('Ctrl Pts',(56.6001364053008,872.308760865999,142.113367607646));
#67284=CARTESIAN_POINT('Ctrl Pts',(56.5392115878473,872.319304548476,142.117531372034));
#67285=CARTESIAN_POINT('Ctrl Pts',(56.419937753833,872.361849860724,142.13501247575));
#67286=CARTESIAN_POINT('Ctrl Pts',(56.3633877006692,872.395075829848,142.148862821418));
#67287=CARTESIAN_POINT('Ctrl Pts',(56.2676088882711,872.479846325149,142.184639702097));
#67288=CARTESIAN_POINT('Ctrl Pts',(56.2293515484587,872.530550570378,142.20621675157));
#67289=CARTESIAN_POINT('Ctrl Pts',(56.1763997004844,872.642841587476,142.254503154028));
#67290=CARTESIAN_POINT('Ctrl Pts',(56.1623578613256,872.703358814639,142.280758867163));
#67291=CARTESIAN_POINT('Ctrl Pts',(56.1608827404138,872.824741915519,142.333957573825));
#67292=CARTESIAN_POINT('Ctrl Pts',(56.173059875041,872.884430875959,142.360376943219));
#67293=CARTESIAN_POINT('Ctrl Pts',(56.2217698082996,872.995794763792,142.410142111349));
#67294=CARTESIAN_POINT('Ctrl Pts',(56.2577798059143,873.046441122238,142.433024237972));
#67295=CARTESIAN_POINT('Ctrl Pts',(56.348953330183,873.131911631132,142.47202087607));
#67296=CARTESIAN_POINT('Ctrl Pts',(56.4031767949244,873.165985195154,142.487787017585));
#67297=CARTESIAN_POINT('Ctrl Pts',(56.5228893958498,873.213074591051,142.509939180269));
#67298=CARTESIAN_POINT('Ctrl Pts',(56.5871943248138,873.225672192475,142.516124114616));
#67299=CARTESIAN_POINT('Ctrl Pts',(56.7177050294111,873.227581857597,142.517926403236));
#67300=CARTESIAN_POINT('Ctrl Pts',(56.7826190887181,873.216829601136,142.513504494232));
#67301=CARTESIAN_POINT('Ctrl Pts',(56.9045621441444,873.173036841854,142.494512977799));
#67302=CARTESIAN_POINT('Ctrl Pts',(56.9603425420374,873.140333886772,142.480089924366));
#67303=CARTESIAN_POINT('Ctrl Pts',(57.0551120863392,873.056999087507,142.443174197959));
#67304=CARTESIAN_POINT('Ctrl Pts',(57.0931127660954,873.007115390226,142.421016670206));
#67305=CARTESIAN_POINT('Ctrl Pts',(57.1459059727482,872.896715691287,142.372072783374));
#67306=CARTESIAN_POINT('Ctrl Pts',(57.160170788179,872.837245341146,142.345753833874));
#67307=CARTESIAN_POINT('Ctrl Pts',(57.1628182600068,872.715622211842,142.292131004574));
#67308=CARTESIAN_POINT('Ctrl Pts',(57.1507466719065,872.654639799362,142.265347796493));
#67309=CARTESIAN_POINT('Ctrl Pts',(57.1013501009362,872.540958533665,142.215589777814));
#67310=CARTESIAN_POINT('Ctrl Pts',(57.0646859878445,872.489327069808,142.193078327265));
#67311=CARTESIAN_POINT('Ctrl Pts',(56.9716045235116,872.402334668021,142.155167421734));
#67312=CARTESIAN_POINT('Ctrl Pts',(56.9161654721059,872.367800826181,142.140123523712));
#67313=CARTESIAN_POINT('Ctrl Pts',(56.7937562436668,872.320668501759,142.119399429729));
#67314=CARTESIAN_POINT('Ctrl Pts',(56.7280090715558,872.308562806958,142.113931476494));
#67315=CARTESIAN_POINT('Ctrl Pts',(56.6615880190493,872.308665685004,142.113638585422));
#67316=CARTESIAN_POINT('Origin',(51.1325126856635,880.408005670941,133.477498108665));
#67317=CARTESIAN_POINT('',(51.1325126856635,875.766823207888,143.764076402871));
#67318=CARTESIAN_POINT('',(51.1325126856635,877.442441730773,144.713325514568));
#67319=CARTESIAN_POINT('Ctrl Pts',(51.1325126856636,875.766823207888,143.764076402872));
#67320=CARTESIAN_POINT('Ctrl Pts',(51.131304761973,875.76682116675,143.764082178035));
#67321=CARTESIAN_POINT('Ctrl Pts',(51.1300967200539,875.766821180395,143.764089066902));
#67322=CARTESIAN_POINT('Ctrl Pts',(51.0035143611211,875.767038023791,143.76492759062));
#67323=CARTESIAN_POINT('Ctrl Pts',(50.8796062726843,875.789394490415,143.777723613443));
#67324=CARTESIAN_POINT('Ctrl Pts',(50.6488971671256,875.875493431376,143.825893678785));
#67325=CARTESIAN_POINT('Ctrl Pts',(50.5445508589289,875.938360214591,143.860790059619));
#67326=CARTESIAN_POINT('Ctrl Pts',(50.368954885655,876.09635398233,143.948721147385));
#67327=CARTESIAN_POINT('Ctrl Pts',(50.2997265485965,876.190109963413,144.001008999435));
#67328=CARTESIAN_POINT('Ctrl Pts',(50.2057276920398,876.396696616052,144.116947363144));
#67329=CARTESIAN_POINT('Ctrl Pts',(50.1825030142982,876.507816098029,144.179655123601));
#67330=CARTESIAN_POINT('Ctrl Pts',(50.1865848263252,876.730024323512,144.305847924143));
#67331=CARTESIAN_POINT('Ctrl Pts',(50.2134090577556,876.839168716171,144.368218448869));
#67332=CARTESIAN_POINT('Ctrl Pts',(50.3129358731998,877.040239015299,144.483589935969));
#67333=CARTESIAN_POINT('Ctrl Pts',(50.3840082053844,877.130689213192,144.535725492343));
#67334=CARTESIAN_POINT('Ctrl Pts',(50.5606018229957,877.281309892263,144.622514965763));
#67335=CARTESIAN_POINT('Ctrl Pts',(50.6638280461508,877.340603774865,144.656653127129));
#67336=CARTESIAN_POINT('Ctrl Pts',(50.8900959243223,877.421328513706,144.702583717026));
#67337=CARTESIAN_POINT('Ctrl Pts',(51.0106612922889,877.442186253871,144.714048356799));
#67338=CARTESIAN_POINT('Ctrl Pts',(51.1325126856635,877.442441730773,144.713325514568));
#67339=CARTESIAN_POINT('',(51.1325126856326,878.138848987347,142.742922044547));
#67340=CARTESIAN_POINT('',(51.1325126856635,881.30190184356,133.793431261802));
#67341=CARTESIAN_POINT('Ctrl Pts',(51.1019995799007,878.138362681097,142.742824118366));
#67342=CARTESIAN_POINT('Ctrl Pts',(51.2203391425413,878.141955492694,142.744093939551));
#67343=CARTESIAN_POINT('Ctrl Pts',(51.3382664322453,878.125667154056,142.73498931258));
#67344=CARTESIAN_POINT('Ctrl Pts',(51.5673565428978,878.053156825002,142.696083764234));
#67345=CARTESIAN_POINT('Ctrl Pts',(51.6754085173438,877.995508026985,142.66556336574));
#67346=CARTESIAN_POINT('Ctrl Pts',(51.8585894689507,877.847523288319,142.588054737409));
#67347=CARTESIAN_POINT('Ctrl Pts',(51.9325364267539,877.759152649319,142.542092025178));
#67348=CARTESIAN_POINT('Ctrl Pts',(52.0397584032032,877.5606352111,142.439695164907));
#67349=CARTESIAN_POINT('Ctrl Pts',(52.07138369246,877.451974309298,142.384045631647));
#67350=CARTESIAN_POINT('Ctrl Pts',(52.0864385917891,877.228343098163,142.270414524496));
#67351=CARTESIAN_POINT('Ctrl Pts',(52.0691298722353,877.115380041048,142.21346497185));
#67352=CARTESIAN_POINT('Ctrl Pts',(51.9864398549688,876.901445910502,142.10639821256));
#67353=CARTESIAN_POINT('Ctrl Pts',(51.9217401782439,876.802565238296,142.057324005392));
#67354=CARTESIAN_POINT('Ctrl Pts',(51.7564866886615,876.636655369949,141.975532938231));
#67355=CARTESIAN_POINT('Ctrl Pts',(51.6590885098741,876.570003109294,141.942967099181));
#67356=CARTESIAN_POINT('Ctrl Pts',(51.4451116594363,876.474882841051,141.89688214976));
#67357=CARTESIAN_POINT('Ctrl Pts',(51.3311922474334,876.446081851696,141.883179055817));
#67358=CARTESIAN_POINT('Ctrl Pts',(51.0967930100967,876.427446066606,141.874987106281));
#67359=CARTESIAN_POINT('Ctrl Pts',(50.9784326146121,876.438000210876,141.880680000862));
#67360=CARTESIAN_POINT('Ctrl Pts',(50.7492227374605,876.498507432607,141.911516759673));
#67361=CARTESIAN_POINT('Ctrl Pts',(50.6408562843865,876.548909725185,141.936876955342));
#67362=CARTESIAN_POINT('Ctrl Pts',(50.4461509548119,876.686992837895,142.006246477512));
#67363=CARTESIAN_POINT('Ctrl Pts',(50.3632833305802,876.775059381454,142.050453960429));
#67364=CARTESIAN_POINT('Ctrl Pts',(50.2423713544919,876.972637761829,142.149947952602));
#67365=CARTESIAN_POINT('Ctrl Pts',(50.2044965712362,877.079752927103,142.204027314726));
#67366=CARTESIAN_POINT('Ctrl Pts',(50.1763390076605,877.302199715689,142.316767841845));
#67367=CARTESIAN_POINT('Ctrl Pts',(50.1869839460711,877.415557116966,142.374435248914));
#67368=CARTESIAN_POINT('Ctrl Pts',(50.2570230022145,877.632880201761,142.485325007758));
#67369=CARTESIAN_POINT('Ctrl Pts',(50.3161973006486,877.734700453816,142.537450795729));
#67370=CARTESIAN_POINT('Ctrl Pts',(50.4675747436943,877.902390297205,142.623340864716));
#67371=CARTESIAN_POINT('Ctrl Pts',(50.5545005668584,877.969565128902,142.657762498737));
#67372=CARTESIAN_POINT('Ctrl Pts',(50.7560044783514,878.075788026719,142.711958634738));
#67373=CARTESIAN_POINT('Ctrl Pts',(50.8698696721942,878.112256677342,142.730396303378));
#67374=CARTESIAN_POINT('Ctrl Pts',(51.0260149820039,878.134001458524,142.740937396534));
#67375=CARTESIAN_POINT('Ctrl Pts',(51.06395166438,878.137207539156,142.742415852119));
#67376=CARTESIAN_POINT('Ctrl Pts',(51.1019995799007,878.138362681097,142.742824118366));
#67377=CARTESIAN_POINT('Ctrl Pts',(51.1325126856635,877.442441730773,144.713325514568));
#67378=CARTESIAN_POINT('Ctrl Pts',(51.1325199189838,877.442441745939,144.713325471659));
#67379=CARTESIAN_POINT('Ctrl Pts',(51.1325271523087,877.442441761051,144.713325428718));
#67380=CARTESIAN_POINT('Ctrl Pts',(51.1325343856381,877.442441776071,144.713325385723));
#67381=CARTESIAN_POINT('Ctrl Pts',(51.2516981149903,877.442689224519,144.712617074273));
#67382=CARTESIAN_POINT('Ctrl Pts',(51.3696091813458,877.423228035679,144.700269032771));
#67383=CARTESIAN_POINT('Ctrl Pts',(51.5966068087232,877.345147660409,144.652704913418));
#67384=CARTESIAN_POINT('Ctrl Pts',(51.702440326515,877.285339664995,144.616826217988));
#67385=CARTESIAN_POINT('Ctrl Pts',(51.8830714745084,877.131995260537,144.526111613188));
#67386=CARTESIAN_POINT('Ctrl Pts',(51.9554005077383,877.039315262831,144.4718160893));
#67387=CARTESIAN_POINT('Ctrl Pts',(52.0549496786397,876.833373267989,144.352618105642));
#67388=CARTESIAN_POINT('Ctrl Pts',(52.0806897870562,876.721757332879,144.288695108183));
#67389=CARTESIAN_POINT('Ctrl Pts',(52.0805052844136,876.497473999723,144.161740641726));
#67390=CARTESIAN_POINT('Ctrl Pts',(52.0553007572354,876.386836737815,144.099838102673));
#67391=CARTESIAN_POINT('Ctrl Pts',(51.9577591242723,876.181490947495,143.986155335694));
#67392=CARTESIAN_POINT('Ctrl Pts',(51.8869610300829,876.088520017704,143.935310368264));
#67393=CARTESIAN_POINT('Ctrl Pts',(51.7086733206128,875.932316781655,143.850685763962));
#67394=CARTESIAN_POINT('Ctrl Pts',(51.6031935937059,875.870504288221,143.817654977638));
#67395=CARTESIAN_POINT('Ctrl Pts',(51.374417798785,875.788047198342,143.774176101606));
#67396=CARTESIAN_POINT('Ctrl Pts',(51.2540638778635,875.767028603952,143.763495258558));
#67397=CARTESIAN_POINT('Ctrl Pts',(51.1325126856636,875.766823207888,143.764076402871));
#67398=CARTESIAN_POINT('Origin',(51.1325126856635,880.408005670941,133.477498108665));
#67399=CARTESIAN_POINT('',(51.1325126856635,878.744589039435,139.684393352153));
#67400=CARTESIAN_POINT('Origin',(51.1325126856635,878.273166808826,139.517776784886));
#67401=CARTESIAN_POINT('',(51.1325126856637,877.048983671841,144.481911856674));
#67402=CARTESIAN_POINT('',(51.1325126856635,880.87942790155,133.644114675932));
#67403=CARTESIAN_POINT('Ctrl Pts',(51.132518179114,876.16532192069,143.981228116023));
#67404=CARTESIAN_POINT('Ctrl Pts',(51.0700489071742,876.165209434297,143.981544323559));
#67405=CARTESIAN_POINT('Ctrl Pts',(51.0081976721465,876.175483592962,143.987602863164));
#67406=CARTESIAN_POINT('Ctrl Pts',(50.8882236513185,876.216940393256,144.011329545291));
#67407=CARTESIAN_POINT('Ctrl Pts',(50.8319197675561,876.249025053008,144.029491946118));
#67408=CARTESIAN_POINT('Ctrl Pts',(50.7365787284554,876.330774521863,144.075669314888));
#67409=CARTESIAN_POINT('Ctrl Pts',(50.6986313258318,876.379724500401,144.103284129777));
#67410=CARTESIAN_POINT('Ctrl Pts',(50.64635605161,876.488046712534,144.164492131436));
#67411=CARTESIAN_POINT('Ctrl Pts',(50.6327518447176,876.546490912549,144.197564296028));
#67412=CARTESIAN_POINT('Ctrl Pts',(50.6322781683162,876.664860241963,144.264690198484));
#67413=CARTESIAN_POINT('Ctrl Pts',(50.6455958134439,876.723721799899,144.298141347072));
#67414=CARTESIAN_POINT('Ctrl Pts',(50.6970449321914,876.831543867453,144.359477076571));
#67415=CARTESIAN_POINT('Ctrl Pts',(50.7339016926261,876.879821070422,144.386967878652));
#67416=CARTESIAN_POINT('Ctrl Pts',(50.8261041217096,876.960595270929,144.432870441603));
#67417=CARTESIAN_POINT('Ctrl Pts',(50.8802560923006,876.992589386614,144.450994984563));
#67418=CARTESIAN_POINT('Ctrl Pts',(50.9992790929795,877.036556088749,144.475618667509));
#67419=CARTESIAN_POINT('Ctrl Pts',(51.0628484643923,877.048220200473,144.481945783096));
#67420=CARTESIAN_POINT('Ctrl Pts',(51.1921045903496,877.049682395447,144.481909272916));
#67421=CARTESIAN_POINT('Ctrl Pts',(51.2564043337221,877.039294826231,144.475447594556));
#67422=CARTESIAN_POINT('Ctrl Pts',(51.3778238204396,876.997203424505,144.45028083773));
#67423=CARTESIAN_POINT('Ctrl Pts',(51.4334953538068,876.965570428101,144.431629797225));
#67424=CARTESIAN_POINT('Ctrl Pts',(51.528560079656,876.884538147418,144.384356054323));
#67425=CARTESIAN_POINT('Ctrl Pts',(51.5666325811411,876.835587573722,144.356007351641));
#67426=CARTESIAN_POINT('Ctrl Pts',(51.6189829601159,876.727008300879,144.293630177779));
#67427=CARTESIAN_POINT('Ctrl Pts',(51.6325178270963,876.668274436505,144.26012346701));
#67428=CARTESIAN_POINT('Ctrl Pts',(51.6325075804319,876.549983706729,144.193137461765));
#67429=CARTESIAN_POINT('Ctrl Pts',(51.6191678203549,876.491492888902,144.160258066154));
#67430=CARTESIAN_POINT('Ctrl Pts',(51.5674031509799,876.382850200371,144.099604111257));
#67431=CARTESIAN_POINT('Ctrl Pts',(51.5296988480654,876.333643902935,144.072350455167));
#67432=CARTESIAN_POINT('Ctrl Pts',(51.4358216161833,876.252131880027,144.027518483365));
#67433=CARTESIAN_POINT('Ctrl Pts',(51.3811186186126,876.220174302848,144.010117109192));
#67434=CARTESIAN_POINT('Ctrl Pts',(51.2611370152663,876.176674159055,143.986728644173));
#67435=CARTESIAN_POINT('Ctrl Pts',(51.1971591532616,876.165438317596,143.980900915744));
#67436=CARTESIAN_POINT('Ctrl Pts',(51.132518179114,876.16532192069,143.981228116023));
#67437=CARTESIAN_POINT('Origin',(66.9612128173492,874.622216250165,131.432604360284));
#67438=CARTESIAN_POINT('',(66.9612128173492,870.055347744271,141.288882307046));
#67439=CARTESIAN_POINT('',(66.9612128173492,871.932747002821,142.107291525763));
#67440=CARTESIAN_POINT('Ctrl Pts',(66.9612128173492,870.055347744271,141.288882307046));
#67441=CARTESIAN_POINT('Ctrl Pts',(66.9607167705809,870.055350023101,141.288875859362));
#67442=CARTESIAN_POINT('Ctrl Pts',(66.9602207056299,870.055352636768,141.288869548692));
#67443=CARTESIAN_POINT('Ctrl Pts',(66.8246828860381,870.056158236702,141.287182812833));
#67444=CARTESIAN_POINT('Ctrl Pts',(66.6910009462347,870.081773298768,141.295664265099));
#67445=CARTESIAN_POINT('Ctrl Pts',(66.4420819935384,870.179635238136,141.331805000495));
#67446=CARTESIAN_POINT('Ctrl Pts',(66.3292781831525,870.250838596208,141.359081080309));
#67447=CARTESIAN_POINT('Ctrl Pts',(66.1401342703794,870.429127841465,141.429249087433));
#67448=CARTESIAN_POINT('Ctrl Pts',(66.06553555221,870.534327130104,141.47141225971));
#67449=CARTESIAN_POINT('Ctrl Pts',(65.9642432607369,870.765176303953,141.566085423473));
#67450=CARTESIAN_POINT('Ctrl Pts',(65.938731577858,870.888601867314,141.617709928411));
#67451=CARTESIAN_POINT('Ctrl Pts',(65.9409408074312,871.135922922694,141.723700049532));
#67452=CARTESIAN_POINT('Ctrl Pts',(65.9683598824257,871.257416868622,141.777030695437));
#67453=CARTESIAN_POINT('Ctrl Pts',(66.0725601507498,871.482836964578,141.878621175579));
#67454=CARTESIAN_POINT('Ctrl Pts',(66.1483333041382,871.584643845217,141.925917988167));
#67455=CARTESIAN_POINT('Ctrl Pts',(66.3382430992424,871.754720048039,142.007542624859));
#67456=CARTESIAN_POINT('Ctrl Pts',(66.4504469292104,871.821545451402,142.041148859883));
#67457=CARTESIAN_POINT('Ctrl Pts',(66.6966715784841,871.911506422729,142.089495835615));
#67458=CARTESIAN_POINT('Ctrl Pts',(66.8282588619279,871.933967163154,142.103839223781));
#67459=CARTESIAN_POINT('Ctrl Pts',(66.9612128173492,871.932747002821,142.107291525763));
#67460=CARTESIAN_POINT('',(66.9612128163858,872.578864209794,140.279177911721));
#67461=CARTESIAN_POINT('',(66.9612128173492,875.585245390407,131.772971443351));
#67462=CARTESIAN_POINT('Ctrl Pts',(67.2484589377317,872.538855492815,140.268673823591));
#67463=CARTESIAN_POINT('Ctrl Pts',(67.3762643718234,872.503542456408,140.256193001679));
#67464=CARTESIAN_POINT('Ctrl Pts',(67.4954837624301,872.445739267827,140.233446488859));
#67465=CARTESIAN_POINT('Ctrl Pts',(67.7033546503243,872.29167391827,140.170142955904));
#67466=CARTESIAN_POINT('Ctrl Pts',(67.7899772810638,872.19691172647,140.130208211362));
#67467=CARTESIAN_POINT('Ctrl Pts',(67.9192470457648,871.982103237673,140.038435144843));
#67468=CARTESIAN_POINT('Ctrl Pts',(67.9604582254089,871.86400787901,139.987434416262));
#67469=CARTESIAN_POINT('Ctrl Pts',(67.9912621529526,871.619677243159,139.881314984221));
#67470=CARTESIAN_POINT('Ctrl Pts',(67.9803356829124,871.495732942861,139.827195945714));
#67471=CARTESIAN_POINT('Ctrl Pts',(67.9069767463482,871.258799856499,139.723359951516));
#67472=CARTESIAN_POINT('Ctrl Pts',(67.8451905755019,871.148088528114,139.6746416514));
#67473=CARTESIAN_POINT('Ctrl Pts',(67.6792233773331,870.955982750718,139.589535632671));
#67474=CARTESIAN_POINT('Ctrl Pts',(67.577028264178,870.876152612627,139.55384071449));
#67475=CARTESIAN_POINT('Ctrl Pts',(67.3433687821695,870.756464611354,139.499134523185));
#67476=CARTESIAN_POINT('Ctrl Pts',(67.2138586163694,870.718316741882,139.480874034868));
#67477=CARTESIAN_POINT('Ctrl Pts',(66.945688478612,870.690780874979,139.464651031496));
#67478=CARTESIAN_POINT('Ctrl Pts',(66.8096886879856,870.701748066281,139.466875733831));
#67479=CARTESIAN_POINT('Ctrl Pts',(66.5511623574619,870.771643743234,139.49148305969));
#67480=CARTESIAN_POINT('Ctrl Pts',(66.4310448250826,870.829411865114,139.513425012589));
#67481=CARTESIAN_POINT('Ctrl Pts',(66.2215605946194,870.9842175614,139.574319617251));
#67482=CARTESIAN_POINT('Ctrl Pts',(66.1342152866182,871.079711543178,139.612671320538));
#67483=CARTESIAN_POINT('Ctrl Pts',(66.0043052718372,871.295546092716,139.701030612986));
#67484=CARTESIAN_POINT('Ctrl Pts',(65.9628435885181,871.413715648899,139.750154364426));
#67485=CARTESIAN_POINT('Ctrl Pts',(65.9311017105071,871.658483946847,139.853666856138));
#67486=CARTESIAN_POINT('Ctrl Pts',(65.9415621693557,871.782770602058,139.907098891405));
#67487=CARTESIAN_POINT('Ctrl Pts',(66.0144120578042,872.02127727974,140.01152687392));
#67488=CARTESIAN_POINT('Ctrl Pts',(66.0767033865923,872.133028475974,140.061465080283));
#67489=CARTESIAN_POINT('Ctrl Pts',(66.2443866059568,872.326043489332,140.14969476242));
#67490=CARTESIAN_POINT('Ctrl Pts',(66.3477028313432,872.405787185121,140.18725922801));
#67491=CARTESIAN_POINT('Ctrl Pts',(66.5822990889336,872.523628960054,140.245052869823));
#67492=CARTESIAN_POINT('Ctrl Pts',(66.7112749142268,872.560641064037,140.264736256022));
#67493=CARTESIAN_POINT('Ctrl Pts',(66.9118522445325,872.580208115589,140.278517007198));
#67494=CARTESIAN_POINT('Ctrl Pts',(66.9796703386908,872.580620499121,140.280429229317));
#67495=CARTESIAN_POINT('Ctrl Pts',(67.1153073912448,872.569075728989,140.27874484049));
#67496=CARTESIAN_POINT('Ctrl Pts',(67.1827652807286,872.557006853263,140.275089128541));
#67497=CARTESIAN_POINT('Ctrl Pts',(67.2484589377317,872.538855492815,140.268673823591));
#67498=CARTESIAN_POINT('Ctrl Pts',(66.9612128173492,871.932747002821,142.107291525763));
#67499=CARTESIAN_POINT('Ctrl Pts',(66.9612307903993,871.932746837877,142.107291992453));
#67500=CARTESIAN_POINT('Ctrl Pts',(66.9612487634744,871.9327466725,142.107292458946));
#67501=CARTESIAN_POINT('Ctrl Pts',(66.9612667365744,871.93274650669,142.107292925239));
#67502=CARTESIAN_POINT('Ctrl Pts',(67.0922423889351,871.931538196034,142.110690951439));
#67503=CARTESIAN_POINT('Ctrl Pts',(67.2220163544519,871.907373314964,142.103447307919));
#67504=CARTESIAN_POINT('Ctrl Pts',(67.4676160932879,871.814778012017,142.067956275113));
#67505=CARTESIAN_POINT('Ctrl Pts',(67.5806061048436,871.746340964445,142.039620789915));
#67506=CARTESIAN_POINT('Ctrl Pts',(67.7721659932508,871.573417494683,141.965567349563));
#67507=CARTESIAN_POINT('Ctrl Pts',(67.8486260601588,871.470433340403,141.920494602424));
#67508=CARTESIAN_POINT('Ctrl Pts',(67.9538488821687,871.243381924432,141.820270582023));
#67509=CARTESIAN_POINT('Ctrl Pts',(67.9814997001897,871.121447991871,141.766076742079));
#67510=CARTESIAN_POINT('Ctrl Pts',(67.9836847296759,870.873817653467,141.656031680037));
#67511=CARTESIAN_POINT('Ctrl Pts',(67.9577540254432,870.750487314886,141.60124461176));
#67512=CARTESIAN_POINT('Ctrl Pts',(67.8549834052962,870.520631288988,141.499387847567));
#67513=CARTESIAN_POINT('Ctrl Pts',(67.7793370832508,870.416290831603,141.453283907477));
#67514=CARTESIAN_POINT('Ctrl Pts',(67.5887677448977,870.241420847348,141.375854989021));
#67515=CARTESIAN_POINT('Ctrl Pts',(67.476040165905,870.172345031139,141.345159267362));
#67516=CARTESIAN_POINT('Ctrl Pts',(67.2280588525592,870.078587319634,141.302364290857));
#67517=CARTESIAN_POINT('Ctrl Pts',(67.0953000153513,870.054731750144,141.290625190902));
#67518=CARTESIAN_POINT('Ctrl Pts',(66.9612128173492,870.055347744271,141.288882307046));
#67519=CARTESIAN_POINT('Origin',(66.9612128173492,874.622216250165,131.432604360284));
#67520=CARTESIAN_POINT('',(66.9612128173492,872.958799618659,137.639499603772));
#67521=CARTESIAN_POINT('Origin',(66.9612128173492,872.48737738805,137.472883036505));
#67522=CARTESIAN_POINT('',(66.9612128173494,871.456787053482,141.889269752637));
#67523=CARTESIAN_POINT('',(66.9612128173492,875.093638480774,131.599220927551));
#67524=CARTESIAN_POINT('Ctrl Pts',(66.961219998814,870.537790077594,141.488562927539));
#67525=CARTESIAN_POINT('Ctrl Pts',(66.9010760576186,870.538139679958,141.487571175934));
#67526=CARTESIAN_POINT('Ctrl Pts',(66.841417267067,870.548499587498,141.490822681978));
#67527=CARTESIAN_POINT('Ctrl Pts',(66.7229066632556,870.590348179204,141.506242708962));
#67528=CARTESIAN_POINT('Ctrl Pts',(66.6659945502401,870.623519583751,141.519155948664));
#67529=CARTESIAN_POINT('Ctrl Pts',(66.5694917223115,870.708265316722,141.55317061355));
#67530=CARTESIAN_POINT('Ctrl Pts',(66.5308478129759,870.758961653873,141.573922734633));
#67531=CARTESIAN_POINT('Ctrl Pts',(66.4771181048806,870.871150633871,141.620724975417));
#67532=CARTESIAN_POINT('Ctrl Pts',(66.4626144142707,870.931539358277,141.646320887713));
#67533=CARTESIAN_POINT('Ctrl Pts',(66.4599960159081,871.054070501487,141.699180043191));
#67534=CARTESIAN_POINT('Ctrl Pts',(66.4720801708997,871.114998491116,141.72592794606));
#67535=CARTESIAN_POINT('Ctrl Pts',(66.5211114613292,871.227511213839,141.776284817272));
#67536=CARTESIAN_POINT('Ctrl Pts',(66.5571264439551,871.278183036104,141.799464578186));
#67537=CARTESIAN_POINT('Ctrl Pts',(66.6483699129627,871.363513524511,141.839485506655));
#67538=CARTESIAN_POINT('Ctrl Pts',(66.7026693894346,871.39742288317,141.855967463947));
#67539=CARTESIAN_POINT('Ctrl Pts',(66.8224749324693,871.443959081405,141.87984779299));
#67540=CARTESIAN_POINT('Ctrl Pts',(66.886794061751,871.456211044856,141.887043560568));
#67541=CARTESIAN_POINT('Ctrl Pts',(67.0172155558393,871.457356377065,141.891005938955));
#67542=CARTESIAN_POINT('Ctrl Pts',(67.0820358816623,871.44624419388,141.887733838793));
#67543=CARTESIAN_POINT('Ctrl Pts',(67.2037935298491,871.401823665282,141.870981604617));
#67544=CARTESIAN_POINT('Ctrl Pts',(67.2594914802127,871.368884478593,141.857635292589));
#67545=CARTESIAN_POINT('Ctrl Pts',(67.354238085846,871.285188088802,141.822575885038));
#67546=CARTESIAN_POINT('Ctrl Pts',(67.392277055294,871.235179744322,141.801175926144));
#67547=CARTESIAN_POINT('Ctrl Pts',(67.4452703769498,871.124589667198,141.753283891179));
#67548=CARTESIAN_POINT('Ctrl Pts',(67.4596537585287,871.065049570772,141.727245902082));
#67549=CARTESIAN_POINT('Ctrl Pts',(67.4625607900712,870.943208554617,141.673658737767));
#67550=CARTESIAN_POINT('Ctrl Pts',(67.4505349671018,870.882082330638,141.646623366797));
#67551=CARTESIAN_POINT('Ctrl Pts',(67.4011072470207,870.768324913195,141.596056913241));
#67552=CARTESIAN_POINT('Ctrl Pts',(67.364382532302,870.716750383278,141.572996890378));
#67553=CARTESIAN_POINT('Ctrl Pts',(67.2711975628139,870.630101118888,141.533846914187));
#67554=CARTESIAN_POINT('Ctrl Pts',(67.2157489892355,870.595812493844,141.518110357346));
#67555=CARTESIAN_POINT('Ctrl Pts',(67.0933507907198,870.54922814529,141.49590606125));
#67556=CARTESIAN_POINT('Ctrl Pts',(67.0276271002878,870.537404068975,141.489657956368));
#67557=CARTESIAN_POINT('Ctrl Pts',(66.961219998814,870.537790077594,141.488562927539));
#67558=CARTESIAN_POINT('Origin',(62.4383719093132,879.633498841219,133.203761188948));
#67559=CARTESIAN_POINT('',(62.4383719093132,874.991697703936,143.49208995005));
#67560=CARTESIAN_POINT('',(62.4383719093099,876.669038396195,144.43646638347));
#67561=CARTESIAN_POINT('Ctrl Pts',(62.4383719093132,874.991697703936,143.49208995005));
#67562=CARTESIAN_POINT('Ctrl Pts',(62.3148834011908,874.992842777131,143.488850098404));
#67563=CARTESIAN_POINT('Ctrl Pts',(62.1925701437443,875.015475261366,143.497224099113));
#67564=CARTESIAN_POINT('Ctrl Pts',(61.9623649287828,875.101797335681,143.536566557516));
#67565=CARTESIAN_POINT('Ctrl Pts',(61.857190621639,875.165174958031,143.567458486917));
#67566=CARTESIAN_POINT('Ctrl Pts',(61.680055266306,875.324104920959,143.64812062898));
#67567=CARTESIAN_POINT('Ctrl Pts',(61.6100265481437,875.418087959246,143.697116123318));
#67568=CARTESIAN_POINT('Ctrl Pts',(61.5141957614568,875.624605575474,143.807569133984));
#67569=CARTESIAN_POINT('Ctrl Pts',(61.4898086927638,875.735289692519,143.868076311795));
#67570=CARTESIAN_POINT('Ctrl Pts',(61.4907877781008,875.959014181235,143.993218927626));
#67571=CARTESIAN_POINT('Ctrl Pts',(61.5168990793443,876.069995481957,144.056748614188));
#67572=CARTESIAN_POINT('Ctrl Pts',(61.6160440799812,876.273147684721,144.175878474448));
#67573=CARTESIAN_POINT('Ctrl Pts',(61.6872214527508,876.363929798732,144.230591602814));
#67574=CARTESIAN_POINT('Ctrl Pts',(61.8644179730801,876.514100247061,144.323908367462));
#67575=CARTESIAN_POINT('Ctrl Pts',(61.9681766740616,876.57272702324,144.361962979427));
#67576=CARTESIAN_POINT('Ctrl Pts',(62.1950042018106,876.650960072077,144.416339691797));
#67577=CARTESIAN_POINT('Ctrl Pts',(62.3155571194363,876.670356145296,144.432428136869));
#67578=CARTESIAN_POINT('Ctrl Pts',(62.4375722925693,876.669047270135,144.436440263785));
#67579=CARTESIAN_POINT('Ctrl Pts',(62.4378388367372,876.669044410875,144.436449028343));
#67580=CARTESIAN_POINT('Ctrl Pts',(62.4381053756728,876.669041452892,144.436457734904));
#67581=CARTESIAN_POINT('Ctrl Pts',(62.4383719093066,876.669038396195,144.436466383471));
#67582=CARTESIAN_POINT('',(62.4383719093132,877.365021216135,142.467263807625));
#67583=CARTESIAN_POINT('',(62.4383719093132,880.527395013838,133.519694342084));
#67584=CARTESIAN_POINT('Ctrl Pts',(62.6055413147402,877.350313629417,142.464300919196));
#67585=CARTESIAN_POINT('Ctrl Pts',(62.72208714417,877.330630015983,142.457344064197));
#67586=CARTESIAN_POINT('Ctrl Pts',(62.8336136664621,877.291603505312,142.440202997864));
#67587=CARTESIAN_POINT('Ctrl Pts',(63.0407880301549,877.175860699171,142.386017629309));
#67588=CARTESIAN_POINT('Ctrl Pts',(63.1330634621422,877.098360066963,142.348480920908));
#67589=CARTESIAN_POINT('Ctrl Pts',(63.2778622256759,876.917873540154,142.259485060922));
#67590=CARTESIAN_POINT('Ctrl Pts',(63.329685673737,876.817039438026,142.20911733911));
#67591=CARTESIAN_POINT('Ctrl Pts',(63.3885551714499,876.602062841949,142.100903255542));
#67592=CARTESIAN_POINT('Ctrl Pts',(63.394333180847,876.489695387477,142.043943701155));
#67593=CARTESIAN_POINT('Ctrl Pts',(63.3573483177835,876.268237368776,141.931080673741));
#67594=CARTESIAN_POINT('Ctrl Pts',(63.3143282299786,876.16125271223,141.87624409014));
#67595=CARTESIAN_POINT('Ctrl Pts',(63.1840901124571,875.968419109575,141.776634971362));
#67596=CARTESIAN_POINT('Ctrl Pts',(63.0980208488533,875.884479178917,141.732841327789));
#67597=CARTESIAN_POINT('Ctrl Pts',(62.8981887649957,875.754748175952,141.663837095797));
#67598=CARTESIAN_POINT('Ctrl Pts',(62.7875969738874,875.708707086128,141.638555941914));
#67599=CARTESIAN_POINT('Ctrl Pts',(62.5564568518299,875.657696550503,141.608060864491));
#67600=CARTESIAN_POINT('Ctrl Pts',(62.4384316484998,875.651880564185,141.602481448338));
#67601=CARTESIAN_POINT('Ctrl Pts',(62.2049338906412,875.679611942394,141.610677223185));
#67602=CARTESIAN_POINT('Ctrl Pts',(62.0916232868256,875.713123975188,141.62448421237));
#67603=CARTESIAN_POINT('Ctrl Pts',(61.881419793599,875.817175719986,141.670711078998));
#67604=CARTESIAN_POINT('Ctrl Pts',(61.7870587196657,875.887667691374,141.703171646909));
#67605=CARTESIAN_POINT('Ctrl Pts',(61.6284825114992,876.060759925578,141.784914577179));
#67606=CARTESIAN_POINT('Ctrl Pts',(61.5677521159699,876.163056594358,141.834151467837));
#67607=CARTESIAN_POINT('Ctrl Pts',(61.4951065763654,876.379815933426,141.940424659816));
#67608=CARTESIAN_POINT('Ctrl Pts',(61.4828038449027,876.49190353717,141.996261449943));
#67609=CARTESIAN_POINT('Ctrl Pts',(61.5066784858156,876.714774750312,142.10915198306));
#67610=CARTESIAN_POINT('Ctrl Pts',(61.5433074498874,876.823447452225,142.165163658863));
#67611=CARTESIAN_POINT('Ctrl Pts',(61.6621002604964,877.022057875704,142.26943973004));
#67612=CARTESIAN_POINT('Ctrl Pts',(61.7435525525451,877.109942462106,142.316640182244));
#67613=CARTESIAN_POINT('Ctrl Pts',(61.930444731815,877.244110818974,142.390682623665));
#67614=CARTESIAN_POINT('Ctrl Pts',(62.0310240273176,877.292704466039,142.418537038328));
#67615=CARTESIAN_POINT('Ctrl Pts',(62.2527021724929,877.356991314408,142.457911555512));
#67616=CARTESIAN_POINT('Ctrl Pts',(62.3725054475672,877.370304133369,142.468165169746));
#67617=CARTESIAN_POINT('Ctrl Pts',(62.5302315213295,877.36094521898,142.467713164468));
#67618=CARTESIAN_POINT('Ctrl Pts',(62.5680701109172,877.356642201572,142.466537650728));
#67619=CARTESIAN_POINT('Ctrl Pts',(62.6055413147402,877.350313629417,142.464300919196));
#67620=CARTESIAN_POINT('Ctrl Pts',(62.4383719093066,876.669038396195,144.436466383471));
#67621=CARTESIAN_POINT('Ctrl Pts',(62.555733234486,876.667692457565,144.440274560546));
#67622=CARTESIAN_POINT('Ctrl Pts',(62.6720670749973,876.647214147807,144.432827703646));
#67623=CARTESIAN_POINT('Ctrl Pts',(62.897044452594,876.567899624079,144.395156694303));
#67624=CARTESIAN_POINT('Ctrl Pts',(63.0024075453455,876.507839463088,144.364089835034));
#67625=CARTESIAN_POINT('Ctrl Pts',(63.1830615484687,876.354660027784,144.281800950729));
#67626=CARTESIAN_POINT('Ctrl Pts',(63.2558086950144,876.262483498011,144.231047193493));
#67627=CARTESIAN_POINT('Ctrl Pts',(63.3580066428205,876.056646754608,144.116235483613));
#67628=CARTESIAN_POINT('Ctrl Pts',(63.3852094653763,875.944453294448,144.052971918191));
#67629=CARTESIAN_POINT('Ctrl Pts',(63.3876075529805,875.719039320324,143.925081024894));
#67630=CARTESIAN_POINT('Ctrl Pts',(63.3632946319265,875.607847438087,143.861618541101));
#67631=CARTESIAN_POINT('Ctrl Pts',(63.2670637567054,875.402165648925,143.74348597352));
#67632=CARTESIAN_POINT('Ctrl Pts',(63.196723652669,875.309310840088,143.689762326666));
#67633=CARTESIAN_POINT('Ctrl Pts',(63.0193151739335,875.15402775659,143.598605428878));
#67634=CARTESIAN_POINT('Ctrl Pts',(62.9143276467654,875.092828857164,143.56189569621));
#67635=CARTESIAN_POINT('Ctrl Pts',(62.6849156051955,875.011174307758,143.510290460012));
#67636=CARTESIAN_POINT('Ctrl Pts',(62.5632257559092,874.990743073138,143.49547525302));
#67637=CARTESIAN_POINT('Ctrl Pts',(62.4395343550587,874.991687400951,143.492120704992));
#67638=CARTESIAN_POINT('Ctrl Pts',(62.4389531191745,874.991692314545,143.492105198705));
#67639=CARTESIAN_POINT('Ctrl Pts',(62.4383719093132,874.991697703936,143.49208995005));
#67640=CARTESIAN_POINT('Origin',(62.4383719093132,879.633498841219,133.203761188948));
#67641=CARTESIAN_POINT('',(62.4383719093132,877.970082209713,139.410656432436));
#67642=CARTESIAN_POINT('Origin',(62.4383719093132,877.498659979104,139.244039865169));
#67643=CARTESIAN_POINT('',(62.4383719093133,876.275109833979,144.206383959985));
#67644=CARTESIAN_POINT('',(62.4383719093132,880.104921071828,133.370377756215));
#67645=CARTESIAN_POINT('Ctrl Pts',(62.4383863925631,875.390537429112,143.708276808823));
#67646=CARTESIAN_POINT('Ctrl Pts',(62.376105965251,875.391147288516,143.706545868688));
#67647=CARTESIAN_POINT('Ctrl Pts',(62.3143704644587,875.402084130781,143.710517980071));
#67648=CARTESIAN_POINT('Ctrl Pts',(62.1951706705049,875.444615587081,143.729978894648));
#67649=CARTESIAN_POINT('Ctrl Pts',(62.1394034980978,875.476857064485,143.74588134496));
#67650=CARTESIAN_POINT('Ctrl Pts',(62.0441551526551,875.558908643506,143.788024886857));
#67651=CARTESIAN_POINT('Ctrl Pts',(62.005960028511,875.608132015386,143.813990237086));
#67652=CARTESIAN_POINT('Ctrl Pts',(61.9530905226921,875.716751261863,143.87259420486));
#67653=CARTESIAN_POINT('Ctrl Pts',(61.939128524658,875.775158862972,143.90471287974));
#67654=CARTESIAN_POINT('Ctrl Pts',(61.9376685681124,875.893313469618,143.970927050264));
#67655=CARTESIAN_POINT('Ctrl Pts',(61.9504235315678,875.951984282128,144.004431762463));
#67656=CARTESIAN_POINT('Ctrl Pts',(62.0008504069484,876.059930606694,144.067317152996));
#67657=CARTESIAN_POINT('Ctrl Pts',(62.0375913341877,876.108434873176,144.096220422258));
#67658=CARTESIAN_POINT('Ctrl Pts',(62.1298179415902,876.189173520707,144.145634475477));
#67659=CARTESIAN_POINT('Ctrl Pts',(62.1841270777158,876.220958291211,144.165839046227));
#67660=CARTESIAN_POINT('Ctrl Pts',(62.3033189923729,876.263969889562,144.194929658026));
#67661=CARTESIAN_POINT('Ctrl Pts',(62.3668774652493,876.275054758898,144.203681029958));
#67662=CARTESIAN_POINT('Ctrl Pts',(62.4958103337154,876.275232094091,144.208600339714));
#67663=CARTESIAN_POINT('Ctrl Pts',(62.5598205189458,876.264336616015,144.20472294943));
#67664=CARTESIAN_POINT('Ctrl Pts',(62.6807329013917,876.221492558253,144.184589799477));
#67665=CARTESIAN_POINT('Ctrl Pts',(62.7362168062647,876.189729164313,144.168388876152));
#67666=CARTESIAN_POINT('Ctrl Pts',(62.8312677686969,876.108822135668,144.125506319516));
#67667=CARTESIAN_POINT('Ctrl Pts',(62.8695264542933,876.06020301376,144.099081885462));
#67668=CARTESIAN_POINT('Ctrl Pts',(62.9232247192187,875.951866843773,144.039272469364));
#67669=CARTESIAN_POINT('Ctrl Pts',(62.9375602010487,875.892960850148,144.006318307079));
#67670=CARTESIAN_POINT('Ctrl Pts',(62.9391134300678,875.77432230511,143.939277709704));
#67671=CARTESIAN_POINT('Ctrl Pts',(62.9264289215955,875.715659761762,143.905800236594));
#67672=CARTESIAN_POINT('Ctrl Pts',(62.8758201252976,875.60689000501,143.843067465165));
#67673=CARTESIAN_POINT('Ctrl Pts',(62.8385821864005,875.557693083714,143.814342200385));
#67674=CARTESIAN_POINT('Ctrl Pts',(62.7444583446654,875.475483173381,143.76543488942));
#67675=CARTESIAN_POINT('Ctrl Pts',(62.6886427479659,875.443145833385,143.745659542972));
#67676=CARTESIAN_POINT('Ctrl Pts',(62.5672261067943,875.400453806565,143.718012081886));
#67677=CARTESIAN_POINT('Ctrl Pts',(62.5031730782759,875.389903028046,143.710077404602));
#67678=CARTESIAN_POINT('Ctrl Pts',(62.4383863925631,875.390537429112,143.708276808823));
#67679=CARTESIAN_POINT('Origin',(76.6453214979932,870.871268259904,130.106892424027));
#67680=CARTESIAN_POINT('',(76.6453214979932,866.303275397976,139.966351605635));
#67681=CARTESIAN_POINT('',(76.6453214979921,868.184856019917,140.772930142153));
#67682=CARTESIAN_POINT('Ctrl Pts',(76.6453214979932,866.303275397976,139.966351605635));
#67683=CARTESIAN_POINT('Ctrl Pts',(76.5119628738476,866.304347994492,139.963316818336));
#67684=CARTESIAN_POINT('Ctrl Pts',(76.379846768452,866.329598642102,139.970253809113));
#67685=CARTESIAN_POINT('Ctrl Pts',(76.1313319090301,866.426503413702,140.003110518868));
#67686=CARTESIAN_POINT('Ctrl Pts',(76.0176747985336,866.49784419209,140.028965220415));
#67687=CARTESIAN_POINT('Ctrl Pts',(75.8269771134016,866.676845950906,140.096285369625));
#67688=CARTESIAN_POINT('Ctrl Pts',(75.7516651901821,866.782573853334,140.137028281501));
#67689=CARTESIAN_POINT('Ctrl Pts',(75.6494772737211,867.01407916826,140.22863620336));
#67690=CARTESIAN_POINT('Ctrl Pts',(75.6234755046857,867.13750965737,140.278587256159));
#67691=CARTESIAN_POINT('Ctrl Pts',(75.6243652570395,867.386516400265,140.382275419247));
#67692=CARTESIAN_POINT('Ctrl Pts',(75.6516267692455,867.509619917659,140.435019246053));
#67693=CARTESIAN_POINT('Ctrl Pts',(75.756035101699,867.736839407519,140.535790665106));
#67694=CARTESIAN_POINT('Ctrl Pts',(75.8317723194575,867.838925833057,140.582888526695));
#67695=CARTESIAN_POINT('Ctrl Pts',(76.0218340465849,868.009264327836,140.665286730341));
#67696=CARTESIAN_POINT('Ctrl Pts',(76.1342919852252,868.075999606575,140.699831282128));
#67697=CARTESIAN_POINT('Ctrl Pts',(76.3807839141933,868.165078796819,140.750995183942));
#67698=CARTESIAN_POINT('Ctrl Pts',(76.5123700762829,868.186869794232,140.767232401553));
#67699=CARTESIAN_POINT('Ctrl Pts',(76.6453214979909,868.184856019917,140.772930142153));
#67700=CARTESIAN_POINT('',(76.6453214965781,868.830144724269,138.947160680077));
#67701=CARTESIAN_POINT('',(76.6453214979932,871.834297400147,130.447259507094));
#67702=CARTESIAN_POINT('Ctrl Pts',(77.1300827245181,868.711403932131,138.915922936985));
#67703=CARTESIAN_POINT('Ctrl Pts',(77.2473082361111,868.651809077314,138.89486009885));
#67704=CARTESIAN_POINT('Ctrl Pts',(77.351015383111,868.571914549659,138.864305759322));
#67705=CARTESIAN_POINT('Ctrl Pts',(77.5197567487852,868.38052807592,138.787811678289));
#67706=CARTESIAN_POINT('Ctrl Pts',(77.5831435862104,868.270900403944,138.742622970067));
#67707=CARTESIAN_POINT('Ctrl Pts',(77.6611216157373,868.035554291658,138.6435912125));
#67708=CARTESIAN_POINT('Ctrl Pts',(77.6747487028992,867.912024628227,138.590669816739));
#67709=CARTESIAN_POINT('Ctrl Pts',(77.6496314710478,867.667130458199,138.484351212652));
#67710=CARTESIAN_POINT('Ctrl Pts',(77.6108976366063,867.548107342416,138.431971487266));
#67711=CARTESIAN_POINT('Ctrl Pts',(77.4855020824012,867.330870219108,138.33509671284));
#67712=CARTESIAN_POINT('Ctrl Pts',(77.3999881714758,867.234755878982,138.291537482276));
#67713=CARTESIAN_POINT('Ctrl Pts',(77.1940931635023,867.079500510575,138.219455644948));
#67714=CARTESIAN_POINT('Ctrl Pts',(77.0760092323133,867.021499353061,138.191475827106));
#67715=CARTESIAN_POINT('Ctrl Pts',(76.8202033122931,866.950315878335,138.153912776674));
#67716=CARTESIAN_POINT('Ctrl Pts',(76.6847800464705,866.93842210285,138.144931373501));
#67717=CARTESIAN_POINT('Ctrl Pts',(76.415948278698,866.964101484819,138.147516439664));
#67718=CARTESIAN_POINT('Ctrl Pts',(76.2852244248027,867.001500174738,138.159082927942));
#67719=CARTESIAN_POINT('Ctrl Pts',(76.0477539225662,867.120547623079,138.201062152901));
#67720=CARTESIAN_POINT('Ctrl Pts',(75.9431056439005,867.200589350415,138.230876351615));
#67721=CARTESIAN_POINT('Ctrl Pts',(75.7727644221043,867.393034589059,138.305074044112));
#67722=CARTESIAN_POINT('Ctrl Pts',(75.7087044733088,867.503532369404,138.348728597479));
#67723=CARTESIAN_POINT('Ctrl Pts',(75.6300648050044,867.740033555641,138.444392178609));
#67724=CARTESIAN_POINT('Ctrl Pts',(75.6160771903657,867.863697967913,138.495457998115));
#67725=CARTESIAN_POINT('Ctrl Pts',(75.6401821455974,868.109223061586,138.599237967042));
#67726=CARTESIAN_POINT('Ctrl Pts',(75.6784796659013,868.228677949967,138.650962292424));
#67727=CARTESIAN_POINT('Ctrl Pts',(75.8037267792447,868.447553819744,138.748452083201));
#67728=CARTESIAN_POINT('Ctrl Pts',(75.8900231716582,868.544580426584,138.793186121453));
#67729=CARTESIAN_POINT('Ctrl Pts',(76.0979913546796,868.700369533179,138.86825890857));
#67730=CARTESIAN_POINT('Ctrl Pts',(76.2172844819361,868.758053321954,138.898026656606));
#67731=CARTESIAN_POINT('Ctrl Pts',(76.4738587020055,868.827221602551,138.938617438612));
#67732=CARTESIAN_POINT('Ctrl Pts',(76.6086352443932,868.838096652377,138.949063105502));
#67733=CARTESIAN_POINT('Ctrl Pts',(76.8096199490018,868.817870132611,138.948779462126));
#67734=CARTESIAN_POINT('Ctrl Pts',(76.8761693785757,868.804967104891,138.945985567369));
#67735=CARTESIAN_POINT('Ctrl Pts',(77.0064626338259,868.767069453388,138.934987178594));
#67736=CARTESIAN_POINT('Ctrl Pts',(77.0698272854177,868.742036463364,138.92674951));
#67737=CARTESIAN_POINT('Ctrl Pts',(77.130082724518,868.711403932131,138.915922936985));
#67738=CARTESIAN_POINT('Ctrl Pts',(76.6453214979909,868.184856019917,140.772930142153));
#67739=CARTESIAN_POINT('Ctrl Pts',(76.6455365781618,868.184852762164,140.772939359587));
#67740=CARTESIAN_POINT('Ctrl Pts',(76.6457516619049,868.184849442101,140.772948549453));
#67741=CARTESIAN_POINT('Ctrl Pts',(76.645966749189,868.184846059724,140.772957711745));
#67742=CARTESIAN_POINT('Ctrl Pts',(76.7758691670263,868.182803265772,140.778491297362));
#67743=CARTESIAN_POINT('Ctrl Pts',(76.9046277809621,868.158075778458,140.773848044284));
#67744=CARTESIAN_POINT('Ctrl Pts',(77.1491128882823,868.064720459959,140.743926410569));
#67745=CARTESIAN_POINT('Ctrl Pts',(77.2619724901293,867.995916165013,140.718416342906));
#67746=CARTESIAN_POINT('Ctrl Pts',(77.4536935388035,867.822471804786,140.649470931866));
#67747=CARTESIAN_POINT('Ctrl Pts',(77.5304169855189,867.719354765232,140.606626501274));
#67748=CARTESIAN_POINT('Ctrl Pts',(77.6366450292619,867.49203730869,140.50967863608));
#67749=CARTESIAN_POINT('Ctrl Pts',(77.6649018006034,867.369962760814,140.456488116416));
#67750=CARTESIAN_POINT('Ctrl Pts',(77.6683867627123,867.123261849436,140.34769961892));
#67751=CARTESIAN_POINT('Ctrl Pts',(77.6435639259179,867.000976223799,140.293149379933));
#67752=CARTESIAN_POINT('Ctrl Pts',(77.5430919170751,866.771200044504,140.189901410266));
#67753=CARTESIAN_POINT('Ctrl Pts',(77.4678598771213,866.666132679206,140.14229096986));
#67754=CARTESIAN_POINT('Ctrl Pts',(77.2778518533872,866.490435172365,140.061702718765));
#67755=CARTESIAN_POINT('Ctrl Pts',(77.1654208526084,866.421119586801,140.029332807694));
#67756=CARTESIAN_POINT('Ctrl Pts',(76.9175992267621,866.326859789564,139.983167794367));
#67757=CARTESIAN_POINT('Ctrl Pts',(76.7846945371961,866.30277197589,139.96977777939));
#67758=CARTESIAN_POINT('Ctrl Pts',(76.6486396341716,866.303252452217,139.966428656905));
#67759=CARTESIAN_POINT('Ctrl Pts',(76.6469804699811,866.30326205495,139.966389358177));
#67760=CARTESIAN_POINT('Ctrl Pts',(76.6453214979932,866.303275397976,139.966351605635));
#67761=CARTESIAN_POINT('Origin',(76.6453214979932,870.871268259904,130.106892424027));
#67762=CARTESIAN_POINT('',(76.6453214979932,869.207851628398,136.313787667516));
#67763=CARTESIAN_POINT('Origin',(76.6453214979932,868.736429397789,136.147171100248));
#67764=CARTESIAN_POINT('',(76.6453214979932,867.707356875089,140.55926334394));
#67765=CARTESIAN_POINT('',(76.6453214979932,871.342690490513,130.273508991294));
#67766=CARTESIAN_POINT('Ctrl Pts',(76.6455915157221,866.78629497717,140.164399194601));
#67767=CARTESIAN_POINT('Ctrl Pts',(76.5847002532572,866.786869833523,140.162674025301));
#67768=CARTESIAN_POINT('Ctrl Pts',(76.5242990128218,866.797712291959,140.165279069441));
#67769=CARTESIAN_POINT('Ctrl Pts',(76.4050919191034,866.840852512441,140.179454220941));
#67770=CARTESIAN_POINT('Ctrl Pts',(76.3481799042497,866.874635171996,140.191698659241));
#67771=CARTESIAN_POINT('Ctrl Pts',(76.2519029134282,866.960596605688,140.224409507011));
#67772=CARTESIAN_POINT('Ctrl Pts',(76.2134725269528,867.011866078816,140.24452996038));
#67773=CARTESIAN_POINT('Ctrl Pts',(76.1604395759368,867.124882016385,140.290073822061));
#67774=CARTESIAN_POINT('Ctrl Pts',(76.1463241275259,867.185474924495,140.315035239601));
#67775=CARTESIAN_POINT('Ctrl Pts',(76.1444190637503,867.307974733356,140.366715590104));
#67776=CARTESIAN_POINT('Ctrl Pts',(76.1567255732018,867.368664155497,140.392928419684));
#67777=CARTESIAN_POINT('Ctrl Pts',(76.2060536755482,867.480923818108,140.442751171601));
#67778=CARTESIAN_POINT('Ctrl Pts',(76.2423002723906,867.531524197334,140.465913652237));
#67779=CARTESIAN_POINT('Ctrl Pts',(76.3340138935697,867.616504965522,140.50632597579));
#67780=CARTESIAN_POINT('Ctrl Pts',(76.3885740530013,867.650117807156,140.523204417909));
#67781=CARTESIAN_POINT('Ctrl Pts',(76.5087908048966,867.695776913516,140.548223781975));
#67782=CARTESIAN_POINT('Ctrl Pts',(76.5732623406447,867.707472088686,140.556156355653));
#67783=CARTESIAN_POINT('Ctrl Pts',(76.7037400351171,867.707339181011,140.56181524903));
#67784=CARTESIAN_POINT('Ctrl Pts',(76.7684757215617,867.69556681531,140.55950677998));
#67785=CARTESIAN_POINT('Ctrl Pts',(76.8898618034568,867.649889340746,140.544752935997));
#67786=CARTESIAN_POINT('Ctrl Pts',(76.9452985494962,867.616407930743,140.532439542117));
#67787=CARTESIAN_POINT('Ctrl Pts',(77.0395056810008,867.53181158141,140.499307691243));
#67788=CARTESIAN_POINT('Ctrl Pts',(77.0772729664222,867.481467380607,140.478786840159));
#67789=CARTESIAN_POINT('Ctrl Pts',(77.1298095814109,867.370372348707,140.432305116792));
#67790=CARTESIAN_POINT('Ctrl Pts',(77.143979729308,867.31066847716,140.406782369924));
#67791=CARTESIAN_POINT('Ctrl Pts',(77.1464962024423,867.189247101387,140.354056506975));
#67792=CARTESIAN_POINT('Ctrl Pts',(77.1345177345304,867.128699899428,140.327356253872));
#67793=CARTESIAN_POINT('Ctrl Pts',(77.0854061738484,867.015453169631,140.276717501026));
#67794=CARTESIAN_POINT('Ctrl Pts',(77.0486577023117,866.963894880086,140.253287852374));
#67795=CARTESIAN_POINT('Ctrl Pts',(76.955439847223,866.877484477876,140.213166841424));
#67796=CARTESIAN_POINT('Ctrl Pts',(76.9000010858462,866.843386980729,140.196829321882));
#67797=CARTESIAN_POINT('Ctrl Pts',(76.7776540030803,866.797253892379,140.173272830889));
#67798=CARTESIAN_POINT('Ctrl Pts',(76.7119713163255,866.785668305157,140.166279864988));
#67799=CARTESIAN_POINT('Ctrl Pts',(76.6455915157221,866.78629497717,140.164399194601));
#67800=CARTESIAN_POINT('Origin',(73.3263803266512,876.659647506777,132.15270150458));
#67801=CARTESIAN_POINT('',(73.3263803266511,872.015461567959,142.447777784718));
#67802=CARTESIAN_POINT('',(73.3263803266511,873.699407765406,143.373464708198));
#67803=CARTESIAN_POINT('Ctrl Pts',(73.3263803266511,872.015461567959,142.447777784718));
#67804=CARTESIAN_POINT('Ctrl Pts',(73.3252176298833,872.015484770283,142.447712136436));
#67805=CARTESIAN_POINT('Ctrl Pts',(73.3240548025254,872.015509884549,142.447647496968));
#67806=CARTESIAN_POINT('Ctrl Pts',(73.2002688528243,872.018386715616,142.440874668704));
#67807=CARTESIAN_POINT('Ctrl Pts',(73.0787775891136,872.042455866726,142.445514355066));
#67808=CARTESIAN_POINT('Ctrl Pts',(72.8502948484491,872.13114453728,142.477079736634));
#67809=CARTESIAN_POINT('Ctrl Pts',(72.7459078121859,872.195304136686,142.503935208013));
#67810=CARTESIAN_POINT('Ctrl Pts',(72.5690591256913,872.355961412184,142.577013059498));
#67811=CARTESIAN_POINT('Ctrl Pts',(72.4988010419257,872.451067030189,142.622660201959));
#67812=CARTESIAN_POINT('Ctrl Pts',(72.4027730473336,872.659160424314,142.727125868623));
#67813=CARTESIAN_POINT('Ctrl Pts',(72.378220020111,872.770126231009,142.784966873483));
#67814=CARTESIAN_POINT('Ctrl Pts',(72.378373092551,872.993744226334,142.906062269608));
#67815=CARTESIAN_POINT('Ctrl Pts',(72.403730713248,873.104265330165,142.968231049123));
#67816=CARTESIAN_POINT('Ctrl Pts',(72.5013305992743,873.307813715298,143.087590079837));
#67817=CARTESIAN_POINT('Ctrl Pts',(72.5724781186642,873.399143569926,143.143755868877));
#67818=CARTESIAN_POINT('Ctrl Pts',(72.7501981240276,873.549623088657,143.241796329609));
#67819=CARTESIAN_POINT('Ctrl Pts',(72.8546655168054,873.607963600326,143.283029544791));
#67820=CARTESIAN_POINT('Ctrl Pts',(73.0826710213486,873.68433173699,143.344733798657));
#67821=CARTESIAN_POINT('Ctrl Pts',(73.2037128729335,873.70238934793,143.36499869336));
#67822=CARTESIAN_POINT('Ctrl Pts',(73.3263031053865,873.699409645139,143.37345938027));
#67823=CARTESIAN_POINT('Ctrl Pts',(73.3263288458507,873.699409019486,143.373461156774));
#67824=CARTESIAN_POINT('Ctrl Pts',(73.3263545862722,873.699408392909,143.373462932751));
#67825=CARTESIAN_POINT('Ctrl Pts',(73.3263803266511,873.699407765406,143.373464708199));
#67826=CARTESIAN_POINT('',(73.3263803266279,874.393769757164,141.408848077495));
#67827=CARTESIAN_POINT('',(73.3263803266512,877.553543679395,132.468634657717));
#67828=CARTESIAN_POINT('Ctrl Pts',(73.6839261380829,874.324464619427,141.394863496905));
#67829=CARTESIAN_POINT('Ctrl Pts',(73.7935846223079,874.282364849322,141.379984013668));
#67830=CARTESIAN_POINT('Ctrl Pts',(73.8938361330003,874.222351782337,141.355425588237));
#67831=CARTESIAN_POINT('Ctrl Pts',(74.0700402359082,874.068617340966,141.287812690312));
#67832=CARTESIAN_POINT('Ctrl Pts',(74.1425062462717,873.974791334929,141.244506042417));
#67833=CARTESIAN_POINT('Ctrl Pts',(74.242594420944,873.770037260412,141.146933209958));
#67834=CARTESIAN_POINT('Ctrl Pts',(74.2700294259057,873.66134888764,141.093789523144));
#67835=CARTESIAN_POINT('Ctrl Pts',(74.2779735653447,873.439751264166,140.983235344466));
#67836=CARTESIAN_POINT('Ctrl Pts',(74.2576517681451,873.328825054649,140.926785174812));
#67837=CARTESIAN_POINT('Ctrl Pts',(74.1702435586778,873.119694009547,140.818278916962));
#67838=CARTESIAN_POINT('Ctrl Pts',(74.1033922868915,873.023597269198,140.767290491347));
#67839=CARTESIAN_POINT('Ctrl Pts',(73.9312980998025,872.860723874628,140.678270323834));
#67840=CARTESIAN_POINT('Ctrl Pts',(73.8276208891447,872.795587240097,140.641122401338));
#67841=CARTESIAN_POINT('Ctrl Pts',(73.6019438319792,872.708022893533,140.587021292463));
#67842=CARTESIAN_POINT('Ctrl Pts',(73.4829918204992,872.684728893535,140.569779729792));
#67843=CARTESIAN_POINT('Ctrl Pts',(73.2447903592873,872.680228675476,140.555722972313));
#67844=CARTESIAN_POINT('Ctrl Pts',(73.1278176323637,872.69770026638,140.558374173904));
#67845=CARTESIAN_POINT('Ctrl Pts',(72.9054263264503,872.770608858555,140.582537104776));
#67846=CARTESIAN_POINT('Ctrl Pts',(72.802117731416,872.825587192415,140.603931011088));
#67847=CARTESIAN_POINT('Ctrl Pts',(72.6201075234333,872.968506117211,140.663894854231));
#67848=CARTESIAN_POINT('Ctrl Pts',(72.5438758603661,873.055903307858,140.702330298631));
#67849=CARTESIAN_POINT('Ctrl Pts',(72.4283593148395,873.256157296893,140.7936731121));
#67850=CARTESIAN_POINT('Ctrl Pts',(72.3924203577145,873.368033603299,140.84629577083));
#67851=CARTESIAN_POINT('Ctrl Pts',(72.371216213266,873.594093159447,140.955855974205));
#67852=CARTESIAN_POINT('Ctrl Pts',(72.3850232219967,873.706031693908,141.011640078203));
#67853=CARTESIAN_POINT('Ctrl Pts',(72.459886631027,873.91911826784,141.121072388753));
#67854=CARTESIAN_POINT('Ctrl Pts',(72.5208987592655,874.018115035693,141.173664262065));
#67855=CARTESIAN_POINT('Ctrl Pts',(72.6832535084843,874.188864594597,141.268093361005));
#67856=CARTESIAN_POINT('Ctrl Pts',(72.7834239381339,874.258750923942,141.308932620179));
#67857=CARTESIAN_POINT('Ctrl Pts',(72.9976627685876,874.353168422772,141.368925763367));
#67858=CARTESIAN_POINT('Ctrl Pts',(73.1074997385821,874.380910460523,141.389410513765));
#67859=CARTESIAN_POINT('Ctrl Pts',(73.3396637187662,874.400222940271,141.412889567333));
#67860=CARTESIAN_POINT('Ctrl Pts',(73.4601690970707,874.389721905566,141.41472655992));
#67861=CARTESIAN_POINT('Ctrl Pts',(73.6125825484943,874.349629111377,141.403412161613));
#67862=CARTESIAN_POINT('Ctrl Pts',(73.6486693173653,874.338000316709,141.399647470316));
#67863=CARTESIAN_POINT('Ctrl Pts',(73.6839261380829,874.324464619427,141.394863496905));
#67864=CARTESIAN_POINT('Ctrl Pts',(73.326380326651,873.699407765406,143.373464708198));
#67865=CARTESIAN_POINT('Ctrl Pts',(73.4455541865396,873.696502524816,143.381684749111));
#67866=CARTESIAN_POINT('Ctrl Pts',(73.5638127610191,873.673771001158,143.378576620235));
#67867=CARTESIAN_POINT('Ctrl Pts',(73.7891815913094,873.589628174773,143.349292845481));
#67868=CARTESIAN_POINT('Ctrl Pts',(73.8934150634961,873.528063536163,143.322787590984));
#67869=CARTESIAN_POINT('Ctrl Pts',(74.0722365373893,873.372608427554,143.24898823875));
#67870=CARTESIAN_POINT('Ctrl Pts',(74.1442639408735,873.279787856864,143.202101863764));
#67871=CARTESIAN_POINT('Ctrl Pts',(74.245332686204,873.074195514028,143.094021647677));
#67872=CARTESIAN_POINT('Ctrl Pts',(74.2724322038226,872.963098967145,143.03364064157));
#67873=CARTESIAN_POINT('Ctrl Pts',(74.2763024569755,872.738025842134,142.908222642779));
#67874=CARTESIAN_POINT('Ctrl Pts',(74.252376118135,872.626100339391,142.844299439973));
#67875=CARTESIAN_POINT('Ctrl Pts',(74.1564803184499,872.419702481987,142.723584293178));
#67876=CARTESIAN_POINT('Ctrl Pts',(74.0860193003306,872.326841366078,142.667777609939));
#67877=CARTESIAN_POINT('Ctrl Pts',(73.9084179013268,872.172564679373,142.571533546893));
#67878=CARTESIAN_POINT('Ctrl Pts',(73.8034116904804,872.112201763111,142.53179768104));
#67879=CARTESIAN_POINT('Ctrl Pts',(73.5731622181586,872.032298544407,142.473285703891));
#67880=CARTESIAN_POINT('Ctrl Pts',(73.450515317133,872.012984378416,142.454786704893));
#67881=CARTESIAN_POINT('Ctrl Pts',(73.3263803266512,872.015461567959,142.447777784718));
#67882=CARTESIAN_POINT('Origin',(73.3263803266512,876.659647506777,132.15270150458));
#67883=CARTESIAN_POINT('',(73.3263803266512,874.99623087527,138.359596748068));
#67884=CARTESIAN_POINT('Origin',(73.3263803266512,874.524808644662,138.192980180801));
#67885=CARTESIAN_POINT('',(73.3263803266513,873.3036828697,143.148464801744));
#67886=CARTESIAN_POINT('',(73.3263803266512,877.131069737385,132.319318071847));
#67887=CARTESIAN_POINT('Ctrl Pts',(73.3261543474481,872.415623888765,142.660222665343));
#67888=CARTESIAN_POINT('Ctrl Pts',(73.2635808346016,872.416966167653,142.656509710482));
#67889=CARTESIAN_POINT('Ctrl Pts',(73.2015028924454,872.428759538996,142.658477288826));
#67890=CARTESIAN_POINT('Ctrl Pts',(73.0828623177025,872.472884406954,142.6738385555));
#67891=CARTESIAN_POINT('Ctrl Pts',(73.0278008495359,872.505435760309,142.687455702834));
#67892=CARTESIAN_POINT('Ctrl Pts',(72.9328968960245,872.588203705615,142.725314756461));
#67893=CARTESIAN_POINT('Ctrl Pts',(72.8945586595841,872.637998254988,142.749439623196));
#67894=CARTESIAN_POINT('Ctrl Pts',(72.8414607066704,872.747505676854,142.804898884148));
#67895=CARTESIAN_POINT('Ctrl Pts',(72.8273702317476,872.806150475822,142.835708181034));
#67896=CARTESIAN_POINT('Ctrl Pts',(72.8254827966869,872.924488598716,142.900090056835));
#67897=CARTESIAN_POINT('Ctrl Pts',(72.8379339450748,872.983065601358,142.933077147691));
#67898=CARTESIAN_POINT('Ctrl Pts',(72.888135507535,873.09202877754,142.996761315637));
#67899=CARTESIAN_POINT('Ctrl Pts',(72.9256152790222,873.141367953334,143.026864461796));
#67900=CARTESIAN_POINT('Ctrl Pts',(73.0193759650266,873.222214252308,143.078896493632));
#67901=CARTESIAN_POINT('Ctrl Pts',(73.0742508764508,873.253498032805,143.100582891959));
#67902=CARTESIAN_POINT('Ctrl Pts',(73.1943348031452,873.294843230481,143.133063454025));
#67903=CARTESIAN_POINT('Ctrl Pts',(73.2582250952364,873.304879362383,143.143734410334));
#67904=CARTESIAN_POINT('Ctrl Pts',(73.387242507356,873.302633468585,143.152699660637));
#67905=CARTESIAN_POINT('Ctrl Pts',(73.4510382316342,873.290560858201,143.151003186636));
#67906=CARTESIAN_POINT('Ctrl Pts',(73.571118027379,873.245549422212,143.135288645358));
#67907=CARTESIAN_POINT('Ctrl Pts',(73.6260541677723,873.212962972271,143.121360974132));
#67908=CARTESIAN_POINT('Ctrl Pts',(73.7201443638919,873.130783389706,143.082748850287));
#67909=CARTESIAN_POINT('Ctrl Pts',(73.757999277323,873.081785889969,143.058298249754));
#67910=CARTESIAN_POINT('Ctrl Pts',(73.8111238250011,872.973256720484,143.001881207675));
#67911=CARTESIAN_POINT('Ctrl Pts',(73.8253525227939,872.914612735053,142.970335404131));
#67912=CARTESIAN_POINT('Ctrl Pts',(73.827311496767,872.795999726558,142.904726626321));
#67913=CARTESIAN_POINT('Ctrl Pts',(73.81473246018,872.737123639636,142.871251525938));
#67914=CARTESIAN_POINT('Ctrl Pts',(73.7642606016394,872.628265145637,142.807605786528));
#67915=CARTESIAN_POINT('Ctrl Pts',(73.7270004349945,872.579191091669,142.777980032369));
#67916=CARTESIAN_POINT('Ctrl Pts',(73.6328721718507,872.497629229533,142.726604661014));
#67917=CARTESIAN_POINT('Ctrl Pts',(73.5770519765085,872.4657615751,142.705265102881));
#67918=CARTESIAN_POINT('Ctrl Pts',(73.4554739759947,872.424152462769,142.674003993632));
#67919=CARTESIAN_POINT('Ctrl Pts',(73.3912060738502,872.414228449145,142.664082671164));
#67920=CARTESIAN_POINT('Ctrl Pts',(73.3261543474481,872.415623888765,142.660222665343));
#67921=CARTESIAN_POINT('Origin',(85.2906675027921,865.303927287174,128.139205748573));
#67922=CARTESIAN_POINT('',(85.2906675027921,860.734189796252,138.003601155341));
#67923=CARTESIAN_POINT('',(85.2906675027932,862.621926189382,138.792762652049));
#67924=CARTESIAN_POINT('Ctrl Pts',(85.2906675027921,860.734189796252,138.003601155341));
#67925=CARTESIAN_POINT('Ctrl Pts',(85.1569502915632,860.735734357018,137.999230999999));
#67926=CARTESIAN_POINT('Ctrl Pts',(85.0244838725072,860.761567555043,138.004939860221));
#67927=CARTESIAN_POINT('Ctrl Pts',(84.7760728436783,860.859607693897,138.035375001082));
#67928=CARTESIAN_POINT('Ctrl Pts',(84.6627547277935,860.931248053407,138.059952772527));
#67929=CARTESIAN_POINT('Ctrl Pts',(84.4722379734115,861.111004191591,138.124631954799));
#67930=CARTESIAN_POINT('Ctrl Pts',(84.3968810421119,861.217299815088,138.1640796615));
#67931=CARTESIAN_POINT('Ctrl Pts',(84.2947142013479,861.449979545937,138.252939966087));
#67932=CARTESIAN_POINT('Ctrl Pts',(84.2687517349878,861.573998336457,138.30145992044));
#67933=CARTESIAN_POINT('Ctrl Pts',(84.2697834501128,861.823678830441,138.402165922697));
#67934=CARTESIAN_POINT('Ctrl Pts',(84.2969413626358,861.946860844076,138.453381612405));
#67935=CARTESIAN_POINT('Ctrl Pts',(84.4009938711906,862.174540017638,138.551836427236));
#67936=CARTESIAN_POINT('Ctrl Pts',(84.476623662278,862.276920998404,138.598148073696));
#67937=CARTESIAN_POINT('Ctrl Pts',(84.6666190362455,862.447710551251,138.680043733148));
#67938=CARTESIAN_POINT('Ctrl Pts',(84.7791777149321,862.51451118956,138.714849843798));
#67939=CARTESIAN_POINT('Ctrl Pts',(85.0258844449915,862.603223168113,138.767654352663));
#67940=CARTESIAN_POINT('Ctrl Pts',(85.1576036840497,862.624581927685,138.78524854889));
#67941=CARTESIAN_POINT('Ctrl Pts',(85.2906675027942,862.621926189382,138.792762652049));
#67942=CARTESIAN_POINT('',(85.2906675011928,863.266061415442,136.970256822865));
#67943=CARTESIAN_POINT('',(85.2906675027921,866.266956427416,128.47957283164));
#67944=CARTESIAN_POINT('Ctrl Pts',(85.9517574437177,863.030512608055,136.908103725293));
#67945=CARTESIAN_POINT('Ctrl Pts',(86.0532797154454,862.94924051595,136.879379418033));
#67946=CARTESIAN_POINT('Ctrl Pts',(86.1369421188726,862.850778238061,136.842262607317));
#67947=CARTESIAN_POINT('Ctrl Pts',(86.2591791549355,862.630556693338,136.755577236539));
#67948=CARTESIAN_POINT('Ctrl Pts',(86.296559890087,862.510943262656,136.706859223314));
#67949=CARTESIAN_POINT('Ctrl Pts',(86.3198381703693,862.265562959298,136.604281043106));
#67950=CARTESIAN_POINT('Ctrl Pts',(86.30528559595,862.142125008828,136.551392061809));
#67951=CARTESIAN_POINT('Ctrl Pts',(86.2253449482614,861.907641753823,136.448753027354));
#67952=CARTESIAN_POINT('Ctrl Pts',(86.1604966038493,861.798883315632,136.400001186342));
#67953=CARTESIAN_POINT('Ctrl Pts',(85.9885448194371,861.611112405503,136.313540768668));
#67954=CARTESIAN_POINT('Ctrl Pts',(85.8830405366813,861.533927385015,136.276671800154));
#67955=CARTESIAN_POINT('Ctrl Pts',(85.6462163187424,861.422544139861,136.220095855634));
#67956=CARTESIAN_POINT('Ctrl Pts',(85.517404403943,861.389009606684,136.200763370681));
#67957=CARTESIAN_POINT('Ctrl Pts',(85.2506319921123,861.369612048728,136.181503215456));
#67958=CARTESIAN_POINT('Ctrl Pts',(85.1152142728158,861.384557787738,136.182007804843));
#67959=CARTESIAN_POINT('Ctrl Pts',(84.8574701132769,861.462419235978,136.20303577885));
#67960=CARTESIAN_POINT('Ctrl Pts',(84.7377354558107,861.524637599491,136.223374379572));
#67961=CARTESIAN_POINT('Ctrl Pts',(84.5316993823201,861.687635195048,136.280887073647));
#67962=CARTESIAN_POINT('Ctrl Pts',(84.4470939893041,861.78643138328,136.317329733415));
#67963=CARTESIAN_POINT('Ctrl Pts',(84.3233405049538,862.008020509159,136.401827861769));
#67964=CARTESIAN_POINT('Ctrl Pts',(84.2853656425202,862.12862962769,136.449056104176));
#67965=CARTESIAN_POINT('Ctrl Pts',(84.2614332515525,862.375295391752,136.548312191037));
#67966=CARTESIAN_POINT('Ctrl Pts',(84.275531031474,862.498948886981,136.59937415209));
#67967=CARTESIAN_POINT('Ctrl Pts',(84.3544293177363,862.734266673987,136.699546513469));
#67968=CARTESIAN_POINT('Ctrl Pts',(84.418890114086,862.843538527003,136.747671809601));
#67969=CARTESIAN_POINT('Ctrl Pts',(84.5910605524689,863.032941225698,136.834744784467));
#67970=CARTESIAN_POINT('Ctrl Pts',(84.6975904420636,863.110859336869,136.872725233798));
#67971=CARTESIAN_POINT('Ctrl Pts',(84.9367543812024,863.222339015667,136.932137569885));
#67972=CARTESIAN_POINT('Ctrl Pts',(85.0668107282356,863.255313033035,136.95317204863));
#67973=CARTESIAN_POINT('Ctrl Pts',(85.3341493861863,863.272563147414,136.975413193998));
#67974=CARTESIAN_POINT('Ctrl Pts',(85.4688362640369,863.256735195217,136.976421116455));
#67975=CARTESIAN_POINT('Ctrl Pts',(85.6614443469277,863.197504832214,136.962352195151));
#67976=CARTESIAN_POINT('Ctrl Pts',(85.723816582504,863.171826061194,136.955042920435));
#67977=CARTESIAN_POINT('Ctrl Pts',(85.8430715999771,863.109198937968,136.93530429961));
#67978=CARTESIAN_POINT('Ctrl Pts',(85.8995736743458,863.072287521466,136.922868393182));
#67979=CARTESIAN_POINT('Ctrl Pts',(85.9517574437177,863.030512608055,136.908103725293));
#67980=CARTESIAN_POINT('Ctrl Pts',(85.2906675027942,862.621926189382,138.792762652049));
#67981=CARTESIAN_POINT('Ctrl Pts',(85.290945444327,862.621920642119,138.792778347385));
#67982=CARTESIAN_POINT('Ctrl Pts',(85.2912233917269,862.621914990079,138.792793998729));
#67983=CARTESIAN_POINT('Ctrl Pts',(85.2915013449265,862.621909233251,138.792809606068));
#67984=CARTESIAN_POINT('Ctrl Pts',(85.4222739334188,862.619200736487,138.800152612201));
#67985=CARTESIAN_POINT('Ctrl Pts',(85.5518994590603,862.593351495863,138.797608133119));
#67986=CARTESIAN_POINT('Ctrl Pts',(85.7966451560299,862.497445813918,138.772211550131));
#67987=CARTESIAN_POINT('Ctrl Pts',(85.9090900912688,862.427638875522,138.749278284685));
#67988=CARTESIAN_POINT('Ctrl Pts',(86.1000182694894,862.252467028972,138.685371076264));
#67989=CARTESIAN_POINT('Ctrl Pts',(86.1763954703557,862.148680883902,138.644948266126));
#67990=CARTESIAN_POINT('Ctrl Pts',(86.2822289290466,861.920215182198,138.552015072588));
#67991=CARTESIAN_POINT('Ctrl Pts',(86.3103476954312,861.797682803914,138.500369231833));
#67992=CARTESIAN_POINT('Ctrl Pts',(86.3136533776107,861.550275897164,138.393491033601));
#67993=CARTESIAN_POINT('Ctrl Pts',(86.2886848594367,861.427774617121,138.339295280087));
#67994=CARTESIAN_POINT('Ctrl Pts',(86.1880560829598,861.198374157071,138.235949113747));
#67995=CARTESIAN_POINT('Ctrl Pts',(86.1129456851299,861.093827162204,138.187855010266));
#67996=CARTESIAN_POINT('Ctrl Pts',(85.922517161301,860.918403685406,138.105222472305));
#67997=CARTESIAN_POINT('Ctrl Pts',(85.8091606440087,860.849161672914,138.071459155492));
#67998=CARTESIAN_POINT('Ctrl Pts',(85.5601911825806,860.756144864372,138.022787569306));
#67999=CARTESIAN_POINT('Ctrl Pts',(85.4272341468802,860.732879332638,138.008174879463));
#68000=CARTESIAN_POINT('Ctrl Pts',(85.2921177777857,860.734173758729,138.003648848846));
#68001=CARTESIAN_POINT('Ctrl Pts',(85.2913926219043,860.734181420438,138.003624853735));
#68002=CARTESIAN_POINT('Ctrl Pts',(85.2906675027921,860.734189796252,138.003601155341));
#68003=CARTESIAN_POINT('Origin',(85.2906675027921,865.303927287174,128.139205748573));
#68004=CARTESIAN_POINT('',(85.2906675027921,863.640510655667,134.346100992061));
#68005=CARTESIAN_POINT('Origin',(85.2906675027921,863.169088425059,134.179484424794));
#68006=CARTESIAN_POINT('',(85.2906675027922,862.1422270283,138.585320544375));
#68007=CARTESIAN_POINT('',(85.2906675027921,865.775349517782,128.30582231584));
#68008=CARTESIAN_POINT('Ctrl Pts',(85.2909807609949,861.218133294598,138.199034698033));
#68009=CARTESIAN_POINT('Ctrl Pts',(85.2303434350245,861.218933212764,138.196657417334));
#68010=CARTESIAN_POINT('Ctrl Pts',(85.1701826148236,861.229928196416,138.198537549954));
#68011=CARTESIAN_POINT('Ctrl Pts',(85.0513057338549,861.27328301916,138.211091519141));
#68012=CARTESIAN_POINT('Ctrl Pts',(84.9944723623471,861.307143102732,138.222456500081));
#68013=CARTESIAN_POINT('Ctrl Pts',(84.8981098725595,861.39330282904,138.253406730414));
#68014=CARTESIAN_POINT('Ctrl Pts',(84.859547589708,861.444727407849,138.272677758026));
#68015=CARTESIAN_POINT('Ctrl Pts',(84.8061722049066,861.558144413647,138.316619598991));
#68016=CARTESIAN_POINT('Ctrl Pts',(84.7918688364119,861.618984002284,138.340846355856));
#68017=CARTESIAN_POINT('Ctrl Pts',(84.7896088285248,861.741938169565,138.391229715717));
#68018=CARTESIAN_POINT('Ctrl Pts',(84.8017276610717,861.802822562984,138.41688990679));
#68019=CARTESIAN_POINT('Ctrl Pts',(84.8511395108544,861.916493943517,138.466414463185));
#68020=CARTESIAN_POINT('Ctrl Pts',(84.8881037391214,861.968088688051,138.489773565644));
#68021=CARTESIAN_POINT('Ctrl Pts',(84.9810975338317,862.05352103395,138.530421121873));
#68022=CARTESIAN_POINT('Ctrl Pts',(85.0358750230947,862.086863109381,138.547428463491));
#68023=CARTESIAN_POINT('Ctrl Pts',(85.156432348358,862.131748439863,138.573113631298));
#68024=CARTESIAN_POINT('Ctrl Pts',(85.2210361814761,862.142942222118,138.581573766579));
#68025=CARTESIAN_POINT('Ctrl Pts',(85.3515751849396,862.141632752248,138.588611080981));
#68026=CARTESIAN_POINT('Ctrl Pts',(85.4162545362392,862.129221489918,138.587149859483));
#68027=CARTESIAN_POINT('Ctrl Pts',(85.5373232492208,862.082269081205,138.574274301085));
#68028=CARTESIAN_POINT('Ctrl Pts',(85.5925269194731,862.048196142289,138.562987216803));
#68029=CARTESIAN_POINT('Ctrl Pts',(85.6861999518173,861.962552220769,138.531886941751));
#68030=CARTESIAN_POINT('Ctrl Pts',(85.7236826757803,861.911777916675,138.512356609832));
#68031=CARTESIAN_POINT('Ctrl Pts',(85.7756902240541,861.799977902879,138.467601511756));
#68032=CARTESIAN_POINT('Ctrl Pts',(85.789600707965,861.740012884334,138.442797730877));
#68033=CARTESIAN_POINT('Ctrl Pts',(85.7916189117067,861.618851684643,138.391378021577));
#68034=CARTESIAN_POINT('Ctrl Pts',(85.7796409391956,861.558824243433,138.365259094939));
#68035=CARTESIAN_POINT('Ctrl Pts',(85.7308878325463,861.446273579123,138.315155727913));
#68036=CARTESIAN_POINT('Ctrl Pts',(85.6943308301417,861.394928575689,138.291686273606));
#68037=CARTESIAN_POINT('Ctrl Pts',(85.601258872647,861.308562553006,138.250914779803));
#68038=CARTESIAN_POINT('Ctrl Pts',(85.545606449769,861.274434173731,138.234029721826));
#68039=CARTESIAN_POINT('Ctrl Pts',(85.4230160348868,861.228610192363,138.209292316302));
#68040=CARTESIAN_POINT('Ctrl Pts',(85.3573492778565,861.217257771454,138.201636669536));
#68041=CARTESIAN_POINT('Ctrl Pts',(85.2909807609949,861.218133294598,138.199034698033));
#68042=CARTESIAN_POINT('Origin',(83.3206797233787,871.616423241051,130.370255407314));
#68043=CARTESIAN_POINT('',(83.3206797233786,866.96815944026,140.67686952441));
#68044=CARTESIAN_POINT('',(83.3206797233787,868.663281554644,141.570935488596));
#68045=CARTESIAN_POINT('Ctrl Pts',(83.3206797233786,866.96815944026,140.67686952441));
#68046=CARTESIAN_POINT('Ctrl Pts',(83.1979733150929,866.971842780361,140.666447941281));
#68047=CARTESIAN_POINT('Ctrl Pts',(83.076211935733,866.996854463994,140.667172424123));
#68048=CARTESIAN_POINT('Ctrl Pts',(82.8486585433656,867.087125090313,140.690637981941));
#68049=CARTESIAN_POINT('Ctrl Pts',(82.7451459390068,867.151320095247,140.713056669224));
#68050=CARTESIAN_POINT('Ctrl Pts',(82.5678423802552,867.312623517907,140.777509980887));
#68051=CARTESIAN_POINT('Ctrl Pts',(82.4966611313868,867.408697682202,140.819281052879));
#68052=CARTESIAN_POINT('Ctrl Pts',(82.3989366110453,867.618659328567,140.916691907774));
#68053=CARTESIAN_POINT('Ctrl Pts',(82.3734964306883,867.730386334333,140.971354297369));
#68054=CARTESIAN_POINT('Ctrl Pts',(82.3717326836918,867.95506733745,141.087157151649));
#68055=CARTESIAN_POINT('Ctrl Pts',(82.3958948815759,868.065798799513,141.147220798035));
#68056=CARTESIAN_POINT('Ctrl Pts',(82.491554647161,868.271676464125,141.265383137167));
#68057=CARTESIAN_POINT('Ctrl Pts',(82.5628631824429,868.364653210316,141.322345659536));
#68058=CARTESIAN_POINT('Ctrl Pts',(82.7414426939018,868.516808745593,141.423460415312));
#68059=CARTESIAN_POINT('Ctrl Pts',(82.8464994784539,868.575268072358,141.466953046361));
#68060=CARTESIAN_POINT('Ctrl Pts',(83.0756963723964,868.650648853518,141.53454681768));
#68061=CARTESIAN_POINT('Ctrl Pts',(83.1974017211958,868.667708457805,141.558410080125));
#68062=CARTESIAN_POINT('Ctrl Pts',(83.3206797233788,868.663281554644,141.570935488596));
#68063=CARTESIAN_POINT('',(83.3206797233787,869.354927286473,139.614004199963));
#68064=CARTESIAN_POINT('',(83.3206797233787,872.51031941367,130.68618856045));
#68065=CARTESIAN_POINT('Ctrl Pts',(83.8529754731604,869.193059772498,139.581251398577));
#68066=CARTESIAN_POINT('Ctrl Pts',(83.9509540102205,869.130383807693,139.55909959192));
#68067=CARTESIAN_POINT('Ctrl Pts',(84.0355490372359,869.052053013329,139.528067061837));
#68068=CARTESIAN_POINT('Ctrl Pts',(84.1730819145392,868.86722819535,139.44946577285));
#68069=CARTESIAN_POINT('Ctrl Pts',(84.2225713908958,868.761316773023,139.401887729917));
#68070=CARTESIAN_POINT('Ctrl Pts',(84.2735746431976,868.541589999515,139.299023039021));
#68071=CARTESIAN_POINT('Ctrl Pts',(84.2754221636958,868.429999817896,139.244853754776));
#68072=CARTESIAN_POINT('Ctrl Pts',(84.2320937478474,868.211908668153,139.135538882559));
#68073=CARTESIAN_POINT('Ctrl Pts',(84.1865603041033,868.107508511897,139.081395240941));
#68074=CARTESIAN_POINT('Ctrl Pts',(84.0525489064174,867.920319473664,138.980644030745));
#68075=CARTESIAN_POINT('Ctrl Pts',(83.9647881720151,867.839544310954,138.935070769086));
#68076=CARTESIAN_POINT('Ctrl Pts',(83.7583592571335,867.714181399806,138.859308075614));
#68077=CARTESIAN_POINT('Ctrl Pts',(83.6416052910264,867.670888821712,138.829880581775));
#68078=CARTESIAN_POINT('Ctrl Pts',(83.3999464308693,867.629636037344,138.79214754597));
#68079=CARTESIAN_POINT('Ctrl Pts',(83.2778329727144,867.630230889189,138.783349111841));
#68080=CARTESIAN_POINT('Ctrl Pts',(83.0429807192215,867.672608849585,138.78586068879));
#68081=CARTESIAN_POINT('Ctrl Pts',(82.9321727381681,867.712652813023,138.79648973059));
#68082=CARTESIAN_POINT('Ctrl Pts',(82.7306074514192,867.827574208798,138.835501407793));
#68083=CARTESIAN_POINT('Ctrl Pts',(82.6418159464984,867.901589075903,138.863623469071));
#68084=CARTESIAN_POINT('Ctrl Pts',(82.4959537432314,868.076999155354,138.935070785635));
#68085=CARTESIAN_POINT('Ctrl Pts',(82.4411831805063,868.177378266506,138.978094479996));
#68086=CARTESIAN_POINT('Ctrl Pts',(82.3737749249685,868.395759544687,139.075844090801));
#68087=CARTESIAN_POINT('Ctrl Pts',(82.3641981111281,868.512146324994,139.130060903623));
#68088=CARTESIAN_POINT('Ctrl Pts',(82.3953620846968,868.737218892493,139.239272271814));
#68089=CARTESIAN_POINT('Ctrl Pts',(82.4346754010858,868.84389336496,139.29319587819));
#68090=CARTESIAN_POINT('Ctrl Pts',(82.557255688024,869.0374138716,139.395712878524));
#68091=CARTESIAN_POINT('Ctrl Pts',(82.639984457656,869.122166355449,139.443270339902));
#68092=CARTESIAN_POINT('Ctrl Pts',(82.8388054638799,869.257124499995,139.525049541975));
#68093=CARTESIAN_POINT('Ctrl Pts',(82.9533161026836,869.305736591076,139.558369765515));
#68094=CARTESIAN_POINT('Ctrl Pts',(83.1855383193989,869.355911163594,139.602725961546));
#68095=CARTESIAN_POINT('Ctrl Pts',(83.2998325612397,869.361442482731,139.615360692469));
#68096=CARTESIAN_POINT('Ctrl Pts',(83.5323356964507,869.334707870404,139.622565145655));
#68097=CARTESIAN_POINT('Ctrl Pts',(83.6482765147052,869.300775739711,139.616120796109));
#68098=CARTESIAN_POINT('Ctrl Pts',(83.788716144608,869.231662099515,139.594549448878));
#68099=CARTESIAN_POINT('Ctrl Pts',(83.8214739277969,869.213211019984,139.588373531273));
#68100=CARTESIAN_POINT('Ctrl Pts',(83.8529754731605,869.193059772498,139.581251398577));
#68101=CARTESIAN_POINT('Ctrl Pts',(83.3206797233788,868.663281554644,141.570935488596));
#68102=CARTESIAN_POINT('Ctrl Pts',(83.3208136591537,868.663276745021,141.570949096866));
#68103=CARTESIAN_POINT('Ctrl Pts',(83.320947596785,868.663271910027,141.570962691749));
#68104=CARTESIAN_POINT('Ctrl Pts',(83.3210815362641,868.66326704966,141.570976273243));
#68105=CARTESIAN_POINT('Ctrl Pts',(83.4409190602393,868.658918411885,141.583127826063));
#68106=CARTESIAN_POINT('Ctrl Pts',(83.5599476170798,868.634346057652,141.584321333876));
#68107=CARTESIAN_POINT('Ctrl Pts',(83.7850979720042,868.546351202737,141.563918959409));
#68108=CARTESIAN_POINT('Ctrl Pts',(83.8886378549942,868.483357003621,141.542234991254));
#68109=CARTESIAN_POINT('Ctrl Pts',(84.0661297463215,868.325657417287,141.477894141923));
#68110=CARTESIAN_POINT('Ctrl Pts',(84.1376668760204,868.232228618615,141.435641327911));
#68111=CARTESIAN_POINT('Ctrl Pts',(84.2385262704065,868.025959966724,141.335701117012));
#68112=CARTESIAN_POINT('Ctrl Pts',(84.2658980052954,867.91492057408,141.278772343917));
#68113=CARTESIAN_POINT('Ctrl Pts',(84.2712520516383,867.689914391234,141.15817441664));
#68114=CARTESIAN_POINT('Ctrl Pts',(84.2482781067566,867.578078907386,141.095565824849));
#68115=CARTESIAN_POINT('Ctrl Pts',(84.1541862593483,867.370714845655,140.974594892567));
#68116=CARTESIAN_POINT('Ctrl Pts',(84.0838525790934,867.277055721332,140.91732411838));
#68117=CARTESIAN_POINT('Ctrl Pts',(83.9062265462893,867.122274782354,140.816925346475));
#68118=CARTESIAN_POINT('Ctrl Pts',(83.8010894313335,867.062087722414,140.774501488061));
#68119=CARTESIAN_POINT('Ctrl Pts',(83.5698228176162,866.982972971342,140.709594402539));
#68120=CARTESIAN_POINT('Ctrl Pts',(83.4461428096556,866.96441517511,140.687536555567));
#68121=CARTESIAN_POINT('Ctrl Pts',(83.3208024761302,866.96815576087,140.6768799527));
#68122=CARTESIAN_POINT('Ctrl Pts',(83.3207410996363,866.968157597897,140.67687473716));
#68123=CARTESIAN_POINT('Ctrl Pts',(83.3206797233786,866.968159440259,140.67686952441));
#68124=CARTESIAN_POINT('Origin',(83.3206797233787,871.616423241051,130.370255407314));
#68125=CARTESIAN_POINT('',(83.3206797233787,869.953006609545,136.577150650802));
#68126=CARTESIAN_POINT('Origin',(83.3206797233787,869.481584378936,136.410534083535));
#68127=CARTESIAN_POINT('',(83.3206797233786,868.264547749415,141.35444894226));
#68128=CARTESIAN_POINT('',(83.3206797233787,872.08784547166,130.536871974581));
#68129=CARTESIAN_POINT('Ctrl Pts',(83.3208923352077,867.370572634924,140.882945801216));
#68130=CARTESIAN_POINT('Ctrl Pts',(83.2585379255171,867.372510723548,140.877382636858));
#68131=CARTESIAN_POINT('Ctrl Pts',(83.1966100897607,867.384878590161,140.877314432226));
#68132=CARTESIAN_POINT('Ctrl Pts',(83.078181283712,867.43016320687,140.888377721573));
#68133=CARTESIAN_POINT('Ctrl Pts',(83.0231454578108,867.463267480699,140.899757361664));
#68134=CARTESIAN_POINT('Ctrl Pts',(82.9286860400494,867.546686619094,140.933039856722));
#68135=CARTESIAN_POINT('Ctrl Pts',(82.890537587744,867.596375775113,140.954753343466));
#68136=CARTESIAN_POINT('Ctrl Pts',(82.8368483641075,867.706138598117,141.006019179575));
#68137=CARTESIAN_POINT('Ctrl Pts',(82.822262021685,867.765208072751,141.035156313976));
#68138=CARTESIAN_POINT('Ctrl Pts',(82.8193298449488,867.884263474365,141.09691953464));
#68139=CARTESIAN_POINT('Ctrl Pts',(82.8312100648549,867.943076473732,141.128963473328));
#68140=CARTESIAN_POINT('Ctrl Pts',(82.8801593896866,868.0524566344,141.191772743508));
#68141=CARTESIAN_POINT('Ctrl Pts',(82.9170035013509,868.101937690783,141.221947076889));
#68142=CARTESIAN_POINT('Ctrl Pts',(83.009959191949,868.18342857881,141.275509009122));
#68143=CARTESIAN_POINT('Ctrl Pts',(83.0649190752211,868.215021557577,141.298539983206));
#68144=CARTESIAN_POINT('Ctrl Pts',(83.1853768504071,868.256450243687,141.334418913629));
#68145=CARTESIAN_POINT('Ctrl Pts',(83.2495943888809,868.266288666004,141.347114898385));
#68146=CARTESIAN_POINT('Ctrl Pts',(83.3790332430002,868.263175011208,141.36049940558));
#68147=CARTESIAN_POINT('Ctrl Pts',(83.4429676032448,868.250582689113,141.361226697384));
#68148=CARTESIAN_POINT('Ctrl Pts',(83.5630303392802,868.204478494439,141.350528099059));
#68149=CARTESIAN_POINT('Ctrl Pts',(83.6179099476324,868.17149099333,141.339236118848));
#68150=CARTESIAN_POINT('Ctrl Pts',(83.7120126809746,868.08870182261,141.305773167139));
#68151=CARTESIAN_POINT('Ctrl Pts',(83.7500132392623,868.039595570044,141.283833595494));
#68152=CARTESIAN_POINT('Ctrl Pts',(83.8038217444869,867.931080451226,141.231913675163));
#68153=CARTESIAN_POINT('Ctrl Pts',(83.8186384842597,867.872629644873,141.202336118948));
#68154=CARTESIAN_POINT('Ctrl Pts',(83.8223754593258,867.753598109998,141.139261029725));
#68155=CARTESIAN_POINT('Ctrl Pts',(83.8105849526875,867.694168199017,141.106304557215));
#68156=CARTESIAN_POINT('Ctrl Pts',(83.7614542221758,867.584234698682,141.042545515433));
#68157=CARTESIAN_POINT('Ctrl Pts',(83.7246512805773,867.534689143135,141.012311531101));
#68158=CARTESIAN_POINT('Ctrl Pts',(83.6312444949943,867.452512065021,140.958868320093));
#68159=CARTESIAN_POINT('Ctrl Pts',(83.5756574156258,867.420476026033,140.9360798409));
#68160=CARTESIAN_POINT('Ctrl Pts',(83.4531182214787,867.378352351999,140.900959048412));
#68161=CARTESIAN_POINT('Ctrl Pts',(83.3874399907159,867.368504212583,140.888883080505));
#68162=CARTESIAN_POINT('Ctrl Pts',(83.3208923352077,867.370572634924,140.882945801216));
#68163=CARTESIAN_POINT('Origin',(92.5194077263639,858.163512847548,125.615541683647));
#68164=CARTESIAN_POINT('',(92.5194077263639,853.591406436911,135.486639673687));
#68165=CARTESIAN_POINT('',(92.5194077263671,855.486945714773,136.253723814067));
#68166=CARTESIAN_POINT('Ctrl Pts',(92.5194077263639,853.591406436911,135.486639673687));
#68167=CARTESIAN_POINT('Ctrl Pts',(92.3869852387689,853.593396837675,135.481008065839));
#68168=CARTESIAN_POINT('Ctrl Pts',(92.2557551130715,853.619204273559,135.485269936815));
#68169=CARTESIAN_POINT('Ctrl Pts',(92.0085420427403,853.716672443918,135.512627696012));
#68170=CARTESIAN_POINT('Ctrl Pts',(91.8952729849214,853.788045926648,135.535713828907));
#68171=CARTESIAN_POINT('Ctrl Pts',(91.7041813968413,853.967450612033,135.597409337442));
#68172=CARTESIAN_POINT('Ctrl Pts',(91.6282910646732,854.073760618473,135.63542470618));
#68173=CARTESIAN_POINT('Ctrl Pts',(91.5248240399265,854.306889833465,135.721369193424));
#68174=CARTESIAN_POINT('Ctrl Pts',(91.498156989476,854.431366263457,135.768440963004));
#68175=CARTESIAN_POINT('Ctrl Pts',(91.4978432522669,854.681894117513,135.866103359209));
#68176=CARTESIAN_POINT('Ctrl Pts',(91.5242112377685,854.805465584329,135.915748516764));
#68177=CARTESIAN_POINT('Ctrl Pts',(91.6273321357412,855.035858649374,136.012159618501));
#68178=CARTESIAN_POINT('Ctrl Pts',(91.7035225991336,855.140199456724,136.05794316828));
#68179=CARTESIAN_POINT('Ctrl Pts',(91.894563280928,855.312867765503,136.138851218061));
#68180=CARTESIAN_POINT('Ctrl Pts',(92.0071264222377,855.37993844689,136.173317235713));
#68181=CARTESIAN_POINT('Ctrl Pts',(92.2540883379612,855.468855656258,136.226582411463));
#68182=CARTESIAN_POINT('Ctrl Pts',(92.3860910407434,855.490051831638,136.24493541706));
#68183=CARTESIAN_POINT('Ctrl Pts',(92.5194077263704,855.486945714773,136.253723814067));
#68184=CARTESIAN_POINT('',(92.5194077248472,856.129737102166,134.435020220354));
#68185=CARTESIAN_POINT('',(92.5194077263639,859.12654198779,125.955908766714));
#68186=CARTESIAN_POINT('Ctrl Pts',(93.32793357901,855.744463731389,134.332967522652));
#68187=CARTESIAN_POINT('Ctrl Pts',(93.4093156004398,855.64506638241,134.297837136329));
#68188=CARTESIAN_POINT('Ctrl Pts',(93.4692768118077,855.53237144291,134.255690021426));
#68189=CARTESIAN_POINT('Ctrl Pts',(93.5396671732254,855.293061111367,134.162258027501));
#68190=CARTESIAN_POINT('Ctrl Pts',(93.5494080886043,855.168778069024,134.111889615515));
#68191=CARTESIAN_POINT('Ctrl Pts',(93.516969247092,854.924305549308,134.009632276761));
#68192=CARTESIAN_POINT('Ctrl Pts',(93.4748730284245,854.806481321232,133.958727374903));
#68193=CARTESIAN_POINT('Ctrl Pts',(93.3436027548005,854.592928423506,133.863485836907));
#68194=CARTESIAN_POINT('Ctrl Pts',(93.2554740842456,854.499329540317,133.820091895569));
#68195=CARTESIAN_POINT('Ctrl Pts',(93.0444811877202,854.349507278583,133.747043814263));
#68196=CARTESIAN_POINT('Ctrl Pts',(92.9235975765563,854.29475660701,133.71810390374));
#68197=CARTESIAN_POINT('Ctrl Pts',(92.6661945033903,854.232349777071,133.678837881516));
#68198=CARTESIAN_POINT('Ctrl Pts',(92.5322843037635,854.224850203096,133.66870703206));
#68199=CARTESIAN_POINT('Ctrl Pts',(92.2662046346305,854.258256659072,133.668109602026));
#68200=CARTESIAN_POINT('Ctrl Pts',(92.136710866001,854.299454317514,133.677892507997));
#68201=CARTESIAN_POINT('Ctrl Pts',(91.9013189712622,854.426184042731,133.716192184587));
#68202=CARTESIAN_POINT('Ctrl Pts',(91.7978064893072,854.510525515979,133.744349840843));
#68203=CARTESIAN_POINT('Ctrl Pts',(91.6322096096441,854.710350802253,133.814878686914));
#68204=CARTESIAN_POINT('Ctrl Pts',(91.5713447639343,854.823562646887,133.85641632742));
#68205=CARTESIAN_POINT('Ctrl Pts',(91.499587638132,855.064526277156,133.947762061178));
#68206=CARTESIAN_POINT('Ctrl Pts',(91.4893575457721,855.189912359493,133.996678644227));
#68207=CARTESIAN_POINT('Ctrl Pts',(91.5211783924667,855.435796401683,134.095658444129));
#68208=CARTESIAN_POINT('Ctrl Pts',(91.562745426317,855.553933683864,134.144770788845));
#68209=CARTESIAN_POINT('Ctrl Pts',(91.6929888099045,855.768526170092,134.23761812767));
#68210=CARTESIAN_POINT('Ctrl Pts',(91.780795636183,855.862708766721,134.280410370037));
#68211=CARTESIAN_POINT('Ctrl Pts',(91.9923647252827,856.014084050154,134.354043169661));
#68212=CARTESIAN_POINT('Ctrl Pts',(92.1144722446957,856.069344892335,134.384015773502));
#68213=CARTESIAN_POINT('Ctrl Pts',(92.3743793281731,856.131368156919,134.425948539406));
#68214=CARTESIAN_POINT('Ctrl Pts',(92.5095148085389,856.13806247407,134.437694882898));
#68215=CARTESIAN_POINT('Ctrl Pts',(92.7759339221879,856.102418823341,134.441241581973));
#68216=CARTESIAN_POINT('Ctrl Pts',(92.9046446726391,856.060488970577,134.433024209589));
#68217=CARTESIAN_POINT('Ctrl Pts',(93.0804582363484,855.964749147531,134.406051609777));
#68218=CARTESIAN_POINT('Ctrl Pts',(93.1359273119399,855.927392662453,134.394615035788));
#68219=CARTESIAN_POINT('Ctrl Pts',(93.2389320751269,855.842740273728,134.367091940892));
#68220=CARTESIAN_POINT('Ctrl Pts',(93.2861021604945,855.795555262804,134.351024998579));
#68221=CARTESIAN_POINT('Ctrl Pts',(93.32793357901,855.744463731389,134.332967522652));
#68222=CARTESIAN_POINT('Ctrl Pts',(92.5194077263704,855.486945714773,136.253723814067));
#68223=CARTESIAN_POINT('Ctrl Pts',(92.5196238573676,855.486940679183,136.253738061683));
#68224=CARTESIAN_POINT('Ctrl Pts',(92.5198399918204,855.48693557973,136.253752284132));
#68225=CARTESIAN_POINT('Ctrl Pts',(92.5200561296971,855.486930416408,136.253766481407));
#68226=CARTESIAN_POINT('Ctrl Pts',(92.6499040778617,855.483828476222,136.262295699054));
#68227=CARTESIAN_POINT('Ctrl Pts',(92.7786346708171,855.457732528654,136.26158192679));
#68228=CARTESIAN_POINT('Ctrl Pts',(93.0225962035067,855.361385542605,136.240833318348));
#68229=CARTESIAN_POINT('Ctrl Pts',(93.1351240435946,855.291130048563,136.220571403863));
#68230=CARTESIAN_POINT('Ctrl Pts',(93.3262758568272,855.115108652454,136.162215494075));
#68231=CARTESIAN_POINT('Ctrl Pts',(93.4028833429568,855.010991636153,136.124644857631));
#68232=CARTESIAN_POINT('Ctrl Pts',(93.5095832636384,854.781822808916,136.036846104054));
#68233=CARTESIAN_POINT('Ctrl Pts',(93.5382981003373,854.658943603091,135.987427530001));
#68234=CARTESIAN_POINT('Ctrl Pts',(93.543028293216,854.410643148742,135.883789969737));
#68235=CARTESIAN_POINT('Ctrl Pts',(93.5187522798023,854.287643953618,135.830580521326));
#68236=CARTESIAN_POINT('Ctrl Pts',(93.4198665220468,854.058385092743,135.72843693595));
#68237=CARTESIAN_POINT('Ctrl Pts',(93.3461919613144,853.954308671273,135.680491457946));
#68238=CARTESIAN_POINT('Ctrl Pts',(93.157337423882,853.777631677803,135.596164976474));
#68239=CARTESIAN_POINT('Ctrl Pts',(93.0433585602817,853.707320562923,135.56082808586));
#68240=CARTESIAN_POINT('Ctrl Pts',(92.7931216418974,853.613345927679,135.509064500091));
#68241=CARTESIAN_POINT('Ctrl Pts',(92.6596620315709,853.589953134473,135.492874846329));
#68242=CARTESIAN_POINT('Ctrl Pts',(92.5229080805847,853.591357987078,135.486790254446));
#68243=CARTESIAN_POINT('Ctrl Pts',(92.521157799348,853.591380132115,135.486714100055));
#68244=CARTESIAN_POINT('Ctrl Pts',(92.5194077263639,853.591406436911,135.486639673688));
#68245=CARTESIAN_POINT('Origin',(92.5194077263639,858.163512847548,125.615541683647));
#68246=CARTESIAN_POINT('',(92.5194077263639,856.500096216042,131.822436927135));
#68247=CARTESIAN_POINT('Origin',(92.5194077263639,856.028673985433,131.655820359868));
#68248=CARTESIAN_POINT('',(92.5194077263641,855.004575041423,136.053840440156));
#68249=CARTESIAN_POINT('',(92.5194077263639,858.634935078157,125.782158250914));
#68250=CARTESIAN_POINT('Ctrl Pts',(92.5197874159677,854.076647188808,135.678402926227));
#68251=CARTESIAN_POINT('Ctrl Pts',(92.4585117931719,854.077656815856,135.675406667411));
#68252=CARTESIAN_POINT('Ctrl Pts',(92.3977223504281,854.089098293605,135.676698335242));
#68253=CARTESIAN_POINT('Ctrl Pts',(92.2785603320437,854.133529362063,135.688044747866));
#68254=CARTESIAN_POINT('Ctrl Pts',(92.2219767659596,854.167746440683,135.698683659406));
#68255=CARTESIAN_POINT('Ctrl Pts',(92.1260534852906,854.254541137588,135.728106029539));
#68256=CARTESIAN_POINT('Ctrl Pts',(92.0876826855216,854.3062519916,135.746594698822));
#68257=CARTESIAN_POINT('Ctrl Pts',(92.034624053689,854.420218150904,135.788973069629));
#68258=CARTESIAN_POINT('Ctrl Pts',(92.0204609285167,854.481324738186,135.81243758112));
#68259=CARTESIAN_POINT('Ctrl Pts',(92.0184661537579,854.604705873835,135.861361862463));
#68260=CARTESIAN_POINT('Ctrl Pts',(92.0306919009851,854.665742659649,135.886337827351));
#68261=CARTESIAN_POINT('Ctrl Pts',(92.0802382756373,854.779570179844,135.934687374985));
#68262=CARTESIAN_POINT('Ctrl Pts',(92.1172050570094,854.83116827952,135.95756949966));
#68263=CARTESIAN_POINT('Ctrl Pts',(92.2102277996603,854.91663570645,135.997708992039));
#68264=CARTESIAN_POINT('Ctrl Pts',(92.2650813235398,854.949957248097,136.01466711033));
#68265=CARTESIAN_POINT('Ctrl Pts',(92.3858052547534,854.99462728357,136.040691835628));
#68266=CARTESIAN_POINT('Ctrl Pts',(92.4505098709428,855.005607101473,136.049529447048));
#68267=CARTESIAN_POINT('Ctrl Pts',(92.5811610900851,855.003670969154,136.057712806867));
#68268=CARTESIAN_POINT('Ctrl Pts',(92.6458634843089,854.99086342945,136.057012613005));
#68269=CARTESIAN_POINT('Ctrl Pts',(92.7668257473756,854.943042171451,136.045937182797));
#68270=CARTESIAN_POINT('Ctrl Pts',(92.8219300964058,854.90853571467,136.035684857441));
#68271=CARTESIAN_POINT('Ctrl Pts',(92.9153449806096,854.822087121721,136.006748439735));
#68272=CARTESIAN_POINT('Ctrl Pts',(92.952700755937,854.770970449032,135.988334955313));
#68273=CARTESIAN_POINT('Ctrl Pts',(93.0045216658271,854.658567997623,135.945655893991));
#68274=CARTESIAN_POINT('Ctrl Pts',(93.0183716537132,854.598357073756,135.921791765898));
#68275=CARTESIAN_POINT('Ctrl Pts',(93.0203356164198,854.476759363803,135.871873177225));
#68276=CARTESIAN_POINT('Ctrl Pts',(93.0083336030846,854.416559419792,135.846303590804));
#68277=CARTESIAN_POINT('Ctrl Pts',(92.959785965243,854.304353847261,135.797112369177));
#68278=CARTESIAN_POINT('Ctrl Pts',(92.9236806560829,854.25343244026,135.773968282823));
#68279=CARTESIAN_POINT('Ctrl Pts',(92.8311363658633,854.166994431878,135.732989350332));
#68280=CARTESIAN_POINT('Ctrl Pts',(92.7752438274135,854.132642228019,135.715670430145));
#68281=CARTESIAN_POINT('Ctrl Pts',(92.6521955638388,854.086780861494,135.689912134253));
#68282=CARTESIAN_POINT('Ctrl Pts',(92.5863456734611,854.075550520771,135.681657495608));
#68283=CARTESIAN_POINT('Ctrl Pts',(92.5197874159677,854.076647188808,135.678402926227));
#68284=CARTESIAN_POINT('Origin',(91.9844712578892,864.72423914453,127.934324344724));
#68285=CARTESIAN_POINT('',(91.9844712578893,860.070334590592,138.256898317882));
#68286=CARTESIAN_POINT('',(91.9844712578948,861.780675301002,139.107905031699));
#68287=CARTESIAN_POINT('Ctrl Pts',(91.9844712578893,860.070334590592,138.256898317882));
#68288=CARTESIAN_POINT('Ctrl Pts',(91.8627158249353,860.075094927363,138.243429497726));
#68289=CARTESIAN_POINT('Ctrl Pts',(91.7417814147924,860.100971972796,138.240598889852));
#68290=CARTESIAN_POINT('Ctrl Pts',(91.5146801986006,860.193007929216,138.256390270714));
#68291=CARTESIAN_POINT('Ctrl Pts',(91.410885331243,860.258332094181,138.274897558361));
#68292=CARTESIAN_POINT('Ctrl Pts',(91.2338481590702,860.421363739986,138.331248363508));
#68293=CARTESIAN_POINT('Ctrl Pts',(91.162822221636,860.517698379504,138.368705872945));
#68294=CARTESIAN_POINT('Ctrl Pts',(91.0640827219528,860.729177979568,138.458223067825));
#68295=CARTESIAN_POINT('Ctrl Pts',(91.0379218314488,860.84226772842,138.509499129176));
#68296=CARTESIAN_POINT('Ctrl Pts',(91.0349795142351,861.06886741443,138.619135384539));
#68297=CARTESIAN_POINT('Ctrl Pts',(91.0583329386905,861.180068266577,138.67640787922));
#68298=CARTESIAN_POINT('Ctrl Pts',(91.1517636407079,861.386358342695,138.790233884351));
#68299=CARTESIAN_POINT('Ctrl Pts',(91.2214484393768,861.479291492061,138.845695359929));
#68300=CARTESIAN_POINT('Ctrl Pts',(91.3989637829188,861.634087737731,138.947624208233));
#68301=CARTESIAN_POINT('Ctrl Pts',(91.5057040424711,861.694093105123,138.993029281356));
#68302=CARTESIAN_POINT('Ctrl Pts',(91.7377050324959,861.769897318938,139.065243611614));
#68303=CARTESIAN_POINT('Ctrl Pts',(91.8603246959307,861.786317685181,139.091940560826));
#68304=CARTESIAN_POINT('Ctrl Pts',(91.9844712579004,861.780675301002,139.107905031699));
#68305=CARTESIAN_POINT('',(91.9844712578892,862.468675832393,137.161287414449));
#68306=CARTESIAN_POINT('',(91.9844712578892,865.618135317149,128.250257497861));
#68307=CARTESIAN_POINT('Ctrl Pts',(92.6682530675173,862.180366103655,137.102728175585));
#68308=CARTESIAN_POINT('Ctrl Pts',(92.7502695251889,862.099853184563,137.074272185756));
#68309=CARTESIAN_POINT('Ctrl Pts',(92.8155108599149,862.006674064341,137.037991754908));
#68310=CARTESIAN_POINT('Ctrl Pts',(92.9083616649202,861.799018927021,136.951321458583));
#68311=CARTESIAN_POINT('Ctrl Pts',(92.9327116796763,861.685790236625,136.901157245529));
#68312=CARTESIAN_POINT('Ctrl Pts',(92.9324009227412,861.461039991637,136.796517089838));
#68313=CARTESIAN_POINT('Ctrl Pts',(92.9085802132645,861.351627285942,136.743117399261));
#68314=CARTESIAN_POINT('Ctrl Pts',(92.8158729018139,861.14701686133,136.638567071437));
#68315=CARTESIAN_POINT('Ctrl Pts',(92.7471178415109,861.053942346796,136.588426294817));
#68316=CARTESIAN_POINT('Ctrl Pts',(92.5723601967429,860.897351377711,136.49848947757));
#68317=CARTESIAN_POINT('Ctrl Pts',(92.4675255649409,860.83566182762,136.459661717188));
#68318=CARTESIAN_POINT('Ctrl Pts',(92.2357838564043,860.753720287111,136.399245605298));
#68319=CARTESIAN_POINT('Ctrl Pts',(92.1110558434138,860.734357835676,136.378275827917));
#68320=CARTESIAN_POINT('Ctrl Pts',(91.8639768320607,860.741537481803,136.357660451801));
#68321=CARTESIAN_POINT('Ctrl Pts',(91.7440388713179,860.766118890054,136.35733967831));
#68322=CARTESIAN_POINT('Ctrl Pts',(91.5227999959679,860.853694088448,136.375825488455));
#68323=CARTESIAN_POINT('Ctrl Pts',(91.4229996012723,860.914608698739,136.393830923029));
#68324=CARTESIAN_POINT('Ctrl Pts',(91.251069703936,861.06654232663,136.445923975402));
#68325=CARTESIAN_POINT('Ctrl Pts',(91.1806759039626,861.15633197131,136.479621376828));
#68326=CARTESIAN_POINT('Ctrl Pts',(91.0773365836193,861.356437160706,136.559796780827));
#68327=CARTESIAN_POINT('Ctrl Pts',(91.0464208576457,861.465307521388,136.60582157008));
#68328=CARTESIAN_POINT('Ctrl Pts',(91.0300669563244,861.69198937351,136.706504884572));
#68329=CARTESIAN_POINT('Ctrl Pts',(91.0472708384882,861.807620334639,136.760454565323));
#68330=CARTESIAN_POINT('Ctrl Pts',(91.129440914888,862.0214618439,136.865696497521));
#68331=CARTESIAN_POINT('Ctrl Pts',(91.1925423583627,862.117987326432,136.916033107454));
#68332=CARTESIAN_POINT('Ctrl Pts',(91.3574821764649,862.283015468729,137.008479942166));
#68333=CARTESIAN_POINT('Ctrl Pts',(91.4583119432808,862.34957786219,137.049608410124));
#68334=CARTESIAN_POINT('Ctrl Pts',(91.6849097744894,862.442378299146,137.116487651892));
#68335=CARTESIAN_POINT('Ctrl Pts',(91.8087559580481,862.467369957056,137.141459615132));
#68336=CARTESIAN_POINT('Ctrl Pts',(92.0488123358252,862.470743163164,137.169274624711));
#68337=CARTESIAN_POINT('Ctrl Pts',(92.1625686427008,862.453675369375,137.173922064465));
#68338=CARTESIAN_POINT('Ctrl Pts',(92.3852494302583,862.381833420401,137.165184058635));
#68339=CARTESIAN_POINT('Ctrl Pts',(92.4915585183589,862.325877002723,137.150955580858));
#68340=CARTESIAN_POINT('Ctrl Pts',(92.6138864410115,862.230723900541,137.120181006694));
#68341=CARTESIAN_POINT('Ctrl Pts',(92.6418835662023,862.206252195131,137.111877196191));
#68342=CARTESIAN_POINT('Ctrl Pts',(92.6682530675173,862.180366103655,137.102728175585));
#68343=CARTESIAN_POINT('Ctrl Pts',(91.9844712579004,861.780675301002,139.107905031699));
#68344=CARTESIAN_POINT('Ctrl Pts',(91.9847252321603,861.78066375803,139.107937691199));
#68345=CARTESIAN_POINT('Ctrl Pts',(91.9849792128138,861.780652122725,139.107970305759));
#68346=CARTESIAN_POINT('Ctrl Pts',(91.9852331998028,861.780640395039,139.108002875342));
#68347=CARTESIAN_POINT('Ctrl Pts',(92.1041663410571,861.775148733354,139.12325406104));
#68348=CARTESIAN_POINT('Ctrl Pts',(92.2223724148456,861.749504142137,139.128370146541));
#68349=CARTESIAN_POINT('Ctrl Pts',(92.4465953442894,861.659347904305,139.11695403917));
#68350=CARTESIAN_POINT('Ctrl Pts',(92.5501112531231,861.595130822051,139.100179018847));
#68351=CARTESIAN_POINT('Ctrl Pts',(92.727211844383,861.435404183338,139.04585931993));
#68352=CARTESIAN_POINT('Ctrl Pts',(92.7986758536721,861.341441607929,139.008776037852));
#68353=CARTESIAN_POINT('Ctrl Pts',(92.900160658882,861.134354217937,138.918422742171));
#68354=CARTESIAN_POINT('Ctrl Pts',(92.9282801907244,861.023150295102,138.865850362895));
#68355=CARTESIAN_POINT('Ctrl Pts',(92.9360129240651,860.797535988778,138.752101290057));
#68356=CARTESIAN_POINT('Ctrl Pts',(92.9144813096627,860.68537949621,138.691920212741));
#68357=CARTESIAN_POINT('Ctrl Pts',(92.8232846241425,860.4763410989,138.573017588116));
#68358=CARTESIAN_POINT('Ctrl Pts',(92.7538593971312,860.381597900411,138.515432329864));
#68359=CARTESIAN_POINT('Ctrl Pts',(92.577630711232,860.225172745614,138.412564543943));
#68360=CARTESIAN_POINT('Ctrl Pts',(92.4728924209734,860.164443079223,138.368035922534));
#68361=CARTESIAN_POINT('Ctrl Pts',(92.242325525263,860.084831516747,138.297703692825));
#68362=CARTESIAN_POINT('Ctrl Pts',(92.1188845109012,860.066208098854,138.272330710447));
#68363=CARTESIAN_POINT('Ctrl Pts',(91.990564827285,860.070109586947,138.257579005833));
#68364=CARTESIAN_POINT('Ctrl Pts',(91.9875177857031,860.070215478877,138.257235330647));
#68365=CARTESIAN_POINT('Ctrl Pts',(91.9844712578893,860.070334590591,138.256898317882));
#68366=CARTESIAN_POINT('Origin',(91.9844712578892,864.72423914453,127.934324344724));
#68367=CARTESIAN_POINT('',(91.9844712578892,863.060822513024,134.141219588213));
#68368=CARTESIAN_POINT('Origin',(91.9844712578892,862.589400282415,133.974603020945));
#68369=CARTESIAN_POINT('',(91.9844712578892,861.377906466998,138.90283513076));
#68370=CARTESIAN_POINT('',(91.9844712578892,865.195661375139,128.100940911991));
#68371=CARTESIAN_POINT('Ctrl Pts',(91.9846725918056,860.475894112785,138.454072412269));
#68372=CARTESIAN_POINT('Ctrl Pts',(91.920362935665,860.478484117757,138.44666658428));
#68373=CARTESIAN_POINT('Ctrl Pts',(91.8564894643335,860.492246409255,138.444883783608));
#68374=CARTESIAN_POINT('Ctrl Pts',(91.7367744281551,860.540932435595,138.452791544227));
#68375=CARTESIAN_POINT('Ctrl Pts',(91.6821403542686,860.575344412562,138.462389293359));
#68376=CARTESIAN_POINT('Ctrl Pts',(91.5893477943355,860.660705211688,138.49183868113));
#68377=CARTESIAN_POINT('Ctrl Pts',(91.5521796696783,860.710782297006,138.511394943521));
#68378=CARTESIAN_POINT('Ctrl Pts',(91.4998807546353,860.821120474435,138.558444180532));
#68379=CARTESIAN_POINT('Ctrl Pts',(91.4857576205996,860.880386978147,138.585587421364));
#68380=CARTESIAN_POINT('Ctrl Pts',(91.4833370573924,860.999900945424,138.643966489552));
#68381=CARTESIAN_POINT('Ctrl Pts',(91.4953968609785,861.058927026634,138.674656249663));
#68382=CARTESIAN_POINT('Ctrl Pts',(91.5444300072723,861.168289090617,138.735417500556));
#68383=CARTESIAN_POINT('Ctrl Pts',(91.5811054278994,861.217528824092,138.764910926337));
#68384=CARTESIAN_POINT('Ctrl Pts',(91.6744672369076,861.299397019212,138.818756454622));
#68385=CARTESIAN_POINT('Ctrl Pts',(91.7304602702546,861.331162118061,138.842583962484));
#68386=CARTESIAN_POINT('Ctrl Pts',(91.8526214401056,861.371715525066,138.880466094217));
#68387=CARTESIAN_POINT('Ctrl Pts',(91.9174404826097,861.380692004442,138.894411746735));
#68388=CARTESIAN_POINT('Ctrl Pts',(92.0476183726505,861.37528556506,138.910772090592));
#68389=CARTESIAN_POINT('Ctrl Pts',(92.1117370714536,861.36136128817,138.913229966425));
#68390=CARTESIAN_POINT('Ctrl Pts',(92.2314396922143,861.312484217547,138.906295317189));
#68391=CARTESIAN_POINT('Ctrl Pts',(92.285884526361,861.27822964846,138.897083743854));
#68392=CARTESIAN_POINT('Ctrl Pts',(92.3786966175915,861.193272480086,138.867932763898));
#68393=CARTESIAN_POINT('Ctrl Pts',(92.4159843165664,861.143403781542,138.848254038664));
#68394=CARTESIAN_POINT('Ctrl Pts',(92.4685134912536,861.033772617879,138.800642507967));
#68395=CARTESIAN_POINT('Ctrl Pts',(92.482818936385,860.97503686455,138.773092214655));
#68396=CARTESIAN_POINT('Ctrl Pts',(92.4858877403505,860.855990276812,138.713567890834));
#68397=CARTESIAN_POINT('Ctrl Pts',(92.4740447195081,860.796878658118,138.682115382241));
#68398=CARTESIAN_POINT('Ctrl Pts',(92.4251369915085,860.687075956209,138.620034389912));
#68399=CARTESIAN_POINT('Ctrl Pts',(92.3882876298724,860.637490360132,138.589996275897));
#68400=CARTESIAN_POINT('Ctrl Pts',(92.2948713795416,860.555557021582,138.536029188218));
#68401=CARTESIAN_POINT('Ctrl Pts',(92.2392727738594,860.523816579573,138.512537365152));
#68402=CARTESIAN_POINT('Ctrl Pts',(92.1168172974433,860.482532432661,138.47525047117));
#68403=CARTESIAN_POINT('Ctrl Pts',(92.0511735362836,860.473215855938,138.461730586569));
#68404=CARTESIAN_POINT('Ctrl Pts',(91.9846725918056,860.475894112785,138.454072412269));
#68405=CARTESIAN_POINT('Origin',(98.0156115335941,849.762095315549,122.646196458769));
#68406=CARTESIAN_POINT('',(98.015611533594,845.187014905945,132.525709033565));
#68407=CARTESIAN_POINT('',(98.0156115335941,847.091594819924,133.267213743794));
#68408=CARTESIAN_POINT('Ctrl Pts',(98.015611533594,845.187014905945,132.525709033565));
#68409=CARTESIAN_POINT('Ctrl Pts',(97.8860206821817,845.189387618146,132.518995719895));
#68410=CARTESIAN_POINT('Ctrl Pts',(97.7575089471629,845.214593932317,132.521688408218));
#68411=CARTESIAN_POINT('Ctrl Pts',(97.5120105461576,845.310119933585,132.545461559902));
#68412=CARTESIAN_POINT('Ctrl Pts',(97.3980938198495,845.381109130524,132.566957650488));
#68413=CARTESIAN_POINT('Ctrl Pts',(97.2050733706479,845.560356389836,132.625726894498));
#68414=CARTESIAN_POINT('Ctrl Pts',(97.1280580197775,845.66700622652,132.662474778526));
#68415=CARTESIAN_POINT('Ctrl Pts',(97.0224968822141,845.901512098029,132.746010158396));
#68416=CARTESIAN_POINT('Ctrl Pts',(96.9949565268277,846.027021178794,132.79196184265));
#68417=CARTESIAN_POINT('Ctrl Pts',(96.9934840518301,846.279305202701,132.887078058931));
#68418=CARTESIAN_POINT('Ctrl Pts',(97.0193040736023,846.403578364203,132.935303568196));
#68419=CARTESIAN_POINT('Ctrl Pts',(97.1210286511537,846.63454771516,133.028555468656));
#68420=CARTESIAN_POINT('Ctrl Pts',(97.1959561217158,846.738944221774,133.072675894541));
#68421=CARTESIAN_POINT('Ctrl Pts',(97.3862532747563,846.914340584495,133.151917655163));
#68422=CARTESIAN_POINT('Ctrl Pts',(97.5001643386863,846.983197005934,133.186150376441));
#68423=CARTESIAN_POINT('Ctrl Pts',(97.749255929632,847.073593462009,133.23920802476));
#68424=CARTESIAN_POINT('Ctrl Pts',(97.8817488809734,847.094933194111,133.257735945125));
#68425=CARTESIAN_POINT('Ctrl Pts',(98.0155294910738,847.091596869053,133.267207936134));
#68426=CARTESIAN_POINT('Ctrl Pts',(98.01555683863,847.091596187038,133.267209872408));
#68427=CARTESIAN_POINT('Ctrl Pts',(98.0155841861368,847.091595503995,133.267211808294));
#68428=CARTESIAN_POINT('Ctrl Pts',(98.0156115335941,847.091594819924,133.267213743794));
#68429=CARTESIAN_POINT('',(98.015611532426,847.733004325138,131.452420025248));
#68430=CARTESIAN_POINT('',(98.0156115335941,850.725124455792,122.986563541837));
#68431=CARTESIAN_POINT('Ctrl Pts',(98.936236838463,847.171692600385,131.303060137992));
#68432=CARTESIAN_POINT('Ctrl Pts',(98.9939218247441,847.058514135643,131.263059039063));
#68433=CARTESIAN_POINT('Ctrl Pts',(99.0275612513901,846.936543658766,131.217633635405));
#68434=CARTESIAN_POINT('Ctrl Pts',(99.0430285415981,846.68872509615,131.121194544736));
#68435=CARTESIAN_POINT('Ctrl Pts',(99.0247039124607,846.565292673627,131.071126770575));
#68436=CARTESIAN_POINT('Ctrl Pts',(98.9379656821865,846.332630237766,130.97304351506));
#68437=CARTESIAN_POINT('Ctrl Pts',(98.8701656260265,846.225696394909,130.925987643825));
#68438=CARTESIAN_POINT('Ctrl Pts',(98.6933028673295,846.04267853967,130.841538223022));
#68439=CARTESIAN_POINT('Ctrl Pts',(98.5857455164236,845.968471543597,130.804998030732));
#68440=CARTESIAN_POINT('Ctrl Pts',(98.3449329098207,845.863421827441,130.74777408195));
#68441=CARTESIAN_POINT('Ctrl Pts',(98.2139531641199,845.83363004536,130.727655487479));
#68442=CARTESIAN_POINT('Ctrl Pts',(97.9472209851749,845.823163418232,130.706746890368));
#68443=CARTESIAN_POINT('Ctrl Pts',(97.8140650190188,845.842129285687,130.705969823394));
#68444=CARTESIAN_POINT('Ctrl Pts',(97.560307050921,845.927050063964,130.723579297893));
#68445=CARTESIAN_POINT('Ctrl Pts',(97.4423967320263,845.992764711925,130.742027337513));
#68446=CARTESIAN_POINT('Ctrl Pts',(97.239644857422,846.162913146625,130.795672655142));
#68447=CARTESIAN_POINT('Ctrl Pts',(97.156878543148,846.265714279697,130.830354579779));
#68448=CARTESIAN_POINT('Ctrl Pts',(97.0389582355761,846.493635253383,130.910813392422));
#68449=CARTESIAN_POINT('Ctrl Pts',(97.0044940229917,846.616293916566,130.955689858244));
#68450=CARTESIAN_POINT('Ctrl Pts',(96.9878693864634,846.866015909571,131.05013109374));
#68451=CARTESIAN_POINT('Ctrl Pts',(97.0058311683029,846.990635805093,131.098776880444));
#68452=CARTESIAN_POINT('Ctrl Pts',(97.092014528966,847.224825990711,131.193623675761));
#68453=CARTESIAN_POINT('Ctrl Pts',(97.1592341379057,847.332182848818,131.238925853845));
#68454=CARTESIAN_POINT('Ctrl Pts',(97.3351303579775,847.51643783525,131.321050893748));
#68455=CARTESIAN_POINT('Ctrl Pts',(97.4424456345311,847.591284427378,131.357009137874));
#68456=CARTESIAN_POINT('Ctrl Pts',(97.6841667899337,847.697740031898,131.414765803074));
#68457=CARTESIAN_POINT('Ctrl Pts',(97.8165152546305,847.727785063144,131.435826286133));
#68458=CARTESIAN_POINT('Ctrl Pts',(98.0858062957287,847.737366409717,131.459224303796));
#68459=CARTESIAN_POINT('Ctrl Pts',(98.2201148404824,847.717359646841,131.461533582153));
#68460=CARTESIAN_POINT('Ctrl Pts',(98.4739706161407,847.630158343464,131.446858062285));
#68461=CARTESIAN_POINT('Ctrl Pts',(98.5910799617756,847.563868469895,131.430031034307));
#68462=CARTESIAN_POINT('Ctrl Pts',(98.7424151099261,847.435709208592,131.391600308076));
#68463=CARTESIAN_POINT('Ctrl Pts',(98.7885567607571,847.388283410839,131.376604898282));
#68464=CARTESIAN_POINT('Ctrl Pts',(98.870809467233,847.285272572634,131.342593306167));
#68465=CARTESIAN_POINT('Ctrl Pts',(98.9065860045221,847.229867804717,131.323621223611));
#68466=CARTESIAN_POINT('Ctrl Pts',(98.936236838463,847.171692600385,131.303060137992));
#68467=CARTESIAN_POINT('Ctrl Pts',(98.0156115335941,847.091594819924,133.267213743794));
#68468=CARTESIAN_POINT('Ctrl Pts',(98.1445998794982,847.088368296269,133.27634281783));
#68469=CARTESIAN_POINT('Ctrl Pts',(98.2724871025139,847.062263821109,133.276878366808));
#68470=CARTESIAN_POINT('Ctrl Pts',(98.5159940599694,846.965770072614,133.259805381712));
#68471=CARTESIAN_POINT('Ctrl Pts',(98.6288368496251,846.895023685516,133.241812544452));
#68472=CARTESIAN_POINT('Ctrl Pts',(98.8203608187985,846.717967585965,133.188537930749));
#68473=CARTESIAN_POINT('Ctrl Pts',(98.8971756269128,846.613412536387,133.15377706999));
#68474=CARTESIAN_POINT('Ctrl Pts',(99.0044970511687,846.383468490965,133.071492895752));
#68475=CARTESIAN_POINT('Ctrl Pts',(99.0337108485038,846.260298058927,133.024740051622));
#68476=CARTESIAN_POINT('Ctrl Pts',(99.0398162769885,846.011238720184,132.925525072838));
#68477=CARTESIAN_POINT('Ctrl Pts',(99.0163400049041,845.887814160082,132.874029437785));
#68478=CARTESIAN_POINT('Ctrl Pts',(98.9190697926459,845.657464834316,132.773966888127));
#68479=CARTESIAN_POINT('Ctrl Pts',(98.8460794673428,845.552803403249,132.72638911324));
#68480=CARTESIAN_POINT('Ctrl Pts',(98.6591898310977,845.375795008331,132.642011323911));
#68481=CARTESIAN_POINT('Ctrl Pts',(98.5467424974315,845.305448130961,132.606138060299));
#68482=CARTESIAN_POINT('Ctrl Pts',(98.2981984872136,845.210182679547,132.551969565868));
#68483=CARTESIAN_POINT('Ctrl Pts',(98.1646041368167,845.18604461951,132.534146128871));
#68484=CARTESIAN_POINT('Ctrl Pts',(98.024693361461,845.186876679982,132.526190973292));
#68485=CARTESIAN_POINT('Ctrl Pts',(98.0201517849047,845.186931777317,132.525944236365));
#68486=CARTESIAN_POINT('Ctrl Pts',(98.015611533594,845.187014905945,132.525709033565));
#68487=CARTESIAN_POINT('Origin',(98.0156115335941,849.762095315549,122.646196458769));
#68488=CARTESIAN_POINT('',(98.0156115335941,848.098678684043,128.853091702258));
#68489=CARTESIAN_POINT('Origin',(98.0156115335941,847.627256453434,128.686475134991));
#68490=CARTESIAN_POINT('',(98.0156115335942,846.606301159591,133.075600622152));
#68491=CARTESIAN_POINT('',(98.0156115335941,850.233517546158,122.812813026036));
#68492=CARTESIAN_POINT('Ctrl Pts',(98.0158176429449,845.673946435203,132.712688122743));
#68493=CARTESIAN_POINT('Ctrl Pts',(97.9557714435446,845.675125151855,132.709278802009));
#68494=CARTESIAN_POINT('Ctrl Pts',(97.8961842020983,845.686350334974,132.70990421349));
#68495=CARTESIAN_POINT('Ctrl Pts',(97.7777646789254,845.730085723621,132.719534051333));
#68496=CARTESIAN_POINT('Ctrl Pts',(97.7208514348171,845.764265697177,132.729309055622));
#68497=CARTESIAN_POINT('Ctrl Pts',(97.6240779947701,845.851282269231,132.757040096443));
#68498=CARTESIAN_POINT('Ctrl Pts',(97.5852405293584,845.903285666734,132.774732778336));
#68499=CARTESIAN_POINT('Ctrl Pts',(97.5313805529879,846.018062097187,132.815590580301));
#68500=CARTESIAN_POINT('Ctrl Pts',(97.5168958887761,846.079669424561,132.838340589156));
#68501=CARTESIAN_POINT('Ctrl Pts',(97.5144934953664,846.203894714416,132.885832892649));
#68502=CARTESIAN_POINT('Ctrl Pts',(97.5265307410666,846.265258809389,132.910095601539));
#68503=CARTESIAN_POINT('Ctrl Pts',(97.5756135745257,846.379420823086,132.957054453336));
#68504=CARTESIAN_POINT('Ctrl Pts',(97.6121657000844,846.431077951219,132.979286002817));
#68505=CARTESIAN_POINT('Ctrl Pts',(97.7052144357998,846.517731302449,133.018934522713));
#68506=CARTESIAN_POINT('Ctrl Pts',(97.7608877180156,846.55177662378,133.03593394772));
#68507=CARTESIAN_POINT('Ctrl Pts',(97.8827489636195,846.596736518061,133.062031613723));
#68508=CARTESIAN_POINT('Ctrl Pts',(97.9475998140662,846.607579006291,133.071000881768));
#68509=CARTESIAN_POINT('Ctrl Pts',(98.0785141005218,846.605130157163,133.079858950843));
#68510=CARTESIAN_POINT('Ctrl Pts',(98.1433357321042,846.591935712411,133.079688276805));
#68511=CARTESIAN_POINT('Ctrl Pts',(98.2643323610686,846.543178024217,133.070008510938));
#68512=CARTESIAN_POINT('Ctrl Pts',(98.3193770988556,846.508158643057,133.060620053119));
#68513=CARTESIAN_POINT('Ctrl Pts',(98.4124730503905,846.420734531687,133.033627780465));
#68514=CARTESIAN_POINT('Ctrl Pts',(98.449625024441,846.369200341769,133.016292420463));
#68515=CARTESIAN_POINT('Ctrl Pts',(98.5010260186287,846.256121175603,132.975779766548));
#68516=CARTESIAN_POINT('Ctrl Pts',(98.5147027976635,846.195673548754,132.952989935427));
#68517=CARTESIAN_POINT('Ctrl Pts',(98.5164362709613,846.073700502084,132.904967362938));
#68518=CARTESIAN_POINT('Ctrl Pts',(98.5043714130655,846.013375760666,132.880202275878));
#68519=CARTESIAN_POINT('Ctrl Pts',(98.4557679898932,845.900960936697,132.832185571587));
#68520=CARTESIAN_POINT('Ctrl Pts',(98.4196344307866,845.849980782542,132.809406976519));
#68521=CARTESIAN_POINT('Ctrl Pts',(98.3270717501001,845.763555478679,132.768740178542));
#68522=CARTESIAN_POINT('Ctrl Pts',(98.2711793890321,845.729285195682,132.751360893904));
#68523=CARTESIAN_POINT('Ctrl Pts',(98.1481682221794,845.683688446436,132.725126126308));
#68524=CARTESIAN_POINT('Ctrl Pts',(98.082340963432,845.672640571612,132.716465203359));
#68525=CARTESIAN_POINT('Ctrl Pts',(98.0158176429449,845.673946435203,132.712688122743));
#68526=CARTESIAN_POINT('Origin',(98.9391056666407,856.284316734599,124.951370193141));
#68527=CARTESIAN_POINT('',(98.9391056666407,851.623398972203,135.2937872253));
#68528=CARTESIAN_POINT('',(98.9391056666684,853.352286325813,136.092318365703));
#68529=CARTESIAN_POINT('Ctrl Pts',(98.9391056666407,851.623398972202,135.2937872253));
#68530=CARTESIAN_POINT('Ctrl Pts',(98.8183330524074,851.629053230436,135.277789158166));
#68531=CARTESIAN_POINT('Ctrl Pts',(98.6983196784671,851.655643037619,135.271807650217));
#68532=CARTESIAN_POINT('Ctrl Pts',(98.4696960988426,851.75000232356,135.280508220464));
#68533=CARTESIAN_POINT('Ctrl Pts',(98.3639034533419,851.817950924658,135.29568569154));
#68534=CARTESIAN_POINT('Ctrl Pts',(98.1869989436827,851.984925764802,135.345082437744));
#68535=CARTESIAN_POINT('Ctrl Pts',(98.1170047732073,852.081550498225,135.378376918119));
#68536=CARTESIAN_POINT('Ctrl Pts',(98.0187924910619,852.294466426923,135.459840255075));
#68537=CARTESIAN_POINT('Ctrl Pts',(97.992575496003,852.408857935065,135.507449115179));
#68538=CARTESIAN_POINT('Ctrl Pts',(97.9895985571535,852.637951606723,135.6103718886));
#68539=CARTESIAN_POINT('Ctrl Pts',(98.0129429608198,852.750255777671,135.664633788996));
#68540=CARTESIAN_POINT('Ctrl Pts',(98.1063157764756,852.958199465322,135.773415305005));
#68541=CARTESIAN_POINT('Ctrl Pts',(98.1758294784201,853.051613466265,135.826864151084));
#68542=CARTESIAN_POINT('Ctrl Pts',(98.3527708738705,853.206970250865,135.926389951305));
#68543=CARTESIAN_POINT('Ctrl Pts',(98.4590917234256,853.266975125199,135.971421132707));
#68544=CARTESIAN_POINT('Ctrl Pts',(98.6911107358913,853.342817425497,136.045288422844));
#68545=CARTESIAN_POINT('Ctrl Pts',(98.8144028011606,853.358837770667,136.073781813223));
#68546=CARTESIAN_POINT('Ctrl Pts',(98.9391056666962,853.352286325813,136.092318365703));
#68547=CARTESIAN_POINT('',(98.9391056666407,854.035930319192,134.158027066904));
#68548=CARTESIAN_POINT('',(98.9391056666407,857.178212907218,125.267303346277));
#68549=CARTESIAN_POINT('Ctrl Pts',(99.7444889898849,853.592871976861,134.067617186048));
#68550=CARTESIAN_POINT('Ctrl Pts',(99.8069588554102,853.498040904391,134.034100676348));
#68551=CARTESIAN_POINT('Ctrl Pts',(99.8499951384563,853.394131802919,133.994027907069));
#68552=CARTESIAN_POINT('Ctrl Pts',(99.8941058454367,853.172904198033,133.90256064147));
#68553=CARTESIAN_POINT('Ctrl Pts',(99.892252186103,853.057446187517,133.851608511254));
#68554=CARTESIAN_POINT('Ctrl Pts',(99.8406410015003,852.83784124837,133.748786880744));
#68555=CARTESIAN_POINT('Ctrl Pts',(99.7921931413572,852.73559013722,133.697918339998));
#68556=CARTESIAN_POINT('Ctrl Pts',(99.654158688674,852.553845516766,133.601449561046));
#68557=CARTESIAN_POINT('Ctrl Pts',(99.5651869378705,852.476401247526,133.556833041976));
#68558=CARTESIAN_POINT('Ctrl Pts',(99.3573207936775,852.357727127421,133.480297322107));
#68559=CARTESIAN_POINT('Ctrl Pts',(99.2399940409375,852.318053092073,133.449250589549));
#68560=CARTESIAN_POINT('Ctrl Pts',(98.9930677634267,852.283546087162,133.405599447528));
#68561=CARTESIAN_POINT('Ctrl Pts',(98.8658169162329,852.289153971247,133.393455031611));
#68562=CARTESIAN_POINT('Ctrl Pts',(98.6241162920994,852.344770186552,133.389958777935));
#68563=CARTESIAN_POINT('Ctrl Pts',(98.5115956931786,852.392387528154,133.397779682731));
#68564=CARTESIAN_POINT('Ctrl Pts',(98.3136393964446,852.521503687909,133.430947474194));
#68565=CARTESIAN_POINT('Ctrl Pts',(98.2292083442512,852.600675071958,133.455405470348));
#68566=CARTESIAN_POINT('Ctrl Pts',(98.0944279978531,852.78300274833,133.518240807862));
#68567=CARTESIAN_POINT('Ctrl Pts',(98.0455084496729,852.884615981437,133.5561170655));
#68568=CARTESIAN_POINT('Ctrl Pts',(97.9892084364286,853.100540941266,133.641883711644));
#68569=CARTESIAN_POINT('Ctrl Pts',(97.9834987127821,853.213040772154,133.689191278475));
#68570=CARTESIAN_POINT('Ctrl Pts',(98.0189139096396,853.4378337081,133.789206986077));
#68571=CARTESIAN_POINT('Ctrl Pts',(98.0621465956036,853.547475589896,133.841039923547));
#68572=CARTESIAN_POINT('Ctrl Pts',(98.1917315482001,853.740332822469,133.938865302342));
#68573=CARTESIAN_POINT('Ctrl Pts',(98.2758632828868,853.822267946685,133.984045185969));
#68574=CARTESIAN_POINT('Ctrl Pts',(98.4759539706325,853.951122680629,134.063707114211));
#68575=CARTESIAN_POINT('Ctrl Pts',(98.5904779899877,853.996344171556,134.097292985126));
#68576=CARTESIAN_POINT('Ctrl Pts',(98.8349492336192,854.042463101807,134.147673402917));
#68577=CARTESIAN_POINT('Ctrl Pts',(98.9627182894318,854.04252045791,134.163832740225));
#68578=CARTESIAN_POINT('Ctrl Pts',(99.2001172126454,853.998579301805,134.174925253276));
#68579=CARTESIAN_POINT('Ctrl Pts',(99.3083638880813,853.95951169045,134.17179721312));
#68580=CARTESIAN_POINT('Ctrl Pts',(99.5114901090276,853.845473567317,134.148145651599));
#68581=CARTESIAN_POINT('Ctrl Pts',(99.6035212496963,853.769862238685,134.12697046325));
#68582=CARTESIAN_POINT('Ctrl Pts',(99.7023911478801,853.652789107984,134.088448609325));
#68583=CARTESIAN_POINT('Ctrl Pts',(99.7244040063591,853.623361565918,134.078393238462));
#68584=CARTESIAN_POINT('Ctrl Pts',(99.7444889898849,853.592871976861,134.067617186048));
#68585=CARTESIAN_POINT('Ctrl Pts',(98.9391056666962,853.352286325813,136.092318365703));
#68586=CARTESIAN_POINT('Ctrl Pts',(98.939500154013,853.352265600853,136.092377004571));
#68587=CARTESIAN_POINT('Ctrl Pts',(98.9398946554667,853.352244650014,136.092435543675));
#68588=CARTESIAN_POINT('Ctrl Pts',(98.9402891708356,853.352223473264,136.092493982953));
#68589=CARTESIAN_POINT('Ctrl Pts',(99.0592907010779,853.345835722816,136.110121594051));
#68590=CARTESIAN_POINT('Ctrl Pts',(99.1775484051736,853.319000264939,136.118369990443));
#68591=CARTESIAN_POINT('Ctrl Pts',(99.4018080526621,853.226000734966,136.114457120838));
#68592=CARTESIAN_POINT('Ctrl Pts',(99.5054334943449,853.160104158027,136.101993730068));
#68593=CARTESIAN_POINT('Ctrl Pts',(99.6819813946448,852.997273581419,136.056858318171));
#68594=CARTESIAN_POINT('Ctrl Pts',(99.7531172255607,852.902132804875,136.02470647874));
#68595=CARTESIAN_POINT('Ctrl Pts',(99.8541472207777,852.69315828628,135.944059927185));
#68596=CARTESIAN_POINT('Ctrl Pts',(99.8823574847066,852.581384720111,135.896238123706));
#68597=CARTESIAN_POINT('Ctrl Pts',(99.8909729788273,852.354888486021,135.790848550981));
#68598=CARTESIAN_POINT('Ctrl Pts',(99.8703042833721,852.242538680081,135.734223356735));
#68599=CARTESIAN_POINT('Ctrl Pts',(99.781359429257,852.032597516905,135.620203352314));
#68600=CARTESIAN_POINT('Ctrl Pts',(99.7130620675111,851.937340913477,135.563924601654));
#68601=CARTESIAN_POINT('Ctrl Pts',(99.537922545271,851.778765319224,135.460734879293));
#68602=CARTESIAN_POINT('Ctrl Pts',(99.4325126092684,851.716986994574,135.41479260724));
#68603=CARTESIAN_POINT('Ctrl Pts',(99.2005875282792,851.636760197283,135.340551393988));
#68604=CARTESIAN_POINT('Ctrl Pts',(99.0764838659736,851.618408610255,135.312666437792));
#68605=CARTESIAN_POINT('Ctrl Pts',(98.9467180969863,851.623063404591,135.294805444485));
#68606=CARTESIAN_POINT('Ctrl Pts',(98.9429115045806,851.623220792814,135.29429136319));
#68607=CARTESIAN_POINT('Ctrl Pts',(98.9391056666407,851.623398972202,135.2937872253));
#68608=CARTESIAN_POINT('Origin',(98.9391056666407,856.284316734599,124.951370193141));
#68609=CARTESIAN_POINT('',(98.9391056666407,854.620900103093,131.158265436629));
#68610=CARTESIAN_POINT('Origin',(98.9391056666407,854.149477872485,130.991648869362));
#68611=CARTESIAN_POINT('',(98.9391056666407,852.944699443349,135.90088057344));
#68612=CARTESIAN_POINT('',(98.9391056666407,856.755738965208,125.117986760408));
#68613=CARTESIAN_POINT('Ctrl Pts',(98.9395892642655,852.032885557983,135.479850729421));
#68614=CARTESIAN_POINT('Ctrl Pts',(98.8757180666484,852.035906692228,135.471117397303));
#68615=CARTESIAN_POINT('Ctrl Pts',(98.8122528025992,852.050048618326,135.467646859426));
#68616=CARTESIAN_POINT('Ctrl Pts',(98.692710416234,852.099580734955,135.471656287059));
#68617=CARTESIAN_POINT('Ctrl Pts',(98.6378647845073,852.13462307584,135.479166262806));
#68618=CARTESIAN_POINT('Ctrl Pts',(98.5448527029889,852.22127493928,135.504311011571));
#68619=CARTESIAN_POINT('Ctrl Pts',(98.5075784482175,852.271924965287,135.52164427711));
#68620=CARTESIAN_POINT('Ctrl Pts',(98.4550628489838,852.383312648024,135.56428857169));
#68621=CARTESIAN_POINT('Ctrl Pts',(98.4407340325358,852.443003475229,135.589264253722));
#68622=CARTESIAN_POINT('Ctrl Pts',(98.4377140072837,852.563652762671,135.643839450189));
#68623=CARTESIAN_POINT('Ctrl Pts',(98.4494848486265,852.623334697028,135.672933059764));
#68624=CARTESIAN_POINT('Ctrl Pts',(98.4980167772103,852.733901385318,135.731225969468));
#68625=CARTESIAN_POINT('Ctrl Pts',(98.5344774809786,852.783621350956,135.759849574892));
#68626=CARTESIAN_POINT('Ctrl Pts',(98.6274652847569,852.866234190975,135.8128740098));
#68627=CARTESIAN_POINT('Ctrl Pts',(98.6833111696002,852.898206244098,135.836745283202));
#68628=CARTESIAN_POINT('Ctrl Pts',(98.8056000180448,852.939039906398,135.875839621481));
#68629=CARTESIAN_POINT('Ctrl Pts',(98.8707933341061,852.947915416463,135.890856481481));
#68630=CARTESIAN_POINT('Ctrl Pts',(99.0016893108325,852.941762373625,135.910068249006));
#68631=CARTESIAN_POINT('Ctrl Pts',(99.0661955044237,852.927197696364,135.914270497187));
#68632=CARTESIAN_POINT('Ctrl Pts',(99.1862581541636,852.876723379701,135.911269008687));
#68633=CARTESIAN_POINT('Ctrl Pts',(99.2407711869484,852.841621887879,135.904259442341));
#68634=CARTESIAN_POINT('Ctrl Pts',(99.3333670282979,852.755072076452,135.879760025277));
#68635=CARTESIAN_POINT('Ctrl Pts',(99.37052279837,852.70457430827,135.86255320979));
#68636=CARTESIAN_POINT('Ctrl Pts',(99.4228570957353,852.593910665641,135.819807893051));
#68637=CARTESIAN_POINT('Ctrl Pts',(99.4372091362825,852.534838887248,135.794639379505));
#68638=CARTESIAN_POINT('Ctrl Pts',(99.4406829537521,852.41538414882,135.739416914261));
#68639=CARTESIAN_POINT('Ctrl Pts',(99.4292979567966,852.356248765524,135.709863105819));
#68640=CARTESIAN_POINT('Ctrl Pts',(99.3813658656915,852.245457750329,135.650155376543));
#68641=CARTESIAN_POINT('Ctrl Pts',(99.3446292315317,852.195136836004,135.620599435966));
#68642=CARTESIAN_POINT('Ctrl Pts',(99.2510883127142,852.112074251995,135.566591556355));
#68643=CARTESIAN_POINT('Ctrl Pts',(99.1951966748328,852.08002644877,135.542613499666));
#68644=CARTESIAN_POINT('Ctrl Pts',(99.0722054420159,852.038765923274,135.503668129575));
#68645=CARTESIAN_POINT('Ctrl Pts',(99.006312753062,852.029729509178,135.488974065284));
#68646=CARTESIAN_POINT('Ctrl Pts',(98.9395892642655,852.032885557983,135.479850729421));
#68647=CARTESIAN_POINT('Origin',(101.539068444395,840.466856951798,119.360944708767));
#68648=CARTESIAN_POINT('',(101.539068444395,835.888254215111,129.250423299054));
#68649=CARTESIAN_POINT('',(101.539068444395,837.802648617342,129.964159054369));
#68650=CARTESIAN_POINT('Ctrl Pts',(101.539068444395,835.888254215111,129.250423299054));
#68651=CARTESIAN_POINT('Ctrl Pts',(101.408193185807,835.891021178919,129.242594496241));
#68652=CARTESIAN_POINT('Ctrl Pts',(101.278433501112,835.917135843883,129.24419041653));
#68653=CARTESIAN_POINT('Ctrl Pts',(101.032404335379,836.014751255025,129.265891721646));
#68654=CARTESIAN_POINT('Ctrl Pts',(100.918992966955,836.086366368608,129.286212271391));
#68655=CARTESIAN_POINT('Ctrl Pts',(100.727010609144,836.266525518918,129.34258003759));
#68656=CARTESIAN_POINT('Ctrl Pts',(100.650479499543,836.37342753972,129.378110054304));
#68657=CARTESIAN_POINT('Ctrl Pts',(100.545469077725,836.608653519278,129.459226820863));
#68658=CARTESIAN_POINT('Ctrl Pts',(100.518149703322,836.734694021807,129.504025258485));
#68659=CARTESIAN_POINT('Ctrl Pts',(100.517185290251,836.988225471177,129.596699776211));
#68660=CARTESIAN_POINT('Ctrl Pts',(100.54336816205,837.113203518004,129.643659444668));
#68661=CARTESIAN_POINT('Ctrl Pts',(100.645838321594,837.345045509499,129.7340401625));
#68662=CARTESIAN_POINT('Ctrl Pts',(100.720971957318,837.449669182678,129.776598389277));
#68663=CARTESIAN_POINT('Ctrl Pts',(100.911075016139,837.625010276468,129.852712581925));
#68664=CARTESIAN_POINT('Ctrl Pts',(101.024400151761,837.693760928369,129.885468116527));
#68665=CARTESIAN_POINT('Ctrl Pts',(101.272801682029,837.784511923031,129.93662585663));
#68666=CARTESIAN_POINT('Ctrl Pts',(101.405308264756,837.806008945146,129.95465139703));
#68667=CARTESIAN_POINT('Ctrl Pts',(101.539068444395,837.802648617342,129.964159054369));
#68668=CARTESIAN_POINT('',(101.539068443729,838.442786669558,128.152962764451));
#68669=CARTESIAN_POINT('',(101.539068444395,841.429886092041,119.701311791834));
#68670=CARTESIAN_POINT('Ctrl Pts',(102.531557458013,837.686870450189,127.950803063132));
#68671=CARTESIAN_POINT('Ctrl Pts',(102.563024298442,837.564857311682,127.907679491566));
#68672=CARTESIAN_POINT('Ctrl Pts',(102.568871736002,837.438973807152,127.860871091535));
#68673=CARTESIAN_POINT('Ctrl Pts',(102.528739960197,837.193599419736,127.765295855082));
#68674=CARTESIAN_POINT('Ctrl Pts',(102.483150660768,837.076500672345,127.717466616018));
#68675=CARTESIAN_POINT('Ctrl Pts',(102.345903918612,836.866034463218,127.627228258059));
#68676=CARTESIAN_POINT('Ctrl Pts',(102.255363212755,836.774791706316,127.585718147521));
#68677=CARTESIAN_POINT('Ctrl Pts',(102.040637720221,836.630579050891,127.514983797339));
#68678=CARTESIAN_POINT('Ctrl Pts',(101.918352461316,836.579148755526,127.486493661749));
#68679=CARTESIAN_POINT('Ctrl Pts',(101.65824481109,836.523738707047,127.446814051124));
#68680=CARTESIAN_POINT('Ctrl Pts',(101.52289337425,836.520339531799,127.436023496924));
#68681=CARTESIAN_POINT('Ctrl Pts',(101.258489565672,836.562506858983,127.433717520182));
#68682=CARTESIAN_POINT('Ctrl Pts',(101.13190738766,836.607211983303,127.442037577493));
#68683=CARTESIAN_POINT('Ctrl Pts',(100.901561561467,836.740105969176,127.47660240677));
#68684=CARTESIAN_POINT('Ctrl Pts',(100.80038793904,836.827531166656,127.502723689185));
#68685=CARTESIAN_POINT('Ctrl Pts',(100.639137314404,837.033751137391,127.56911790816));
#68686=CARTESIAN_POINT('Ctrl Pts',(100.5807344529,837.150541704662,127.608744172187));
#68687=CARTESIAN_POINT('Ctrl Pts',(100.515644400704,837.396598446102,127.695612778794));
#68688=CARTESIAN_POINT('Ctrl Pts',(100.509087072713,837.523322218678,127.741925991822));
#68689=CARTESIAN_POINT('Ctrl Pts',(100.548321501849,837.770803650285,127.835575337108));
#68690=CARTESIAN_POINT('Ctrl Pts',(100.593690141832,837.88914769441,127.88200302558));
#68691=CARTESIAN_POINT('Ctrl Pts',(100.730469390048,838.1012429664,127.969040730821));
#68692=CARTESIAN_POINT('Ctrl Pts',(100.82040375461,838.19302634567,128.008838714542));
#68693=CARTESIAN_POINT('Ctrl Pts',(101.034265302307,838.33865752761,128.077312795068));
#68694=CARTESIAN_POINT('Ctrl Pts',(101.156398836596,838.390766443303,128.105234774994));
#68695=CARTESIAN_POINT('Ctrl Pts',(101.417707683903,838.447373310773,128.145373209846));
#68696=CARTESIAN_POINT('Ctrl Pts',(101.554512830897,838.450746041076,128.157006799272));
#68697=CARTESIAN_POINT('Ctrl Pts',(101.821418518916,838.4071919293,128.161624948071));
#68698=CARTESIAN_POINT('Ctrl Pts',(101.949030200169,838.361229671913,128.154760676441));
#68699=CARTESIAN_POINT('Ctrl Pts',(102.179227922305,838.226060145171,128.12313156339));
#68700=CARTESIAN_POINT('Ctrl Pts',(102.279617622767,838.13821678036,128.098686802327));
#68701=CARTESIAN_POINT('Ctrl Pts',(102.399860283198,837.983144987605,128.050744276872));
#68702=CARTESIAN_POINT('Ctrl Pts',(102.434657897715,837.927698355838,128.032914032947));
#68703=CARTESIAN_POINT('Ctrl Pts',(102.492563709514,837.810798236508,127.993993498926));
#68704=CARTESIAN_POINT('Ctrl Pts',(102.51538309237,837.749586791852,127.972969140337));
#68705=CARTESIAN_POINT('Ctrl Pts',(102.531557458013,837.686870450189,127.950803063132));
#68706=CARTESIAN_POINT('Ctrl Pts',(101.539068444395,837.802648617343,129.964159054369));
#68707=CARTESIAN_POINT('Ctrl Pts',(101.539102971817,837.802647749944,129.964161508574));
#68708=CARTESIAN_POINT('Ctrl Pts',(101.539137499323,837.802646880888,129.96416396221));
#68709=CARTESIAN_POINT('Ctrl Pts',(101.539172026912,837.802646010177,129.964166415277));
#68710=CARTESIAN_POINT('Ctrl Pts',(101.669676912657,837.799354961388,129.973438339675));
#68711=CARTESIAN_POINT('Ctrl Pts',(101.799001755468,837.772464643173,129.974424179339));
#68712=CARTESIAN_POINT('Ctrl Pts',(102.043583294327,837.67359624361,129.959030090533));
#68713=CARTESIAN_POINT('Ctrl Pts',(102.156230418727,837.601692148446,129.942446541966));
#68714=CARTESIAN_POINT('Ctrl Pts',(102.346855325263,837.422331778836,129.892852604008));
#68715=CARTESIAN_POINT('Ctrl Pts',(102.423091998765,837.316702513936,129.860351826956));
#68716=CARTESIAN_POINT('Ctrl Pts',(102.529109749153,837.084964808974,129.782959530906));
#68717=CARTESIAN_POINT('Ctrl Pts',(102.557728197776,836.96111900325,129.73880586743));
#68718=CARTESIAN_POINT('Ctrl Pts',(102.562863469046,836.710965174577,129.644414079336));
#68719=CARTESIAN_POINT('Ctrl Pts',(102.539021640317,836.58715827539,129.595095832061));
#68720=CARTESIAN_POINT('Ctrl Pts',(102.441167288692,836.356187406874,129.498391015763));
#68721=CARTESIAN_POINT('Ctrl Pts',(102.367882229711,836.251366198201,129.451977434468));
#68722=CARTESIAN_POINT('Ctrl Pts',(102.181334733362,836.075241602747,129.369240539844));
#68723=CARTESIAN_POINT('Ctrl Pts',(102.069827431732,836.005635100728,129.333727665471));
#68724=CARTESIAN_POINT('Ctrl Pts',(101.821459192417,835.910508245188,129.278628271386));
#68725=CARTESIAN_POINT('Ctrl Pts',(101.686695903781,835.886572425089,129.25982944876));
#68726=CARTESIAN_POINT('Ctrl Pts',(101.546490993202,835.888116081824,129.250874816581));
#68727=CARTESIAN_POINT('Ctrl Pts',(101.542779269904,835.888175760864,129.250645276237));
#68728=CARTESIAN_POINT('Ctrl Pts',(101.539068444395,835.888254215111,129.250423299054));
#68729=CARTESIAN_POINT('Origin',(101.539068444395,840.466856951798,119.360944708767));
#68730=CARTESIAN_POINT('',(101.539068444395,838.803440320292,125.567839952255));
#68731=CARTESIAN_POINT('Origin',(101.539068444395,838.332018089683,125.401223384988));
#68732=CARTESIAN_POINT('',(101.539068444395,837.314405062769,129.780892315957));
#68733=CARTESIAN_POINT('',(101.539068444395,840.938279182407,119.527561276034));
#68734=CARTESIAN_POINT('Ctrl Pts',(101.539325607471,836.377250220821,129.431561262802));
#68735=CARTESIAN_POINT('Ctrl Pts',(101.478599217227,836.378563737303,129.427751092737));
#68736=CARTESIAN_POINT('Ctrl Pts',(101.418348588659,836.390191952138,129.42795637229));
#68737=CARTESIAN_POINT('Ctrl Pts',(101.299561870893,836.434963708252,129.436671899503));
#68738=CARTESIAN_POINT('Ctrl Pts',(101.242859179905,836.469521653125,129.445845031852));
#68739=CARTESIAN_POINT('Ctrl Pts',(101.146561424509,836.557193391539,129.472232645901));
#68740=CARTESIAN_POINT('Ctrl Pts',(101.107965019525,836.609458055559,129.489191250003));
#68741=CARTESIAN_POINT('Ctrl Pts',(101.05448093305,836.72477574853,129.528532546431));
#68742=CARTESIAN_POINT('Ctrl Pts',(101.040163727406,836.786676466367,129.550522517419));
#68743=CARTESIAN_POINT('Ctrl Pts',(101.038095594994,836.911506260466,129.596503839619));
#68744=CARTESIAN_POINT('Ctrl Pts',(101.050324199247,836.973174531978,129.620030557596));
#68745=CARTESIAN_POINT('Ctrl Pts',(101.09979898472,837.087766866978,129.665544897754));
#68746=CARTESIAN_POINT('Ctrl Pts',(101.136514375652,837.139553119855,129.687082712585));
#68747=CARTESIAN_POINT('Ctrl Pts',(101.229740746087,837.226246637234,129.725488753147));
#68748=CARTESIAN_POINT('Ctrl Pts',(101.285380892132,837.260235735861,129.741963049638));
#68749=CARTESIAN_POINT('Ctrl Pts',(101.407240373126,837.305106476048,129.767432035295));
#68750=CARTESIAN_POINT('Ctrl Pts',(101.472149039858,837.315847036994,129.776276272621));
#68751=CARTESIAN_POINT('Ctrl Pts',(101.603175272831,837.313027043415,129.785315557002));
#68752=CARTESIAN_POINT('Ctrl Pts',(101.668051054937,837.299536686526,129.785438357248));
#68753=CARTESIAN_POINT('Ctrl Pts',(101.789039205539,837.250024635162,129.776751672538));
#68754=CARTESIAN_POINT('Ctrl Pts',(101.844033504356,837.214553736411,129.768052581997));
#68755=CARTESIAN_POINT('Ctrl Pts',(101.936865232963,837.126207584309,129.742747967812));
#68756=CARTESIAN_POINT('Ctrl Pts',(101.973843483836,837.074228458178,129.726402325773));
#68757=CARTESIAN_POINT('Ctrl Pts',(102.024840563852,836.96036444174,129.687995625057));
#68758=CARTESIAN_POINT('Ctrl Pts',(102.038330626816,836.899594262713,129.666306731107));
#68759=CARTESIAN_POINT('Ctrl Pts',(102.039750071531,836.777078728272,129.620357918605));
#68760=CARTESIAN_POINT('Ctrl Pts',(102.027569425668,836.716546909429,129.596546638139));
#68761=CARTESIAN_POINT('Ctrl Pts',(101.978789182878,836.603790937744,129.550088078679));
#68762=CARTESIAN_POINT('Ctrl Pts',(101.942578690059,836.552700977587,129.527903887479));
#68763=CARTESIAN_POINT('Ctrl Pts',(101.850290191676,836.466559787651,129.488184276716));
#68764=CARTESIAN_POINT('Ctrl Pts',(101.794893766359,836.432541051752,129.471097603998));
#68765=CARTESIAN_POINT('Ctrl Pts',(101.672245845522,836.386870444056,129.444727205074));
#68766=CARTESIAN_POINT('Ctrl Pts',(101.606132947174,836.375805172937,129.435752971297));
#68767=CARTESIAN_POINT('Ctrl Pts',(101.539325607471,836.377250220821,129.431561262802));
#68768=CARTESIAN_POINT('Origin',(103.880632053932,846.665521119814,121.551762362789));
#68769=CARTESIAN_POINT('',(103.880632053932,841.996470226746,131.917191143814));
#68770=CARTESIAN_POINT('',(103.880632054005,843.746368801472,132.656273473763));
#68771=CARTESIAN_POINT('Ctrl Pts',(103.880632053932,841.996470226746,131.917191143814));
#68772=CARTESIAN_POINT('Ctrl Pts',(103.761418994746,842.002764179425,131.899383135524));
#68773=CARTESIAN_POINT('Ctrl Pts',(103.642927426757,842.029653537582,131.890776429531));
#68774=CARTESIAN_POINT('Ctrl Pts',(103.415568339074,842.124451135479,131.892834505147));
#68775=CARTESIAN_POINT('Ctrl Pts',(103.309582766932,842.192992750961,131.904249163847));
#68776=CARTESIAN_POINT('Ctrl Pts',(103.131806387883,842.3615930436,131.945830480073));
#68777=CARTESIAN_POINT('Ctrl Pts',(103.061164311068,842.459284930544,131.975182682802));
#68778=CARTESIAN_POINT('Ctrl Pts',(102.961685480668,842.674661775683,132.048736802417));
#68779=CARTESIAN_POINT('Ctrl Pts',(102.934780773326,842.790397205374,132.092432269426));
#68780=CARTESIAN_POINT('Ctrl Pts',(102.930580638678,843.022320992322,132.187972370811));
#68781=CARTESIAN_POINT('Ctrl Pts',(102.953328321717,843.136043768445,132.238811317241));
#68782=CARTESIAN_POINT('Ctrl Pts',(103.04554288982,843.346392623877,132.341453813949));
#68783=CARTESIAN_POINT('Ctrl Pts',(103.114292890983,843.44077504051,132.392223053204));
#68784=CARTESIAN_POINT('Ctrl Pts',(103.289422454791,843.597819372278,132.487730165283));
#68785=CARTESIAN_POINT('Ctrl Pts',(103.394577644932,843.658540376311,132.531468337365));
#68786=CARTESIAN_POINT('Ctrl Pts',(103.627529007129,843.737014458413,132.605909436609));
#68787=CARTESIAN_POINT('Ctrl Pts',(103.753419529693,843.753606470952,132.635795328422));
#68788=CARTESIAN_POINT('Ctrl Pts',(103.880632054078,843.746368801472,132.656273473763));
#68789=CARTESIAN_POINT('',(103.880632053932,844.42519506336,130.735613386816));
#68790=CARTESIAN_POINT('',(103.880632053932,847.559417292433,121.867695515926));
#68791=CARTESIAN_POINT('Ctrl Pts',(104.772417774909,843.805892092828,130.608567344288));
#68792=CARTESIAN_POINT('Ctrl Pts',(104.8126108154,843.700887439897,130.571455147021));
#68793=CARTESIAN_POINT('Ctrl Pts',(104.831561154686,843.590835653455,130.52921134503));
#68794=CARTESIAN_POINT('Ctrl Pts',(104.82500391408,843.365886614736,130.436428798797));
#68795=CARTESIAN_POINT('Ctrl Pts',(104.797027594465,843.253384664035,130.386521440141));
#68796=CARTESIAN_POINT('Ctrl Pts',(104.69637163862,843.048868933494,130.289032846508));
#68797=CARTESIAN_POINT('Ctrl Pts',(104.625414031777,842.958450539467,130.242346388363));
#68798=CARTESIAN_POINT('Ctrl Pts',(104.448085205806,842.807957456829,130.156922960298));
#68799=CARTESIAN_POINT('Ctrl Pts',(104.342785256947,842.749764919734,130.119110654766));
#68800=CARTESIAN_POINT('Ctrl Pts',(104.110895361281,842.674669280196,130.057977044444));
#68801=CARTESIAN_POINT('Ctrl Pts',(103.986204229695,842.658978478078,130.035406798003));
#68802=CARTESIAN_POINT('Ctrl Pts',(103.734885246423,842.673846056906,130.009206304506));
#68803=CARTESIAN_POINT('Ctrl Pts',(103.610673037664,842.704373161885,130.005869184416));
#68804=CARTESIAN_POINT('Ctrl Pts',(103.384914277831,842.806313174553,130.018745328133));
#68805=CARTESIAN_POINT('Ctrl Pts',(103.284728730839,842.875009045625,130.034016098454));
#68806=CARTESIAN_POINT('Ctrl Pts',(103.118706652789,843.040194350758,130.079931946323));
#68807=CARTESIAN_POINT('Ctrl Pts',(103.053334985224,843.134210726847,130.109636664957));
#68808=CARTESIAN_POINT('Ctrl Pts',(102.961594737649,843.338985902304,130.180405708178));
#68809=CARTESIAN_POINT('Ctrl Pts',(102.936287460259,843.447954787142,130.220881702022));
#68810=CARTESIAN_POINT('Ctrl Pts',(102.929487334851,843.670132778008,130.308858380912));
#68811=CARTESIAN_POINT('Ctrl Pts',(102.949233155853,843.781241674513,130.355674344468));
#68812=CARTESIAN_POINT('Ctrl Pts',(103.034869636845,843.994038758867,130.451450312228));
#68813=CARTESIAN_POINT('Ctrl Pts',(103.10224165078,844.092720052682,130.499409407044));
#68814=CARTESIAN_POINT('Ctrl Pts',(103.273577995327,844.255756903701,130.586695254));
#68815=CARTESIAN_POINT('Ctrl Pts',(103.375063060711,844.31929796989,130.625374055142));
#68816=CARTESIAN_POINT('Ctrl Pts',(103.601559694902,844.405879202998,130.690095097829));
#68817=CARTESIAN_POINT('Ctrl Pts',(103.724772717604,844.42754167909,130.715354415762));
#68818=CARTESIAN_POINT('Ctrl Pts',(103.976432807209,844.424495509366,130.748358223679));
#68819=CARTESIAN_POINT('Ctrl Pts',(104.102540614433,844.399394443665,130.755625723465));
#68820=CARTESIAN_POINT('Ctrl Pts',(104.326906610974,844.309693794209,130.750545283255));
#68821=CARTESIAN_POINT('Ctrl Pts',(104.424912755827,844.250187158244,130.74019340023));
#68822=CARTESIAN_POINT('Ctrl Pts',(104.599606819597,844.098708198734,130.703308980291));
#68823=CARTESIAN_POINT('Ctrl Pts',(104.673337810374,844.006670349102,130.676328103615));
#68824=CARTESIAN_POINT('Ctrl Pts',(104.744428595113,843.872754633768,130.631853510398));
#68825=CARTESIAN_POINT('Ctrl Pts',(104.759495119332,843.839652638115,130.620499463309));
#68826=CARTESIAN_POINT('Ctrl Pts',(104.772417774909,843.805892092828,130.608567344288));
#68827=CARTESIAN_POINT('Ctrl Pts',(103.880632054078,843.746368801472,132.656273473763));
#68828=CARTESIAN_POINT('Ctrl Pts',(103.881160973326,843.746338708974,132.656358616993));
#68829=CARTESIAN_POINT('Ctrl Pts',(103.881689915481,843.746308204289,132.65644359717));
#68830=CARTESIAN_POINT('Ctrl Pts',(103.882218879997,843.746277287993,132.656528414428));
#68831=CARTESIAN_POINT('Ctrl Pts',(104.000111953979,843.739386812049,132.675432077867));
#68832=CARTESIAN_POINT('Ctrl Pts',(104.117202505183,843.712143462111,132.685935518663));
#68833=CARTESIAN_POINT('Ctrl Pts',(104.341086575488,843.617919766937,132.688493236018));
#68834=CARTESIAN_POINT('Ctrl Pts',(104.445405730643,843.550569397786,132.679921995478));
#68835=CARTESIAN_POINT('Ctrl Pts',(104.622400594513,843.384739558509,132.643405301328));
#68836=CARTESIAN_POINT('Ctrl Pts',(104.693630663002,843.288270086762,132.616029026027));
#68837=CARTESIAN_POINT('Ctrl Pts',(104.794656317807,843.077120754238,132.545243715783));
#68838=CARTESIAN_POINT('Ctrl Pts',(104.823133455667,842.964636400798,132.502515759332));
#68839=CARTESIAN_POINT('Ctrl Pts',(104.832904630706,842.736744645383,132.406576776194));
#68840=CARTESIAN_POINT('Ctrl Pts',(104.813221128518,842.623802822434,132.354239694833));
#68841=CARTESIAN_POINT('Ctrl Pts',(104.72683280558,842.412571907182,132.247131410046));
#68842=CARTESIAN_POINT('Ctrl Pts',(104.660136378731,842.316726408412,132.193427031619));
#68843=CARTESIAN_POINT('Ctrl Pts',(104.487180076312,842.155399720145,132.092336428288));
#68844=CARTESIAN_POINT('Ctrl Pts',(104.381734313182,842.092122389083,132.046070064516));
#68845=CARTESIAN_POINT('Ctrl Pts',(104.149121756987,842.009881560872,131.96947168897));
#68846=CARTESIAN_POINT('Ctrl Pts',(104.024314095971,841.991104888684,131.939632183285));
#68847=CARTESIAN_POINT('Ctrl Pts',(103.891939809102,841.995919629985,131.918900720637));
#68848=CARTESIAN_POINT('Ctrl Pts',(103.886285118654,841.996171768489,131.918035596797));
#68849=CARTESIAN_POINT('Ctrl Pts',(103.880632053932,841.996470226746,131.917191143814));
#68850=CARTESIAN_POINT('Origin',(103.880632053932,846.665521119814,121.551762362789));
#68851=CARTESIAN_POINT('',(103.880632053932,845.002104488308,127.758657606278));
#68852=CARTESIAN_POINT('Origin',(103.880632053932,844.530682257699,127.592041039011));
#68853=CARTESIAN_POINT('',(103.880632053932,843.333459423775,132.479895063748));
#68854=CARTESIAN_POINT('',(103.880632053932,847.136943350423,121.718378930056));
#68855=CARTESIAN_POINT('Ctrl Pts',(103.881088470536,842.410563859926,132.090219465587));
#68856=CARTESIAN_POINT('Ctrl Pts',(103.817092215407,842.413949745358,132.080464189414));
#68857=CARTESIAN_POINT('Ctrl Pts',(103.75351903137,842.428618923509,132.075655595089));
#68858=CARTESIAN_POINT('Ctrl Pts',(103.633730778617,842.479484772073,132.076489885268));
#68859=CARTESIAN_POINT('Ctrl Pts',(103.578725442098,842.515371453365,132.0822077029));
#68860=CARTESIAN_POINT('Ctrl Pts',(103.485742631032,842.603755906287,132.103520938011));
#68861=CARTESIAN_POINT('Ctrl Pts',(103.448557329042,842.655212023092,132.118810526531));
#68862=CARTESIAN_POINT('Ctrl Pts',(103.396625286578,842.767504521097,132.157065325446));
#68863=CARTESIAN_POINT('Ctrl Pts',(103.382440944718,842.827178549087,132.179638197222));
#68864=CARTESIAN_POINT('Ctrl Pts',(103.379101074122,842.948537065295,132.229852956544));
#68865=CARTESIAN_POINT('Ctrl Pts',(103.390690579609,843.00891419442,132.257076050657));
#68866=CARTESIAN_POINT('Ctrl Pts',(103.438881153461,843.120693738879,132.312143980886));
#68867=CARTESIAN_POINT('Ctrl Pts',(103.475122932878,843.170891088879,132.339427178499));
#68868=CARTESIAN_POINT('Ctrl Pts',(103.567612870714,843.254286502661,132.390561028732));
#68869=CARTESIAN_POINT('Ctrl Pts',(103.623151706139,843.28652571091,132.413890342806));
#68870=CARTESIAN_POINT('Ctrl Pts',(103.746193962561,843.32824636792,132.45337119734));
#68871=CARTESIAN_POINT('Ctrl Pts',(103.812668259895,843.33716584272,132.469105204232));
#68872=CARTESIAN_POINT('Ctrl Pts',(103.945240784138,843.32993698082,132.49015269318));
#68873=CARTESIAN_POINT('Ctrl Pts',(104.010142440204,843.314538856143,132.495556583241));
#68874=CARTESIAN_POINT('Ctrl Pts',(104.130534587574,843.2620111768,132.49553865509));
#68875=CARTESIAN_POINT('Ctrl Pts',(104.18505622567,843.225750167681,132.490300568786));
#68876=CARTESIAN_POINT('Ctrl Pts',(104.277094571263,843.136966665675,132.469753950187));
#68877=CARTESIAN_POINT('Ctrl Pts',(104.313843549289,843.085501608901,132.454748833412));
#68878=CARTESIAN_POINT('Ctrl Pts',(104.365170041522,842.973292777513,132.416594690365));
#68879=CARTESIAN_POINT('Ctrl Pts',(104.379095303301,842.913711995107,132.39381795739));
#68880=CARTESIAN_POINT('Ctrl Pts',(104.381951538699,842.79348344918,132.343127519791));
#68881=CARTESIAN_POINT('Ctrl Pts',(104.370444031482,842.734126561631,132.315683716556));
#68882=CARTESIAN_POINT('Ctrl Pts',(104.322715092642,842.623323395167,132.259674785956));
#68883=CARTESIAN_POINT('Ctrl Pts',(104.286455149685,842.573201116069,132.231671660714));
#68884=CARTESIAN_POINT('Ctrl Pts',(104.193572972612,842.489679052634,132.179265997727));
#68885=CARTESIAN_POINT('Ctrl Pts',(104.13753505549,842.457322967167,132.155419485912));
#68886=CARTESIAN_POINT('Ctrl Pts',(104.014163787141,842.415884110923,132.115845159717));
#68887=CARTESIAN_POINT('Ctrl Pts',(103.948010756191,842.407023165371,132.100420771544));
#68888=CARTESIAN_POINT('Ctrl Pts',(103.881088470536,842.410563859926,132.090219465587));
#68889=CARTESIAN_POINT('Origin',(102.935786484342,830.684044276295,115.903367699502));
#68890=CARTESIAN_POINT('',(102.935786484342,826.101475377183,125.804068085843));
#68891=CARTESIAN_POINT('',(102.935786484349,828.025971426816,126.489222402778));
#68892=CARTESIAN_POINT('Ctrl Pts',(102.935786484342,826.101475377183,125.804068085843));
#68893=CARTESIAN_POINT('Ctrl Pts',(102.806520930159,826.10448001969,125.795566798752));
#68894=CARTESIAN_POINT('Ctrl Pts',(102.678312485991,826.130360223824,125.79598194708));
#68895=CARTESIAN_POINT('Ctrl Pts',(102.433403951682,826.227124308982,125.814770529169));
#68896=CARTESIAN_POINT('Ctrl Pts',(102.319726709598,826.298624618765,125.833589843808));
#68897=CARTESIAN_POINT('Ctrl Pts',(102.127025707492,826.478590648783,125.887021052632));
#68898=CARTESIAN_POINT('Ctrl Pts',(102.050015789127,826.585389329037,125.921132104669));
#68899=CARTESIAN_POINT('Ctrl Pts',(101.943582951435,826.821037134934,125.999668746766));
#68900=CARTESIAN_POINT('Ctrl Pts',(101.915516701988,826.947665274344,126.043356460436));
#68901=CARTESIAN_POINT('Ctrl Pts',(101.913308128373,827.203050219501,126.133923369079));
#68902=CARTESIAN_POINT('Ctrl Pts',(101.939159834502,827.329260407403,126.179899382231));
#68903=CARTESIAN_POINT('Ctrl Pts',(102.041408202899,827.563187765812,126.267968264977));
#68904=CARTESIAN_POINT('Ctrl Pts',(102.116476686542,827.66870249053,126.309229803067));
#68905=CARTESIAN_POINT('Ctrl Pts',(102.305938517745,827.845039138649,126.382417259864));
#68906=CARTESIAN_POINT('Ctrl Pts',(102.418390800487,827.914181419715,126.413657184712));
#68907=CARTESIAN_POINT('Ctrl Pts',(102.666926931412,828.006894840134,126.462803160003));
#68908=CARTESIAN_POINT('Ctrl Pts',(102.800720750187,828.029186105331,126.480126843192));
#68909=CARTESIAN_POINT('Ctrl Pts',(102.935786484357,828.025971426816,126.489222402778));
#68910=CARTESIAN_POINT('',(102.935786484219,828.665071698505,124.680962392358));
#68911=CARTESIAN_POINT('',(102.935786484342,831.647073416538,116.243734782569));
#68912=CARTESIAN_POINT('Ctrl Pts',(103.956762674324,827.704529521989,124.422706018157));
#68913=CARTESIAN_POINT('Ctrl Pts',(103.960636116979,827.579014269356,124.378344680962));
#68914=CARTESIAN_POINT('Ctrl Pts',(103.938436004372,827.454751264983,124.332109020517));
#68915=CARTESIAN_POINT('Ctrl Pts',(103.844459113732,827.222666636853,124.241230834666));
#68916=CARTESIAN_POINT('Ctrl Pts',(103.773597615158,827.117107807912,124.197480193245));
#68917=CARTESIAN_POINT('Ctrl Pts',(103.591840702334,826.938253886779,124.118414687492));
#68918=CARTESIAN_POINT('Ctrl Pts',(103.482516410088,826.866817140815,124.083904691373));
#68919=CARTESIAN_POINT('Ctrl Pts',(103.239312718108,826.767983869091,124.029208950841));
#68920=CARTESIAN_POINT('Ctrl Pts',(103.107644003807,826.741719636915,124.009613353496));
#68921=CARTESIAN_POINT('Ctrl Pts',(102.839609262409,826.738646886536,123.988431514896));
#68922=CARTESIAN_POINT('Ctrl Pts',(102.705801641709,826.761920551898,123.987068045066));
#68923=CARTESIAN_POINT('Ctrl Pts',(102.455281918683,826.855115228523,124.00279686017));
#68924=CARTESIAN_POINT('Ctrl Pts',(102.340805777403,826.92370849611,124.019559795587));
#68925=CARTESIAN_POINT('Ctrl Pts',(102.143939311041,827.098937915499,124.069087399524));
#68926=CARTESIAN_POINT('Ctrl Pts',(102.063924157867,827.204318367303,124.101554676348));
#68927=CARTESIAN_POINT('Ctrl Pts',(101.95122220926,827.437686201415,124.177543868812));
#68928=CARTESIAN_POINT('Ctrl Pts',(101.919735285824,827.563384571856,124.220318451882));
#68929=CARTESIAN_POINT('Ctrl Pts',(101.910320236622,827.816824541311,124.309796541087));
#68930=CARTESIAN_POINT('Ctrl Pts',(101.931956379922,827.942054049341,124.355581630465));
#68931=CARTESIAN_POINT('Ctrl Pts',(102.025335141902,828.176393918699,124.444586302996));
#68932=CARTESIAN_POINT('Ctrl Pts',(102.096127812757,828.283226731668,124.486945532886));
#68933=CARTESIAN_POINT('Ctrl Pts',(102.277525039041,828.463791686724,124.562839357267));
#68934=CARTESIAN_POINT('Ctrl Pts',(102.386243595941,828.535889168149,124.5956796786));
#68935=CARTESIAN_POINT('Ctrl Pts',(102.628723695406,828.63629828649,124.648170751724));
#68936=CARTESIAN_POINT('Ctrl Pts',(102.76033766592,828.663261599384,124.667205424798));
#68937=CARTESIAN_POINT('Ctrl Pts',(103.029813754604,828.667269300677,124.688753534586));
#68938=CARTESIAN_POINT('Ctrl Pts',(103.165096542509,828.643678947569,124.690857458015));
#68939=CARTESIAN_POINT('Ctrl Pts',(103.417951818128,828.54861811161,124.677271387714));
#68940=CARTESIAN_POINT('Ctrl Pts',(103.53328939306,828.478580324885,124.661898009401));
#68941=CARTESIAN_POINT('Ctrl Pts',(103.729768316606,828.301128445595,124.615324882301));
#68942=CARTESIAN_POINT('Ctrl Pts',(103.80905086026,828.195480110099,124.584587242151));
#68943=CARTESIAN_POINT('Ctrl Pts',(103.892945851721,828.020178899464,124.529494955938));
#68944=CARTESIAN_POINT('Ctrl Pts',(103.914878607193,827.959110461282,124.509677775407));
#68945=CARTESIAN_POINT('Ctrl Pts',(103.945906762478,827.833397257411,124.467642399112));
#68946=CARTESIAN_POINT('Ctrl Pts',(103.954771674371,827.769045995908,124.44550832301));
#68947=CARTESIAN_POINT('Ctrl Pts',(103.956762674324,827.704529521989,124.422706018157));
#68948=CARTESIAN_POINT('Ctrl Pts',(102.935786484357,828.025971426816,126.489222402778));
#68949=CARTESIAN_POINT('Ctrl Pts',(102.936009125898,828.025966127759,126.489237395844));
#68950=CARTESIAN_POINT('Ctrl Pts',(102.936231770901,828.02596075942,126.489252366484));
#68951=CARTESIAN_POINT('Ctrl Pts',(102.93645441933,828.025955321793,126.489267314693));
#68952=CARTESIAN_POINT('Ctrl Pts',(103.066090593206,828.022789284825,126.497970851115));
#68953=CARTESIAN_POINT('Ctrl Pts',(103.194520386692,827.996185249279,126.4989298261));
#68954=CARTESIAN_POINT('Ctrl Pts',(103.438768938464,827.89765768665,126.484743511593));
#68955=CARTESIAN_POINT('Ctrl Pts',(103.551819217782,827.825349857432,126.469245354155));
#68956=CARTESIAN_POINT('Ctrl Pts',(103.742949719137,827.644788252355,126.422798925592));
#68957=CARTESIAN_POINT('Ctrl Pts',(103.81936605789,827.538401028909,126.392341299576));
#68958=CARTESIAN_POINT('Ctrl Pts',(103.925503874168,827.305224409805,126.319664335284));
#68959=CARTESIAN_POINT('Ctrl Pts',(103.954228823691,827.180739103681,126.278157789586));
#68960=CARTESIAN_POINT('Ctrl Pts',(103.959736028277,826.929431334742,126.18901812719));
#68961=CARTESIAN_POINT('Ctrl Pts',(103.936257027715,826.805122853584,126.142255913342));
#68962=CARTESIAN_POINT('Ctrl Pts',(103.839310186563,826.573014584314,126.049830578665));
#68963=CARTESIAN_POINT('Ctrl Pts',(103.766529342937,826.467617737881,126.005105066546));
#68964=CARTESIAN_POINT('Ctrl Pts',(103.580846949938,826.290260502289,125.924501776525));
#68965=CARTESIAN_POINT('Ctrl Pts',(103.469625196976,826.220105319395,125.889443620195));
#68966=CARTESIAN_POINT('Ctrl Pts',(103.222400347441,826.12439655287,125.834342041166));
#68967=CARTESIAN_POINT('Ctrl Pts',(103.088569987809,826.100182034503,125.814986042936));
#68968=CARTESIAN_POINT('Ctrl Pts',(102.947203763653,826.101254653806,125.80483616287));
#68969=CARTESIAN_POINT('Ctrl Pts',(102.941494092056,826.101342709816,125.804443452755));
#68970=CARTESIAN_POINT('Ctrl Pts',(102.935786484342,826.101475377183,125.804068085843));
#68971=CARTESIAN_POINT('Origin',(102.935786484342,830.684044276295,115.903367699502));
#68972=CARTESIAN_POINT('',(102.935786484342,829.020627644789,122.11026294299));
#68973=CARTESIAN_POINT('Origin',(102.935786484342,828.54920541418,121.943646375723));
#68974=CARTESIAN_POINT('',(102.935786484342,827.534953974529,126.313804085861));
#68975=CARTESIAN_POINT('',(102.935786484342,831.155466506904,116.069984266769));
#68976=CARTESIAN_POINT('Ctrl Pts',(102.936069390333,826.592865577367,125.978431996048));
#68977=CARTESIAN_POINT('Ctrl Pts',(102.874475063288,826.594269262267,125.974355848731));
#68978=CARTESIAN_POINT('Ctrl Pts',(102.813382543912,826.606334528243,125.974269675768));
#68979=CARTESIAN_POINT('Ctrl Pts',(102.694097165491,826.652275454842,125.982332226208));
#68980=CARTESIAN_POINT('Ctrl Pts',(102.637633481101,826.687254983315,125.991012593791));
#68981=CARTESIAN_POINT('Ctrl Pts',(102.541823826425,826.77573937831,126.016257939734));
#68982=CARTESIAN_POINT('Ctrl Pts',(102.503484011035,826.828406677805,126.032585966355));
#68983=CARTESIAN_POINT('Ctrl Pts',(102.451024353403,826.943445517041,126.070238122327));
#68984=CARTESIAN_POINT('Ctrl Pts',(102.437032368536,827.004523954009,126.091106467414));
#68985=CARTESIAN_POINT('Ctrl Pts',(102.43467602439,827.129071128835,126.135243922408));
#68986=CARTESIAN_POINT('Ctrl Pts',(102.446858456483,827.191297661732,126.15810438915));
#68987=CARTESIAN_POINT('Ctrl Pts',(102.496410196976,827.306804910587,126.202258301628));
#68988=CARTESIAN_POINT('Ctrl Pts',(102.53318051434,827.358955585124,126.223116337427));
#68989=CARTESIAN_POINT('Ctrl Pts',(102.626356702174,827.446043555937,126.260181537004));
#68990=CARTESIAN_POINT('Ctrl Pts',(102.681790369339,827.480148773743,126.276033643539));
#68991=CARTESIAN_POINT('Ctrl Pts',(102.804191383321,827.525687790986,126.300796577117));
#68992=CARTESIAN_POINT('Ctrl Pts',(102.869987789968,827.536584258163,126.309438485901));
#68993=CARTESIAN_POINT('Ctrl Pts',(103.00197251611,827.533314830037,126.318195636516));
#68994=CARTESIAN_POINT('Ctrl Pts',(103.066887885629,827.519502290332,126.318335541075));
#68995=CARTESIAN_POINT('Ctrl Pts',(103.187853521999,827.469163160649,126.310105508394));
#68996=CARTESIAN_POINT('Ctrl Pts',(103.242781380914,827.433173883405,126.301832843899));
#68997=CARTESIAN_POINT('Ctrl Pts',(103.335254496134,827.343738134208,126.277759976895));
#68998=CARTESIAN_POINT('Ctrl Pts',(103.371972275781,827.291208543319,126.262212102189));
#68999=CARTESIAN_POINT('Ctrl Pts',(103.422286201787,827.176391343456,126.225662856712));
#69000=CARTESIAN_POINT('Ctrl Pts',(103.435416496703,827.115238992875,126.205022925311));
#69001=CARTESIAN_POINT('Ctrl Pts',(103.436141839161,826.99216514814,126.161215576118));
#69002=CARTESIAN_POINT('Ctrl Pts',(103.423674641188,826.931463217743,126.138477589341));
#69003=CARTESIAN_POINT('Ctrl Pts',(103.374439161389,826.818496913598,126.093945388958));
#69004=CARTESIAN_POINT('Ctrl Pts',(103.338066005267,826.767379056222,126.072597250757));
#69005=CARTESIAN_POINT('Ctrl Pts',(103.245988382357,826.681699434716,126.034351642809));
#69006=CARTESIAN_POINT('Ctrl Pts',(103.191123271933,826.648011870649,126.017840711501));
#69007=CARTESIAN_POINT('Ctrl Pts',(103.06908825276,826.602406166871,125.991896511813));
#69008=CARTESIAN_POINT('Ctrl Pts',(103.002919813313,826.591342110291,125.982855977693));
#69009=CARTESIAN_POINT('Ctrl Pts',(102.936069390333,826.592865577367,125.978431996048));
#69010=CARTESIAN_POINT('Origin',(106.593082004564,836.288239824643,117.884080028985));
#69011=CARTESIAN_POINT('',(106.593082004564,831.610248993976,128.2748033254));
#69012=CARTESIAN_POINT('',(106.593082004635,833.382657080601,128.950197605091));
#69013=CARTESIAN_POINT('Ctrl Pts',(106.593082004564,831.610248993976,128.2748033254));
#69014=CARTESIAN_POINT('Ctrl Pts',(106.469739565798,831.61723941511,128.255024740483));
#69015=CARTESIAN_POINT('Ctrl Pts',(106.347303886464,831.64652201565,128.244402170008));
#69016=CARTESIAN_POINT('Ctrl Pts',(106.117480999544,831.747323237994,128.242611307471));
#69017=CARTESIAN_POINT('Ctrl Pts',(106.012399500629,831.818118670509,128.251564465386));
#69018=CARTESIAN_POINT('Ctrl Pts',(105.836647244662,831.991227608674,128.287581412267));
#69019=CARTESIAN_POINT('Ctrl Pts',(105.767133138537,832.091226896752,128.313942603965));
#69020=CARTESIAN_POINT('Ctrl Pts',(105.671659373922,832.308315912299,128.380321896406));
#69021=CARTESIAN_POINT('Ctrl Pts',(105.64644226575,832.42309642187,128.419581506658));
#69022=CARTESIAN_POINT('Ctrl Pts',(105.64363986978,832.655742776992,128.507039382574));
#69023=CARTESIAN_POINT('Ctrl Pts',(105.667249562721,832.771111027246,128.554492226706));
#69024=CARTESIAN_POINT('Ctrl Pts',(105.761343927845,832.983609420419,128.650543959949));
#69025=CARTESIAN_POINT('Ctrl Pts',(105.830797577804,833.078528931949,128.698148401477));
#69026=CARTESIAN_POINT('Ctrl Pts',(106.006514792163,833.235579097993,128.787930084183));
#69027=CARTESIAN_POINT('Ctrl Pts',(106.111252208483,833.295947377084,128.829193637811));
#69028=CARTESIAN_POINT('Ctrl Pts',(106.34260804147,833.373732025045,128.900310965665));
#69029=CARTESIAN_POINT('Ctrl Pts',(106.467281320242,833.390008779794,128.929396825915));
#69030=CARTESIAN_POINT('Ctrl Pts',(106.593082004706,833.382657080601,128.950197605091));
#69031=CARTESIAN_POINT('',(106.593082004564,834.056466383016,127.043732422434));
#69032=CARTESIAN_POINT('',(106.593082004564,837.182135997262,118.200013182122));
#69033=CARTESIAN_POINT('Ctrl Pts',(107.532294808004,833.247164435627,126.876755726751));
#69034=CARTESIAN_POINT('Ctrl Pts',(107.548454394724,833.136575409437,126.837669823023));
#69035=CARTESIAN_POINT('Ctrl Pts',(107.54249056949,833.025236699112,126.794971178588));
#69036=CARTESIAN_POINT('Ctrl Pts',(107.485551964177,832.806579904812,126.704412524435));
#69037=CARTESIAN_POINT('Ctrl Pts',(107.432675683693,832.702090199864,126.657336964529));
#69038=CARTESIAN_POINT('Ctrl Pts',(107.287374104876,832.521948109869,126.568462840168));
#69039=CARTESIAN_POINT('Ctrl Pts',(107.197007939246,832.447516409023,126.527426620317));
#69040=CARTESIAN_POINT('Ctrl Pts',(106.9881348606,832.3352947557,126.455529610318));
#69041=CARTESIAN_POINT('Ctrl Pts',(106.871108826735,832.299134044525,126.425504097532));
#69042=CARTESIAN_POINT('Ctrl Pts',(106.625329880769,832.271373928425,126.38110046283));
#69043=CARTESIAN_POINT('Ctrl Pts',(106.49872397112,832.280585895651,126.367331697681));
#69044=CARTESIAN_POINT('Ctrl Pts',(106.253996127618,832.34461020012,126.358504854285));
#69045=CARTESIAN_POINT('Ctrl Pts',(106.138251226854,832.39891632184,126.363572043295));
#69046=CARTESIAN_POINT('Ctrl Pts',(105.938301072436,832.543042787827,126.391358307029));
#69047=CARTESIAN_POINT('Ctrl Pts',(105.854829166522,832.629938551605,126.41306153524));
#69048=CARTESIAN_POINT('Ctrl Pts',(105.72799726863,832.824144791397,126.469234363367));
#69049=CARTESIAN_POINT('Ctrl Pts',(105.684542041252,832.928945580426,126.502750658433));
#69050=CARTESIAN_POINT('Ctrl Pts',(105.639851381538,833.147240642146,126.578298086916));
#69051=CARTESIAN_POINT('Ctrl Pts',(105.639262424399,833.25877576474,126.619681076013));
#69052=CARTESIAN_POINT('Ctrl Pts',(105.682259384937,833.477366759787,126.706389989212));
#69053=CARTESIAN_POINT('Ctrl Pts',(105.726597763458,833.582125107827,126.750961454064));
#69054=CARTESIAN_POINT('Ctrl Pts',(105.858712803437,833.773343681452,126.839110846006));
#69055=CARTESIAN_POINT('Ctrl Pts',(105.947279665046,833.856571908926,126.88160830431));
#69056=CARTESIAN_POINT('Ctrl Pts',(106.152879181124,833.982255567292,126.955692269105));
#69057=CARTESIAN_POINT('Ctrl Pts',(106.267282192868,834.024402784345,126.986809760084));
#69058=CARTESIAN_POINT('Ctrl Pts',(106.510285783741,834.064457978969,127.035086926522));
#69059=CARTESIAN_POINT('Ctrl Pts',(106.636802809456,834.061372969921,127.051599645854));
#69060=CARTESIAN_POINT('Ctrl Pts',(106.88465299152,834.008826857744,127.067108499236));
#69061=CARTESIAN_POINT('Ctrl Pts',(107.003588033846,833.959442793996,127.065793565877));
#69062=CARTESIAN_POINT('Ctrl Pts',(107.205115233036,833.827537429491,127.045796551336));
#69063=CARTESIAN_POINT('Ctrl Pts',(107.288597508492,833.750045845327,127.029088179082));
#69064=CARTESIAN_POINT('Ctrl Pts',(107.427224446225,833.567517731427,126.981229937407));
#69065=CARTESIAN_POINT('Ctrl Pts',(107.479432889011,833.462999668539,126.949838131088));
#69066=CARTESIAN_POINT('Ctrl Pts',(107.519637551879,833.318054914236,126.901465502322));
#69067=CARTESIAN_POINT('Ctrl Pts',(107.527099262435,833.282720439317,126.889322421523));
#69068=CARTESIAN_POINT('Ctrl Pts',(107.532294808004,833.247164435627,126.876755726751));
#69069=CARTESIAN_POINT('Ctrl Pts',(106.593082004706,833.382657080601,128.950197605091));
#69070=CARTESIAN_POINT('Ctrl Pts',(106.593566586252,833.382628762013,128.950277729248));
#69071=CARTESIAN_POINT('Ctrl Pts',(106.594051184575,833.382600092925,128.95035773022));
#69072=CARTESIAN_POINT('Ctrl Pts',(106.594535799255,833.38257107329,128.950437607906));
#69073=CARTESIAN_POINT('Ctrl Pts',(106.718490536038,833.375148431477,128.970868721557));
#69074=CARTESIAN_POINT('Ctrl Pts',(106.841376115117,833.344915423,128.982894032538));
#69075=CARTESIAN_POINT('Ctrl Pts',(107.069826980962,833.242557646128,128.988278417489));
#69076=CARTESIAN_POINT('Ctrl Pts',(107.173550330991,833.171754496403,128.981766361638));
#69077=CARTESIAN_POINT('Ctrl Pts',(107.347645321587,832.999315246611,128.950570955162));
#69078=CARTESIAN_POINT('Ctrl Pts',(107.41687218612,832.899849741347,128.926474465598));
#69079=CARTESIAN_POINT('Ctrl Pts',(107.51281361132,832.684051168875,128.863181751529));
#69080=CARTESIAN_POINT('Ctrl Pts',(107.538662259665,832.570042501173,128.824695839511));
#69081=CARTESIAN_POINT('Ctrl Pts',(107.543353913986,832.340478653054,128.737506920593));
#69082=CARTESIAN_POINT('Ctrl Pts',(107.52155108143,832.227438682135,128.68963989793));
#69083=CARTESIAN_POINT('Ctrl Pts',(107.431703158797,832.01661241602,128.590606090183));
#69084=CARTESIAN_POINT('Ctrl Pts',(107.363697477087,831.921395459319,128.54044669291));
#69085=CARTESIAN_POINT('Ctrl Pts',(107.189301746346,831.762226072258,128.445120679388));
#69086=CARTESIAN_POINT('Ctrl Pts',(107.083886573825,831.700446812157,128.401002341125));
#69087=CARTESIAN_POINT('Ctrl Pts',(106.850930292356,831.620656774394,128.326243839117));
#69088=CARTESIAN_POINT('Ctrl Pts',(106.725438767296,831.603433977474,128.29630366665));
#69089=CARTESIAN_POINT('Ctrl Pts',(106.596684952895,831.610049564228,128.275382995262));
#69090=CARTESIAN_POINT('Ctrl Pts',(106.594883381751,831.610146901093,128.275092185357));
#69091=CARTESIAN_POINT('Ctrl Pts',(106.593082004564,831.610248993975,128.2748033254));
#69092=CARTESIAN_POINT('Origin',(106.593082004564,836.288239824643,117.884080028985));
#69093=CARTESIAN_POINT('',(106.593082004564,834.624823193137,124.090975272474));
#69094=CARTESIAN_POINT('Origin',(106.593082004564,834.153400962528,123.924358705207));
#69095=CARTESIAN_POINT('',(106.593082004564,832.964211408695,128.789483496701));
#69096=CARTESIAN_POINT('',(106.593082004564,836.759662055252,118.050696596252));
#69097=CARTESIAN_POINT('Ctrl Pts',(106.593366660624,832.02945867497,128.433356001948));
#69098=CARTESIAN_POINT('Ctrl Pts',(106.529229872268,832.033084018716,128.422988938261));
#69099=CARTESIAN_POINT('Ctrl Pts',(106.465562429969,832.048176387402,128.417210567738));
#69100=CARTESIAN_POINT('Ctrl Pts',(106.344515676303,832.100634675078,128.415463730008));
#69101=CARTESIAN_POINT('Ctrl Pts',(106.288518675592,832.138112024034,128.419788627033));
#69102=CARTESIAN_POINT('Ctrl Pts',(106.195294077639,832.229555154974,128.43811226833));
#69103=CARTESIAN_POINT('Ctrl Pts',(106.158509650955,832.282139172819,128.451657695177));
#69104=CARTESIAN_POINT('Ctrl Pts',(106.107748472945,832.396354998587,128.486163431682));
#69105=CARTESIAN_POINT('Ctrl Pts',(106.09418295559,832.456768272901,128.506730952175));
#69106=CARTESIAN_POINT('Ctrl Pts',(106.092103923698,832.578126861548,128.552413755081));
#69107=CARTESIAN_POINT('Ctrl Pts',(106.103748191406,832.637801790198,128.577075359564));
#69108=CARTESIAN_POINT('Ctrl Pts',(106.151528610457,832.749639875857,128.627895107614));
#69109=CARTESIAN_POINT('Ctrl Pts',(106.187801996539,832.80036912786,128.653537993184));
#69110=CARTESIAN_POINT('Ctrl Pts',(106.280135616138,832.884421758021,128.701911539482));
#69111=CARTESIAN_POINT('Ctrl Pts',(106.33536955164,832.916828547416,128.72415136493));
#69112=CARTESIAN_POINT('Ctrl Pts',(106.457595851277,832.958840007983,128.762366164734));
#69113=CARTESIAN_POINT('Ctrl Pts',(106.523547910496,832.967875206953,128.777939067417));
#69114=CARTESIAN_POINT('Ctrl Pts',(106.657248103403,832.960845441647,128.800142247882));
#69115=CARTESIAN_POINT('Ctrl Pts',(106.723796670554,832.944694340638,128.806517052477));
#69116=CARTESIAN_POINT('Ctrl Pts',(106.845790324969,832.88983692334,128.808763319625));
#69117=CARTESIAN_POINT('Ctrl Pts',(106.90044739155,832.852405460387,128.804961284532));
#69118=CARTESIAN_POINT('Ctrl Pts',(106.99212519188,832.761229910569,128.787811655891));
#69119=CARTESIAN_POINT('Ctrl Pts',(107.028515633763,832.708620735536,128.774771708297));
#69120=CARTESIAN_POINT('Ctrl Pts',(107.078724348598,832.594535865148,128.740911588646));
#69121=CARTESIAN_POINT('Ctrl Pts',(107.092100143423,832.534283978702,128.720471727768));
#69122=CARTESIAN_POINT('Ctrl Pts',(107.093969569075,832.413137018149,128.674484579145));
#69123=CARTESIAN_POINT('Ctrl Pts',(107.082180859807,832.353551432732,128.649383923729));
#69124=CARTESIAN_POINT('Ctrl Pts',(107.034299560962,832.24257144573,128.59765875814));
#69125=CARTESIAN_POINT('Ctrl Pts',(106.998277536441,832.19250631668,128.571560224117));
#69126=CARTESIAN_POINT('Ctrl Pts',(106.905797872564,832.108583894106,128.521815529678));
#69127=CARTESIAN_POINT('Ctrl Pts',(106.849745265658,832.076014003546,128.498746767882));
#69128=CARTESIAN_POINT('Ctrl Pts',(106.726368574756,832.034423712299,128.459756828865));
#69129=CARTESIAN_POINT('Ctrl Pts',(106.660208106405,832.025680449965,128.444160246175));
#69130=CARTESIAN_POINT('Ctrl Pts',(106.593366660624,832.02945867497,128.433356001948));
#69131=CARTESIAN_POINT('Origin',(102.144722372893,820.841213146102,112.424578137575));
#69132=CARTESIAN_POINT('',(102.144722372892,816.254389947185,122.337315571232));
#69133=CARTESIAN_POINT('',(102.144722372897,818.188798096017,122.994424754414));
#69134=CARTESIAN_POINT('Ctrl Pts',(102.144722372892,816.254389947185,122.337315571232));
#69135=CARTESIAN_POINT('Ctrl Pts',(102.01448283502,816.257559043848,122.3283489802));
#69136=CARTESIAN_POINT('Ctrl Pts',(101.885333726022,816.284085748256,122.328050406789));
#69137=CARTESIAN_POINT('Ctrl Pts',(101.639205011226,816.382794367041,122.345203847486));
#69138=CARTESIAN_POINT('Ctrl Pts',(101.525237096631,816.455477147213,122.363071347237));
#69139=CARTESIAN_POINT('Ctrl Pts',(101.33324081447,816.637328130539,122.414444751396));
#69140=CARTESIAN_POINT('Ctrl Pts',(101.256924249962,816.744528982366,122.44735071358));
#69141=CARTESIAN_POINT('Ctrl Pts',(101.151828310525,816.980361239478,122.523340516029));
#69142=CARTESIAN_POINT('Ctrl Pts',(101.124248130998,817.106731592453,122.565686789286));
#69143=CARTESIAN_POINT('Ctrl Pts',(101.12242427395,817.361930091502,122.653628596318));
#69144=CARTESIAN_POINT('Ctrl Pts',(101.148341013592,817.488234278117,122.698352287058));
#69145=CARTESIAN_POINT('Ctrl Pts',(101.250666563817,817.722869309163,122.783883616561));
#69146=CARTESIAN_POINT('Ctrl Pts',(101.325914958908,817.828934815759,122.823867312529));
#69147=CARTESIAN_POINT('Ctrl Pts',(101.515724899758,818.006218208579,122.894269023263));
#69148=CARTESIAN_POINT('Ctrl Pts',(101.628300437093,818.075786292927,122.924039736244));
#69149=CARTESIAN_POINT('Ctrl Pts',(101.876649923645,818.169079109118,122.970299909665));
#69150=CARTESIAN_POINT('Ctrl Pts',(102.010057204773,818.19167386802,122.986288091447));
#69151=CARTESIAN_POINT('Ctrl Pts',(102.144722372902,818.188798096017,122.994424754414));
#69152=CARTESIAN_POINT('',(102.14472237325,818.827174390792,121.18821315261));
#69153=CARTESIAN_POINT('',(102.144722372893,821.804242286345,112.764945220642));
#69154=CARTESIAN_POINT('Ctrl Pts',(103.149564180549,817.660946014935,120.872963773621));
#69155=CARTESIAN_POINT('Ctrl Pts',(103.125674937399,817.537414267004,120.829303474101));
#69156=CARTESIAN_POINT('Ctrl Pts',(103.076397526074,817.420234466966,120.785571257734));
#69157=CARTESIAN_POINT('Ctrl Pts',(102.932682761671,817.211704355957,120.70301803522));
#69158=CARTESIAN_POINT('Ctrl Pts',(102.839646051471,817.122387338972,120.6650077997));
#69159=CARTESIAN_POINT('Ctrl Pts',(102.621322617236,816.983180158415,120.599954793548));
#69160=CARTESIAN_POINT('Ctrl Pts',(102.497992734769,816.934798730656,120.573593326978));
#69161=CARTESIAN_POINT('Ctrl Pts',(102.236940011704,816.8859357297,120.536558770922));
#69162=CARTESIAN_POINT('Ctrl Pts',(102.101642396639,816.886127045467,120.526313459366));
#69163=CARTESIAN_POINT('Ctrl Pts',(101.83739496844,816.935801832543,120.52377438526));
#69164=CARTESIAN_POINT('Ctrl Pts',(101.710979198984,816.984862841166,120.531525035075));
#69165=CARTESIAN_POINT('Ctrl Pts',(101.485292475534,817.125248122336,120.563932606559));
#69166=CARTESIAN_POINT('Ctrl Pts',(101.387925527677,817.214834393102,120.588115179616));
#69167=CARTESIAN_POINT('Ctrl Pts',(101.233142430397,817.424911210335,120.649959033043));
#69168=CARTESIAN_POINT('Ctrl Pts',(101.177782792624,817.543706890498,120.687167705484));
#69169=CARTESIAN_POINT('Ctrl Pts',(101.118555136005,817.794112423427,120.769178597195));
#69170=CARTESIAN_POINT('Ctrl Pts',(101.115360280281,817.923247652267,120.813167882312));
#69171=CARTESIAN_POINT('Ctrl Pts',(101.162031716901,818.172995627507,120.90134109584));
#69172=CARTESIAN_POINT('Ctrl Pts',(101.21091572821,818.291236803578,120.944656272247));
#69173=CARTESIAN_POINT('Ctrl Pts',(101.354357723054,818.502108459169,121.025366483967));
#69174=CARTESIAN_POINT('Ctrl Pts',(101.447480445364,818.592697757262,121.061984706085));
#69175=CARTESIAN_POINT('Ctrl Pts',(101.665567720486,818.733675018226,121.123886899891));
#69176=CARTESIAN_POINT('Ctrl Pts',(101.788318947099,818.782834550997,121.148620174046));
#69177=CARTESIAN_POINT('Ctrl Pts',(102.048820054437,818.833399767813,121.183494725859));
#69178=CARTESIAN_POINT('Ctrl Pts',(102.18416229911,818.833908535048,121.193179467386));
#69179=CARTESIAN_POINT('Ctrl Pts',(102.450028231007,818.784865476997,121.195977643805));
#69180=CARTESIAN_POINT('Ctrl Pts',(102.577876152832,818.735199674138,121.188865621007));
#69181=CARTESIAN_POINT('Ctrl Pts',(102.805630027172,818.592511939164,121.158446593098));
#69182=CARTESIAN_POINT('Ctrl Pts',(102.903652690307,818.501330804433,121.135600440196));
#69183=CARTESIAN_POINT('Ctrl Pts',(103.057825743493,818.289130385116,121.076746003304));
#69184=CARTESIAN_POINT('Ctrl Pts',(103.112536102743,818.170203762147,121.041315367079));
#69185=CARTESIAN_POINT('Ctrl Pts',(103.156416811535,817.982240369834,120.981747837426));
#69186=CARTESIAN_POINT('Ctrl Pts',(103.164526141302,817.918194852751,120.960878456479));
#69187=CARTESIAN_POINT('Ctrl Pts',(103.167320560797,817.789129935012,120.917658471095));
#69188=CARTESIAN_POINT('Ctrl Pts',(103.161843562539,817.724442941614,120.895405735981));
#69189=CARTESIAN_POINT('Ctrl Pts',(103.149564180549,817.660946014935,120.872963773621));
#69190=CARTESIAN_POINT('Ctrl Pts',(102.144722372902,818.188798096017,122.994424754414));
#69191=CARTESIAN_POINT('Ctrl Pts',(102.144921974185,818.188793833536,122.99443681461));
#69192=CARTESIAN_POINT('Ctrl Pts',(102.145121578235,818.188789515112,122.99444885751));
#69193=CARTESIAN_POINT('Ctrl Pts',(102.145321185027,818.188785140742,122.994460883112));
#69194=CARTESIAN_POINT('Ctrl Pts',(102.276018833491,818.185920910063,123.002334953166));
#69195=CARTESIAN_POINT('Ctrl Pts',(102.405450290849,818.159117399055,123.002667847017));
#69196=CARTESIAN_POINT('Ctrl Pts',(102.650512819559,818.059523212747,122.988014642784));
#69197=CARTESIAN_POINT('Ctrl Pts',(102.76345024988,817.986634529791,122.97280862151));
#69198=CARTESIAN_POINT('Ctrl Pts',(102.954123678733,817.804611259951,122.928076170702));
#69199=CARTESIAN_POINT('Ctrl Pts',(103.030215612037,817.697335910332,122.899013288643));
#69200=CARTESIAN_POINT('Ctrl Pts',(103.135434359748,817.462463797933,122.830052773349));
#69201=CARTESIAN_POINT('Ctrl Pts',(103.163681801997,817.337182959394,122.790834743897));
#69202=CARTESIAN_POINT('Ctrl Pts',(103.168279574962,817.08454906744,122.706661062042));
#69203=CARTESIAN_POINT('Ctrl Pts',(103.144479540307,816.959702721951,122.662524637957));
#69204=CARTESIAN_POINT('Ctrl Pts',(103.047084629083,816.726621903064,122.574967012687));
#69205=CARTESIAN_POINT('Ctrl Pts',(102.974184798905,816.62082493286,122.5324356244));
#69206=CARTESIAN_POINT('Ctrl Pts',(102.788264169511,816.442764856226,122.455239610837));
#69207=CARTESIAN_POINT('Ctrl Pts',(102.676884053809,816.372408509239,122.42138543827));
#69208=CARTESIAN_POINT('Ctrl Pts',(102.430524716656,816.277126019276,122.367880826043));
#69209=CARTESIAN_POINT('Ctrl Pts',(102.29788291689,816.253140111851,122.3487674368));
#69210=CARTESIAN_POINT('Ctrl Pts',(102.157209430967,816.254139835481,122.338194956278));
#69211=CARTESIAN_POINT('Ctrl Pts',(102.150964647552,816.254238054971,122.337745332615));
#69212=CARTESIAN_POINT('Ctrl Pts',(102.144722372892,816.254389947185,122.337315571232));
#69213=CARTESIAN_POINT('Origin',(102.144722372893,820.841213146102,112.424578137575));
#69214=CARTESIAN_POINT('',(102.144722372893,819.177796514596,118.631473381063));
#69215=CARTESIAN_POINT('Origin',(102.144722372893,818.706374283987,118.464856813796));
#69216=CARTESIAN_POINT('',(102.144722372893,817.695341518356,122.825907659524));
#69217=CARTESIAN_POINT('',(102.144722372893,821.312635376711,112.591194704842));
#69218=CARTESIAN_POINT('Ctrl Pts',(102.144732739577,816.748420555005,122.504208514761));
#69219=CARTESIAN_POINT('Ctrl Pts',(102.082926213998,816.749872861288,122.500095537239));
#69220=CARTESIAN_POINT('Ctrl Pts',(102.021641901999,816.76211826188,122.49983554938));
#69221=CARTESIAN_POINT('Ctrl Pts',(101.902064442961,816.808636819692,122.507325850532));
#69222=CARTESIAN_POINT('Ctrl Pts',(101.845509411206,816.844022033751,122.515598795588));
#69223=CARTESIAN_POINT('Ctrl Pts',(101.749938477978,816.933202929328,122.539823115067));
#69224=CARTESIAN_POINT('Ctrl Pts',(101.711824469246,816.986063262919,122.555508832254));
#69225=CARTESIAN_POINT('Ctrl Pts',(101.659266657108,817.102456110172,122.592085811327));
#69226=CARTESIAN_POINT('Ctrl Pts',(101.645383934472,817.164835103884,122.612612541681));
#69227=CARTESIAN_POINT('Ctrl Pts',(101.644106180934,817.290698493168,122.655611028783));
#69228=CARTESIAN_POINT('Ctrl Pts',(101.65675679843,817.352913990414,122.677649309188));
#69229=CARTESIAN_POINT('Ctrl Pts',(101.707115239758,817.468441092188,122.72016248875));
#69230=CARTESIAN_POINT('Ctrl Pts',(101.744281836181,817.520600863929,122.740213358666));
#69231=CARTESIAN_POINT('Ctrl Pts',(101.838182831566,817.607598727747,122.77570469556));
#69232=CARTESIAN_POINT('Ctrl Pts',(101.893952197496,817.641585061121,122.790799450178));
#69233=CARTESIAN_POINT('Ctrl Pts',(102.016836789362,817.686674346669,122.814181924386));
#69234=CARTESIAN_POINT('Ctrl Pts',(102.082758896603,817.697254907804,122.822218828137));
#69235=CARTESIAN_POINT('Ctrl Pts',(102.214775570901,817.69321892032,122.830091342823));
#69236=CARTESIAN_POINT('Ctrl Pts',(102.279591222087,817.678966204137,122.829957578635));
#69237=CARTESIAN_POINT('Ctrl Pts',(102.400208867725,817.627657586543,122.821614891196));
#69238=CARTESIAN_POINT('Ctrl Pts',(102.45488301693,817.591125059419,122.813496122556));
#69239=CARTESIAN_POINT('Ctrl Pts',(102.546662548993,817.500589627919,122.790178445001));
#69240=CARTESIAN_POINT('Ctrl Pts',(102.582955436481,817.447506317204,122.775221177029));
#69241=CARTESIAN_POINT('Ctrl Pts',(102.632278395286,817.331714167397,122.740216771296));
#69242=CARTESIAN_POINT('Ctrl Pts',(102.644883606345,817.270147421615,122.720516185985));
#69243=CARTESIAN_POINT('Ctrl Pts',(102.644557862627,817.146454664415,122.678761190402));
#69244=CARTESIAN_POINT('Ctrl Pts',(102.631604154655,817.085548920734,122.657115130615));
#69245=CARTESIAN_POINT('Ctrl Pts',(102.581493193793,816.972361457722,122.614685200656));
#69246=CARTESIAN_POINT('Ctrl Pts',(102.544745732041,816.921234710257,122.594327355879));
#69247=CARTESIAN_POINT('Ctrl Pts',(102.452028501185,816.835709539048,122.557770320426));
#69248=CARTESIAN_POINT('Ctrl Pts',(102.396899514493,816.802207792346,122.541947773768));
#69249=CARTESIAN_POINT('Ctrl Pts',(102.27553269161,816.757561985037,122.517228039019));
#69250=CARTESIAN_POINT('Ctrl Pts',(102.210446181577,816.746876445483,122.508581481974));
#69251=CARTESIAN_POINT('Ctrl Pts',(102.144732739577,816.748420555005,122.504208514761));
#69252=CARTESIAN_POINT('Origin',(106.957908439915,825.606009837406,114.108618509208));
#69253=CARTESIAN_POINT('',(106.957908439915,820.918639451936,124.525880166841));
#69254=CARTESIAN_POINT('',(106.957908439943,822.714037109275,125.136228125604));
#69255=CARTESIAN_POINT('Ctrl Pts',(106.957908439915,820.918639451935,124.525880166841));
#69256=CARTESIAN_POINT('Ctrl Pts',(106.834925181281,820.925791453,124.505644410275));
#69257=CARTESIAN_POINT('Ctrl Pts',(106.712929193591,820.955387903885,124.493716319717));
#69258=CARTESIAN_POINT('Ctrl Pts',(106.483232995468,821.05718149143,124.48782534621));
#69259=CARTESIAN_POINT('Ctrl Pts',(106.377868908004,821.128953076226,124.494135968551));
#69260=CARTESIAN_POINT('Ctrl Pts',(106.200587221442,821.305509989051,124.524310281196));
#69261=CARTESIAN_POINT('Ctrl Pts',(106.130232003092,821.408347994478,124.547757301054));
#69262=CARTESIAN_POINT('Ctrl Pts',(106.035173096044,821.630095879669,124.607839960344));
#69263=CARTESIAN_POINT('Ctrl Pts',(106.010538595136,821.746405328518,124.643583786556));
#69264=CARTESIAN_POINT('Ctrl Pts',(106.009133011291,821.980490748669,124.723295580061));
#69265=CARTESIAN_POINT('Ctrl Pts',(106.032860954363,822.095809796808,124.766502341402));
#69266=CARTESIAN_POINT('Ctrl Pts',(106.12680995675,822.309749177369,124.854856915442));
#69267=CARTESIAN_POINT('Ctrl Pts',(106.196498804425,822.405912616758,124.899089097247));
#69268=CARTESIAN_POINT('Ctrl Pts',(106.372588764774,822.564856895177,124.982741063986));
#69269=CARTESIAN_POINT('Ctrl Pts',(106.477298528654,822.625902635073,125.021302078196));
#69270=CARTESIAN_POINT('Ctrl Pts',(106.708338259671,822.704652344538,125.088258991379));
#69271=CARTESIAN_POINT('Ctrl Pts',(106.83262340867,822.721212144327,125.115927197065));
#69272=CARTESIAN_POINT('Ctrl Pts',(106.957908439971,822.714037109275,125.136228125604));
#69273=CARTESIAN_POINT('',(106.957908439915,823.382883520564,123.243804867125));
#69274=CARTESIAN_POINT('',(106.957908439915,826.499906010025,114.424551662345));
#69275=CARTESIAN_POINT('Ctrl Pts',(107.903500219465,822.378156070275,123.035280408344));
#69276=CARTESIAN_POINT('Ctrl Pts',(107.894920100932,822.266815941935,122.995929039701));
#69277=CARTESIAN_POINT('Ctrl Pts',(107.864302758957,822.159102313565,122.954511621887));
#69278=CARTESIAN_POINT('Ctrl Pts',(107.759471279212,821.956476440659,122.869618837775));
#69279=CARTESIAN_POINT('Ctrl Pts',(107.684005985044,821.864704993812,122.827038340615));
#69280=CARTESIAN_POINT('Ctrl Pts',(107.500409159485,821.717155731259,122.749683624278));
#69281=CARTESIAN_POINT('Ctrl Pts',(107.394583870129,821.662166004448,122.715518855886));
#69282=CARTESIAN_POINT('Ctrl Pts',(107.16329529463,821.593563026828,122.659038161755));
#69283=CARTESIAN_POINT('Ctrl Pts',(107.039657774991,821.581251338835,122.637441700713));
#69284=CARTESIAN_POINT('Ctrl Pts',(106.790731498044,821.602514999532,122.610364727493));
#69285=CARTESIAN_POINT('Ctrl Pts',(106.667744096107,821.636460901695,122.605337771844));
#69286=CARTESIAN_POINT('Ctrl Pts',(106.440303173469,821.747275688919,122.613048268249));
#69287=CARTESIAN_POINT('Ctrl Pts',(106.338084188269,821.823181366092,122.625749470995));
#69288=CARTESIAN_POINT('Ctrl Pts',(106.172681420484,822.003513190906,122.666331933578));
#69289=CARTESIAN_POINT('Ctrl Pts',(106.109571278476,822.104934787982,122.693169082771));
#69290=CARTESIAN_POINT('Ctrl Pts',(106.027472723286,822.319845397616,122.756659535749));
#69291=CARTESIAN_POINT('Ctrl Pts',(106.007833138054,822.430898689888,122.79238567702));
#69292=CARTESIAN_POINT('Ctrl Pts',(106.01214526248,822.653195141141,122.869347331955));
#69293=CARTESIAN_POINT('Ctrl Pts',(106.036300365844,822.762394930614,122.909904935309));
#69294=CARTESIAN_POINT('Ctrl Pts',(106.127215238831,822.967715671916,122.991923691824));
#69295=CARTESIAN_POINT('Ctrl Pts',(106.194208374972,823.061441406852,123.032595857908));
#69296=CARTESIAN_POINT('Ctrl Pts',(106.367027912732,823.22244189507,123.110065156012));
#69297=CARTESIAN_POINT('Ctrl Pts',(106.472918825171,823.286399950998,123.145751883668));
#69298=CARTESIAN_POINT('Ctrl Pts',(106.703795827351,823.368830119372,123.204548601583));
#69299=CARTESIAN_POINT('Ctrl Pts',(106.826116824876,823.387518710045,123.227375020255));
#69300=CARTESIAN_POINT('Ctrl Pts',(107.07500694945,823.378828739677,123.258423996052));
#69301=CARTESIAN_POINT('Ctrl Pts',(107.199298577057,823.350889359037,123.266152339495));
#69302=CARTESIAN_POINT('Ctrl Pts',(107.432506609306,823.250671846939,123.264812507143));
#69303=CARTESIAN_POINT('Ctrl Pts',(107.539070854672,823.17894149244,123.255599638526));
#69304=CARTESIAN_POINT('Ctrl Pts',(107.708951550872,823.010230739755,123.222594354461));
#69305=CARTESIAN_POINT('Ctrl Pts',(107.774261380901,822.917994312338,123.200674655697));
#69306=CARTESIAN_POINT('Ctrl Pts',(107.870762530212,822.712165723077,123.144581237638));
#69307=CARTESIAN_POINT('Ctrl Pts',(107.899166665534,822.599659199883,123.110366039151));
#69308=CARTESIAN_POINT('Ctrl Pts',(107.906728069839,822.449980974197,123.060320441437));
#69309=CARTESIAN_POINT('Ctrl Pts',(107.906258854175,822.413953564389,123.047932454002));
#69310=CARTESIAN_POINT('Ctrl Pts',(107.903500219465,822.378156070276,123.035280408344));
#69311=CARTESIAN_POINT('Ctrl Pts',(106.957908439971,822.714037109275,125.136228125604));
#69312=CARTESIAN_POINT('Ctrl Pts',(106.958225949864,822.714018925581,125.136279574254));
#69313=CARTESIAN_POINT('Ctrl Pts',(106.958543466198,822.71400058948,125.136330975481));
#69314=CARTESIAN_POINT('Ctrl Pts',(106.958860988855,822.713982100959,125.136382329263));
#69315=CARTESIAN_POINT('Ctrl Pts',(107.082183504009,822.706801350697,125.156327606682));
#69316=CARTESIAN_POINT('Ctrl Pts',(107.204315847898,822.676748446124,125.168784705021));
#69317=CARTESIAN_POINT('Ctrl Pts',(107.433103833348,822.574019529265,125.177189969658));
#69318=CARTESIAN_POINT('Ctrl Pts',(107.537700475697,822.501998097256,125.172968233913));
#69319=CARTESIAN_POINT('Ctrl Pts',(107.712795108306,822.326444658996,125.147723308565));
#69320=CARTESIAN_POINT('Ctrl Pts',(107.782301520331,822.225112537125,125.12723078329));
#69321=CARTESIAN_POINT('Ctrl Pts',(107.877977001318,822.005904816772,125.072143002326));
#69322=CARTESIAN_POINT('Ctrl Pts',(107.903664443433,821.890420768215,125.038250930893));
#69323=CARTESIAN_POINT('Ctrl Pts',(107.908029172466,821.65853590756,124.960632384663));
#69324=CARTESIAN_POINT('Ctrl Pts',(107.886442783627,821.544640051224,124.917698480754));
#69325=CARTESIAN_POINT('Ctrl Pts',(107.797513666835,821.332093544325,124.827822923118));
#69326=CARTESIAN_POINT('Ctrl Pts',(107.730340044753,821.236057615969,124.781807555512));
#69327=CARTESIAN_POINT('Ctrl Pts',(107.558029632007,821.075177001686,124.693188387097));
#69328=CARTESIAN_POINT('Ctrl Pts',(107.453962582539,821.012564342653,124.651570996227));
#69329=CARTESIAN_POINT('Ctrl Pts',(107.221766398994,820.930086273414,124.578987427032));
#69330=CARTESIAN_POINT('Ctrl Pts',(107.095367494674,820.91191116206,124.548954811932));
#69331=CARTESIAN_POINT('Ctrl Pts',(106.964318597556,820.918281957199,124.526940418755));
#69332=CARTESIAN_POINT('Ctrl Pts',(106.96111318255,820.918453082482,124.526407477571));
#69333=CARTESIAN_POINT('Ctrl Pts',(106.957908439915,820.918639451935,124.525880166841));
#69334=CARTESIAN_POINT('Origin',(106.957908439915,825.606009837406,114.108618509208));
#69335=CARTESIAN_POINT('',(106.957908439915,823.9425932059,120.315513752696));
#69336=CARTESIAN_POINT('Origin',(106.957908439915,823.471170975291,120.148897185429));
#69337=CARTESIAN_POINT('',(106.957908439915,822.290121186054,124.990991458137));
#69338=CARTESIAN_POINT('',(106.957908439915,826.077432068015,114.275235076475));
#69339=CARTESIAN_POINT('Ctrl Pts',(106.958222165921,821.343250545434,124.669150226088));
#69340=CARTESIAN_POINT('Ctrl Pts',(106.892818314994,821.346999101619,124.658420971245));
#69341=CARTESIAN_POINT('Ctrl Pts',(106.827973941537,821.362822182442,124.652039907669));
#69342=CARTESIAN_POINT('Ctrl Pts',(106.706127188088,821.417263436913,124.648701539818));
#69343=CARTESIAN_POINT('Ctrl Pts',(106.650342596402,821.455633557114,124.651879470715));
#69344=CARTESIAN_POINT('Ctrl Pts',(106.557641531978,821.549011664705,124.667387009783));
#69345=CARTESIAN_POINT('Ctrl Pts',(106.521165926485,821.60268099703,124.679330397564));
#69346=CARTESIAN_POINT('Ctrl Pts',(106.471381547181,821.718859927245,124.710292783712));
#69347=CARTESIAN_POINT('Ctrl Pts',(106.458365251161,821.780114158469,124.728931282838));
#69348=CARTESIAN_POINT('Ctrl Pts',(106.457475142972,821.902759510721,124.770570785216));
#69349=CARTESIAN_POINT('Ctrl Pts',(106.469617489539,821.962874942451,124.793139263138));
#69350=CARTESIAN_POINT('Ctrl Pts',(106.518091875654,822.075026388566,124.839711185584));
#69351=CARTESIAN_POINT('Ctrl Pts',(106.554351749362,822.125697829141,124.863239789614));
#69352=CARTESIAN_POINT('Ctrl Pts',(106.646693326278,822.210122721922,124.908110195148));
#69353=CARTESIAN_POINT('Ctrl Pts',(106.702091361353,822.24275767519,124.928957256173));
#69354=CARTESIAN_POINT('Ctrl Pts',(106.824493076789,822.284924682606,124.965086126507));
#69355=CARTESIAN_POINT('Ctrl Pts',(106.890407855879,822.29387030579,124.979979312455));
#69356=CARTESIAN_POINT('Ctrl Pts',(107.023922870188,822.286456511742,125.001761775637));
#69357=CARTESIAN_POINT('Ctrl Pts',(107.090317110489,822.269963943636,125.008388908033));
#69358=CARTESIAN_POINT('Ctrl Pts',(107.212406525572,822.214057763881,125.012129928141));
#69359=CARTESIAN_POINT('Ctrl Pts',(107.267258714984,822.175707090314,125.009439146229));
#69360=CARTESIAN_POINT('Ctrl Pts',(107.358868248356,822.082477678299,124.995170712216));
#69361=CARTESIAN_POINT('Ctrl Pts',(107.395075626198,822.028754809419,124.983875259776));
#69362=CARTESIAN_POINT('Ctrl Pts',(107.444481559075,821.912698140194,124.953991540321));
#69363=CARTESIAN_POINT('Ctrl Pts',(107.457416616252,821.851624437337,124.935777180103));
#69364=CARTESIAN_POINT('Ctrl Pts',(107.458374458683,821.729254849129,124.894454762244));
#69365=CARTESIAN_POINT('Ctrl Pts',(107.44629735527,821.669267360435,124.871770656094));
#69366=CARTESIAN_POINT('Ctrl Pts',(107.398096093024,821.557651868738,124.824619385304));
#69367=CARTESIAN_POINT('Ctrl Pts',(107.362122648394,821.507365458191,124.800638495034));
#69368=CARTESIAN_POINT('Ctrl Pts',(107.270199522723,821.423229564206,124.754549414011));
#69369=CARTESIAN_POINT('Ctrl Pts',(107.214773418277,821.390617372222,124.732966782589));
#69370=CARTESIAN_POINT('Ctrl Pts',(107.091840519965,821.348340849408,124.695551428081));
#69371=CARTESIAN_POINT('Ctrl Pts',(107.0253371481,821.339403917476,124.680160185553));
#69372=CARTESIAN_POINT('Ctrl Pts',(106.958222165921,821.343250545434,124.669150226088));
#69373=CARTESIAN_POINT('Origin',(99.2004494076648,811.368542512753,109.076615819925));
#69374=CARTESIAN_POINT('',(99.2004494076648,806.777379182049,119.001633152524));
#69375=CARTESIAN_POINT('',(99.200449407666,808.721073021462,119.632469552402));
#69376=CARTESIAN_POINT('Ctrl Pts',(99.2004494076648,806.777379182049,119.001633152524));
#69377=CARTESIAN_POINT('Ctrl Pts',(99.070502125323,806.780520677886,118.992744654824));
#69378=CARTESIAN_POINT('Ctrl Pts',(98.9416808923822,806.807078066664,118.992024529602));
#69379=CARTESIAN_POINT('Ctrl Pts',(98.6948096590929,806.906338889037,119.007670425697));
#69380=CARTESIAN_POINT('Ctrl Pts',(98.5799610544503,806.980050408541,119.024646475322));
#69381=CARTESIAN_POINT('Ctrl Pts',(98.3874632645327,807.163969124872,119.0740877708));
#69382=CARTESIAN_POINT('Ctrl Pts',(98.3112963781483,807.271951410195,119.10587854437));
#69383=CARTESIAN_POINT('Ctrl Pts',(98.2069661211874,807.508722169788,119.179510555792));
#69384=CARTESIAN_POINT('Ctrl Pts',(98.1797558642064,807.63514960335,119.220591621919));
#69385=CARTESIAN_POINT('Ctrl Pts',(98.1783519247404,807.890441700475,119.306045394217));
#69386=CARTESIAN_POINT('Ctrl Pts',(98.2043440701219,808.016792532354,119.349568694292));
#69387=CARTESIAN_POINT('Ctrl Pts',(98.3067294635506,808.251973127116,119.432723418524));
#69388=CARTESIAN_POINT('Ctrl Pts',(98.3821106445267,808.358483040857,119.47153464452));
#69389=CARTESIAN_POINT('Ctrl Pts',(98.5722066780431,808.536635542329,119.539347110914));
#69390=CARTESIAN_POINT('Ctrl Pts',(98.6849255663226,808.606633366165,119.567727414568));
#69391=CARTESIAN_POINT('Ctrl Pts',(98.9331184060169,808.700554506976,119.611047527071));
#69392=CARTESIAN_POINT('Ctrl Pts',(99.0661564394842,808.723512096891,119.625568471686));
#69393=CARTESIAN_POINT('Ctrl Pts',(99.2004494076673,808.721073021462,119.632469552402));
#69394=CARTESIAN_POINT('',(99.2004494083662,809.359064969247,117.827345415779));
#69395=CARTESIAN_POINT('',(99.2004494076648,812.331571652995,109.416982902992));
#69396=CARTESIAN_POINT('Ctrl Pts',(100.145240424235,807.995072722745,117.456717099162));
#69397=CARTESIAN_POINT('Ctrl Pts',(100.094632569839,807.878923409672,117.415666001911));
#69398=CARTESIAN_POINT('Ctrl Pts',(100.020431519131,807.773979948127,117.376258521595));
#69399=CARTESIAN_POINT('Ctrl Pts',(99.8332599057883,807.598239666649,117.305294334309));
#69400=CARTESIAN_POINT('Ctrl Pts',(99.7221141346367,807.529156510007,117.274435429664));
#69401=CARTESIAN_POINT('Ctrl Pts',(99.4767659606996,807.4358977698,117.225622157036));
#69402=CARTESIAN_POINT('Ctrl Pts',(99.3448205956772,807.412813339474,117.208201505304));
#69403=CARTESIAN_POINT('Ctrl Pts',(99.0773280981939,807.416327555735,117.18967883004));
#69404=CARTESIAN_POINT('Ctrl Pts',(98.9443147373734,807.44310766981,117.18883089946));
#69405=CARTESIAN_POINT('Ctrl Pts',(98.6954035029874,807.543634913197,117.204264804051));
#69406=CARTESIAN_POINT('Ctrl Pts',(98.5819045605111,807.61647073709,117.220418278023));
#69407=CARTESIAN_POINT('Ctrl Pts',(98.3909144294154,807.798147422045,117.267419628734));
#69408=CARTESIAN_POINT('Ctrl Pts',(98.3149120778216,807.904914060929,117.297674325197));
#69409=CARTESIAN_POINT('Ctrl Pts',(98.2089771137064,808.140827241832,117.368649623739));
#69410=CARTESIAN_POINT('Ctrl Pts',(98.180692473151,808.267911814532,117.408787871265));
#69411=CARTESIAN_POINT('Ctrl Pts',(98.1775276413204,808.524500252524,117.492984010829));
#69412=CARTESIAN_POINT('Ctrl Pts',(98.2027644838337,808.651451187789,117.536201292689));
#69413=CARTESIAN_POINT('Ctrl Pts',(98.3034826405417,808.886593304448,117.619212301592));
#69414=CARTESIAN_POINT('Ctrl Pts',(98.3774780539923,808.99265750479,117.658223722759));
#69415=CARTESIAN_POINT('Ctrl Pts',(98.5647141782149,809.170759968649,117.727352193347));
#69416=CARTESIAN_POINT('Ctrl Pts',(98.6760970421638,809.24108338769,117.756807768096));
#69417=CARTESIAN_POINT('Ctrl Pts',(98.9213429057008,809.336145749598,117.802482083006));
#69418=CARTESIAN_POINT('Ctrl Pts',(99.0527619843972,809.360117781331,117.818313242053));
#69419=CARTESIAN_POINT('Ctrl Pts',(99.319898951195,809.35839567637,117.834707685165));
#69420=CARTESIAN_POINT('Ctrl Pts',(99.4530543644905,809.332297145673,117.834988507322));
#69421=CARTESIAN_POINT('Ctrl Pts',(99.7036905226119,809.232070307862,117.819696604127));
#69422=CARTESIAN_POINT('Ctrl Pts',(99.8185160106895,809.158356311189,117.804085135945));
#69423=CARTESIAN_POINT('Ctrl Pts',(100.011214546557,808.974003026396,117.75894009294));
#69424=CARTESIAN_POINT('Ctrl Pts',(100.087638237152,808.865534790757,117.729984093654));
#69425=CARTESIAN_POINT('Ctrl Pts',(100.19276731775,808.627638321872,117.662047803397));
#69426=CARTESIAN_POINT('Ctrl Pts',(100.220514387367,808.500540419521,117.623729160557));
#69427=CARTESIAN_POINT('Ctrl Pts',(100.222463015951,808.308035479834,117.562556494394));
#69428=CARTESIAN_POINT('Ctrl Pts',(100.216394503391,808.243787723999,117.54161563543));
#69429=CARTESIAN_POINT('Ctrl Pts',(100.190833057555,808.116978949041,117.499193047242));
#69430=CARTESIAN_POINT('Ctrl Pts',(100.171253520251,808.054774981796,117.477817897587));
#69431=CARTESIAN_POINT('Ctrl Pts',(100.145240424235,807.995072722745,117.456717099161));
#69432=CARTESIAN_POINT('Ctrl Pts',(99.2004494076673,808.721073021462,119.632469552402));
#69433=CARTESIAN_POINT('Ctrl Pts',(99.200586744741,808.721070527098,119.632476609914));
#69434=CARTESIAN_POINT('Ctrl Pts',(99.200724083128,808.721068006178,119.632483659442));
#69435=CARTESIAN_POINT('Ctrl Pts',(99.2008614228201,808.7210654587,119.632490700987));
#69436=CARTESIAN_POINT('Ctrl Pts',(99.33388906559,808.71859796325,119.639311162565));
#69437=CARTESIAN_POINT('Ctrl Pts',(99.4655696532678,808.691255145031,119.63853277349));
#69438=CARTESIAN_POINT('Ctrl Pts',(99.712247169163,808.589609722891,119.622079579624));
#69439=CARTESIAN_POINT('Ctrl Pts',(99.8247810219441,808.515978218443,119.606464544674));
#69440=CARTESIAN_POINT('Ctrl Pts',(100.014384327843,808.332222414994,119.562047452818));
#69441=CARTESIAN_POINT('Ctrl Pts',(100.089785827074,808.22393248243,119.533688885553));
#69442=CARTESIAN_POINT('Ctrl Pts',(100.193249467711,807.987145590484,119.467265048762));
#69443=CARTESIAN_POINT('Ctrl Pts',(100.220519811164,807.860970612968,119.429851256551));
#69444=CARTESIAN_POINT('Ctrl Pts',(100.223098984371,807.607013193112,119.35006909109));
#69445=CARTESIAN_POINT('Ctrl Pts',(100.198405529581,807.481713981814,119.308472097133));
#69446=CARTESIAN_POINT('Ctrl Pts',(100.099517844319,807.248088427224,119.226081439652));
#69447=CARTESIAN_POINT('Ctrl Pts',(100.026095080398,807.142182897061,119.18611795792));
#69448=CARTESIAN_POINT('Ctrl Pts',(99.8393587726141,806.964053277967,119.113389542738));
#69449=CARTESIAN_POINT('Ctrl Pts',(99.7276750239694,806.893805083307,119.08140358225));
#69450=CARTESIAN_POINT('Ctrl Pts',(99.4807845745175,806.799011735487,119.030587569192));
#69451=CARTESIAN_POINT('Ctrl Pts',(99.3479058494294,806.775507972555,119.012302017345));
#69452=CARTESIAN_POINT('Ctrl Pts',(99.2090987505836,806.777196046337,119.002233713168));
#69453=CARTESIAN_POINT('Ctrl Pts',(99.2047734549445,806.77727464753,119.001928920805));
#69454=CARTESIAN_POINT('Ctrl Pts',(99.2004494076648,806.777379182049,119.001633152524));
#69455=CARTESIAN_POINT('Origin',(99.2004494076648,811.368542512753,109.076615819925));
#69456=CARTESIAN_POINT('',(99.2004494076648,809.705125881246,115.283511063413));
#69457=CARTESIAN_POINT('Origin',(99.2004494076648,809.233703650638,115.116894496146));
#69458=CARTESIAN_POINT('',(99.200449407665,808.225611598495,119.469624934516));
#69459=CARTESIAN_POINT('',(99.2004494076648,811.839964743362,109.243232387192));
#69460=CARTESIAN_POINT('Ctrl Pts',(99.2004115835223,807.274154639319,119.160759867218));
#69461=CARTESIAN_POINT('Ctrl Pts',(99.1397213644481,807.275531840299,119.156877014434));
#69462=CARTESIAN_POINT('Ctrl Pts',(99.0795379805894,807.287376987541,119.156535673506));
#69463=CARTESIAN_POINT('Ctrl Pts',(98.960417403472,807.332987270617,119.163351434566));
#69464=CARTESIAN_POINT('Ctrl Pts',(98.9033819848119,807.36837213651,119.171194805266));
#69465=CARTESIAN_POINT('Ctrl Pts',(98.8070984504213,807.457722147422,119.194382736858));
#69466=CARTESIAN_POINT('Ctrl Pts',(98.7686928520005,807.510685755188,119.209447504984));
#69467=CARTESIAN_POINT('Ctrl Pts',(98.7156373230637,807.627269030948,119.244647843334));
#69468=CARTESIAN_POINT('Ctrl Pts',(98.7014746143982,807.689707769768,119.264418740293));
#69469=CARTESIAN_POINT('Ctrl Pts',(98.6995305723522,807.815826186176,119.305877483558));
#69470=CARTESIAN_POINT('Ctrl Pts',(98.7117934003778,807.878240954595,119.327147245798));
#69471=CARTESIAN_POINT('Ctrl Pts',(98.7613718581357,807.99444038258,119.368183710536));
#69472=CARTESIAN_POINT('Ctrl Pts',(98.798189395984,808.047056399957,119.387537685907));
#69473=CARTESIAN_POINT('Ctrl Pts',(98.8915121173824,808.135102119885,119.421708911796));
#69474=CARTESIAN_POINT('Ctrl Pts',(98.9470626901652,808.169663840158,119.436190961412));
#69475=CARTESIAN_POINT('Ctrl Pts',(99.069580924823,808.215889230352,119.458476424783));
#69476=CARTESIAN_POINT('Ctrl Pts',(99.1353408400831,808.227049587905,119.466049692863));
#69477=CARTESIAN_POINT('Ctrl Pts',(99.2684764061568,808.224112205193,119.473361392877));
#69478=CARTESIAN_POINT('Ctrl Pts',(99.3345258202417,808.209884026469,119.472979998211));
#69479=CARTESIAN_POINT('Ctrl Pts',(99.4562573321618,808.158095773898,119.464319915616));
#69480=CARTESIAN_POINT('Ctrl Pts',(99.5109465614735,808.121458069389,119.456266835239));
#69481=CARTESIAN_POINT('Ctrl Pts',(99.6027239678335,808.03054605062,119.433507669961));
#69482=CARTESIAN_POINT('Ctrl Pts',(99.6389928983616,807.977181748975,119.419032476278));
#69483=CARTESIAN_POINT('Ctrl Pts',(99.6881807593334,807.860770555768,119.385380213024));
#69484=CARTESIAN_POINT('Ctrl Pts',(99.7007016654658,807.798867500261,119.366535657893));
#69485=CARTESIAN_POINT('Ctrl Pts',(99.7001896061441,807.674552715984,119.326735277047));
#69486=CARTESIAN_POINT('Ctrl Pts',(99.6871769384752,807.613355970545,119.306166858106));
#69487=CARTESIAN_POINT('Ctrl Pts',(99.6370076919849,807.499627299614,119.26588784107));
#69488=CARTESIAN_POINT('Ctrl Pts',(99.6002835803374,807.448247335238,119.246579276215));
#69489=CARTESIAN_POINT('Ctrl Pts',(99.507633262563,807.362223910903,119.211861011593));
#69490=CARTESIAN_POINT('Ctrl Pts',(99.4525465553774,807.32849823702,119.196813179721));
#69491=CARTESIAN_POINT('Ctrl Pts',(99.3312150161737,807.283471426747,119.173239863295));
#69492=CARTESIAN_POINT('Ctrl Pts',(99.2661202392978,807.272663558442,119.1649637907));
#69493=CARTESIAN_POINT('Ctrl Pts',(99.2004115835223,807.274154639319,119.160759867218));
#69494=CARTESIAN_POINT('Origin',(104.959166694129,815.085695867571,110.390383588546));
#69495=CARTESIAN_POINT('',(104.959166694129,810.388915181948,120.834270597794));
#69496=CARTESIAN_POINT('',(104.959166694201,812.206764196253,121.381095048935));
#69497=CARTESIAN_POINT('Ctrl Pts',(104.959166694129,810.388915181948,120.834270597794));
#69498=CARTESIAN_POINT('Ctrl Pts',(104.833354697547,810.396090006485,120.813970264862));
#69499=CARTESIAN_POINT('Ctrl Pts',(104.708759033778,810.427066256375,120.801480936088));
#69500=CARTESIAN_POINT('Ctrl Pts',(104.477220223402,810.532733747189,120.793740466415));
#69501=CARTESIAN_POINT('Ctrl Pts',(104.372257408679,810.606238567556,120.798463261266));
#69502=CARTESIAN_POINT('Ctrl Pts',(104.196557349567,810.786119026573,120.824322727236));
#69503=CARTESIAN_POINT('Ctrl Pts',(104.127207777786,810.890491609221,120.845060648666));
#69504=CARTESIAN_POINT('Ctrl Pts',(104.034135082436,811.115448129756,120.899100248007));
#69505=CARTESIAN_POINT('Ctrl Pts',(104.010557106957,811.233486460713,120.931626595927));
#69506=CARTESIAN_POINT('Ctrl Pts',(104.011622017921,811.469001588448,121.003997677175));
#69507=CARTESIAN_POINT('Ctrl Pts',(104.035980782298,811.584079574372,121.043055246401));
#69508=CARTESIAN_POINT('Ctrl Pts',(104.13038978535,811.79822607484,121.123250107242));
#69509=CARTESIAN_POINT('Ctrl Pts',(104.200081347412,811.894788176856,121.16356608195));
#69510=CARTESIAN_POINT('Ctrl Pts',(104.376274369614,812.055146075277,121.240129540311));
#69511=CARTESIAN_POINT('Ctrl Pts',(104.481238947464,812.116971344385,121.275548912842));
#69512=CARTESIAN_POINT('Ctrl Pts',(104.71173856663,812.196511893003,121.336909024889));
#69513=CARTESIAN_POINT('Ctrl Pts',(104.835002671733,812.213423877213,121.362252254993));
#69514=CARTESIAN_POINT('Ctrl Pts',(104.959166694272,812.206764196252,121.381095048935));
#69515=CARTESIAN_POINT('',(104.959166694129,812.870928637576,119.501918880835));
#69516=CARTESIAN_POINT('',(104.959166694129,815.979592040189,110.706316741682));
#69517=CARTESIAN_POINT('Ctrl Pts',(105.86981055157,811.673894817626,119.252032293924));
#69518=CARTESIAN_POINT('Ctrl Pts',(105.836865720135,811.566669685013,119.214135304005));
#69519=CARTESIAN_POINT('Ctrl Pts',(105.782932986183,811.467334710957,119.175679186124));
#69520=CARTESIAN_POINT('Ctrl Pts',(105.634790270708,811.289777808233,119.099646624304));
#69521=CARTESIAN_POINT('Ctrl Pts',(105.540034158333,811.21487478293,119.063027998075));
#69522=CARTESIAN_POINT('Ctrl Pts',(105.326166148304,811.106713071755,118.999594175106));
#69523=CARTESIAN_POINT('Ctrl Pts',(105.209506808175,811.073770892273,118.973221755938));
#69524=CARTESIAN_POINT('Ctrl Pts',(104.965911156416,811.052227491311,118.933373508499));
#69525=CARTESIAN_POINT('Ctrl Pts',(104.841065703891,811.064539707011,118.920479968192));
#69526=CARTESIAN_POINT('Ctrl Pts',(104.599871368744,811.134372823572,118.910569084063));
#69527=CARTESIAN_POINT('Ctrl Pts',(104.485877614143,811.191802834625,118.913842207101));
#69528=CARTESIAN_POINT('Ctrl Pts',(104.285663872071,811.344996893095,118.936530971902));
#69529=CARTESIAN_POINT('Ctrl Pts',(104.201438262591,811.439378660212,118.955762249989));
#69530=CARTESIAN_POINT('Ctrl Pts',(104.077811776079,811.648352401452,119.00646773496));
#69531=CARTESIAN_POINT('Ctrl Pts',(104.037821614021,811.7599909238,119.036915891242));
#69532=CARTESIAN_POINT('Ctrl Pts',(104.004044502348,811.986384458144,119.104464798348));
#69533=CARTESIAN_POINT('Ctrl Pts',(104.009078903378,812.098885079567,119.140702474712));
#69534=CARTESIAN_POINT('Ctrl Pts',(104.062205351414,812.315489543703,119.215652388806));
#69535=CARTESIAN_POINT('Ctrl Pts',(104.110048821356,812.417554494439,119.253688298738));
#69536=CARTESIAN_POINT('Ctrl Pts',(104.244908190584,812.600501697837,119.32779948993));
#69537=CARTESIAN_POINT('Ctrl Pts',(104.331628162827,812.678994933161,119.363087975246));
#69538=CARTESIAN_POINT('Ctrl Pts',(104.537599155287,812.802458436634,119.427290432846));
#69539=CARTESIAN_POINT('Ctrl Pts',(104.656186177563,812.84417141477,119.45511499733));
#69540=CARTESIAN_POINT('Ctrl Pts',(104.90225023298,812.879338180881,119.497207229687));
#69541=CARTESIAN_POINT('Ctrl Pts',(105.027143201732,812.87352862247,119.511375173558));
#69542=CARTESIAN_POINT('Ctrl Pts',(105.271042167254,812.816004758216,119.525164598919));
#69543=CARTESIAN_POINT('Ctrl Pts',(105.38767625621,812.764190374834,119.524454708563));
#69544=CARTESIAN_POINT('Ctrl Pts',(105.596049828579,812.620213474278,119.507648827693));
#69545=CARTESIAN_POINT('Ctrl Pts',(105.685585908109,812.529050176458,119.491567699377));
#69546=CARTESIAN_POINT('Ctrl Pts',(105.816395499718,812.330541934538,119.448030974393));
#69547=CARTESIAN_POINT('Ctrl Pts',(105.860678531356,812.227445189219,119.422272871814));
#69548=CARTESIAN_POINT('Ctrl Pts',(105.910836328957,812.007083146204,119.361042839447));
#69549=CARTESIAN_POINT('Ctrl Pts',(105.914194759803,811.891429049704,119.325715182053));
#69550=CARTESIAN_POINT('Ctrl Pts',(105.888782435894,811.743519795637,119.276294798763));
#69551=CARTESIAN_POINT('Ctrl Pts',(105.880402800986,811.708369279896,119.264216735362));
#69552=CARTESIAN_POINT('Ctrl Pts',(105.86981055157,811.673894817626,119.252032293924));
#69553=CARTESIAN_POINT('Ctrl Pts',(104.959166694272,812.206764196252,121.381095048935));
#69554=CARTESIAN_POINT('Ctrl Pts',(104.95976504612,812.206732102959,121.381185853182));
#69555=CARTESIAN_POINT('Ctrl Pts',(104.960363418914,812.206699462338,121.381276506184));
#69556=CARTESIAN_POINT('Ctrl Pts',(104.960961811862,812.206666274312,121.381367007803));
#69557=CARTESIAN_POINT('Ctrl Pts',(104.961270619604,812.20664914724,121.381413712231));
#69558=CARTESIAN_POINT('Ctrl Pts',(104.961579425527,812.20663187478,121.381460375256));
#69559=CARTESIAN_POINT('Ctrl Pts',(105.08829317379,812.199484690219,121.400590952754));
#69560=CARTESIAN_POINT('Ctrl Pts',(105.213220126502,812.168057685697,121.412579751966));
#69561=CARTESIAN_POINT('Ctrl Pts',(105.444394943492,812.061069588652,121.421057355886));
#69562=CARTESIAN_POINT('Ctrl Pts',(105.548796916412,811.986861848353,121.417613934371));
#69563=CARTESIAN_POINT('Ctrl Pts',(105.722606586098,811.80646593797,121.395560660536));
#69564=CARTESIAN_POINT('Ctrl Pts',(105.791053424735,811.702422734513,121.377392055017));
#69565=CARTESIAN_POINT('Ctrl Pts',(105.883424042089,811.478434068685,121.328333330863));
#69566=CARTESIAN_POINT('Ctrl Pts',(105.907181000798,811.360909031746,121.298113580969));
#69567=CARTESIAN_POINT('Ctrl Pts',(105.907320692346,811.126329823532,121.22882367717));
#69568=CARTESIAN_POINT('Ctrl Pts',(105.883889697256,811.011729202174,121.190508316358));
#69569=CARTESIAN_POINT('Ctrl Pts',(105.79189616721,810.798781561893,121.11002111123));
#69570=CARTESIAN_POINT('Ctrl Pts',(105.723811054966,810.702972235351,121.068691777476));
#69571=CARTESIAN_POINT('Ctrl Pts',(105.550353727072,810.542693327016,120.988421443388));
#69572=CARTESIAN_POINT('Ctrl Pts',(105.44611494346,810.480561578632,120.95039969055));
#69573=CARTESIAN_POINT('Ctrl Pts',(105.214531673714,810.399358552366,120.883442085345));
#69574=CARTESIAN_POINT('Ctrl Pts',(105.089028914393,810.381929682426,120.855358187615));
#69575=CARTESIAN_POINT('Ctrl Pts',(104.961339507698,810.388793050608,120.834621757548));
#69576=CARTESIAN_POINT('Ctrl Pts',(104.960253055459,810.388853228779,120.834445887092));
#69577=CARTESIAN_POINT('Ctrl Pts',(104.959166694129,810.388915181948,120.834270597794));
#69578=CARTESIAN_POINT('Origin',(104.959166694129,815.085695867571,110.390383588546));
#69579=CARTESIAN_POINT('',(104.959166694129,813.422279236064,116.597278832034));
#69580=CARTESIAN_POINT('Origin',(104.959166694129,812.950857005456,116.430662264767));
#69581=CARTESIAN_POINT('',(104.95916669413,811.777693521472,121.250443152468));
#69582=CARTESIAN_POINT('',(104.959166694129,815.557118098179,110.557000155813));
#69583=CARTESIAN_POINT('Ctrl Pts',(104.959670529459,810.818979506244,120.962111840113));
#69584=CARTESIAN_POINT('Ctrl Pts',(104.894942761524,810.822555013975,120.951799624401));
#69585=CARTESIAN_POINT('Ctrl Pts',(104.830824769369,810.838109254016,120.945314369594));
#69586=CARTESIAN_POINT('Ctrl Pts',(104.709436333555,810.892082012198,120.940681817555));
#69587=CARTESIAN_POINT('Ctrl Pts',(104.653463593158,810.930579058416,120.942788160454));
#69588=CARTESIAN_POINT('Ctrl Pts',(104.559429700388,811.025385114038,120.955629050457));
#69589=CARTESIAN_POINT('Ctrl Pts',(104.522160656818,811.080687145236,120.96618812564));
#69590=CARTESIAN_POINT('Ctrl Pts',(104.472191438664,811.199560019998,120.993985714608));
#69591=CARTESIAN_POINT('Ctrl Pts',(104.459349743312,811.261703340205,121.010761381756));
#69592=CARTESIAN_POINT('Ctrl Pts',(104.458988517942,811.385844599149,121.048419577696));
#69593=CARTESIAN_POINT('Ctrl Pts',(104.471338074762,811.446569770682,121.068891947692));
#69594=CARTESIAN_POINT('Ctrl Pts',(104.519900222239,811.559184108116,121.111032659457));
#69595=CARTESIAN_POINT('Ctrl Pts',(104.555717462033,811.609852674374,121.13226633793));
#69596=CARTESIAN_POINT('Ctrl Pts',(104.647365244939,811.695210236629,121.173222002652));
#69597=CARTESIAN_POINT('Ctrl Pts',(104.702733253995,811.72852066068,121.192454311888));
#69598=CARTESIAN_POINT('Ctrl Pts',(104.824904954755,811.771734163302,121.225910966599));
#69599=CARTESIAN_POINT('Ctrl Pts',(104.890536365835,811.781112203955,121.239785223859));
#69600=CARTESIAN_POINT('Ctrl Pts',(105.023429752435,811.774503425035,121.260426083977));
#69601=CARTESIAN_POINT('Ctrl Pts',(105.089467976359,811.758385156089,121.266948375166));
#69602=CARTESIAN_POINT('Ctrl Pts',(105.212859326362,811.70237139337,121.271621923929));
#69603=CARTESIAN_POINT('Ctrl Pts',(105.269039177046,811.662833636879,121.269677039047));
#69604=CARTESIAN_POINT('Ctrl Pts',(105.36163070635,811.567034614157,121.257482410398));
#69605=CARTESIAN_POINT('Ctrl Pts',(105.397798846797,811.512211077012,121.247609667748));
#69606=CARTESIAN_POINT('Ctrl Pts',(105.446628074815,811.394067836774,121.221177016886));
#69607=CARTESIAN_POINT('Ctrl Pts',(105.459169310893,811.332025327319,121.204972130901));
#69608=CARTESIAN_POINT('Ctrl Pts',(105.459164088117,811.208186328606,121.168069472528));
#69609=CARTESIAN_POINT('Ctrl Pts',(105.446725523884,811.147677185787,121.147773275748));
#69610=CARTESIAN_POINT('Ctrl Pts',(105.398035971004,811.035343098214,121.105407009963));
#69611=CARTESIAN_POINT('Ctrl Pts',(105.362081549874,810.984819644039,121.08377943449));
#69612=CARTESIAN_POINT('Ctrl Pts',(105.270614628522,810.900339483112,121.041960105072));
#69613=CARTESIAN_POINT('Ctrl Pts',(105.215732219555,810.867574479576,121.022241947609));
#69614=CARTESIAN_POINT('Ctrl Pts',(105.0933620194,810.824512770352,120.987420522973));
#69615=CARTESIAN_POINT('Ctrl Pts',(105.02679190406,810.815271777684,120.972805397389));
#69616=CARTESIAN_POINT('Ctrl Pts',(104.959670529459,810.818979506244,120.962111840113));
#69617=CARTESIAN_POINT('Origin',(94.2316464454274,802.680033537841,106.005802765141));
#69618=CARTESIAN_POINT('',(94.2316464454273,798.084680646679,115.94267397259));
#69619=CARTESIAN_POINT('',(94.2316464454283,800.036659745791,116.550068192181));
#69620=CARTESIAN_POINT('Ctrl Pts',(94.2316464454273,798.084680646679,115.94267397259));
#69621=CARTESIAN_POINT('Ctrl Pts',(94.1037999764411,798.087573511576,115.934488947264));
#69622=CARTESIAN_POINT('Ctrl Pts',(93.9770394345588,798.113304203478,115.933720303641));
#69623=CARTESIAN_POINT('Ctrl Pts',(93.7310611758891,798.210787294472,115.94805993517));
#69624=CARTESIAN_POINT('Ctrl Pts',(93.6153702918267,798.284480283536,115.964086371598));
#69625=CARTESIAN_POINT('Ctrl Pts',(93.4215142720861,798.468719806565,116.011286173827));
#69626=CARTESIAN_POINT('Ctrl Pts',(93.344747526796,798.576953819916,116.041784848021));
#69627=CARTESIAN_POINT('Ctrl Pts',(93.2393598302505,798.814238392117,116.112803621196));
#69628=CARTESIAN_POINT('Ctrl Pts',(93.2115917482419,798.940881351409,116.152571621789));
#69629=CARTESIAN_POINT('Ctrl Pts',(93.208974616995,799.197042906534,116.23565830297));
#69630=CARTESIAN_POINT('Ctrl Pts',(93.2344173963583,799.324033750943,116.27814988591));
#69631=CARTESIAN_POINT('Ctrl Pts',(93.3361029824329,799.561135843543,116.359462776658));
#69632=CARTESIAN_POINT('Ctrl Pts',(93.411528378302,799.668818063266,116.39744946001));
#69633=CARTESIAN_POINT('Ctrl Pts',(93.6022010781517,799.849092800142,116.463350069855));
#69634=CARTESIAN_POINT('Ctrl Pts',(93.715421127415,799.920017866629,116.490653651625));
#69635=CARTESIAN_POINT('Ctrl Pts',(93.9641490083928,800.015112070195,116.531380470685));
#69636=CARTESIAN_POINT('Ctrl Pts',(94.0970897622964,800.038582583248,116.54449292373));
#69637=CARTESIAN_POINT('Ctrl Pts',(94.2313049710666,800.036664680118,116.550054059785));
#69638=CARTESIAN_POINT('Ctrl Pts',(94.2314187968175,800.036663053575,116.550058776095));
#69639=CARTESIAN_POINT('Ctrl Pts',(94.2315326216066,800.036661408799,116.550063486893));
#69640=CARTESIAN_POINT('Ctrl Pts',(94.2316464454292,800.036659745791,116.550068192181));
#69641=CARTESIAN_POINT('',(94.2316464463135,800.674576417418,114.745157040706));
#69642=CARTESIAN_POINT('',(94.2316464454274,803.643062678083,106.346169848208));
#69643=CARTESIAN_POINT('Ctrl Pts',(95.0750947698766,799.129354690295,114.323272367424));
#69644=CARTESIAN_POINT('Ctrl Pts',(94.9999801103154,799.025664094407,114.286624602379));
#69645=CARTESIAN_POINT('Ctrl Pts',(94.9040983621953,798.937575318805,114.253174138367));
#69646=CARTESIAN_POINT('Ctrl Pts',(94.6816501975664,798.802427106374,114.19655656175));
#69647=CARTESIAN_POINT('Ctrl Pts',(94.5572529690001,798.756685541673,114.173947365479));
#69648=CARTESIAN_POINT('Ctrl Pts',(94.2956029478729,798.71366877426,114.142891306016));
#69649=CARTESIAN_POINT('Ctrl Pts',(94.160808745891,798.71701742042,114.1348129979));
#69650=CARTESIAN_POINT('Ctrl Pts',(93.8985671797012,798.773026664621,114.134843841723));
#69651=CARTESIAN_POINT('Ctrl Pts',(93.773651395262,798.825366769294,114.143029676665));
#69652=CARTESIAN_POINT('Ctrl Pts',(93.5509549700396,798.972628891492,114.174981268742));
#69653=CARTESIAN_POINT('Ctrl Pts',(93.4553333029572,799.066187929153,114.198459027646));
#69654=CARTESIAN_POINT('Ctrl Pts',(93.3073869494175,799.281452184646,114.25733136225));
#69655=CARTESIAN_POINT('Ctrl Pts',(93.2560708615511,799.400835692059,114.292045286953));
#69656=CARTESIAN_POINT('Ctrl Pts',(93.2036138968648,799.652445029388,114.368568138269));
#69657=CARTESIAN_POINT('Ctrl Pts',(93.2036404280434,799.78232989443,114.409696103859));
#69658=CARTESIAN_POINT('Ctrl Pts',(93.2566767393386,800.033976221112,114.492145534065));
#69659=CARTESIAN_POINT('Ctrl Pts',(93.309242308972,800.153217174935,114.53263784761));
#69660=CARTESIAN_POINT('Ctrl Pts',(93.4596053190206,800.363477914753,114.606854936056));
#69661=CARTESIAN_POINT('Ctrl Pts',(93.5554781799771,800.452708687867,114.639916854467));
#69662=CARTESIAN_POINT('Ctrl Pts',(93.7783253164892,800.590173152952,114.694682481267));
#69663=CARTESIAN_POINT('Ctrl Pts',(93.9031003564464,800.637094044925,114.715866811105));
#69664=CARTESIAN_POINT('Ctrl Pts',(94.1647863873439,800.681921004229,114.743786234978));
#69665=CARTESIAN_POINT('Ctrl Pts',(94.2991296737661,800.679556797199,114.750309276137));
#69666=CARTESIAN_POINT('Ctrl Pts',(94.5612273327101,800.625389157071,114.748167692582));
#69667=CARTESIAN_POINT('Ctrl Pts',(94.6863763841176,800.573693442765,114.739401603949));
#69668=CARTESIAN_POINT('Ctrl Pts',(94.9108287656632,800.426386781562,114.707470098182));
#69669=CARTESIAN_POINT('Ctrl Pts',(95.0076133951727,800.331702868478,114.684447152005));
#69670=CARTESIAN_POINT('Ctrl Pts',(95.1568347418816,800.11346636752,114.62732663394));
#69671=CARTESIAN_POINT('Ctrl Pts',(95.2083193779351,799.992322807333,114.593890746079));
#69672=CARTESIAN_POINT('Ctrl Pts',(95.2598098406563,799.738905820011,114.520468979456));
#69673=CARTESIAN_POINT('Ctrl Pts',(95.2593809405527,799.609100770489,114.481193539207));
#69674=CARTESIAN_POINT('Ctrl Pts',(95.2193123245112,799.420373405143,114.421355995634));
#69675=CARTESIAN_POINT('Ctrl Pts',(95.1993311927414,799.358707089507,114.401327504981));
#69676=CARTESIAN_POINT('Ctrl Pts',(95.1465310394155,799.239663709715,114.361649470194));
#69677=CARTESIAN_POINT('Ctrl Pts',(95.1137046827979,799.182653006514,114.34210979577));
#69678=CARTESIAN_POINT('Ctrl Pts',(95.0750947698766,799.129354690295,114.323272367424));
#69679=CARTESIAN_POINT('Ctrl Pts',(94.2316464454292,800.036659745791,116.550068192181));
#69680=CARTESIAN_POINT('Ctrl Pts',(94.3629815577469,800.03474089155,116.555497367452));
#69681=CARTESIAN_POINT('Ctrl Pts',(94.4930290911779,800.008544361815,116.553607102351));
#69682=CARTESIAN_POINT('Ctrl Pts',(94.7387571810064,799.909432676774,116.535734906483));
#69683=CARTESIAN_POINT('Ctrl Pts',(94.8517243323247,799.836549716512,116.519650101181));
#69684=CARTESIAN_POINT('Ctrl Pts',(95.0425762648668,799.653547815694,116.475207272092));
#69685=CARTESIAN_POINT('Ctrl Pts',(95.1186759198018,799.54518290088,116.447268899553));
#69686=CARTESIAN_POINT('Ctrl Pts',(95.2234050866694,799.30761221254,116.382725886987));
#69687=CARTESIAN_POINT('Ctrl Pts',(95.2512304695178,799.180719506938,116.346745494667));
#69688=CARTESIAN_POINT('Ctrl Pts',(95.2547001758982,798.9252096553,116.2707184679));
#69689=CARTESIAN_POINT('Ctrl Pts',(95.2304713001988,798.799051363495,116.231399994923));
#69690=CARTESIAN_POINT('Ctrl Pts',(95.1325932139514,798.563756070618,116.153912952651));
#69691=CARTESIAN_POINT('Ctrl Pts',(95.0598469876302,798.456974144627,116.116507492673));
#69692=CARTESIAN_POINT('Ctrl Pts',(94.8745204754859,798.276892259145,116.048434832477));
#69693=CARTESIAN_POINT('Ctrl Pts',(94.7635953773627,798.205571730331,116.018490318587));
#69694=CARTESIAN_POINT('Ctrl Pts',(94.51783746284,798.108448470284,115.970676477465));
#69695=CARTESIAN_POINT('Ctrl Pts',(94.3853136008111,798.083809800227,115.953347247582));
#69696=CARTESIAN_POINT('Ctrl Pts',(94.244581197857,798.084446452881,115.943520848752));
#69697=CARTESIAN_POINT('Ctrl Pts',(94.2381124317385,798.084534336617,115.943087939922));
#69698=CARTESIAN_POINT('Ctrl Pts',(94.2316464454274,798.084680646679,115.94267397259));
#69699=CARTESIAN_POINT('Origin',(94.2316464454274,802.680033537841,106.005802765141));
#69700=CARTESIAN_POINT('',(94.2316464454274,801.016616906335,112.212698008629));
#69701=CARTESIAN_POINT('Origin',(94.2316464454274,800.545194675726,112.046081441362));
#69702=CARTESIAN_POINT('',(94.2316464454273,799.539662874025,116.391567948387));
#69703=CARTESIAN_POINT('',(94.2316464454274,803.15145576845,106.172419332408));
#69704=CARTESIAN_POINT('Ctrl Pts',(94.2315455714384,798.584150826436,116.094176309146));
#69705=CARTESIAN_POINT('Ctrl Pts',(94.1720167839962,798.585389073316,116.090708873649));
#69706=CARTESIAN_POINT('Ctrl Pts',(94.1129792196732,798.59675826626,116.090478889328));
#69707=CARTESIAN_POINT('Ctrl Pts',(93.9946726488584,798.641170624584,116.096978630705));
#69708=CARTESIAN_POINT('Ctrl Pts',(93.9374123628351,798.676241270424,116.104496291945));
#69709=CARTESIAN_POINT('Ctrl Pts',(93.8405508411949,798.765138501411,116.12675935922));
#69710=CARTESIAN_POINT('Ctrl Pts',(93.8017859963506,798.817969151388,116.141237585891));
#69711=CARTESIAN_POINT('Ctrl Pts',(93.747874153489,798.934517249859,116.175145732248));
#69712=CARTESIAN_POINT('Ctrl Pts',(93.7332320968561,798.997065630691,116.194229136661));
#69713=CARTESIAN_POINT('Ctrl Pts',(93.7302997148241,799.123771859812,116.234338289418));
#69714=CARTESIAN_POINT('Ctrl Pts',(93.7421239774015,799.186659370225,116.254961776196));
#69715=CARTESIAN_POINT('Ctrl Pts',(93.7910594266082,799.304088700895,116.294762786258));
#69716=CARTESIAN_POINT('Ctrl Pts',(93.8277332777928,799.357420213033,116.313531040647));
#69717=CARTESIAN_POINT('Ctrl Pts',(93.9210127782908,799.44679212484,116.346498174468));
#69718=CARTESIAN_POINT('Ctrl Pts',(93.976636914046,799.481962276886,116.360374414023));
#69719=CARTESIAN_POINT('Ctrl Pts',(94.0991749479439,799.529119031612,116.381413843585));
#69720=CARTESIAN_POINT('Ctrl Pts',(94.1648222621132,799.540710146109,116.388393061611));
#69721=CARTESIAN_POINT('Ctrl Pts',(94.2974551609734,799.53863205019,116.39469475252));
#69722=CARTESIAN_POINT('Ctrl Pts',(94.3631216359456,799.524965765282,116.393953466352));
#69723=CARTESIAN_POINT('Ctrl Pts',(94.4858428735472,799.473824363662,116.384887449622));
#69724=CARTESIAN_POINT('Ctrl Pts',(94.5416225021999,799.436709724106,116.376607261033));
#69725=CARTESIAN_POINT('Ctrl Pts',(94.6342417498175,799.344776383757,116.353764068761));
#69726=CARTESIAN_POINT('Ctrl Pts',(94.6705215309892,799.291157621273,116.339530351243));
#69727=CARTESIAN_POINT('Ctrl Pts',(94.7196172889772,799.174109948565,116.306774352671));
#69728=CARTESIAN_POINT('Ctrl Pts',(94.7320397422235,799.111825090876,116.288573175419));
#69729=CARTESIAN_POINT('Ctrl Pts',(94.731235177814,798.986812617055,116.250406160606));
#69730=CARTESIAN_POINT('Ctrl Pts',(94.7180796550034,798.925294694194,116.230810008027));
#69731=CARTESIAN_POINT('Ctrl Pts',(94.6676781540853,798.811053796892,116.192631015984));
#69732=CARTESIAN_POINT('Ctrl Pts',(94.6309178831475,798.75946002571,116.174423147786));
#69733=CARTESIAN_POINT('Ctrl Pts',(94.5383015328304,798.67305163928,116.141785703591));
#69734=CARTESIAN_POINT('Ctrl Pts',(94.4833043525867,798.639145479472,116.127692793331));
#69735=CARTESIAN_POINT('Ctrl Pts',(94.3621547000017,798.593752761756,116.105678738551));
#69736=CARTESIAN_POINT('Ctrl Pts',(94.2971516425527,798.582786167145,116.097997734537));
#69737=CARTESIAN_POINT('Ctrl Pts',(94.2315455714384,798.584150826436,116.094176309146));
#69738=CARTESIAN_POINT('Origin',(100.684211372524,805.187086117687,106.891879975103));
#69739=CARTESIAN_POINT('',(100.684211372524,800.481296738109,117.361256037865));
#69740=CARTESIAN_POINT('',(100.684211372529,802.320089444705,117.848822743518));
#69741=CARTESIAN_POINT('Ctrl Pts',(100.684211372524,800.481296738109,117.361256037865));
#69742=CARTESIAN_POINT('Ctrl Pts',(100.565597463437,800.487609223464,117.34339559352));
#69743=CARTESIAN_POINT('Ctrl Pts',(100.448076354088,800.515369438104,117.331648409742));
#69744=CARTESIAN_POINT('Ctrl Pts',(100.219870360019,800.6139776104,117.321501328638));
#69745=CARTESIAN_POINT('Ctrl Pts',(100.112326389534,800.686724346148,117.324169705703));
#69746=CARTESIAN_POINT('Ctrl Pts',(99.9321222227121,800.866182147369,117.344893473142));
#69747=CARTESIAN_POINT('Ctrl Pts',(99.8606366181137,800.970741458563,117.362530678582));
#69748=CARTESIAN_POINT('Ctrl Pts',(99.7628167677313,801.198311150468,117.410042766362));
#69749=CARTESIAN_POINT('Ctrl Pts',(99.7370892623527,801.318928499893,117.439338383031));
#69750=CARTESIAN_POINT('Ctrl Pts',(99.7352187437462,801.561038000097,117.505395977054));
#69751=CARTESIAN_POINT('Ctrl Pts',(99.7590399517933,801.680005233789,117.541448176051));
#69752=CARTESIAN_POINT('Ctrl Pts',(99.8537940863741,801.900197902703,117.615189173687));
#69753=CARTESIAN_POINT('Ctrl Pts',(99.9237276110613,801.999066864586,117.652087516984));
#69754=CARTESIAN_POINT('Ctrl Pts',(100.100456009115,802.162851115463,117.721750207133));
#69755=CARTESIAN_POINT('Ctrl Pts',(100.205366872227,802.226036346363,117.753785216086));
#69756=CARTESIAN_POINT('Ctrl Pts',(100.436170978144,802.308107240893,117.809174515615));
#69757=CARTESIAN_POINT('Ctrl Pts',(100.559745617076,802.326050958506,117.83195533243));
#69758=CARTESIAN_POINT('Ctrl Pts',(100.684211372533,802.320089444705,117.848822743518));
#69759=CARTESIAN_POINT('',(100.684211372524,802.980040408452,115.981568120976));
#69760=CARTESIAN_POINT('',(100.684211372524,806.080982290306,107.207813128239));
#69761=CARTESIAN_POINT('Ctrl Pts',(101.520107801531,801.602208259166,115.69235748013));
#69762=CARTESIAN_POINT('Ctrl Pts',(101.464238104416,801.5037843751,115.657571149245));
#69763=CARTESIAN_POINT('Ctrl Pts',(101.389347097758,801.417215440319,115.623626981594));
#69764=CARTESIAN_POINT('Ctrl Pts',(101.204367694086,801.272669922271,115.559261760087));
#69765=CARTESIAN_POINT('Ctrl Pts',(101.094462060306,801.21804825099,115.529811250606));
#69766=CARTESIAN_POINT('Ctrl Pts',(100.859669924098,801.154347390131,115.482091396508));
#69767=CARTESIAN_POINT('Ctrl Pts',(100.737275106152,801.145094747659,115.464091661275));
#69768=CARTESIAN_POINT('Ctrl Pts',(100.492018677018,801.171995094994,115.44136507362));
#69769=CARTESIAN_POINT('Ctrl Pts',(100.371421636957,801.208629912145,115.437067963642));
#69770=CARTESIAN_POINT('Ctrl Pts',(100.148500593435,801.324455445357,115.443412355749));
#69771=CARTESIAN_POINT('Ctrl Pts',(100.048482560249,801.403093371002,115.454181073391));
#69772=CARTESIAN_POINT('Ctrl Pts',(99.884246300006,801.592403311696,115.489634412983));
#69773=CARTESIAN_POINT('Ctrl Pts',(99.8216951295365,801.70133020946,115.514006432386));
#69774=CARTESIAN_POINT('Ctrl Pts',(99.7452479949851,801.930130635538,115.571719338632));
#69775=CARTESIAN_POINT('Ctrl Pts',(99.7301255748518,802.047230646471,115.604097769774));
#69776=CARTESIAN_POINT('Ctrl Pts',(99.7461461285556,802.275383801483,115.672268586362));
#69777=CARTESIAN_POINT('Ctrl Pts',(99.775634488365,802.384463322736,115.707297130171));
#69778=CARTESIAN_POINT('Ctrl Pts',(99.8752533793037,802.585931190253,115.77689725886));
#69779=CARTESIAN_POINT('Ctrl Pts',(99.9446942266083,802.676373623328,115.810825377793));
#69780=CARTESIAN_POINT('Ctrl Pts',(100.117604090515,802.828821835627,115.874157193571));
#69781=CARTESIAN_POINT('Ctrl Pts',(100.220260819943,802.888548418159,115.902812908805));
#69782=CARTESIAN_POINT('Ctrl Pts',(100.450381346375,802.968796583903,115.951741603823));
#69783=CARTESIAN_POINT('Ctrl Pts',(100.57648165657,802.986261794649,115.970996186868));
#69784=CARTESIAN_POINT('Ctrl Pts',(100.826978585255,802.972220883698,115.995696761168));
#69785=CARTESIAN_POINT('Ctrl Pts',(100.948985103197,802.941944340169,116.001217244638));
#69786=CARTESIAN_POINT('Ctrl Pts',(101.177233354518,802.837632128631,115.998470084945));
#69787=CARTESIAN_POINT('Ctrl Pts',(101.281112435463,802.763965563543,115.990036894187));
#69788=CARTESIAN_POINT('Ctrl Pts',(101.455544622951,802.582053781247,115.959823542551));
#69789=CARTESIAN_POINT('Ctrl Pts',(101.52413938033,802.475220200409,115.938204005999));
#69790=CARTESIAN_POINT('Ctrl Pts',(101.610160860499,802.255224661463,115.887072943205));
#69791=CARTESIAN_POINT('Ctrl Pts',(101.631481712771,802.145626771598,115.859017116172));
#69792=CARTESIAN_POINT('Ctrl Pts',(101.633104022222,801.920133478107,115.795973526267));
#69793=CARTESIAN_POINT('Ctrl Pts',(101.611269969049,801.806310259357,115.761292963019));
#69794=CARTESIAN_POINT('Ctrl Pts',(101.553994557423,801.666595107358,115.714768652655));
#69795=CARTESIAN_POINT('Ctrl Pts',(101.538070733526,801.633852990164,115.70354179879));
#69796=CARTESIAN_POINT('Ctrl Pts',(101.520107801531,801.602208259166,115.69235748013));
#69797=CARTESIAN_POINT('Ctrl Pts',(100.684211372533,802.320089444705,117.848822743518));
#69798=CARTESIAN_POINT('Ctrl Pts',(100.684435662878,802.320078701911,117.848853139006));
#69799=CARTESIAN_POINT('Ctrl Pts',(100.68465995612,802.320067881495,117.848883515272));
#69800=CARTESIAN_POINT('Ctrl Pts',(100.684884252216,802.320056983452,117.848913872309));
#69801=CARTESIAN_POINT('Ctrl Pts',(100.802607848229,802.314337058754,117.864847005342));
#69802=CARTESIAN_POINT('Ctrl Pts',(100.919059102557,802.287333175311,117.87521746394));
#69803=CARTESIAN_POINT('Ctrl Pts',(101.147144227793,802.189808666365,117.884515701304));
#69804=CARTESIAN_POINT('Ctrl Pts',(101.255373087228,802.116609400356,117.882288300134));
#69805=CARTESIAN_POINT('Ctrl Pts',(101.435390440464,801.936613260541,117.864091786616));
#69806=CARTESIAN_POINT('Ctrl Pts',(101.506500565247,801.832286897255,117.848629204703));
#69807=CARTESIAN_POINT('Ctrl Pts',(101.603817387354,801.606453595449,117.806329558644));
#69808=CARTESIAN_POINT('Ctrl Pts',(101.629942246869,801.487327405553,117.780075013444));
#69809=CARTESIAN_POINT('Ctrl Pts',(101.634319351748,801.249250657437,117.719627397482));
#69810=CARTESIAN_POINT('Ctrl Pts',(101.613095827351,801.132674566714,117.686123284468));
#69811=CARTESIAN_POINT('Ctrl Pts',(101.525519281691,800.915574808855,117.615412566743));
#69812=CARTESIAN_POINT('Ctrl Pts',(101.459956708144,800.817438648366,117.578951020177));
#69813=CARTESIAN_POINT('Ctrl Pts',(101.291347353662,800.651683474917,117.507413567051));
#69814=CARTESIAN_POINT('Ctrl Pts',(101.189526852653,800.58641025219,117.473155863602));
#69815=CARTESIAN_POINT('Ctrl Pts',(100.962093260562,800.498315436644,117.411860821667));
#69816=CARTESIAN_POINT('Ctrl Pts',(100.838396201997,800.477202847779,117.385606217155));
#69817=CARTESIAN_POINT('Ctrl Pts',(100.703437945377,800.480414707131,117.364190083619));
#69818=CARTESIAN_POINT('Ctrl Pts',(100.693821067041,800.480785322067,117.362703030173));
#69819=CARTESIAN_POINT('Ctrl Pts',(100.684211372524,800.481296738109,117.361256037865));
#69820=CARTESIAN_POINT('Origin',(100.684211372524,805.187086117687,106.891879975103));
#69821=CARTESIAN_POINT('',(100.684211372524,803.523669486181,113.098775218591));
#69822=CARTESIAN_POINT('Origin',(100.684211372524,803.052247255572,112.932158651324));
#69823=CARTESIAN_POINT('',(100.684211372525,801.886384714253,117.731282369494));
#69824=CARTESIAN_POINT('',(100.684211372524,805.658508348296,107.05849654237));
#69825=CARTESIAN_POINT('Ctrl Pts',(100.68460553067,800.916635666742,117.47417310411));
#69826=CARTESIAN_POINT('Ctrl Pts',(100.621007780188,800.919891930241,117.464809433934));
#69827=CARTESIAN_POINT('Ctrl Pts',(100.558064699032,800.934856410941,117.458728634147));
#69828=CARTESIAN_POINT('Ctrl Pts',(100.437014956238,800.987800885012,117.453675701706));
#69829=CARTESIAN_POINT('Ctrl Pts',(100.380442230377,801.026501484678,117.455151425979));
#69830=CARTESIAN_POINT('Ctrl Pts',(100.285601512585,801.122037875001,117.466029264185));
#69831=CARTESIAN_POINT('Ctrl Pts',(100.248042152197,801.177825667902,117.475256698663));
#69832=CARTESIAN_POINT('Ctrl Pts',(100.197078508039,801.299145482615,117.500145751283));
#69833=CARTESIAN_POINT('Ctrl Pts',(100.184010548787,801.363408718905,117.515512547569));
#69834=CARTESIAN_POINT('Ctrl Pts',(100.184411022147,801.490348899504,117.549816644459));
#69835=CARTESIAN_POINT('Ctrl Pts',(100.19712771743,801.551744919999,117.568292146279));
#69836=CARTESIAN_POINT('Ctrl Pts',(100.246372778483,801.665394250182,117.606273737637));
#69837=CARTESIAN_POINT('Ctrl Pts',(100.282388052149,801.716469180971,117.625384893445));
#69838=CARTESIAN_POINT('Ctrl Pts',(100.374395891752,801.802641376072,117.662253270929));
#69839=CARTESIAN_POINT('Ctrl Pts',(100.429913984255,801.836325612348,117.679561067638));
#69840=CARTESIAN_POINT('Ctrl Pts',(100.552386419393,801.880116640256,117.709647845865));
#69841=CARTESIAN_POINT('Ctrl Pts',(100.618127726179,801.889650682728,117.722095834828));
#69842=CARTESIAN_POINT('Ctrl Pts',(100.751151899359,801.883076433634,117.740588031741));
#69843=CARTESIAN_POINT('Ctrl Pts',(100.817156319277,801.86680642142,117.74639924812));
#69844=CARTESIAN_POINT('Ctrl Pts',(100.940355474473,801.810232669805,117.750553218458));
#69845=CARTESIAN_POINT('Ctrl Pts',(100.996343911969,801.770249775246,117.748796216972));
#69846=CARTESIAN_POINT('Ctrl Pts',(101.088671570435,801.673147054687,117.737899059487));
#69847=CARTESIAN_POINT('Ctrl Pts',(101.1246722087,801.617342435969,117.729042799405));
#69848=CARTESIAN_POINT('Ctrl Pts',(101.172763582946,801.497233275492,117.705382376412));
#69849=CARTESIAN_POINT('Ctrl Pts',(101.184806915195,801.434193341402,117.690896042429));
#69850=CARTESIAN_POINT('Ctrl Pts',(101.183577064562,801.308768134617,117.657985660818));
#69851=CARTESIAN_POINT('Ctrl Pts',(101.170578582854,801.247637242075,117.639930834331));
#69852=CARTESIAN_POINT('Ctrl Pts',(101.120930273629,801.134485545129,117.602277962336));
#69853=CARTESIAN_POINT('Ctrl Pts',(101.08473464511,801.083700422408,117.583075919145));
#69854=CARTESIAN_POINT('Ctrl Pts',(100.993069398449,800.998815427795,117.545850400744));
#69855=CARTESIAN_POINT('Ctrl Pts',(100.938303975563,800.965888860509,117.528250577822));
#69856=CARTESIAN_POINT('Ctrl Pts',(100.816713774663,800.922634136733,117.497084754619));
#69857=CARTESIAN_POINT('Ctrl Pts',(100.750903588543,800.913241145012,117.483934347904));
#69858=CARTESIAN_POINT('Ctrl Pts',(100.68460553067,800.916635666742,117.47417310411));
#69859=CARTESIAN_POINT('Origin',(87.4554740185927,795.155415755662,103.346348239111));
#69860=CARTESIAN_POINT('',(87.4554740185928,790.556275448677,113.293935499859));
#69861=CARTESIAN_POINT('',(87.4554740185921,792.515241382411,113.881561282156));
#69862=CARTESIAN_POINT('Ctrl Pts',(87.4554740185928,790.556275448677,113.293935499859));
#69863=CARTESIAN_POINT('Ctrl Pts',(87.3253835403675,790.558833935716,113.286696557857));
#69864=CARTESIAN_POINT('Ctrl Pts',(87.196490100472,790.585213672252,113.286640186896));
#69865=CARTESIAN_POINT('Ctrl Pts',(86.9510050932038,790.68414220408,113.30175998056));
#69866=CARTESIAN_POINT('Ctrl Pts',(86.8373330070788,790.757222748724,113.317305304562));
#69867=CARTESIAN_POINT('Ctrl Pts',(86.6439779511395,790.941666492189,113.362990726077));
#69868=CARTESIAN_POINT('Ctrl Pts',(86.5666464608927,791.051678904515,113.392865238414));
#69869=CARTESIAN_POINT('Ctrl Pts',(86.4617431746276,791.291841553572,113.46226762902));
#69870=CARTESIAN_POINT('Ctrl Pts',(86.4346036414111,791.419372801328,113.500980286296));
#69871=CARTESIAN_POINT('Ctrl Pts',(86.4335451310337,791.676048198694,113.581630641002));
#69872=CARTESIAN_POINT('Ctrl Pts',(86.4594916050411,791.802665589228,113.622746811084));
#69873=CARTESIAN_POINT('Ctrl Pts',(86.5615665326647,792.038862265696,113.701322838691));
#69874=CARTESIAN_POINT('Ctrl Pts',(86.6368262096136,792.146066595192,113.737981543165));
#69875=CARTESIAN_POINT('Ctrl Pts',(86.8269999019267,792.326114157772,113.801356412446));
#69876=CARTESIAN_POINT('Ctrl Pts',(86.9400511911567,792.397174921811,113.827444669032));
#69877=CARTESIAN_POINT('Ctrl Pts',(87.1884857841945,792.492857385716,113.865606097001));
#69878=CARTESIAN_POINT('Ctrl Pts',(87.3213432683372,792.516721113301,113.877374555419));
#69879=CARTESIAN_POINT('Ctrl Pts',(87.4554740185915,792.515241382411,113.881561282156));
#69880=CARTESIAN_POINT('',(87.4554740194762,793.153312948626,112.076211874431));
#69881=CARTESIAN_POINT('',(87.4554740185927,796.118444895904,103.686715322178));
#69882=CARTESIAN_POINT('Ctrl Pts',(88.1607169118288,791.451266338037,111.609576149122));
#69883=CARTESIAN_POINT('Ctrl Pts',(88.0643783181657,791.364566235938,111.578933399469));
#69884=CARTESIAN_POINT('Ctrl Pts',(87.9510063651193,791.297213863075,111.55281188182));
#69885=CARTESIAN_POINT('Ctrl Pts',(87.703003701421,791.208685891007,111.512671475582));
#69886=CARTESIAN_POINT('Ctrl Pts',(87.5707917712519,791.18837351027,111.499049813342));
#69887=CARTESIAN_POINT('Ctrl Pts',(87.3042752643939,791.197696432798,111.486492371261));
#69888=CARTESIAN_POINT('Ctrl Pts',(87.1725233788929,791.227458982215,111.487749630293));
#69889=CARTESIAN_POINT('Ctrl Pts',(86.926993958815,791.333786780458,111.505564753685));
#69890=CARTESIAN_POINT('Ctrl Pts',(86.8156351699496,791.409540973779,111.522025919791));
#69891=CARTESIAN_POINT('Ctrl Pts',(86.6288864562886,791.597377858824,111.568318005939));
#69892=CARTESIAN_POINT('Ctrl Pts',(86.5553211902952,791.707702804868,111.597721404156));
#69893=CARTESIAN_POINT('Ctrl Pts',(86.4568845798862,791.947382859653,111.665223108358));
#69894=CARTESIAN_POINT('Ctrl Pts',(86.4324975150293,792.074268318309,111.702588476465));
#69895=CARTESIAN_POINT('Ctrl Pts',(86.4358111708451,792.330747607466,111.780832533536));
#69896=CARTESIAN_POINT('Ctrl Pts',(86.4641477142182,792.457821778439,111.82096710474));
#69897=CARTESIAN_POINT('Ctrl Pts',(86.571067227339,792.693616971415,111.897814207958));
#69898=CARTESIAN_POINT('Ctrl Pts',(86.6486641564619,792.799959219119,111.933747682322));
#69899=CARTESIAN_POINT('Ctrl Pts',(86.8421004347898,792.976150499397,111.995923470997));
#69900=CARTESIAN_POINT('Ctrl Pts',(86.9556606391781,793.04462709533,112.021650160957));
#69901=CARTESIAN_POINT('Ctrl Pts',(87.2043792987772,793.135360830149,112.059899566507));
#69902=CARTESIAN_POINT('Ctrl Pts',(87.3370932467606,793.15676534977,112.072065546988));
#69903=CARTESIAN_POINT('Ctrl Pts',(87.603782509758,793.14923193107,112.081479041617));
#69904=CARTESIAN_POINT('Ctrl Pts',(87.735178557639,793.120533767559,112.078694771524));
#69905=CARTESIAN_POINT('Ctrl Pts',(87.9807819833479,793.016054500426,112.058771356649));
#69906=CARTESIAN_POINT('Ctrl Pts',(88.0924550587883,792.940890436587,112.04171075922));
#69907=CARTESIAN_POINT('Ctrl Pts',(88.280914017646,792.752665522551,111.995317358397));
#69908=CARTESIAN_POINT('Ctrl Pts',(88.3554278358524,792.641006456432,111.966294818769));
#69909=CARTESIAN_POINT('Ctrl Pts',(88.4546503045072,792.398149932101,111.900472751406));
#69910=CARTESIAN_POINT('Ctrl Pts',(88.4789457603734,792.269496796233,111.864382725405));
#69911=CARTESIAN_POINT('Ctrl Pts',(88.4745472249191,792.011413142734,111.789311601055));
#69912=CARTESIAN_POINT('Ctrl Pts',(88.4459611000876,791.884483393573,111.751052389241));
#69913=CARTESIAN_POINT('Ctrl Pts',(88.3656264302111,791.707687626158,111.695431876093));
#69914=CARTESIAN_POINT('Ctrl Pts',(88.3326059505706,791.65127360835,111.677259725208));
#69915=CARTESIAN_POINT('Ctrl Pts',(88.2548747098177,791.545165491077,111.642153449871));
#69916=CARTESIAN_POINT('Ctrl Pts',(88.2102362031898,791.495831319252,111.625326921377));
#69917=CARTESIAN_POINT('Ctrl Pts',(88.1607169118288,791.451266338037,111.609576149122));
#69918=CARTESIAN_POINT('Ctrl Pts',(87.4554740185915,792.515241382411,113.881561282156));
#69919=CARTESIAN_POINT('Ctrl Pts',(87.4556313038014,792.51523964724,113.881566191621));
#69920=CARTESIAN_POINT('Ctrl Pts',(87.4557885907617,792.515237877217,113.881571090672));
#69921=CARTESIAN_POINT('Ctrl Pts',(87.4559458794601,792.51523607234,113.88157597931));
#69922=CARTESIAN_POINT('Ctrl Pts',(87.5897196818356,792.513701026646,113.885733758297));
#69923=CARTESIAN_POINT('Ctrl Pts',(87.7221304679224,792.48698234073,113.882287404633));
#69924=CARTESIAN_POINT('Ctrl Pts',(87.9692910476553,792.386040321447,113.861297284005));
#69925=CARTESIAN_POINT('Ctrl Pts',(88.0816233688188,792.312761486658,113.843958857174));
#69926=CARTESIAN_POINT('Ctrl Pts',(88.27107813599,792.128893080232,113.797858523711));
#69927=CARTESIAN_POINT('Ctrl Pts',(88.3463653590261,792.020033605798,113.769527284561));
#69928=CARTESIAN_POINT('Ctrl Pts',(88.4493240949078,791.781375308773,113.705355350815));
#69929=CARTESIAN_POINT('Ctrl Pts',(88.4761629535876,791.653875512941,113.670125305321));
#69930=CARTESIAN_POINT('Ctrl Pts',(88.4775703915665,791.397338462735,113.596761650743));
#69931=CARTESIAN_POINT('Ctrl Pts',(88.4523270331002,791.270732909266,113.559317028448));
#69932=CARTESIAN_POINT('Ctrl Pts',(88.352644593571,791.03491230642,113.486357641548));
#69933=CARTESIAN_POINT('Ctrl Pts',(88.2792053821163,790.927985879112,113.451541753603));
#69934=CARTESIAN_POINT('Ctrl Pts',(88.0928731410458,790.74781645978,113.38871562496));
#69935=CARTESIAN_POINT('Ctrl Pts',(87.9816782173191,790.67652309315,113.361362910284));
#69936=CARTESIAN_POINT('Ctrl Pts',(87.7355450627523,790.57956158465,113.318082029999));
#69937=CARTESIAN_POINT('Ctrl Pts',(87.602927570816,790.555130225739,113.302663470199));
#69938=CARTESIAN_POINT('Ctrl Pts',(87.46431459015,790.556129104338,113.294435645327));
#69939=CARTESIAN_POINT('Ctrl Pts',(87.4598936134117,790.556188528587,113.29418143016));
#69940=CARTESIAN_POINT('Ctrl Pts',(87.4554740185928,790.556275448677,113.293935499859));
#69941=CARTESIAN_POINT('Origin',(87.4554740185927,795.155415755662,103.346348239111));
#69942=CARTESIAN_POINT('',(87.4554740185927,793.491999124156,109.553243482599));
#69943=CARTESIAN_POINT('Origin',(87.4554740185927,793.020576893547,109.386626915332));
#69944=CARTESIAN_POINT('',(87.4554740185929,792.017155209494,113.726143089487));
#69945=CARTESIAN_POINT('',(87.4554740185927,795.626837986271,103.512964806378));
#69946=CARTESIAN_POINT('Ctrl Pts',(87.4558353843692,791.058204607979,113.438480800653));
#69947=CARTESIAN_POINT('Ctrl Pts',(87.395107247592,791.059227064835,113.435456167651));
#69948=CARTESIAN_POINT('Ctrl Pts',(87.3348995885395,791.070852031802,113.435634171487));
#69949=CARTESIAN_POINT('Ctrl Pts',(87.2167107569296,791.115870353922,113.442780376535));
#69950=CARTESIAN_POINT('Ctrl Pts',(87.1604601911993,791.150557842721,113.450245615535));
#69951=CARTESIAN_POINT('Ctrl Pts',(87.0639823201067,791.239230814299,113.472089618104));
#69952=CARTESIAN_POINT('Ctrl Pts',(87.0250007280466,791.292656297874,113.486368535044));
#69953=CARTESIAN_POINT('Ctrl Pts',(86.97120869868,791.410235149184,113.519607311488));
#69954=CARTESIAN_POINT('Ctrl Pts',(86.9567656762087,791.473148774376,113.538202487516));
#69955=CARTESIAN_POINT('Ctrl Pts',(86.9543510749744,791.600168419128,113.577075897066));
#69956=CARTESIAN_POINT('Ctrl Pts',(86.9663334441194,791.663006437193,113.596957774219));
#69957=CARTESIAN_POINT('Ctrl Pts',(87.0153338852697,791.780259083898,113.635175325558));
#69958=CARTESIAN_POINT('Ctrl Pts',(87.0518717596475,791.833495684237,113.653123712744));
#69959=CARTESIAN_POINT('Ctrl Pts',(87.1447619274761,791.92296559278,113.684508529733));
#69960=CARTESIAN_POINT('Ctrl Pts',(87.2001840939746,791.958299358853,113.697629236997));
#69961=CARTESIAN_POINT('Ctrl Pts',(87.3224539291836,792.006003370917,113.717251192452));
#69962=CARTESIAN_POINT('Ctrl Pts',(87.3880698750024,792.017908178443,113.723562835045));
#69963=CARTESIAN_POINT('Ctrl Pts',(87.520768401157,792.016428181589,113.728643294519));
#69964=CARTESIAN_POINT('Ctrl Pts',(87.5865243342633,792.003006760077,113.727350725679));
#69965=CARTESIAN_POINT('Ctrl Pts',(87.7094371416667,791.95220367027,113.717403344035));
#69966=CARTESIAN_POINT('Ctrl Pts',(87.7653025822814,791.915177376151,113.708804172052));
#69967=CARTESIAN_POINT('Ctrl Pts',(87.8580165693196,791.823281958596,113.685701418338));
#69968=CARTESIAN_POINT('Ctrl Pts',(87.8943120590452,791.769630662339,113.671529488309));
#69969=CARTESIAN_POINT('Ctrl Pts',(87.9434399741854,791.652359129353,113.639319851069));
#69970=CARTESIAN_POINT('Ctrl Pts',(87.9558689387087,791.589875652282,113.621594279242));
#69971=CARTESIAN_POINT('Ctrl Pts',(87.9550612009504,791.46438483847,113.584763385552));
#69972=CARTESIAN_POINT('Ctrl Pts',(87.941909781826,791.402578289912,113.566010139522));
#69973=CARTESIAN_POINT('Ctrl Pts',(87.8915435035756,791.28773862627,113.529745722553));
#69974=CARTESIAN_POINT('Ctrl Pts',(87.854835680133,791.235819579664,113.512584483153));
#69975=CARTESIAN_POINT('Ctrl Pts',(87.7623478554504,791.148734486793,113.482024002091));
#69976=CARTESIAN_POINT('Ctrl Pts',(87.7074350431466,791.114474968365,113.46893721144));
#69977=CARTESIAN_POINT('Ctrl Pts',(87.5863960038133,791.06838547699,113.448685678688));
#69978=CARTESIAN_POINT('Ctrl Pts',(87.5214233020689,791.057100328814,113.441747480497));
#69979=CARTESIAN_POINT('Ctrl Pts',(87.4558353843692,791.058204607979,113.438480800653));
#69980=CARTESIAN_POINT('Origin',(94.3198785361657,796.342797332624,103.766009064469));
#69981=CARTESIAN_POINT('',(94.3198785361658,791.628833734555,114.258513129312));
#69982=CARTESIAN_POINT('',(94.3198785361643,793.486184007617,114.693573355438));
#69983=CARTESIAN_POINT('Ctrl Pts',(94.3198785361657,791.628833734555,114.258513129312));
#69984=CARTESIAN_POINT('Ctrl Pts',(94.1999499248709,791.634446460657,114.242632572521));
#69985=CARTESIAN_POINT('Ctrl Pts',(94.0812954380223,791.662262567034,114.232209180336));
#69986=CARTESIAN_POINT('Ctrl Pts',(93.8516234337685,791.76205508106,114.223379074728));
#69987=CARTESIAN_POINT('Ctrl Pts',(93.7437966718754,791.835907160681,114.225910125099));
#69988=CARTESIAN_POINT('Ctrl Pts',(93.5637859343271,792.018065718583,114.244860681593));
#69989=CARTESIAN_POINT('Ctrl Pts',(93.4927273759246,792.124227158106,114.260909216245));
#69990=CARTESIAN_POINT('Ctrl Pts',(93.3965014592787,792.354666749605,114.304040522256));
#69991=CARTESIAN_POINT('Ctrl Pts',(93.3717288972453,792.476536734482,114.330575378483));
#69992=CARTESIAN_POINT('Ctrl Pts',(93.3718592883235,792.720755578022,114.390286018557));
#69993=CARTESIAN_POINT('Ctrl Pts',(93.396584521875,792.840619688169,114.422817130483));
#69994=CARTESIAN_POINT('Ctrl Pts',(93.4920515896565,793.060255122526,114.488485061245));
#69995=CARTESIAN_POINT('Ctrl Pts',(93.5608758781305,793.158154030557,114.520920811344));
#69996=CARTESIAN_POINT('Ctrl Pts',(93.7359386640734,793.323143670412,114.582575607507));
#69997=CARTESIAN_POINT('Ctrl Pts',(93.8410620672137,793.387779917198,114.611055630856));
#69998=CARTESIAN_POINT('Ctrl Pts',(94.0720804840438,793.472214532577,114.659675359076));
#69999=CARTESIAN_POINT('Ctrl Pts',(94.1955226391717,793.491216149227,114.679335495051));
#70000=CARTESIAN_POINT('Ctrl Pts',(94.3198785361628,793.486184007617,114.693573355438));
#70001=CARTESIAN_POINT('',(94.3198785361658,794.142531891777,112.836513228217));
#70002=CARTESIAN_POINT('',(94.3198785361657,797.236693505242,104.081942217606));
#70003=CARTESIAN_POINT('Ctrl Pts',(95.0444948517157,792.603277426813,112.511830837539));
#70004=CARTESIAN_POINT('Ctrl Pts',(94.9681420627759,792.517956387316,112.481675495271));
#70005=CARTESIAN_POINT('Ctrl Pts',(94.8755658797698,792.447982939598,112.45359673427));
#70006=CARTESIAN_POINT('Ctrl Pts',(94.6618342754716,792.342948464805,112.403196052339));
#70007=CARTESIAN_POINT('Ctrl Pts',(94.5415825238692,792.311134687531,112.381806624325));
#70008=CARTESIAN_POINT('Ctrl Pts',(94.2961278044905,792.29502482342,112.35090703876));
#70009=CARTESIAN_POINT('Ctrl Pts',(94.1733467495875,792.310068361198,112.341494395709));
#70010=CARTESIAN_POINT('Ctrl Pts',(93.9371484259024,792.384679404209,112.335630382237));
#70011=CARTESIAN_POINT('Ctrl Pts',(93.8260704676456,792.444272506174,112.339447506925));
#70012=CARTESIAN_POINT('Ctrl Pts',(93.6311654350456,792.601503327518,112.360425928841));
#70013=CARTESIAN_POINT('Ctrl Pts',(93.5494943912638,792.698146085825,112.377558163555));
#70014=CARTESIAN_POINT('Ctrl Pts',(93.4284135255128,792.915730082367,112.42300451116));
#70015=CARTESIAN_POINT('Ctrl Pts',(93.3902705803588,793.034635459477,112.450903262794));
#70016=CARTESIAN_POINT('Ctrl Pts',(93.3643439043819,793.273580817536,112.512201731264));
#70017=CARTESIAN_POINT('Ctrl Pts',(93.3747501484993,793.391148187109,112.544745342764));
#70018=CARTESIAN_POINT('Ctrl Pts',(93.4398681925082,793.611260754879,112.61007434376));
#70019=CARTESIAN_POINT('Ctrl Pts',(93.492521728272,793.712200265137,112.642225932259));
#70020=CARTESIAN_POINT('Ctrl Pts',(93.634279238555,793.889748468439,112.703372042273));
#70021=CARTESIAN_POINT('Ctrl Pts',(93.7222825649812,793.964588664721,112.731785802808));
#70022=CARTESIAN_POINT('Ctrl Pts',(93.9256859327996,794.079745384989,112.781937543513));
#70023=CARTESIAN_POINT('Ctrl Pts',(94.0397928277342,794.117991354328,112.80300128323));
#70024=CARTESIAN_POINT('Ctrl Pts',(94.2840055168934,794.151234546987,112.835316830307));
#70025=CARTESIAN_POINT('Ctrl Pts',(94.4121079263567,794.143509044532,112.845668162958));
#70026=CARTESIAN_POINT('Ctrl Pts',(94.6560898105082,794.080466793332,112.853050005612));
#70027=CARTESIAN_POINT('Ctrl Pts',(94.7698776073542,794.026823753307,112.850311978594));
#70028=CARTESIAN_POINT('Ctrl Pts',(94.9724996006353,793.879813616375,112.832473927347));
#70029=CARTESIAN_POINT('Ctrl Pts',(95.059083659264,793.787272735817,112.817369914873));
#70030=CARTESIAN_POINT('Ctrl Pts',(95.1919509382598,793.574908514864,112.776393641032));
#70031=CARTESIAN_POINT('Ctrl Pts',(95.2366064534347,793.456852177874,112.750807602725));
#70032=CARTESIAN_POINT('Ctrl Pts',(95.2740802707046,793.224618632098,112.695351214234));
#70033=CARTESIAN_POINT('Ctrl Pts',(95.2715071200559,793.113162902256,112.666638763691));
#70034=CARTESIAN_POINT('Ctrl Pts',(95.2245230386503,792.892164821833,112.605183934184));
#70035=CARTESIAN_POINT('Ctrl Pts',(95.1784507543524,792.785070913745,112.572881737015));
#70036=CARTESIAN_POINT('Ctrl Pts',(95.091815465336,792.659616872689,112.531397785795));
#70037=CARTESIAN_POINT('Ctrl Pts',(95.0690433999653,792.630709399946,112.521526225028));
#70038=CARTESIAN_POINT('Ctrl Pts',(95.0444948517157,792.603277426813,112.511830837539));
#70039=CARTESIAN_POINT('Ctrl Pts',(94.3198785361628,793.486184007617,114.693573355438));
#70040=CARTESIAN_POINT('Ctrl Pts',(94.3201814479661,793.486171750095,114.693608036672));
#70041=CARTESIAN_POINT('Ctrl Pts',(94.3204843651896,793.486159349951,114.693642685738));
#70042=CARTESIAN_POINT('Ctrl Pts',(94.3207872877309,793.486146807212,114.693677302633));
#70043=CARTESIAN_POINT('Ctrl Pts',(94.4423918214916,793.481111678678,114.707573830169));
#70044=CARTESIAN_POINT('Ctrl Pts',(94.5625357875021,793.453193046693,114.716031266773));
#70045=CARTESIAN_POINT('Ctrl Pts',(94.7922669428879,793.352783548108,114.72183342988));
#70046=CARTESIAN_POINT('Ctrl Pts',(94.8989193818404,793.27921826343,114.718591452997));
#70047=CARTESIAN_POINT('Ctrl Pts',(95.0771734259361,793.097584299186,114.700348787123));
#70048=CARTESIAN_POINT('Ctrl Pts',(95.1475849800514,792.991489731101,114.685632475545));
#70049=CARTESIAN_POINT('Ctrl Pts',(95.2428140827892,792.761842676514,114.646576000968));
#70050=CARTESIAN_POINT('Ctrl Pts',(95.2675201285011,792.640606010834,114.622726955487));
#70051=CARTESIAN_POINT('Ctrl Pts',(95.2683867434948,792.399142181889,114.56861189477));
#70052=CARTESIAN_POINT('Ctrl Pts',(95.2453382283517,792.281206003213,114.5389585584));
#70053=CARTESIAN_POINT('Ctrl Pts',(95.1543423974781,792.062682966526,114.476969392351));
#70054=CARTESIAN_POINT('Ctrl Pts',(95.0875621480027,791.964278660992,114.445284321032));
#70055=CARTESIAN_POINT('Ctrl Pts',(94.917408983588,791.798660843659,114.383399649576));
#70056=CARTESIAN_POINT('Ctrl Pts',(94.8155072818632,791.733605575997,114.353897130141));
#70057=CARTESIAN_POINT('Ctrl Pts',(94.5884072818366,791.645850916826,114.301068719493));
#70058=CARTESIAN_POINT('Ctrl Pts',(94.4652144984493,791.624923860551,114.278443245546));
#70059=CARTESIAN_POINT('Ctrl Pts',(94.3337109841025,791.628260380662,114.26036233615));
#70060=CARTESIAN_POINT('Ctrl Pts',(94.3267926411482,791.628510150573,114.259428672615));
#70061=CARTESIAN_POINT('Ctrl Pts',(94.3198785361657,791.628833734555,114.258513129312));
#70062=CARTESIAN_POINT('Origin',(94.3198785361657,796.342797332624,103.766009064469));
#70063=CARTESIAN_POINT('',(94.3198785361657,794.679380701117,109.972904307957));
#70064=CARTESIAN_POINT('Origin',(94.3198785361657,794.207958470509,109.80628774069));
#70065=CARTESIAN_POINT('',(94.3198785361661,793.048520242422,114.587234610521));
#70066=CARTESIAN_POINT('',(94.3198785361657,796.814219563232,103.932625631736));
#70067=CARTESIAN_POINT('Ctrl Pts',(94.320132853432,792.068989614922,114.357800917805));
#70068=CARTESIAN_POINT('Ctrl Pts',(94.2558845129119,792.071870312483,114.34955225228));
#70069=CARTESIAN_POINT('Ctrl Pts',(94.1923734261032,792.086837793992,114.344260223503));
#70070=CARTESIAN_POINT('Ctrl Pts',(94.0707675637118,792.140271091967,114.340101298925));
#70071=CARTESIAN_POINT('Ctrl Pts',(94.0142103222728,792.179363601755,114.341603445623));
#70072=CARTESIAN_POINT('Ctrl Pts',(93.9196147486483,792.275909218629,114.351676321105));
#70073=CARTESIAN_POINT('Ctrl Pts',(93.8822830362313,792.332341891131,114.360098786826));
#70074=CARTESIAN_POINT('Ctrl Pts',(93.831982898663,792.454929539717,114.382657156202));
#70075=CARTESIAN_POINT('Ctrl Pts',(93.8192954142479,792.519837184099,114.396528711945));
#70076=CARTESIAN_POINT('Ctrl Pts',(93.820486150406,792.64814158871,114.427423727633));
#70077=CARTESIAN_POINT('Ctrl Pts',(93.8336339592185,792.710277096339,114.44404492511));
#70078=CARTESIAN_POINT('Ctrl Pts',(93.8837406828856,792.825043932107,114.478024980643));
#70079=CARTESIAN_POINT('Ctrl Pts',(93.9200613152844,792.876551036056,114.495030166895));
#70080=CARTESIAN_POINT('Ctrl Pts',(94.0116076704564,792.962564793434,114.52731434934));
#70081=CARTESIAN_POINT('Ctrl Pts',(94.0659626484193,792.99609415452,114.542248458834));
#70082=CARTESIAN_POINT('Ctrl Pts',(94.1870028280717,793.040955950859,114.568392489085));
#70083=CARTESIAN_POINT('Ctrl Pts',(94.2526817079928,793.051211161219,114.579220108645));
#70084=CARTESIAN_POINT('Ctrl Pts',(94.38550251449,793.045894251701,114.595061971422));
#70085=CARTESIAN_POINT('Ctrl Pts',(94.4513180486207,793.030209918373,114.599883283801));
#70086=CARTESIAN_POINT('Ctrl Pts',(94.5742614986078,792.974690065251,114.602936647887));
#70087=CARTESIAN_POINT('Ctrl Pts',(94.6301533962583,792.935159572096,114.601082410372));
#70088=CARTESIAN_POINT('Ctrl Pts',(94.7239589495765,792.837293923143,114.590847168586));
#70089=CARTESIAN_POINT('Ctrl Pts',(94.7609089747412,792.779740229671,114.582519860644));
#70090=CARTESIAN_POINT('Ctrl Pts',(94.8091723737712,792.656692137025,114.560728524722));
#70091=CARTESIAN_POINT('Ctrl Pts',(94.820903005339,792.592637919736,114.547644054107));
#70092=CARTESIAN_POINT('Ctrl Pts',(94.8187304551029,792.465460926339,114.518211213071));
#70093=CARTESIAN_POINT('Ctrl Pts',(94.8052311361328,792.403555179987,114.502193492514));
#70094=CARTESIAN_POINT('Ctrl Pts',(94.7546532948325,792.289337576872,114.469035257421));
#70095=CARTESIAN_POINT('Ctrl Pts',(94.7182021582776,792.238167579766,114.452241610956));
#70096=CARTESIAN_POINT('Ctrl Pts',(94.6263637072458,792.152732315397,114.41981955295));
#70097=CARTESIAN_POINT('Ctrl Pts',(94.5717907076032,792.119552374481,114.404553672576));
#70098=CARTESIAN_POINT('Ctrl Pts',(94.4509524927302,792.075778742696,114.377581681358));
#70099=CARTESIAN_POINT('Ctrl Pts',(94.3857738824115,792.066046473503,114.366228386724));
#70100=CARTESIAN_POINT('Ctrl Pts',(94.320132853432,792.068989614922,114.357800917805));
#70101=CARTESIAN_POINT('Origin',(79.1680833778957,789.12355107042,101.214483166102));
#70102=CARTESIAN_POINT('',(79.1680833778957,784.521269383513,111.170958596584));
#70103=CARTESIAN_POINT('',(79.1680833778933,786.485704177605,111.743110873507));
#70104=CARTESIAN_POINT('Ctrl Pts',(79.1680833778957,784.521269383513,111.170958596584));
#70105=CARTESIAN_POINT('Ctrl Pts',(79.038495696276,784.523265496311,111.165310827197));
#70106=CARTESIAN_POINT('Ctrl Pts',(78.9101098282529,784.549054756029,111.166348335575));
#70107=CARTESIAN_POINT('Ctrl Pts',(78.6648563956979,784.64702740394,111.182602796984));
#70108=CARTESIAN_POINT('Ctrl Pts',(78.5510113593147,784.719983514685,111.198215982747));
#70109=CARTESIAN_POINT('Ctrl Pts',(78.3577721073245,784.904104430857,111.243062158392));
#70110=CARTESIAN_POINT('Ctrl Pts',(78.2805387846432,785.013781548247,111.271978423286));
#70111=CARTESIAN_POINT('Ctrl Pts',(78.1749393444207,785.254319059402,111.339231469695));
#70112=CARTESIAN_POINT('Ctrl Pts',(78.1474056758301,785.382730633137,111.376865511259));
#70113=CARTESIAN_POINT('Ctrl Pts',(78.1459781683731,785.640747173049,111.455208626358));
#70114=CARTESIAN_POINT('Ctrl Pts',(78.1717295877595,785.767807313328,111.495109588889));
#70115=CARTESIAN_POINT('Ctrl Pts',(78.273406477683,786.004861637992,111.571382975723));
#70116=CARTESIAN_POINT('Ctrl Pts',(78.3484317678547,786.112483420382,111.606975788103));
#70117=CARTESIAN_POINT('Ctrl Pts',(78.5384170098812,786.293721588223,111.668363723664));
#70118=CARTESIAN_POINT('Ctrl Pts',(78.651613522809,786.365445649623,111.693512375684));
#70119=CARTESIAN_POINT('Ctrl Pts',(78.9004957422719,786.462335228399,111.729575505573));
#70120=CARTESIAN_POINT('Ctrl Pts',(79.0336437867644,786.486733189265,111.740199404495));
#70121=CARTESIAN_POINT('Ctrl Pts',(79.1680833778909,786.485704177605,111.743110873507));
#70122=CARTESIAN_POINT('',(79.1680835138952,787.124199228011,109.936563266432));
#70123=CARTESIAN_POINT('',(79.1680833778957,790.086580210662,101.554850249169));
#70124=CARTESIAN_POINT('Ctrl Pts',(79.1681795594068,785.157640373189,109.370420786304));
#70125=CARTESIAN_POINT('Ctrl Pts',(79.0565797522559,785.159241406153,109.365859313369));
#70126=CARTESIAN_POINT('Ctrl Pts',(78.9457819465785,785.178473450502,109.366298254558));
#70127=CARTESIAN_POINT('Ctrl Pts',(78.7265698659691,785.253237743471,109.377746616587));
#70128=CARTESIAN_POINT('Ctrl Pts',(78.6206603918319,785.310837457545,109.389472296133));
#70129=CARTESIAN_POINT('Ctrl Pts',(78.4275363459733,785.463361212243,109.424812809634));
#70130=CARTESIAN_POINT('Ctrl Pts',(78.3437763000745,785.559247033304,109.448885211934));
#70131=CARTESIAN_POINT('Ctrl Pts',(78.2134481698245,785.781248379293,109.507869903562));
#70132=CARTESIAN_POINT('Ctrl Pts',(78.170515240135,785.906601377911,109.542743822392));
#70133=CARTESIAN_POINT('Ctrl Pts',(78.138113216936,786.162880012295,109.616690752767));
#70134=CARTESIAN_POINT('Ctrl Pts',(78.1479261701268,786.291213783879,109.654959003555));
#70135=CARTESIAN_POINT('Ctrl Pts',(78.2185590898771,786.537459021962,109.73045827924));
#70136=CARTESIAN_POINT('Ctrl Pts',(78.2790855396499,786.652878229769,109.766931827713));
#70137=CARTESIAN_POINT('Ctrl Pts',(78.4014042193265,786.80273854244,109.81573447721));
#70138=CARTESIAN_POINT('Ctrl Pts',(78.4464156775749,786.848044803181,109.830755023382));
#70139=CARTESIAN_POINT('Ctrl Pts',(78.5276488495495,786.915345202534,109.853522695068));
#70140=CARTESIAN_POINT('Ctrl Pts',(78.5613237813886,786.939871433717,109.861949059357));
#70141=CARTESIAN_POINT('Ctrl Pts',(78.6122234302917,786.972312574428,109.873294366734));
#70142=CARTESIAN_POINT('Ctrl Pts',(78.6282237847542,786.981900133383,109.876677423032));
#70143=CARTESIAN_POINT('Ctrl Pts',(78.6800743540025,787.011060352869,109.887066973852));
#70144=CARTESIAN_POINT('Ctrl Pts',(78.7169099836728,787.028960880562,109.893601975046));
#70145=CARTESIAN_POINT('Ctrl Pts',(78.8104233941452,787.06769306263,109.908178372036));
#70146=CARTESIAN_POINT('Ctrl Pts',(78.8681305988221,787.085897604127,109.915463717021));
#70147=CARTESIAN_POINT('Ctrl Pts',(79.0505347378378,787.126488872437,109.933433787981));
#70148=CARTESIAN_POINT('Ctrl Pts',(79.1783040990978,787.131582708756,109.939053170193));
#70149=CARTESIAN_POINT('Ctrl Pts',(79.4186547082694,787.098065123817,109.937057113325));
#70150=CARTESIAN_POINT('Ctrl Pts',(79.5298324975125,787.063489177882,109.9305786734));
#70151=CARTESIAN_POINT('Ctrl Pts',(79.7432385910014,786.956343208234,109.906549140195));
#70152=CARTESIAN_POINT('Ctrl Pts',(79.8424503831905,786.882079522847,109.888431314368));
#70153=CARTESIAN_POINT('Ctrl Pts',(80.0145709545595,786.696935900433,109.841223391061));
#70154=CARTESIAN_POINT('Ctrl Pts',(80.0835267510673,786.585589075789,109.811899048607));
#70155=CARTESIAN_POINT('Ctrl Pts',(80.1744357085788,786.342185570965,109.746150987676));
#70156=CARTESIAN_POINT('Ctrl Pts',(80.194744647275,786.212165496029,109.710248988596));
#70157=CARTESIAN_POINT('Ctrl Pts',(80.1821719388566,785.957447745236,109.638155686157));
#70158=CARTESIAN_POINT('Ctrl Pts',(80.151388104458,785.835021624015,109.602665897182));
#70159=CARTESIAN_POINT('Ctrl Pts',(80.0532344749418,785.628376756236,109.540856566718));
#70160=CARTESIAN_POINT('Ctrl Pts',(79.9938852893904,785.5425129798,109.51440542654));
#70161=CARTESIAN_POINT('Ctrl Pts',(79.8848830861954,785.429005086173,109.478057780923));
#70162=CARTESIAN_POINT('Ctrl Pts',(79.8449493356518,785.393657675966,109.466468752377));
#70163=CARTESIAN_POINT('Ctrl Pts',(79.7713452998875,785.338412853611,109.447843058239));
#70164=CARTESIAN_POINT('Ctrl Pts',(79.7390644081123,785.316994753261,109.44045036512));
#70165=CARTESIAN_POINT('Ctrl Pts',(79.6714344178052,785.277552470138,109.426460432741));
#70166=CARTESIAN_POINT('Ctrl Pts',(79.6361006665203,785.25963252552,109.419892656151));
#70167=CARTESIAN_POINT('Ctrl Pts',(79.5489861370645,785.221665691564,109.405416390313));
#70168=CARTESIAN_POINT('Ctrl Pts',(79.4963809031319,785.203648626529,109.398030619956));
#70169=CARTESIAN_POINT('Ctrl Pts',(79.353127519043,785.167153960785,109.381405109918));
#70170=CARTESIAN_POINT('Ctrl Pts',(79.2608542603522,785.156310843551,109.374208724212));
#70171=CARTESIAN_POINT('Ctrl Pts',(79.1681795594068,785.157640373189,109.370420786304));
#70172=CARTESIAN_POINT('Ctrl Pts',(79.1680833778909,786.485704177605,111.743110873507));
#70173=CARTESIAN_POINT('Ctrl Pts',(79.1683342559757,786.485702257363,111.743116306607));
#70174=CARTESIAN_POINT('Ctrl Pts',(79.1685851385565,786.485700248557,111.743121712917));
#70175=CARTESIAN_POINT('Ctrl Pts',(79.1688360255834,786.485698151175,111.743127092434));
#70176=CARTESIAN_POINT('Ctrl Pts',(79.3012650675521,786.484591062022,111.745966634573));
#70177=CARTESIAN_POINT('Ctrl Pts',(79.4323797174744,786.458827904345,111.741285419696));
#70178=CARTESIAN_POINT('Ctrl Pts',(79.6797094223275,786.359744177615,111.717947885726));
#70179=CARTESIAN_POINT('Ctrl Pts',(79.793137031013,786.286507288579,111.699276102561));
#70180=CARTESIAN_POINT('Ctrl Pts',(79.9834912650403,786.102592066859,111.651054921246));
#70181=CARTESIAN_POINT('Ctrl Pts',(80.0588282398736,785.993956923702,111.622054381437));
#70182=CARTESIAN_POINT('Ctrl Pts',(80.1619713641202,785.75518273005,111.557451980046));
#70183=CARTESIAN_POINT('Ctrl Pts',(80.1888360425792,785.627321415419,111.522459349039));
#70184=CARTESIAN_POINT('Ctrl Pts',(80.1901211924972,785.369735829489,111.450680705186));
#70185=CARTESIAN_POINT('Ctrl Pts',(80.1647227470622,785.242438260541,111.414560270241));
#70186=CARTESIAN_POINT('Ctrl Pts',(80.0647138465169,785.005337739439,111.345213681305));
#70187=CARTESIAN_POINT('Ctrl Pts',(79.9912014713939,784.897755455922,111.312628812));
#70188=CARTESIAN_POINT('Ctrl Pts',(79.8049953118768,784.716389260766,111.254659744362));
#70189=CARTESIAN_POINT('Ctrl Pts',(79.6940807464636,784.644452980825,111.229853398051));
#70190=CARTESIAN_POINT('Ctrl Pts',(79.4486018155069,784.546097890281,111.191277080136));
#70191=CARTESIAN_POINT('Ctrl Pts',(79.3163753921155,784.520912812566,111.177958377518));
#70192=CARTESIAN_POINT('Ctrl Pts',(79.17771772435,784.521153871509,111.171387654279));
#70193=CARTESIAN_POINT('Ctrl Pts',(79.1728997211776,784.521195194636,111.171168505395));
#70194=CARTESIAN_POINT('Ctrl Pts',(79.1680833778957,784.521269383513,111.170958596584));
#70195=CARTESIAN_POINT('Origin',(79.1680833778957,789.12355107042,101.214483166102));
#70196=CARTESIAN_POINT('',(79.1680833778957,787.460134438913,107.421378409591));
#70197=CARTESIAN_POINT('Origin',(79.1680833778957,786.988712208305,107.254761842323));
#70198=CARTESIAN_POINT('',(79.1680833778957,785.986909477983,111.589697374877));
#70199=CARTESIAN_POINT('',(79.1680833778957,789.594973301029,101.381099733369));
#70200=CARTESIAN_POINT('Ctrl Pts',(79.168391228125,785.025267490352,111.309649943081));
#70201=CARTESIAN_POINT('Ctrl Pts',(79.1078113239188,785.026049952496,111.307324126406));
#70202=CARTESIAN_POINT('Ctrl Pts',(79.0477543483745,785.037433740011,111.308041886352));
#70203=CARTESIAN_POINT('Ctrl Pts',(78.9296590831869,785.082033877263,111.315939718856));
#70204=CARTESIAN_POINT('Ctrl Pts',(78.8733783944443,785.116614078641,111.323598158908));
#70205=CARTESIAN_POINT('Ctrl Pts',(78.7767143522893,785.205313456759,111.345474505223));
#70206=CARTESIAN_POINT('Ctrl Pts',(78.7376263001179,785.258921662493,111.359603684456));
#70207=CARTESIAN_POINT('Ctrl Pts',(78.6837515456947,785.376962714069,111.39225754236));
#70208=CARTESIAN_POINT('Ctrl Pts',(78.6693173014704,785.440147786728,111.410425573342));
#70209=CARTESIAN_POINT('Ctrl Pts',(78.6670054811591,785.567666045195,111.448251480179));
#70210=CARTESIAN_POINT('Ctrl Pts',(78.6790458407191,785.630729446568,111.467524072511));
#70211=CARTESIAN_POINT('Ctrl Pts',(78.7281758927332,785.748442952833,111.504439064488));
#70212=CARTESIAN_POINT('Ctrl Pts',(78.764785065948,785.801911256534,111.521706560736));
#70213=CARTESIAN_POINT('Ctrl Pts',(78.8578837140739,785.891877981657,111.551701619793));
#70214=CARTESIAN_POINT('Ctrl Pts',(78.9134602960854,785.92745074866,111.564119512674));
#70215=CARTESIAN_POINT('Ctrl Pts',(79.0360374096544,785.97552759956,111.582295989573));
#70216=CARTESIAN_POINT('Ctrl Pts',(79.1017960228523,785.987568308633,111.587879222444));
#70217=CARTESIAN_POINT('Ctrl Pts',(79.2345371614157,785.986249018773,111.591520099771));
#70218=CARTESIAN_POINT('Ctrl Pts',(79.300189046162,785.972926127975,111.589552837808));
#70219=CARTESIAN_POINT('Ctrl Pts',(79.4226520444541,785.922417318756,111.578458139247));
#70220=CARTESIAN_POINT('Ctrl Pts',(79.4782117458125,785.885665419543,111.569424779973));
#70221=CARTESIAN_POINT('Ctrl Pts',(79.5707205852793,785.794147622431,111.545764836594));
#70222=CARTESIAN_POINT('Ctrl Pts',(79.6070148570429,785.74050344117,111.531441926772));
#70223=CARTESIAN_POINT('Ctrl Pts',(79.6561448310223,785.623044702354,111.499315924094));
#70224=CARTESIAN_POINT('Ctrl Pts',(79.6685427342927,785.560358099776,111.481820512201));
#70225=CARTESIAN_POINT('Ctrl Pts',(79.667599460703,785.434364550547,111.445870573146));
#70226=CARTESIAN_POINT('Ctrl Pts',(79.6543460022899,785.372256211283,111.42775664183));
#70227=CARTESIAN_POINT('Ctrl Pts',(79.6037679482855,785.256860725903,111.393118016673));
#70228=CARTESIAN_POINT('Ctrl Pts',(79.5669857453052,785.204666448264,111.376920019965));
#70229=CARTESIAN_POINT('Ctrl Pts',(79.4744461441153,785.117087834358,111.348427387096));
#70230=CARTESIAN_POINT('Ctrl Pts',(79.4195852814138,785.082576929838,111.33641404502));
#70231=CARTESIAN_POINT('Ctrl Pts',(79.2987116446366,785.035975259901,111.318181335789));
#70232=CARTESIAN_POINT('Ctrl Pts',(79.2338606263067,785.024421874527,111.312163479871));
#70233=CARTESIAN_POINT('Ctrl Pts',(79.168391228125,785.025267490352,111.309649943081));
#70234=CARTESIAN_POINT('Origin',(86.1443200694598,788.939367371895,101.149386415032));
#70235=CARTESIAN_POINT('',(86.1443200694599,784.218471557535,111.661504380944));
#70236=CARTESIAN_POINT('',(86.1443200694503,786.091238748752,112.052944227269));
#70237=CARTESIAN_POINT('Ctrl Pts',(86.1443200694599,784.218471557536,111.661504380944));
#70238=CARTESIAN_POINT('Ctrl Pts',(86.0232438014687,784.223073791487,111.64848289436));
#70239=CARTESIAN_POINT('Ctrl Pts',(85.9035767255775,784.250562154714,111.640293350206));
#70240=CARTESIAN_POINT('Ctrl Pts',(85.6727855885495,784.350654196083,111.634594772174));
#70241=CARTESIAN_POINT('Ctrl Pts',(85.5649088275317,784.425006936018,111.637854698421));
#70242=CARTESIAN_POINT('Ctrl Pts',(85.385137013404,784.608767941465,111.656521250761));
#70243=CARTESIAN_POINT('Ctrl Pts',(85.3144201570192,784.716099024219,111.671616691658));
#70244=CARTESIAN_POINT('Ctrl Pts',(85.2194105317485,784.948790966923,111.711418723205));
#70245=CARTESIAN_POINT('Ctrl Pts',(85.1953917516291,785.071771854287,111.735628162361));
#70246=CARTESIAN_POINT('Ctrl Pts',(85.1971198637617,785.317934859568,111.789674249004));
#70247=CARTESIAN_POINT('Ctrl Pts',(85.2225773921297,785.438692239883,111.818935351978));
#70248=CARTESIAN_POINT('Ctrl Pts',(85.319467638155,785.660230273347,111.877649929256));
#70249=CARTESIAN_POINT('Ctrl Pts',(85.3890318696257,785.759126606001,111.906487526506));
#70250=CARTESIAN_POINT('Ctrl Pts',(85.5636352728739,785.923988162167,111.960079069209));
#70251=CARTESIAN_POINT('Ctrl Pts',(85.6667991916973,785.988348088792,111.984291303336));
#70252=CARTESIAN_POINT('Ctrl Pts',(85.8957661859035,786.074845854189,112.025409242133));
#70253=CARTESIAN_POINT('Ctrl Pts',(86.0195494801765,786.095201758359,112.041731351737));
#70254=CARTESIAN_POINT('Ctrl Pts',(86.1443200694407,786.091238748751,112.052944227269));
#70255=CARTESIAN_POINT('',(86.1443200694599,786.744690678997,110.20407786539));
#70256=CARTESIAN_POINT('',(86.1443200694598,789.833263544514,101.465319568169));
#70257=CARTESIAN_POINT('Ctrl Pts',(86.7259870614681,785.070398779602,109.849456642294));
#70258=CARTESIAN_POINT('Ctrl Pts',(86.6324881639625,785.001909523517,109.825250221801));
#70259=CARTESIAN_POINT('Ctrl Pts',(86.5262728280359,784.95163570823,109.804133977455));
#70260=CARTESIAN_POINT('Ctrl Pts',(86.2931301198167,784.890885113085,109.769384716974));
#70261=CARTESIAN_POINT('Ctrl Pts',(86.1677878289683,784.883408955391,109.756597027203));
#70262=CARTESIAN_POINT('Ctrl Pts',(85.9223980754791,784.915940279537,109.742888883384));
#70263=CARTESIAN_POINT('Ctrl Pts',(85.804596904887,784.954824781141,109.741902443628));
#70264=CARTESIAN_POINT('Ctrl Pts',(85.5877796868017,785.074328280863,109.751904943332));
#70265=CARTESIAN_POINT('Ctrl Pts',(85.4910754501357,785.154511963793,109.762999476033));
#70266=CARTESIAN_POINT('Ctrl Pts',(85.3327047136388,785.346751334975,109.796351104006));
#70267=CARTESIAN_POINT('Ctrl Pts',(85.2729500757762,785.45740894643,109.818436662026));
#70268=CARTESIAN_POINT('Ctrl Pts',(85.2003164193624,785.694189460527,109.870667708466));
#70269=CARTESIAN_POINT('Ctrl Pts',(85.1882487292566,785.818070558252,109.900325048123));
#70270=CARTESIAN_POINT('Ctrl Pts',(85.2139756320044,786.057035713228,109.961630513494));
#70271=CARTESIAN_POINT('Ctrl Pts',(85.2494557375695,786.170055885681,109.992566991673));
#70272=CARTESIAN_POINT('Ctrl Pts',(85.3608253008893,786.372679070545,110.051714652982));
#70273=CARTESIAN_POINT('Ctrl Pts',(85.4343428004351,786.461115416521,110.079447200168));
#70274=CARTESIAN_POINT('Ctrl Pts',(85.6120434466344,786.607006292119,110.129404539419));
#70275=CARTESIAN_POINT('Ctrl Pts',(85.7147630845295,786.662946425091,110.151138378081));
#70276=CARTESIAN_POINT('Ctrl Pts',(85.9397702530505,786.735648969544,110.18628537658));
#70277=CARTESIAN_POINT('Ctrl Pts',(86.0603402946392,786.75063917116,110.199129741105));
#70278=CARTESIAN_POINT('Ctrl Pts',(86.307971880145,786.735142098257,110.214218829165));
#70279=CARTESIAN_POINT('Ctrl Pts',(86.4324776988788,786.702383891835,110.21572275723));
#70280=CARTESIAN_POINT('Ctrl Pts',(86.6592813594046,786.592688230903,110.206615706328));
#70281=CARTESIAN_POINT('Ctrl Pts',(86.7598773624179,786.517800411025,110.196369055275));
#70282=CARTESIAN_POINT('Ctrl Pts',(86.9280175442621,786.33404887482,110.165545350349));
#70283=CARTESIAN_POINT('Ctrl Pts',(86.9935224417377,786.226436443181,110.145114541764));
#70284=CARTESIAN_POINT('Ctrl Pts',(87.079017874582,785.992433144348,110.096490285624));
#70285=CARTESIAN_POINT('Ctrl Pts',(87.0977824872587,785.868092066369,110.068683007201));
#70286=CARTESIAN_POINT('Ctrl Pts',(87.0850708559952,785.633404663581,110.012359342614));
#70287=CARTESIAN_POINT('Ctrl Pts',(87.0587161614571,785.524815594854,109.984660067105));
#70288=CARTESIAN_POINT('Ctrl Pts',(86.9651791190065,785.317742728665,109.928126879479));
#70289=CARTESIAN_POINT('Ctrl Pts',(86.8968821834878,785.221982460985,109.899830374314));
#70290=CARTESIAN_POINT('Ctrl Pts',(86.7846733949305,785.116233260758,109.865310780573));
#70291=CARTESIAN_POINT('Ctrl Pts',(86.756048336616,785.09241908601,109.857239363654));
#70292=CARTESIAN_POINT('Ctrl Pts',(86.7259870614681,785.070398779602,109.849456642294));
#70293=CARTESIAN_POINT('Ctrl Pts',(86.1443200694407,786.091238748751,112.052944227269));
#70294=CARTESIAN_POINT('Ctrl Pts',(86.1446495235245,786.091228284509,112.052973834628));
#70295=CARTESIAN_POINT('Ctrl Pts',(86.1449789844855,786.091217650699,112.053003406431));
#70296=CARTESIAN_POINT('Ctrl Pts',(86.1453084521914,786.091206847301,112.053032942666));
#70297=CARTESIAN_POINT('Ctrl Pts',(86.2684868787339,786.08716776983,112.064075684971));
#70298=CARTESIAN_POINT('Ctrl Pts',(86.3901386013758,786.059510627326,112.069930167044));
#70299=CARTESIAN_POINT('Ctrl Pts',(86.6199199055224,785.959244886059,112.071277448783));
#70300=CARTESIAN_POINT('Ctrl Pts',(86.7253881253119,785.886477628309,112.066498366302));
#70301=CARTESIAN_POINT('Ctrl Pts',(86.9039325757279,785.704443352265,112.046848165786));
#70302=CARTESIAN_POINT('Ctrl Pts',(86.9748800396098,785.596346451338,112.032016692792));
#70303=CARTESIAN_POINT('Ctrl Pts',(87.0694458972329,785.362733236678,111.994548640001));
#70304=CARTESIAN_POINT('Ctrl Pts',(87.0932243693923,785.239656152849,111.972401425732));
#70305=CARTESIAN_POINT('Ctrl Pts',(87.0915567043042,784.994789033857,111.923368043958));
#70306=CARTESIAN_POINT('Ctrl Pts',(87.0670010783056,784.87522123426,111.897005218452));
#70307=CARTESIAN_POINT('Ctrl Pts',(86.9729694945433,784.654587721567,111.842899430378));
#70308=CARTESIAN_POINT('Ctrl Pts',(86.9049801725677,784.555495185941,111.815704126075));
#70309=CARTESIAN_POINT('Ctrl Pts',(86.7332512703618,784.389390804322,111.763339720698));
#70310=CARTESIAN_POINT('Ctrl Pts',(86.6312613812925,784.324240890815,111.738734258038));
#70311=CARTESIAN_POINT('Ctrl Pts',(86.404729652754,784.236310932174,111.695148800306));
#70312=CARTESIAN_POINT('Ctrl Pts',(86.2823161654338,784.215182880036,111.676744306655));
#70313=CARTESIAN_POINT('Ctrl Pts',(86.153871706826,784.218144173277,111.662538917529));
#70314=CARTESIAN_POINT('Ctrl Pts',(86.1490947922307,784.218290065393,111.662017891887));
#70315=CARTESIAN_POINT('Ctrl Pts',(86.1443200694599,784.218471557536,111.661504380944));
#70316=CARTESIAN_POINT('Origin',(86.1443200694598,788.939367371895,101.149386415032));
#70317=CARTESIAN_POINT('',(86.1443200694598,787.275950740389,107.356281658521));
#70318=CARTESIAN_POINT('Origin',(86.1443200694598,786.80452850978,107.189665091254));
#70319=CARTESIAN_POINT('',(86.1443200694602,785.650395405619,111.955601728935));
#70320=CARTESIAN_POINT('',(86.1443200694598,789.410789602504,101.316002982299));
#70321=CARTESIAN_POINT('Ctrl Pts',(86.1447175963381,784.662722492406,111.749205968351));
#70322=CARTESIAN_POINT('Ctrl Pts',(86.0790639755617,784.665072798417,111.742399408785));
#70323=CARTESIAN_POINT('Ctrl Pts',(86.0142265421774,784.680172569735,111.738315514435));
#70324=CARTESIAN_POINT('Ctrl Pts',(85.8916808562695,784.734517684191,111.736071683426));
#70325=CARTESIAN_POINT('Ctrl Pts',(85.8354078768984,784.773940501574,111.73811386647));
#70326=CARTESIAN_POINT('Ctrl Pts',(85.7415320712461,784.871287659228,111.748325758983));
#70327=CARTESIAN_POINT('Ctrl Pts',(85.7046579955178,784.928223230305,111.756366924686));
#70328=CARTESIAN_POINT('Ctrl Pts',(85.6553823759995,785.051794067799,111.777325443641));
#70329=CARTESIAN_POINT('Ctrl Pts',(85.6432461955908,785.117220056091,111.790011282445));
#70330=CARTESIAN_POINT('Ctrl Pts',(85.6455161442487,785.246771479336,111.817998634657));
#70331=CARTESIAN_POINT('Ctrl Pts',(85.6592911271632,785.309661546211,111.832963427702));
#70332=CARTESIAN_POINT('Ctrl Pts',(85.7106978120086,785.425525656657,111.863214412855));
#70333=CARTESIAN_POINT('Ctrl Pts',(85.7475800563947,785.477429862313,111.878189971105));
#70334=CARTESIAN_POINT('Ctrl Pts',(85.8399717853424,785.56385445823,111.906221565601));
#70335=CARTESIAN_POINT('Ctrl Pts',(85.8945059412723,785.59749810403,111.918988579773));
#70336=CARTESIAN_POINT('Ctrl Pts',(86.0152688124681,785.642383286418,111.94084131766));
#70337=CARTESIAN_POINT('Ctrl Pts',(86.0804048705909,785.652738356333,111.949627123714));
#70338=CARTESIAN_POINT('Ctrl Pts',(86.2125174373546,785.647901267344,111.961977841987));
#70339=CARTESIAN_POINT('Ctrl Pts',(86.2781371435774,785.632404365839,111.96534462441));
#70340=CARTESIAN_POINT('Ctrl Pts',(86.4004134430373,785.577245284638,111.96621938934));
#70341=CARTESIAN_POINT('Ctrl Pts',(86.4558315704492,785.537966698863,111.963685501028));
#70342=CARTESIAN_POINT('Ctrl Pts',(86.5488817521974,785.440581970136,111.953068499387));
#70343=CARTESIAN_POINT('Ctrl Pts',(86.5855214737621,785.383219071274,111.945039413769));
#70344=CARTESIAN_POINT('Ctrl Pts',(86.6337998151398,785.259613954274,111.92470894953));
#70345=CARTESIAN_POINT('Ctrl Pts',(86.6455115360651,785.194658947201,111.912674115002));
#70346=CARTESIAN_POINT('Ctrl Pts',(86.6429589584479,785.065677491729,111.886098320221));
#70347=CARTESIAN_POINT('Ctrl Pts',(86.6291498617514,785.00283709202,111.871843492542));
#70348=CARTESIAN_POINT('Ctrl Pts',(86.5778838978083,784.887159236913,111.842774131275));
#70349=CARTESIAN_POINT('Ctrl Pts',(86.5412040515293,784.835369261024,111.828254525587));
#70350=CARTESIAN_POINT('Ctrl Pts',(86.449203178204,784.749006572816,111.800581738242));
#70351=CARTESIAN_POINT('Ctrl Pts',(86.3948239620984,784.715383134124,111.787724194351));
#70352=CARTESIAN_POINT('Ctrl Pts',(86.2746031816651,784.670674004925,111.765270017627));
#70353=CARTESIAN_POINT('Ctrl Pts',(86.2099024020029,784.660388969307,111.755963924078));
#70354=CARTESIAN_POINT('Ctrl Pts',(86.1447175963381,784.662722492406,111.749205968351));
#70355=CARTESIAN_POINT('Origin',(58.6359451072587,790.091644456036,101.556640124838));
#70356=CARTESIAN_POINT('',(58.6359451072587,787.962812675165,112.230333666846));
#70357=CARTESIAN_POINT('Origin',(58.6359451072587,786.501713859367,111.713931907829));
#70358=CARTESIAN_POINT('',(58.6359451072371,788.629270889217,110.344667535143));
#70359=CARTESIAN_POINT('',(58.6359451072587,791.552743271833,102.073041883855));
#70360=CARTESIAN_POINT('Ctrl Pts',(58.6360112917652,785.683487034017,109.378598502357));
#70361=CARTESIAN_POINT('Ctrl Pts',(58.5934212586555,785.683433325671,109.378745005346));
#70362=CARTESIAN_POINT('Ctrl Pts',(58.5508491600315,785.685061751144,109.379400993085));
#70363=CARTESIAN_POINT('Ctrl Pts',(58.4173803867427,785.695459149166,109.383059322162));
#70364=CARTESIAN_POINT('Ctrl Pts',(58.3272019823704,785.710247041297,109.387879412916));
#70365=CARTESIAN_POINT('Ctrl Pts',(58.1169108226222,785.763387269929,109.404785756253));
#70366=CARTESIAN_POINT('Ctrl Pts',(57.9993169496857,785.808384142461,109.418879104229));
#70367=CARTESIAN_POINT('Ctrl Pts',(57.7083753933041,785.961349932394,109.466595888032));
#70368=CARTESIAN_POINT('Ctrl Pts',(57.549602335207,786.089615809777,109.506455074143));
#70369=CARTESIAN_POINT('Ctrl Pts',(57.3072455168803,786.381429583381,109.597965461416));
#70370=CARTESIAN_POINT('Ctrl Pts',(57.2194361224958,786.537537172826,109.647229099602));
#70371=CARTESIAN_POINT('Ctrl Pts',(57.1021429212925,786.880874522943,109.756900187524));
#70372=CARTESIAN_POINT('Ctrl Pts',(57.0772865499598,787.066323531765,109.816823279474));
#70373=CARTESIAN_POINT('Ctrl Pts',(57.1017554907427,787.447084244517,109.941562652666));
#70374=CARTESIAN_POINT('Ctrl Pts',(57.1554751227801,787.638481920637,110.005204307833));
#70375=CARTESIAN_POINT('Ctrl Pts',(57.3373200955687,787.986600043651,110.122429031596));
#70376=CARTESIAN_POINT('Ctrl Pts',(57.4624095156542,788.140469086084,110.175006241827));
#70377=CARTESIAN_POINT('Ctrl Pts',(57.7707058476356,788.395594787389,110.262919683401));
#70378=CARTESIAN_POINT('Ctrl Pts',(57.9517378698733,788.493398842964,110.297056511618));
#70379=CARTESIAN_POINT('Ctrl Pts',(58.2603293965507,788.590081206249,110.330899840703));
#70380=CARTESIAN_POINT('Ctrl Pts',(58.3768393456003,788.61302604832,110.338966249576));
#70381=CARTESIAN_POINT('Ctrl Pts',(58.5824662727724,788.630747755917,110.345190272108));
#70382=CARTESIAN_POINT('Ctrl Pts',(58.6704756685845,788.631255966232,110.345365104003));
#70383=CARTESIAN_POINT('Ctrl Pts',(58.846119991235,788.618166081974,110.340738557602));
#70384=CARTESIAN_POINT('Ctrl Pts',(58.9334289239458,788.60451362539,110.335918003867));
#70385=CARTESIAN_POINT('Ctrl Pts',(59.1324646379154,788.556625662076,110.319031637685));
#70386=CARTESIAN_POINT('Ctrl Pts',(59.2422582641522,788.517294170075,110.305172525968));
#70387=CARTESIAN_POINT('Ctrl Pts',(59.5300463347398,788.377244135138,110.255992915242));
#70388=CARTESIAN_POINT('Ctrl Pts',(59.69297781754,788.253988261049,110.21285265492));
#70389=CARTESIAN_POINT('Ctrl Pts',(59.9418603811138,787.97228364501,110.115406156515));
#70390=CARTESIAN_POINT('Ctrl Pts',(60.0328374740205,787.822121236338,110.063867581492));
#70391=CARTESIAN_POINT('Ctrl Pts',(60.1592605008424,787.488996131706,109.95100437375));
#70392=CARTESIAN_POINT('Ctrl Pts',(60.1900602977308,787.307524498111,109.890279344063));
#70393=CARTESIAN_POINT('Ctrl Pts',(60.179817887963,786.930798802891,109.766154932587));
#70394=CARTESIAN_POINT('Ctrl Pts',(60.134099569607,786.739118347925,109.704065529562));
#70395=CARTESIAN_POINT('Ctrl Pts',(59.9674977422645,786.38397477116,109.590909967842));
#70396=CARTESIAN_POINT('Ctrl Pts',(59.8485748527781,786.223833018589,109.540878268881));
#70397=CARTESIAN_POINT('Ctrl Pts',(59.5519042990591,785.955495691196,109.458296014561));
#70398=CARTESIAN_POINT('Ctrl Pts',(59.3767380367989,785.850226829109,109.426628824816));
#70399=CARTESIAN_POINT('Ctrl Pts',(59.0721263972114,785.739320213053,109.393885592828));
#70400=CARTESIAN_POINT('Ctrl Pts',(58.9543318038803,785.71092437552,109.385708176056));
#70401=CARTESIAN_POINT('Ctrl Pts',(58.768546670276,785.687730857853,109.379377275714));
#70402=CARTESIAN_POINT('Ctrl Pts',(58.7023139431371,785.683570645264,109.378370431706));
#70403=CARTESIAN_POINT('Ctrl Pts',(58.6360112917652,785.683487034017,109.378598502357));
#70404=CARTESIAN_POINT('Origin',(58.6359451072587,790.091644456036,101.556640124838));
#70405=CARTESIAN_POINT('',(58.6359451072587,788.42822782453,107.763535368326));
#70406=CARTESIAN_POINT('Origin',(58.6359451072587,787.956805593921,107.596918801059));
#70407=CARTESIAN_POINT('',(58.6359451072587,786.973136089976,111.880548475096));
#70408=CARTESIAN_POINT('',(58.6359451072587,790.563066686645,101.723256692105));
#70409=CARTESIAN_POINT('Origin',(58.6359451072587,786.501713859367,111.713931907829));
#70410=CARTESIAN_POINT('Origin',(63.9954594876854,787.256016761222,100.554433351629));
#70411=CARTESIAN_POINT('',(63.9954594876854,784.853467741515,111.131385959978));
#70412=CARTESIAN_POINT('Origin',(63.9954594876854,783.666086164553,110.71172513462));
#70413=CARTESIAN_POINT('',(63.9954594857071,785.501764606246,109.297105257399));
#70414=CARTESIAN_POINT('',(63.9954594876854,788.443398338184,100.974094176987));
#70415=CARTESIAN_POINT('Ctrl Pts',(63.9953219214531,783.079207789871,108.593010247634));
#70416=CARTESIAN_POINT('Ctrl Pts',(63.9634403507654,783.079109028351,108.593300132773));
#70417=CARTESIAN_POINT('Ctrl Pts',(63.9315697531246,783.080181855706,108.593908199));
#70418=CARTESIAN_POINT('Ctrl Pts',(63.8289234252417,783.087422140518,108.596893307604));
#70419=CARTESIAN_POINT('Ctrl Pts',(63.7586533599441,783.098216849211,108.600519814419));
#70420=CARTESIAN_POINT('Ctrl Pts',(63.5894835574832,783.138648577437,108.613170508994));
#70421=CARTESIAN_POINT('Ctrl Pts',(63.492731028879,783.174459467676,108.623847392199));
#70422=CARTESIAN_POINT('Ctrl Pts',(63.253827423507,783.29729116606,108.659648845313));
#70423=CARTESIAN_POINT('Ctrl Pts',(63.1233366762046,783.401071291594,108.689263983923));
#70424=CARTESIAN_POINT('Ctrl Pts',(62.9237206983426,783.638023348043,108.756633023886));
#70425=CARTESIAN_POINT('Ctrl Pts',(62.8510266210737,783.76488426197,108.792627068914));
#70426=CARTESIAN_POINT('Ctrl Pts',(62.7522703730241,784.044938749867,108.872466935751));
#70427=CARTESIAN_POINT('Ctrl Pts',(62.7300370223754,784.196796038279,108.915963009024));
#70428=CARTESIAN_POINT('Ctrl Pts',(62.7454369677152,784.509441867852,109.006232398207));
#70429=CARTESIAN_POINT('Ctrl Pts',(62.7866177928744,784.667138668229,109.052161077309));
#70430=CARTESIAN_POINT('Ctrl Pts',(62.9298158258099,784.955764713402,109.136849485736));
#70431=CARTESIAN_POINT('Ctrl Pts',(63.0296412381602,785.084217827181,109.174863410891));
#70432=CARTESIAN_POINT('Ctrl Pts',(63.2751955144117,785.296604402606,109.237831898397));
#70433=CARTESIAN_POINT('Ctrl Pts',(63.4184661898421,785.378531055751,109.262175722522));
#70434=CARTESIAN_POINT('Ctrl Pts',(63.667628860898,785.46356478289,109.287013767226));
#70435=CARTESIAN_POINT('Ctrl Pts',(63.764701445428,785.484786995277,109.293063915288));
#70436=CARTESIAN_POINT('Ctrl Pts',(63.9325074295607,785.501990879562,109.297504334598));
#70437=CARTESIAN_POINT('Ctrl Pts',(64.0021477557783,785.503592658949,109.297636891416));
#70438=CARTESIAN_POINT('Ctrl Pts',(64.1030708741173,785.497921031115,109.295349331963));
#70439=CARTESIAN_POINT('Ctrl Pts',(64.1344987271119,785.495018209405,109.294284466736));
#70440=CARTESIAN_POINT('Ctrl Pts',(64.2359926197191,785.481945868022,109.289698310745));
#70441=CARTESIAN_POINT('Ctrl Pts',(64.3052734101441,785.46725232174,109.284776957922));
#70442=CARTESIAN_POINT('Ctrl Pts',(64.4724952156569,785.417318882363,109.268421434084));
#70443=CARTESIAN_POINT('Ctrl Pts',(64.5678269053854,785.37583971053,109.25506930429));
#70444=CARTESIAN_POINT('Ctrl Pts',(64.7996433554226,785.239469992345,109.211746232437));
#70445=CARTESIAN_POINT('Ctrl Pts',(64.9234968634013,785.128812661035,109.177042998576));
#70446=CARTESIAN_POINT('Ctrl Pts',(65.1074081567735,784.882051521045,109.100960786265));
#70447=CARTESIAN_POINT('Ctrl Pts',(65.1716361928218,784.75219348862,109.061393699662));
#70448=CARTESIAN_POINT('Ctrl Pts',(65.2523304975,784.467614714687,108.976030377366));
#70449=CARTESIAN_POINT('Ctrl Pts',(65.2646432854445,784.314365839574,108.930768839063));
#70450=CARTESIAN_POINT('Ctrl Pts',(65.2284965205647,784.003194891884,108.840502095042));
#70451=CARTESIAN_POINT('Ctrl Pts',(65.1771813281799,783.848496517605,108.796520752538));
#70452=CARTESIAN_POINT('Ctrl Pts',(65.0163323663172,783.569217945263,108.718703210265));
#70453=CARTESIAN_POINT('Ctrl Pts',(64.9092886404542,783.446815684077,108.685434649322));
#70454=CARTESIAN_POINT('Ctrl Pts',(64.663337821583,783.256502698469,108.634942560308));
#70455=CARTESIAN_POINT('Ctrl Pts',(64.5298007662076,783.186419871577,108.617004866245));
#70456=CARTESIAN_POINT('Ctrl Pts',(64.3041632931217,783.114389570073,108.599522013241));
#70457=CARTESIAN_POINT('Ctrl Pts',(64.2190831819158,783.09634971238,108.595451984538));
#70458=CARTESIAN_POINT('Ctrl Pts',(64.0871325449022,783.081923075148,108.592835710093));
#70459=CARTESIAN_POINT('Ctrl Pts',(64.0412455965643,783.079350050488,108.592592683799));
#70460=CARTESIAN_POINT('Ctrl Pts',(63.9953219214531,783.079207789871,108.593010247634));
#70461=CARTESIAN_POINT('Origin',(63.9954594876854,787.256016761222,100.554433351629));
#70462=CARTESIAN_POINT('',(63.9954594876854,785.592600129715,106.761328595117));
#70463=CARTESIAN_POINT('Origin',(63.9954594876854,785.121177899107,106.59471202785));
#70464=CARTESIAN_POINT('',(63.9954594876854,784.137508395162,110.878341701887));
#70465=CARTESIAN_POINT('',(63.9954594876854,787.72743899183,100.721049918896));
#70466=CARTESIAN_POINT('Origin',(63.9954594876854,783.666086164553,110.71172513462));
#70467=CARTESIAN_POINT('Origin',(69.7316732616476,784.848060912957,99.7033802796288));
#70468=CARTESIAN_POINT('',(69.7316732616476,780.243496355298,109.666314827831));
#70469=CARTESIAN_POINT('',(69.7316732616476,782.211734062764,110.227707202932));
#70470=CARTESIAN_POINT('Ctrl Pts',(69.7316732616476,780.243496355298,109.666314827831));
#70471=CARTESIAN_POINT('Ctrl Pts',(69.6035672430037,780.244787361547,109.662662075552));
#70472=CARTESIAN_POINT('Ctrl Pts',(69.4766151361266,780.269448399822,109.66520829645));
#70473=CARTESIAN_POINT('Ctrl Pts',(69.2322800901463,780.365064241757,109.683393659838));
#70474=CARTESIAN_POINT('Ctrl Pts',(69.1181296682301,780.437328831716,109.699517539606));
#70475=CARTESIAN_POINT('Ctrl Pts',(68.9240377574953,780.620598551093,109.744397312699));
#70476=CARTESIAN_POINT('Ctrl Pts',(68.8462981895684,780.730166662832,109.772845259494));
#70477=CARTESIAN_POINT('Ctrl Pts',(68.7393590255276,780.971532284846,109.838678474064));
#70478=CARTESIAN_POINT('Ctrl Pts',(68.7112664462007,781.100986137373,109.875432840945));
#70479=CARTESIAN_POINT('Ctrl Pts',(68.7093271581908,781.360711137878,109.951681513805));
#70480=CARTESIAN_POINT('Ctrl Pts',(68.734888715193,781.48841604878,109.99038369636));
#70481=CARTESIAN_POINT('Ctrl Pts',(68.8361969648346,781.726416524879,110.064246696049));
#70482=CARTESIAN_POINT('Ctrl Pts',(68.9108964899515,781.834388247012,110.09866460518));
#70483=CARTESIAN_POINT('Ctrl Pts',(69.1003519106522,782.016639712931,110.157928290986));
#70484=CARTESIAN_POINT('Ctrl Pts',(69.2134117469588,782.088957655794,110.182124916369));
#70485=CARTESIAN_POINT('Ctrl Pts',(69.4627339866786,782.187316552922,110.216316324272));
#70486=CARTESIAN_POINT('Ctrl Pts',(69.5965420190118,782.212351494003,110.225960252934));
#70487=CARTESIAN_POINT('Ctrl Pts',(69.7316732616476,782.211734062764,110.227707202932));
#70488=CARTESIAN_POINT('',(69.7316732616702,782.827991978286,108.484076986977));
#70489=CARTESIAN_POINT('',(69.7316732616476,785.811090053199,100.043747362696));
#70490=CARTESIAN_POINT('Ctrl Pts',(69.7318153101166,780.843131484731,107.96971688462));
#70491=CARTESIAN_POINT('Ctrl Pts',(69.6375166661361,780.843123464971,107.969700221094));
#70492=CARTESIAN_POINT('Ctrl Pts',(69.5436863369083,780.855844728437,107.972854971));
#70493=CARTESIAN_POINT('Ctrl Pts',(69.3498604307255,780.909428975668,107.986198881597));
#70494=CARTESIAN_POINT('Ctrl Pts',(69.2520257946803,780.953570742773,107.997208303356));
#70495=CARTESIAN_POINT('Ctrl Pts',(69.066034155537,781.075016085042,108.027624702619));
#70496=CARTESIAN_POINT('Ctrl Pts',(68.9809430616127,781.154056140655,108.047476812565));
#70497=CARTESIAN_POINT('Ctrl Pts',(68.8369280171959,781.343018442622,108.09522531929));
#70498=CARTESIAN_POINT('Ctrl Pts',(68.7815223568898,781.453176152445,108.123203489822));
#70499=CARTESIAN_POINT('Ctrl Pts',(68.7120864656617,781.694966148047,108.185096763272));
#70500=CARTESIAN_POINT('Ctrl Pts',(68.7016897333903,781.825286227403,108.218711938315));
#70501=CARTESIAN_POINT('Ctrl Pts',(68.7331310173967,782.083699019231,108.285943406331));
#70502=CARTESIAN_POINT('Ctrl Pts',(68.7752474341524,782.209277021531,108.318911524792));
#70503=CARTESIAN_POINT('Ctrl Pts',(68.9042942849275,782.431927565488,108.377788983928));
#70504=CARTESIAN_POINT('Ctrl Pts',(68.9878862493639,782.52808328057,108.403427529047));
#70505=CARTESIAN_POINT('Ctrl Pts',(69.1679476320414,782.669766803881,108.441373804505));
#70506=CARTESIAN_POINT('Ctrl Pts',(69.2575787692492,782.720713653666,108.455089385681));
#70507=CARTESIAN_POINT('Ctrl Pts',(69.3974062319674,782.77466023747,108.469640517441));
#70508=CARTESIAN_POINT('Ctrl Pts',(69.4423610085247,782.78860039153,108.473406421392));
#70509=CARTESIAN_POINT('Ctrl Pts',(69.5193886940357,782.806907027757,108.478356459356));
#70510=CARTESIAN_POINT('Ctrl Pts',(69.5509692571673,782.812897783851,108.479977975895));
#70511=CARTESIAN_POINT('Ctrl Pts',(69.5972351897966,782.819495838748,108.481765566566));
#70512=CARTESIAN_POINT('Ctrl Pts',(69.6117239400673,782.821255703991,108.482242684802));
#70513=CARTESIAN_POINT('Ctrl Pts',(69.6598980083961,782.826093843841,108.483555443499));
#70514=CARTESIAN_POINT('Ctrl Pts',(69.6937024021389,782.82785262878,108.484034748969));
#70515=CARTESIAN_POINT('Ctrl Pts',(69.7812581577431,782.828192666179,108.484137200691));
#70516=CARTESIAN_POINT('Ctrl Pts',(69.8349132823111,782.824297482342,108.483090758963));
#70517=CARTESIAN_POINT('Ctrl Pts',(70.0101826552149,782.798006972545,108.476017453203));
#70518=CARTESIAN_POINT('Ctrl Pts',(70.1278787078675,782.758355117418,108.46533673211));
#70519=CARTESIAN_POINT('Ctrl Pts',(70.3339499104518,782.645177411981,108.435015348839));
#70520=CARTESIAN_POINT('Ctrl Pts',(70.4224938188007,782.575529540903,108.41640815476));
#70521=CARTESIAN_POINT('Ctrl Pts',(70.5788384608645,782.403800346269,108.370809734002));
#70522=CARTESIAN_POINT('Ctrl Pts',(70.6428826418601,782.300835790732,108.343609142235));
#70523=CARTESIAN_POINT('Ctrl Pts',(70.7337278085516,782.068686347582,108.282720458236));
#70524=CARTESIAN_POINT('Ctrl Pts',(70.756201634141,781.940232393222,108.249260428266));
#70525=CARTESIAN_POINT('Ctrl Pts',(70.7492205034136,781.680447870711,108.182080885617));
#70526=CARTESIAN_POINT('Ctrl Pts',(70.7191587872933,781.551574287505,108.149001405295));
#70527=CARTESIAN_POINT('Ctrl Pts',(70.6125196859197,781.319341010621,108.089744252411));
#70528=CARTESIAN_POINT('Ctrl Pts',(70.5396356529601,781.216909345899,108.063778162935));
#70529=CARTESIAN_POINT('Ctrl Pts',(70.3668838768826,781.050843319014,108.021841613514));
#70530=CARTESIAN_POINT('Ctrl Pts',(70.2712145987063,780.985782176087,108.005491425853));
#70531=CARTESIAN_POINT('Ctrl Pts',(70.1249540501647,780.918778107505,107.988680456899));
#70532=CARTESIAN_POINT('Ctrl Pts',(70.0823247393464,780.902550520314,107.984613344889));
#70533=CARTESIAN_POINT('Ctrl Pts',(70.0100858773551,780.880366181054,107.979055333505));
#70534=CARTESIAN_POINT('Ctrl Pts',(69.981070662606,780.872807249459,107.977162193431));
#70535=CARTESIAN_POINT('Ctrl Pts',(69.9385231381707,780.863659801175,107.9748710505));
#70536=CARTESIAN_POINT('Ctrl Pts',(69.9252359670773,780.861072118211,107.97422289459));
#70537=CARTESIAN_POINT('Ctrl Pts',(69.8812466666154,780.85338880199,107.972298086294));
#70538=CARTESIAN_POINT('Ctrl Pts',(69.8503570209193,780.849403477812,107.971299120077));
#70539=CARTESIAN_POINT('Ctrl Pts',(69.7902241224452,780.844357945566,107.970031639992));
#70540=CARTESIAN_POINT('Ctrl Pts',(69.7610268792052,780.84313396907,107.9697220466));
#70541=CARTESIAN_POINT('Ctrl Pts',(69.7318153101166,780.843131484731,107.96971688462));
#70542=CARTESIAN_POINT('Ctrl Pts',(69.7316732616476,782.211734062764,110.227707202932));
#70543=CARTESIAN_POINT('Ctrl Pts',(69.7316954699837,782.211733961292,110.227707490037));
#70544=CARTESIAN_POINT('Ctrl Pts',(69.7317176783555,782.211733859126,110.227707776929));
#70545=CARTESIAN_POINT('Ctrl Pts',(69.7317398867631,782.211733756267,110.227708063609));
#70546=CARTESIAN_POINT('Ctrl Pts',(69.8622261603718,782.211129405869,110.229392460867));
#70547=CARTESIAN_POINT('Ctrl Pts',(69.9914866175043,782.186613743472,110.223694823434));
#70548=CARTESIAN_POINT('Ctrl Pts',(70.2371565191121,782.090835500069,110.198437316032));
#70549=CARTESIAN_POINT('Ctrl Pts',(70.3506491877387,782.019141974026,110.178736812215));
#70550=CARTESIAN_POINT('Ctrl Pts',(70.543227682407,781.836814223691,110.128355921939));
#70551=CARTESIAN_POINT('Ctrl Pts',(70.6200878658936,781.72766524519,110.098098321078));
#70552=CARTESIAN_POINT('Ctrl Pts',(70.7247209820805,781.488141554969,110.031897147834));
#70553=CARTESIAN_POINT('Ctrl Pts',(70.7520158281456,781.360305818121,109.996652313396));
#70554=CARTESIAN_POINT('Ctrl Pts',(70.7540837955846,781.102112045273,109.925362383202));
#70555=CARTESIAN_POINT('Ctrl Pts',(70.7289530754057,780.974189437589,109.889977778559));
#70556=CARTESIAN_POINT('Ctrl Pts',(70.6293282700264,780.735611054836,109.823162945647));
#70557=CARTESIAN_POINT('Ctrl Pts',(70.5559653922169,780.627143860887,109.792333028749));
#70558=CARTESIAN_POINT('Ctrl Pts',(70.3701780264163,780.444035907159,109.738572393098));
#70559=CARTESIAN_POINT('Ctrl Pts',(70.2596061933404,780.371134110865,109.71614292612));
#70560=CARTESIAN_POINT('Ctrl Pts',(70.014929907433,780.270740964709,109.682309327284));
#70561=CARTESIAN_POINT('Ctrl Pts',(69.8831882168743,780.244411879854,109.671279865138));
#70562=CARTESIAN_POINT('Ctrl Pts',(69.7437009133202,780.243426643835,109.666671384854));
#70563=CARTESIAN_POINT('Ctrl Pts',(69.7376858169251,780.243435762934,109.666486266887));
#70564=CARTESIAN_POINT('Ctrl Pts',(69.7316732616476,780.243496355298,109.666314827831));
#70565=CARTESIAN_POINT('Origin',(69.7316732616476,784.848060912957,99.7033802796288));
#70566=CARTESIAN_POINT('',(69.7316732616476,783.184644281451,105.910275523117));
#70567=CARTESIAN_POINT('Origin',(69.7316732616476,782.713222050842,105.74365895585));
#70568=CARTESIAN_POINT('',(69.7316732616477,781.712527445781,110.075459176648));
#70569=CARTESIAN_POINT('',(69.7316732616476,785.319483143566,99.8699968468959));
#70570=CARTESIAN_POINT('Ctrl Pts',(69.7316871691062,780.74901083613,109.800715486367));
#70571=CARTESIAN_POINT('Ctrl Pts',(69.671752121605,780.74953320695,109.799232496016));
#70572=CARTESIAN_POINT('Ctrl Pts',(69.6123290057934,780.760469738631,109.800621919992));
#70573=CARTESIAN_POINT('Ctrl Pts',(69.4947140649738,780.804060409493,109.809524830073));
#70574=CARTESIAN_POINT('Ctrl Pts',(69.4383492748769,780.838298428812,109.81753740878));
#70575=CARTESIAN_POINT('Ctrl Pts',(69.3418554820246,780.926088143699,109.839629880153));
#70576=CARTESIAN_POINT('Ctrl Pts',(69.3028556001647,780.97898794651,109.853562786702));
#70577=CARTESIAN_POINT('Ctrl Pts',(69.248306083352,781.096348059627,109.885619453726));
#70578=CARTESIAN_POINT('Ctrl Pts',(69.2333981377799,781.159700758797,109.903446295939));
#70579=CARTESIAN_POINT('Ctrl Pts',(69.2302393778081,781.287681037935,109.940384059098));
#70580=CARTESIAN_POINT('Ctrl Pts',(69.2418695451783,781.351037439978,109.959120308888));
#70581=CARTESIAN_POINT('Ctrl Pts',(69.2902265851311,781.469464002387,109.994878145109));
#70582=CARTESIAN_POINT('Ctrl Pts',(69.3264580649211,781.523358506002,110.011539592825));
#70583=CARTESIAN_POINT('Ctrl Pts',(69.4189546875642,781.614390712454,110.040336968888));
#70584=CARTESIAN_POINT('Ctrl Pts',(69.47433436397,781.650573234726,110.052168466974));
#70585=CARTESIAN_POINT('Ctrl Pts',(69.5967834155184,781.699943203055,110.069178647964));
#70586=CARTESIAN_POINT('Ctrl Pts',(69.6626225671268,781.712621277087,110.074181823424));
#70587=CARTESIAN_POINT('Ctrl Pts',(69.7956063968911,781.712452000456,110.076645244186));
#70588=CARTESIAN_POINT('Ctrl Pts',(69.8614120152285,781.699661409441,110.074100249503));
#70589=CARTESIAN_POINT('Ctrl Pts',(69.9840574489736,781.650163219912,110.061939433147));
#70590=CARTESIAN_POINT('Ctrl Pts',(70.0396784273824,781.61396764452,110.052455127742));
#70591=CARTESIAN_POINT('Ctrl Pts',(70.1333093264964,781.522674617827,110.027916585964));
#70592=CARTESIAN_POINT('Ctrl Pts',(70.1703088101643,781.468407055534,110.013086799895));
#70593=CARTESIAN_POINT('Ctrl Pts',(70.2198014414364,781.350076068002,109.98043089558));
#70594=CARTESIAN_POINT('Ctrl Pts',(70.2321756068971,781.287299512487,109.96296408948));
#70595=CARTESIAN_POINT('Ctrl Pts',(70.2311408101823,781.160963301958,109.927482256949));
#70596=CARTESIAN_POINT('Ctrl Pts',(70.2177973847371,781.098603084693,109.909801900932));
#70597=CARTESIAN_POINT('Ctrl Pts',(70.1670042938586,780.982688784419,109.876431007625));
#70598=CARTESIAN_POINT('Ctrl Pts',(70.1301132607978,780.93021566454,109.861049269477));
#70599=CARTESIAN_POINT('Ctrl Pts',(70.0374327039456,780.842138208812,109.834445527333));
#70600=CARTESIAN_POINT('Ctrl Pts',(69.9825676271291,780.807371885577,109.823474718377));
#70601=CARTESIAN_POINT('Ctrl Pts',(69.8617888039196,780.760268603994,109.80733304511));
#70602=CARTESIAN_POINT('Ctrl Pts',(69.7970484500052,780.748441172346,109.802332739593));
#70603=CARTESIAN_POINT('Ctrl Pts',(69.7316871691062,780.74901083613,109.800715486367));
#70604=CARTESIAN_POINT('Origin',(76.5148471080835,783.300361650383,99.1563709925214));
#70605=CARTESIAN_POINT('',(76.5148471080835,778.574131435236,109.683582026066));
#70606=CARTESIAN_POINT('',(76.5148471080829,780.458567154633,110.042007126776));
#70607=CARTESIAN_POINT('Ctrl Pts',(76.514847108083,778.574131435236,109.683582026066));
#70608=CARTESIAN_POINT('Ctrl Pts',(76.3993676990878,778.577277784233,109.674679796912));
#70609=CARTESIAN_POINT('Ctrl Pts',(76.2850892439373,778.601440476607,109.669618110618));
#70610=CARTESIAN_POINT('Ctrl Pts',(76.0594426807239,778.693156619548,109.667865902568));
#70611=CARTESIAN_POINT('Ctrl Pts',(75.9517734184118,778.763815415005,109.672078130935));
#70612=CARTESIAN_POINT('Ctrl Pts',(75.7681870593439,778.942824194081,109.690747962663));
#70613=CARTESIAN_POINT('Ctrl Pts',(75.6944842980661,779.050091998023,109.705201132879));
#70614=CARTESIAN_POINT('Ctrl Pts',(75.5942072843244,779.284079485405,109.742375593649));
#70615=CARTESIAN_POINT('Ctrl Pts',(75.5678813662372,779.408400063706,109.764643013575));
#70616=CARTESIAN_POINT('Ctrl Pts',(75.565727455983,779.657383154022,109.81371832909));
#70617=CARTESIAN_POINT('Ctrl Pts',(75.5892879813095,779.779671946231,109.839993287732));
#70618=CARTESIAN_POINT('Ctrl Pts',(75.683429476057,780.00682706611,109.892701961643));
#70619=CARTESIAN_POINT('Ctrl Pts',(75.7528306138902,780.109481613965,109.918588311159));
#70620=CARTESIAN_POINT('Ctrl Pts',(75.9290060646397,780.281540500099,109.966063702635));
#70621=CARTESIAN_POINT('Ctrl Pts',(76.0339230674475,780.34912793396,109.987141839437));
#70622=CARTESIAN_POINT('Ctrl Pts',(76.2653154207896,780.439483817083,110.021351270875));
#70623=CARTESIAN_POINT('Ctrl Pts',(76.3893196857779,780.46129526995,110.034120738728));
#70624=CARTESIAN_POINT('Ctrl Pts',(76.514424819782,780.458576425092,110.041980614868));
#70625=CARTESIAN_POINT('Ctrl Pts',(76.5145655843954,780.458573365928,110.041989458569));
#70626=CARTESIAN_POINT('Ctrl Pts',(76.5147063471654,780.458570275774,110.041998295872));
#70627=CARTESIAN_POINT('Ctrl Pts',(76.5148471080822,780.458567154633,110.042007126776));
#70628=CARTESIAN_POINT('',(76.5148471806244,781.109526725105,108.200192607479));
#70629=CARTESIAN_POINT('',(76.5148471080835,784.194257823002,99.4723041456579));
#70630=CARTESIAN_POINT('Ctrl Pts',(76.514831644203,779.24561539752,107.783696123679));
#70631=CARTESIAN_POINT('Ctrl Pts',(76.4180353514781,779.247364784066,107.778751175432));
#70632=CARTESIAN_POINT('Ctrl Pts',(76.3219311476675,779.263698487753,107.777022587367));
#70633=CARTESIAN_POINT('Ctrl Pts',(76.1279621245816,779.327377634286,107.780321234634));
#70634=CARTESIAN_POINT('Ctrl Pts',(76.0323909289794,779.377369947571,107.786062306385));
#70635=CARTESIAN_POINT('Ctrl Pts',(75.8546355067824,779.511324331408,107.805933942219));
#70636=CARTESIAN_POINT('Ctrl Pts',(75.7756668708024,779.596699549882,107.820568463536));
#70637=CARTESIAN_POINT('Ctrl Pts',(75.6476359593787,779.797628781069,107.858447778253));
#70638=CARTESIAN_POINT('Ctrl Pts',(75.6024452365978,779.913162559872,107.88192076001));
#70639=CARTESIAN_POINT('Ctrl Pts',(75.5594285117788,780.154853299432,107.934096117601));
#70640=CARTESIAN_POINT('Ctrl Pts',(75.5623603358809,780.278831393633,107.962349095975));
#70641=CARTESIAN_POINT('Ctrl Pts',(75.615458548658,780.509909590215,108.017692493094));
#70642=CARTESIAN_POINT('Ctrl Pts',(75.6620100400825,780.615617596105,108.044259935867));
#70643=CARTESIAN_POINT('Ctrl Pts',(75.7837114236965,780.791750850276,108.090821603474));
#70644=CARTESIAN_POINT('Ctrl Pts',(75.8533174078007,780.863847185439,108.110907193139));
#70645=CARTESIAN_POINT('Ctrl Pts',(75.9649093399525,780.946983095817,108.135617499223));
#70646=CARTESIAN_POINT('Ctrl Pts',(75.9978133672779,780.968393995628,108.142187591245));
#70647=CARTESIAN_POINT('Ctrl Pts',(76.0540770976014,781.000133229645,108.152294329216));
#70648=CARTESIAN_POINT('Ctrl Pts',(76.0766440693645,781.011680863023,108.156074323909));
#70649=CARTESIAN_POINT('Ctrl Pts',(76.1099870320813,781.027069544935,108.161271590755));
#70650=CARTESIAN_POINT('Ctrl Pts',(76.1203879333148,781.031642925937,108.162840226802));
#70651=CARTESIAN_POINT('Ctrl Pts',(76.1543808544028,781.045860726047,108.167797903732));
#70652=CARTESIAN_POINT('Ctrl Pts',(76.1783011256814,781.054744321638,108.17102661096));
#70653=CARTESIAN_POINT('Ctrl Pts',(76.2404182218449,781.074994282979,108.178757274167));
#70654=CARTESIAN_POINT('Ctrl Pts',(76.279055543525,781.084951373524,108.182953898065));
#70655=CARTESIAN_POINT('Ctrl Pts',(76.4259133199425,781.113121698612,108.196663471679));
#70656=CARTESIAN_POINT('Ctrl Pts',(76.5366332654775,781.115159364184,108.202549062815));
#70657=CARTESIAN_POINT('Ctrl Pts',(76.7467266245878,781.083119054231,108.205515526864));
#70658=CARTESIAN_POINT('Ctrl Pts',(76.8449287800089,781.051754027594,108.203161155164));
#70659=CARTESIAN_POINT('Ctrl Pts',(77.0362488598872,780.95546122091,108.190693288838));
#70660=CARTESIAN_POINT('Ctrl Pts',(77.1265272632014,780.888412414372,108.179972970967));
#70661=CARTESIAN_POINT('Ctrl Pts',(77.2858000956765,780.720658390469,108.150152757721));
#70662=CARTESIAN_POINT('Ctrl Pts',(77.3510998144554,780.619139837436,108.130710489576));
#70663=CARTESIAN_POINT('Ctrl Pts',(77.4423037104024,780.392593318821,108.084936330138));
#70664=CARTESIAN_POINT('Ctrl Pts',(77.4651733722019,780.268754142177,108.058732275219));
#70665=CARTESIAN_POINT('Ctrl Pts',(77.460423090042,780.024264504341,108.004686491891));
#70666=CARTESIAN_POINT('Ctrl Pts',(77.4344837795554,779.90582397136,107.977404578711));
#70667=CARTESIAN_POINT('Ctrl Pts',(77.3403426958463,779.691325828456,107.925588225535));
#70668=CARTESIAN_POINT('Ctrl Pts',(77.275167465429,779.59625590887,107.901421104215));
#70669=CARTESIAN_POINT('Ctrl Pts',(77.1485457300168,779.470552156053,107.867262620632));
#70670=CARTESIAN_POINT('Ctrl Pts',(77.0986714243861,779.43040869639,107.855840432614));
#70671=CARTESIAN_POINT('Ctrl Pts',(77.0197460740544,779.379395763315,107.840465230297));
#70672=CARTESIAN_POINT('Ctrl Pts',(76.9937825261499,779.364346051898,107.835781128276));
#70673=CARTESIAN_POINT('Ctrl Pts',(76.9559862388099,779.344816952569,107.829475585546));
#70674=CARTESIAN_POINT('Ctrl Pts',(76.9447478175009,779.339294036391,107.827661933166));
#70675=CARTESIAN_POINT('Ctrl Pts',(76.9233453499745,779.329305838269,107.824322280644));
#70676=CARTESIAN_POINT('Ctrl Pts',(76.913207592371,779.324792731181,107.822787417808));
#70677=CARTESIAN_POINT('Ctrl Pts',(76.8806247515721,779.310976754472,107.818003065628));
#70678=CARTESIAN_POINT('Ctrl Pts',(76.8578814781205,779.302359717227,107.814885052182));
#70679=CARTESIAN_POINT('Ctrl Pts',(76.7995339020959,779.282805479904,107.80743700553));
#70680=CARTESIAN_POINT('Ctrl Pts',(76.7635447008317,779.273070095954,107.803345164877));
#70681=CARTESIAN_POINT('Ctrl Pts',(76.6573892522873,779.250975576363,107.792708414698));
#70682=CARTESIAN_POINT('Ctrl Pts',(76.5862038497717,779.244325497125,107.787342253638));
#70683=CARTESIAN_POINT('Ctrl Pts',(76.514831644203,779.24561539752,107.783696123679));
#70684=CARTESIAN_POINT('Ctrl Pts',(76.5148471080822,780.458567154633,110.042007126776));
#70685=CARTESIAN_POINT('Ctrl Pts',(76.6337470667696,780.455930744863,110.049466542098));
#70686=CARTESIAN_POINT('Ctrl Pts',(76.75132498731,780.431190888614,110.052357661743));
#70687=CARTESIAN_POINT('Ctrl Pts',(76.9783672850955,780.33771267233,110.049168030248));
#70688=CARTESIAN_POINT('Ctrl Pts',(77.0846276507624,780.267360411898,110.042582133196));
#70689=CARTESIAN_POINT('Ctrl Pts',(77.2653867807146,780.089441577228,110.020720096866));
#70690=CARTESIAN_POINT('Ctrl Pts',(77.3376895014433,779.983064117638,110.005538897587));
#70691=CARTESIAN_POINT('Ctrl Pts',(77.4361924532665,779.750562444307,109.968984768886));
#70692=CARTESIAN_POINT('Ctrl Pts',(77.4619661878394,779.6266845279,109.947991738727));
#70693=CARTESIAN_POINT('Ctrl Pts',(77.4638292103386,779.378852369871,109.902888612438));
#70694=CARTESIAN_POINT('Ctrl Pts',(77.4406618765805,779.257087152449,109.879215104217));
#70695=CARTESIAN_POINT('Ctrl Pts',(77.3488465804086,779.031885320795,109.831856464833));
#70696=CARTESIAN_POINT('Ctrl Pts',(77.2818291751373,778.930277434427,109.808610358476));
#70697=CARTESIAN_POINT('Ctrl Pts',(77.1120683540937,778.759369035873,109.7648949071));
#70698=CARTESIAN_POINT('Ctrl Pts',(77.0112915204305,778.691632890328,109.74485262965));
#70699=CARTESIAN_POINT('Ctrl Pts',(76.7871998036966,778.598293118821,109.710176384091));
#70700=CARTESIAN_POINT('Ctrl Pts',(76.666119806469,778.57411896189,109.695974807137));
#70701=CARTESIAN_POINT('Ctrl Pts',(76.5338265306903,778.573756358675,109.685070457189));
#70702=CARTESIAN_POINT('Ctrl Pts',(76.5243327688691,778.573872989167,109.684313269209));
#70703=CARTESIAN_POINT('Ctrl Pts',(76.514847108083,778.574131435236,109.683582026066));
#70704=CARTESIAN_POINT('Origin',(76.5148471080835,783.300361650383,99.1563709925214));
#70705=CARTESIAN_POINT('',(76.5148471080835,781.636945018877,105.36326623601));
#70706=CARTESIAN_POINT('Origin',(76.5148471080835,781.165522788268,105.196649668743));
#70707=CARTESIAN_POINT('',(76.5148471080838,780.015385701083,109.951280040382));
#70708=CARTESIAN_POINT('',(76.5148471080835,783.771783880992,99.3229875597885));
#70709=CARTESIAN_POINT('Ctrl Pts',(76.5148947017357,779.021561102855,109.762289290823));
#70710=CARTESIAN_POINT('Ctrl Pts',(76.4518262861511,779.023201131602,109.757631004561));
#70711=CARTESIAN_POINT('Ctrl Pts',(76.3894985517755,779.036703118335,109.7552102727));
#70712=CARTESIAN_POINT('Ctrl Pts',(76.2689368492823,779.087240744129,109.755141278728));
#70713=CARTESIAN_POINT('Ctrl Pts',(76.2124402604689,779.125265246733,109.75782168149));
#70714=CARTESIAN_POINT('Ctrl Pts',(76.1168758251058,779.220851900717,109.768409205877));
#70715=CARTESIAN_POINT('Ctrl Pts',(76.0788657754288,779.277710086336,109.776270092476));
#70716=CARTESIAN_POINT('Ctrl Pts',(76.027540498281,779.401750848085,109.796090763673));
#70717=CARTESIAN_POINT('Ctrl Pts',(76.0144959120489,779.467728702121,109.807838553993));
#70718=CARTESIAN_POINT('Ctrl Pts',(76.0152094779895,779.599784913144,109.833544517842));
#70719=CARTESIAN_POINT('Ctrl Pts',(76.0287247659368,779.664607941793,109.847236327804));
#70720=CARTESIAN_POINT('Ctrl Pts',(76.080163032521,779.783187552507,109.874308836184));
#70721=CARTESIAN_POINT('Ctrl Pts',(76.1169069858755,779.836044195316,109.887420776371));
#70722=CARTESIAN_POINT('Ctrl Pts',(76.2090455817878,779.92425976037,109.911502582937));
#70723=CARTESIAN_POINT('Ctrl Pts',(76.2633930890826,779.958818427281,109.922236706845));
#70724=CARTESIAN_POINT('Ctrl Pts',(76.383161440213,780.005285055043,109.939955024941));
#70725=CARTESIAN_POINT('Ctrl Pts',(76.4473757677932,780.016618263657,109.946739816801));
#70726=CARTESIAN_POINT('Ctrl Pts',(76.5786960284056,780.014232887792,109.955579176616));
#70727=CARTESIAN_POINT('Ctrl Pts',(76.6444324708125,779.999885421406,109.957415725242));
#70728=CARTESIAN_POINT('Ctrl Pts',(76.7672110100923,779.946704481258,109.955807955404));
#70729=CARTESIAN_POINT('Ctrl Pts',(76.8229528836136,779.908243036874,109.952347864267));
#70730=CARTESIAN_POINT('Ctrl Pts',(76.9168486009974,779.812057440101,109.940668067622));
#70731=CARTESIAN_POINT('Ctrl Pts',(76.9539474521059,779.7550646679,109.932516521091));
#70732=CARTESIAN_POINT('Ctrl Pts',(77.0038949556281,779.630161429046,109.912606063472));
#70733=CARTESIAN_POINT('Ctrl Pts',(77.0161343447144,779.563326456839,109.901006232884));
#70734=CARTESIAN_POINT('Ctrl Pts',(77.0133936677518,779.431600469514,109.876304221486));
#70735=CARTESIAN_POINT('Ctrl Pts',(76.9993563813161,779.367890126478,109.863483506371));
#70736=CARTESIAN_POINT('Ctrl Pts',(76.9475114155277,779.25069328556,109.837969434959));
#70737=CARTESIAN_POINT('Ctrl Pts',(76.9105617769154,779.198180512831,109.825516779465));
#70738=CARTESIAN_POINT('Ctrl Pts',(76.8182338016144,779.110685050023,109.802360911615));
#70739=CARTESIAN_POINT('Ctrl Pts',(76.7639017167637,779.076515588863,109.791885825037));
#70740=CARTESIAN_POINT('Ctrl Pts',(76.6440547087193,779.030765133784,109.77413470203));
#70741=CARTESIAN_POINT('Ctrl Pts',(76.5797369607959,779.019874947149,109.767078594656));
#70742=CARTESIAN_POINT('Ctrl Pts',(76.5148947017357,779.021561102855,109.762289290823));
#70743=CARTESIAN_POINT('Origin',(49.8616909408951,789.819881063962,101.460589746734));
#70744=CARTESIAN_POINT('',(49.8616909408951,787.691049283091,112.134283288743));
#70745=CARTESIAN_POINT('Origin',(49.8616909408951,786.229950467293,111.617881529726));
#70746=CARTESIAN_POINT('',(49.8616909408921,788.356889677166,110.250365206929));
#70747=CARTESIAN_POINT('',(49.8616909408951,791.28097987976,101.976991505752));
#70748=CARTESIAN_POINT('Ctrl Pts',(49.8617079781007,785.404291899084,109.303575373784));
#70749=CARTESIAN_POINT('Ctrl Pts',(49.7676926679438,785.404362943854,109.30337125909));
#70750=CARTESIAN_POINT('Ctrl Pts',(49.6738757965654,785.412651079779,109.305592005123));
#70751=CARTESIAN_POINT('Ctrl Pts',(49.4535286376546,785.45172627305,109.316630690403));
#70752=CARTESIAN_POINT('Ctrl Pts',(49.3291213344782,785.489761649913,109.327604661277));
#70753=CARTESIAN_POINT('Ctrl Pts',(49.0241319985413,785.625342980891,109.367331509502));
#70754=CARTESIAN_POINT('Ctrl Pts',(48.8562818266121,785.743328335843,109.402334396085));
#70755=CARTESIAN_POINT('Ctrl Pts',(48.5927373548287,786.019828245371,109.486021720799));
#70756=CARTESIAN_POINT('Ctrl Pts',(48.4935087823663,786.170739513764,109.532284505719));
#70757=CARTESIAN_POINT('Ctrl Pts',(48.3512585319294,786.507867112647,109.637402838476));
#70758=CARTESIAN_POINT('Ctrl Pts',(48.3131258693887,786.692615778466,109.695909053814));
#70759=CARTESIAN_POINT('Ctrl Pts',(48.3109094764101,787.07419402014,109.818734075163));
#70760=CARTESIAN_POINT('Ctrl Pts',(48.3504748358042,787.267409522545,109.881982780353));
#70761=CARTESIAN_POINT('Ctrl Pts',(48.5055399820578,787.625379184826,110.000744981419));
#70762=CARTESIAN_POINT('Ctrl Pts',(48.6186335944683,787.786982634862,110.055173428279));
#70763=CARTESIAN_POINT('Ctrl Pts',(48.8962360723346,788.05206050288,110.145208205056));
#70764=CARTESIAN_POINT('Ctrl Pts',(49.0551921775635,788.15595017432,110.180888215185));
#70765=CARTESIAN_POINT('Ctrl Pts',(49.3352507605499,788.274117089113,110.221619234482));
#70766=CARTESIAN_POINT('Ctrl Pts',(49.4452666326186,788.30724323978,110.233086243973));
#70767=CARTESIAN_POINT('Ctrl Pts',(49.6057395464989,788.337526862762,110.243593015385));
#70768=CARTESIAN_POINT('Ctrl Pts',(49.653754051446,788.344389614199,110.245979085644));
#70769=CARTESIAN_POINT('Ctrl Pts',(49.7453512028576,788.353348125892,110.24910349082));
#70770=CARTESIAN_POINT('Ctrl Pts',(49.7888422204462,788.355856881116,110.249984436697));
#70771=CARTESIAN_POINT('Ctrl Pts',(49.9254329935966,788.3582845325,110.250868019599));
#70772=CARTESIAN_POINT('Ctrl Pts',(50.0184483895708,788.35201288507,110.248730998659));
#70773=CARTESIAN_POINT('Ctrl Pts',(50.2366629592677,788.318458684918,110.237233788291));
#70774=CARTESIAN_POINT('Ctrl Pts',(50.359990076467,788.284298710163,110.225504745927));
#70775=CARTESIAN_POINT('Ctrl Pts',(50.6665356503412,788.158695640584,110.1825522443));
#70776=CARTESIAN_POINT('Ctrl Pts',(50.8373902774286,788.046281950615,110.144231210847));
#70777=CARTESIAN_POINT('Ctrl Pts',(51.1071657268225,787.779712973997,110.054512603112));
#70778=CARTESIAN_POINT('Ctrl Pts',(51.2097362504084,787.633520136832,110.005711544725));
#70779=CARTESIAN_POINT('Ctrl Pts',(51.3602314613403,787.304549943211,109.897343739963));
#70780=CARTESIAN_POINT('Ctrl Pts',(51.4034506949656,787.123097039,109.838301729158));
#70781=CARTESIAN_POINT('Ctrl Pts',(51.4177260726775,786.742509044268,109.716247190298));
#70782=CARTESIAN_POINT('Ctrl Pts',(51.3839977191523,786.546761045433,109.654435255415));
#70783=CARTESIAN_POINT('Ctrl Pts',(51.2392011316539,786.180937203769,109.540429527722));
#70784=CARTESIAN_POINT('Ctrl Pts',(51.1304148323752,786.014132992575,109.489219371059));
#70785=CARTESIAN_POINT('Ctrl Pts',(50.8554263874236,785.733905823956,109.403839258539));
#70786=CARTESIAN_POINT('Ctrl Pts',(50.6933678422754,785.621739854714,109.370007790432));
#70787=CARTESIAN_POINT('Ctrl Pts',(50.405460289627,785.493805216268,109.331324617886));
#70788=CARTESIAN_POINT('Ctrl Pts',(50.2918449324859,785.457865663585,109.320428626121));
#70789=CARTESIAN_POINT('Ctrl Pts',(50.1260492019831,785.425118040149,109.310356501147));
#70790=CARTESIAN_POINT('Ctrl Pts',(50.0765905941517,785.417724363462,109.308055221418));
#70791=CARTESIAN_POINT('Ctrl Pts',(49.9995534843385,785.409853193075,109.305547076538));
#70792=CARTESIAN_POINT('Ctrl Pts',(49.9721902681169,785.40776168142,109.304864181674));
#70793=CARTESIAN_POINT('Ctrl Pts',(49.9171162080564,785.404963658094,109.303906357104));
#70794=CARTESIAN_POINT('Ctrl Pts',(49.8894145804647,785.404270961971,109.303635527015));
#70795=CARTESIAN_POINT('Ctrl Pts',(49.8617079781007,785.404291899084,109.303575373784));
#70796=CARTESIAN_POINT('Origin',(49.8616909408951,789.819881063962,101.460589746734));
#70797=CARTESIAN_POINT('',(49.8616909408951,788.156464432456,107.667484990223));
#70798=CARTESIAN_POINT('Origin',(49.8616909408951,787.685042201847,107.500868422956));
#70799=CARTESIAN_POINT('',(49.8616909408951,786.701372697902,111.784498096993));
#70800=CARTESIAN_POINT('',(49.8616909408951,790.291303294571,101.627206314001));
#70801=CARTESIAN_POINT('Origin',(49.8616909408951,786.229950467293,111.617881529726));
#70802=CARTESIAN_POINT('Origin',(54.4787875961369,785.995601683377,100.108960015908));
#70803=CARTESIAN_POINT('',(54.4787875961369,783.593052663671,110.685912624258));
#70804=CARTESIAN_POINT('Origin',(54.4787875961369,782.405671086709,110.266251798899));
#70805=CARTESIAN_POINT('',(54.478787593146,784.202196751102,108.962410158872));
#70806=CARTESIAN_POINT('',(54.4787875961369,787.182983260339,100.528620841266));
#70807=CARTESIAN_POINT('Ctrl Pts',(54.4787613439502,781.7532554678,108.332966912952));
#70808=CARTESIAN_POINT('Ctrl Pts',(54.441743110491,781.753222920922,108.333061316267));
#70809=CARTESIAN_POINT('Ctrl Pts',(54.404743397955,781.754788427287,108.333532251668));
#70810=CARTESIAN_POINT('Ctrl Pts',(54.2822477200637,781.765282273289,108.336343481529));
#70811=CARTESIAN_POINT('Ctrl Pts',(54.19764331156,781.78117975144,108.340322846354));
#70812=CARTESIAN_POINT('Ctrl Pts',(53.9948553830075,781.840822325286,108.354981136571));
#70813=CARTESIAN_POINT('Ctrl Pts',(53.8805354429768,781.893729811182,108.367826941627));
#70814=CARTESIAN_POINT('Ctrl Pts',(53.6368509780762,782.053722918414,108.406735456799));
#70815=CARTESIAN_POINT('Ctrl Pts',(53.5177635875451,782.171407049685,108.435400678503));
#70816=CARTESIAN_POINT('Ctrl Pts',(53.3414506216402,782.433570469098,108.500102041471));
#70817=CARTESIAN_POINT('Ctrl Pts',(53.2813799982236,782.572883340683,108.53481473864));
#70818=CARTESIAN_POINT('Ctrl Pts',(53.2137683839407,782.873756350904,108.61085716836));
#70819=CARTESIAN_POINT('Ctrl Pts',(53.2101006971323,783.033403080544,108.651770527474));
#70820=CARTESIAN_POINT('Ctrl Pts',(53.2661104858377,783.348621422983,108.733700125082));
#70821=CARTESIAN_POINT('Ctrl Pts',(53.3267536550586,783.500952144515,108.773896898691));
#70822=CARTESIAN_POINT('Ctrl Pts',(53.504303031476,783.771396303741,108.846012919171));
#70823=CARTESIAN_POINT('Ctrl Pts',(53.6185214866455,783.887464323063,108.877357309535));
#70824=CARTESIAN_POINT('Ctrl Pts',(53.8606944177274,784.052893312023,108.922203052909));
#70825=CARTESIAN_POINT('Ctrl Pts',(53.9801599983939,784.109783748746,108.937697650171));
#70826=CARTESIAN_POINT('Ctrl Pts',(54.1913981916706,784.173035287721,108.954822938411));
#70827=CARTESIAN_POINT('Ctrl Pts',(54.2787172502997,784.189691046238,108.959292271416));
#70828=CARTESIAN_POINT('Ctrl Pts',(54.4058424335231,784.200693360855,108.962121681923));
#70829=CARTESIAN_POINT('Ctrl Pts',(54.4446999649238,784.202311169321,108.962502321777));
#70830=CARTESIAN_POINT('Ctrl Pts',(54.5201306433969,784.202077402492,108.962303774754));
#70831=CARTESIAN_POINT('Ctrl Pts',(54.556665812149,784.200426679941,108.961780463746));
#70832=CARTESIAN_POINT('Ctrl Pts',(54.6774398422457,784.189866283269,108.958633295975));
#70833=CARTESIAN_POINT('Ctrl Pts',(54.7608095113816,784.174286626917,108.954157454479));
#70834=CARTESIAN_POINT('Ctrl Pts',(54.9624804209552,784.115736682213,108.937574207204));
#70835=CARTESIAN_POINT('Ctrl Pts',(55.0768886143016,784.063463607035,108.922906058606));
#70836=CARTESIAN_POINT('Ctrl Pts',(55.3206565963673,783.905198823348,108.878991328144));
#70837=CARTESIAN_POINT('Ctrl Pts',(55.4397708406798,783.788705596441,108.846964888092));
#70838=CARTESIAN_POINT('Ctrl Pts',(55.615563991354,783.529311797718,108.776827455255));
#70839=CARTESIAN_POINT('Ctrl Pts',(55.6753801870606,783.391838660484,108.740105558444));
#70840=CARTESIAN_POINT('Ctrl Pts',(55.7433455670921,783.093937032578,108.661830405782));
#70841=CARTESIAN_POINT('Ctrl Pts',(55.747541805163,782.935359102455,108.620847036898));
#70842=CARTESIAN_POINT('Ctrl Pts',(55.6931651547547,782.619842413916,108.540746426938));
#70843=CARTESIAN_POINT('Ctrl Pts',(55.6330277655128,782.466165913169,108.502504324794));
#70844=CARTESIAN_POINT('Ctrl Pts',(55.4562033671363,782.192596973632,108.435558693061));
#70845=CARTESIAN_POINT('Ctrl Pts',(55.3421455779861,782.074729036396,108.407314164759));
#70846=CARTESIAN_POINT('Ctrl Pts',(55.102262000797,781.907952451745,108.367912857511));
#70847=CARTESIAN_POINT('Ctrl Pts',(54.9854616312421,781.85073328133,108.354635429623));
#70848=CARTESIAN_POINT('Ctrl Pts',(54.7769126032848,781.785401373428,108.339727471207));
#70849=CARTESIAN_POINT('Ctrl Pts',(54.6894493740972,781.767693079593,108.335791010007));
#70850=CARTESIAN_POINT('Ctrl Pts',(54.56023897283,781.755263741237,108.333215484316));
#70851=CARTESIAN_POINT('Ctrl Pts',(54.5195130740058,781.753291297213,108.332862988533));
#70852=CARTESIAN_POINT('Ctrl Pts',(54.4787613439502,781.7532554678,108.332966912952));
#70853=CARTESIAN_POINT('Origin',(54.4787875961369,785.995601683377,100.108960015908));
#70854=CARTESIAN_POINT('',(54.4787875961369,784.332185051871,106.315855259396));
#70855=CARTESIAN_POINT('Origin',(54.4787875961369,783.860762821262,106.149238692129));
#70856=CARTESIAN_POINT('',(54.4787875961369,782.877093317318,110.432868366167));
#70857=CARTESIAN_POINT('',(54.4787875961369,786.467023913986,100.275576583175));
#70858=CARTESIAN_POINT('Origin',(54.4787875961369,782.405671086709,110.266251798899));
#70859=CARTESIAN_POINT('Origin',(59.5586600728479,782.515804719233,98.8790820269056));
#70860=CARTESIAN_POINT('',(59.5586600728479,777.909975348877,108.845595215772));
#70861=CARTESIAN_POINT('',(59.5586600728476,779.880261212077,109.401192572043));
#70862=CARTESIAN_POINT('Ctrl Pts',(59.5586600728479,777.909975348877,108.845595215772));
#70863=CARTESIAN_POINT('Ctrl Pts',(59.4291990673829,777.91049817199,108.844115948479));
#70864=CARTESIAN_POINT('Ctrl Pts',(59.3009284172275,777.934959562234,108.848763253711));
#70865=CARTESIAN_POINT('Ctrl Pts',(59.0556946989573,778.030849155894,108.870598307995));
#70866=CARTESIAN_POINT('Ctrl Pts',(58.9418416420412,778.103121953752,108.88806442479));
#70867=CARTESIAN_POINT('Ctrl Pts',(58.74928633604,778.285885134678,108.934346625436));
#70868=CARTESIAN_POINT('Ctrl Pts',(58.6724738350208,778.394655560504,108.962745613571));
#70869=CARTESIAN_POINT('Ctrl Pts',(58.5662614311178,778.635055050951,109.027613408059));
#70870=CARTESIAN_POINT('Ctrl Pts',(58.5382704963566,778.764520150491,109.063524881249));
#70871=CARTESIAN_POINT('Ctrl Pts',(58.5362892225246,779.025665920847,109.137955372544));
#70872=CARTESIAN_POINT('Ctrl Pts',(58.5622340711796,779.154770996146,109.175734907046));
#70873=CARTESIAN_POINT('Ctrl Pts',(58.6646293609599,779.394225107181,109.247313761704));
#70874=CARTESIAN_POINT('Ctrl Pts',(58.7396089284805,779.502385677257,109.280427829676));
#70875=CARTESIAN_POINT('Ctrl Pts',(58.9290740373455,779.684475554637,109.337061172406));
#70876=CARTESIAN_POINT('Ctrl Pts',(59.0416896628259,779.756621160249,109.360005194922));
#70877=CARTESIAN_POINT('Ctrl Pts',(59.2900609887602,779.855132045876,109.391905804919));
#70878=CARTESIAN_POINT('Ctrl Pts',(59.4234209987155,779.880427292854,109.400506321648));
#70879=CARTESIAN_POINT('Ctrl Pts',(59.5581144817012,779.880262020816,109.401189846532));
#70880=CARTESIAN_POINT('Ctrl Pts',(59.5582963477946,779.880261797662,109.401190769442));
#70881=CARTESIAN_POINT('Ctrl Pts',(59.5584782115162,779.880261528082,109.401191677945));
#70882=CARTESIAN_POINT('Ctrl Pts',(59.5586600728473,779.880261212077,109.401192572043));
#70883=CARTESIAN_POINT('',(59.5586599619933,780.382502020465,107.980160521771));
#70884=CARTESIAN_POINT('',(59.5586600728479,783.478833859476,99.2194491099729));
#70885=CARTESIAN_POINT('Ctrl Pts',(59.5585491494349,778.363426758698,107.562607121697));
#70886=CARTESIAN_POINT('Ctrl Pts',(59.5294255770194,778.363280482099,107.563030485534));
#70887=CARTESIAN_POINT('Ctrl Pts',(59.5003138937717,778.364372249146,107.563688873113));
#70888=CARTESIAN_POINT('Ctrl Pts',(59.4015656073238,778.372291690413,107.56672194487));
#70889=CARTESIAN_POINT('Ctrl Pts',(59.3326533420484,778.384994224227,107.570198769266));
#70890=CARTESIAN_POINT('Ctrl Pts',(59.1636091293877,778.434441252366,107.582209556769));
#70891=CARTESIAN_POINT('Ctrl Pts',(59.0671044538631,778.479949504058,107.592353971292));
#70892=CARTESIAN_POINT('Ctrl Pts',(58.8827141924712,778.605073588118,107.619175068383));
#70893=CARTESIAN_POINT('Ctrl Pts',(58.7982697036429,778.686824389758,107.636226209408));
#70894=CARTESIAN_POINT('Ctrl Pts',(58.6572472071341,778.880408884885,107.676181399548));
#70895=CARTESIAN_POINT('Ctrl Pts',(58.6037710511383,778.992165009854,107.699055336428));
#70896=CARTESIAN_POINT('Ctrl Pts',(58.5378796772744,779.236225650972,107.749029077805));
#70897=CARTESIAN_POINT('Ctrl Pts',(58.5288235093464,779.367247621908,107.775874454381));
#70898=CARTESIAN_POINT('Ctrl Pts',(58.561979389092,779.629633019458,107.829819050094));
#70899=CARTESIAN_POINT('Ctrl Pts',(58.6055834773226,779.758412562268,107.856393029058));
#70900=CARTESIAN_POINT('Ctrl Pts',(58.7400981352003,779.989310878681,107.90400057502));
#70901=CARTESIAN_POINT('Ctrl Pts',(58.8287469694599,780.089759546732,107.924681723633));
#70902=CARTESIAN_POINT('Ctrl Pts',(59.0252516290962,780.239845227271,107.955078134323));
#70903=CARTESIAN_POINT('Ctrl Pts',(59.1270603864985,780.293646593864,107.965721056196));
#70904=CARTESIAN_POINT('Ctrl Pts',(59.3057541081849,780.352904596454,107.976669592383));
#70905=CARTESIAN_POINT('Ctrl Pts',(59.3779718308474,780.368590782434,107.979278478185));
#70906=CARTESIAN_POINT('Ctrl Pts',(59.4828077019629,780.379908954376,107.98051405783));
#70907=CARTESIAN_POINT('Ctrl Pts',(59.5144794615612,780.381868619709,107.98056231909));
#70908=CARTESIAN_POINT('Ctrl Pts',(59.575358043458,780.382844540222,107.98003169514));
#70909=CARTESIAN_POINT('Ctrl Pts',(59.6045295458972,780.382083679894,107.979503034302));
#70910=CARTESIAN_POINT('Ctrl Pts',(59.6983456308999,780.375675157192,107.976916910588));
#70911=CARTESIAN_POINT('Ctrl Pts',(59.7624609963608,780.365199776645,107.973785596302));
#70912=CARTESIAN_POINT('Ctrl Pts',(59.9149854483869,780.325301462213,107.962995276125));
#70913=CARTESIAN_POINT('Ctrl Pts',(60.0010793251777,780.289815471754,107.954011127531));
#70914=CARTESIAN_POINT('Ctrl Pts',(60.1978052761289,780.175483739639,107.926179956891));
#70915=CARTESIAN_POINT('Ctrl Pts',(60.2993869198372,780.085379168819,107.904985883879));
#70916=CARTESIAN_POINT('Ctrl Pts',(60.4529183290253,779.881546509522,107.858559180971));
#70917=CARTESIAN_POINT('Ctrl Pts',(60.5073867157846,779.772539579672,107.834288910627));
#70918=CARTESIAN_POINT('Ctrl Pts',(60.5767321158997,779.532917109774,107.782308502156));
#70919=CARTESIAN_POINT('Ctrl Pts',(60.5880863263182,779.40348322835,107.754948412995));
#70920=CARTESIAN_POINT('Ctrl Pts',(60.5603355536008,779.141304299766,107.701103856231));
#70921=CARTESIAN_POINT('Ctrl Pts',(60.5191745110486,779.011132679903,107.675221898375));
#70922=CARTESIAN_POINT('Ctrl Pts',(60.3890230476198,778.776360454652,107.630087794799));
#70923=CARTESIAN_POINT('Ctrl Pts',(60.3022131966845,778.673409220668,107.611109854969));
#70924=CARTESIAN_POINT('Ctrl Pts',(60.1106674953454,778.520005118074,107.584107313255));
#70925=CARTESIAN_POINT('Ctrl Pts',(60.0125986298598,778.464686810371,107.574958497107));
#70926=CARTESIAN_POINT('Ctrl Pts',(59.8387978799252,778.401096831037,107.565444890544));
#70927=CARTESIAN_POINT('Ctrl Pts',(59.7677184226025,778.38333941888,107.563158622208));
#70928=CARTESIAN_POINT('Ctrl Pts',(59.6500013167806,778.366942132872,107.561858168359));
#70929=CARTESIAN_POINT('Ctrl Pts',(59.6043070376603,778.363656583124,107.561941947973));
#70930=CARTESIAN_POINT('Ctrl Pts',(59.5585491494349,778.363426758698,107.562607121697));
#70931=CARTESIAN_POINT('Ctrl Pts',(59.5586600728473,779.880261212077,109.401192572043));
#70932=CARTESIAN_POINT('Ctrl Pts',(59.6914009222063,779.880030560098,109.401845175036));
#70933=CARTESIAN_POINT('Ctrl Pts',(59.8228682597227,779.855074343606,109.394801961274));
#70934=CARTESIAN_POINT('Ctrl Pts',(60.069947360309,779.757802072863,109.366432215607));
#70935=CARTESIAN_POINT('Ctrl Pts',(60.1829276319018,779.685886859264,109.345235094438));
#70936=CARTESIAN_POINT('Ctrl Pts',(60.3739939760634,779.503559113016,109.292043017165));
#70937=CARTESIAN_POINT('Ctrl Pts',(60.4499691725986,779.394731015658,109.260531934029));
#70938=CARTESIAN_POINT('Ctrl Pts',(60.5531420895566,779.155699974923,109.192357702164));
#70939=CARTESIAN_POINT('Ctrl Pts',(60.5797286821778,779.027987850295,109.156404113416));
#70940=CARTESIAN_POINT('Ctrl Pts',(60.5804013048047,778.769831416606,109.084656777137));
#70941=CARTESIAN_POINT('Ctrl Pts',(60.5545203707955,778.641837121719,109.049536430204));
#70942=CARTESIAN_POINT('Ctrl Pts',(60.4534436120453,778.403052677336,108.984414894268));
#70943=CARTESIAN_POINT('Ctrl Pts',(60.3793731555848,778.294441897652,108.954991469578));
#70944=CARTESIAN_POINT('Ctrl Pts',(60.1924972720798,778.111184060679,108.905023096645));
#70945=CARTESIAN_POINT('Ctrl Pts',(60.081585500179,778.038190504168,108.884915276922));
#70946=CARTESIAN_POINT('Ctrl Pts',(59.8367167955085,777.937641500065,108.856116983007));
#70947=CARTESIAN_POINT('Ctrl Pts',(59.7051391273397,777.911150010299,108.847721080187));
#70948=CARTESIAN_POINT('Ctrl Pts',(59.5675001500342,777.90996754457,108.845703368576));
#70949=CARTESIAN_POINT('Ctrl Pts',(59.5630794180022,777.909957501527,108.845645712775));
#70950=CARTESIAN_POINT('Ctrl Pts',(59.558660072848,777.909975348877,108.845595215772));
#70951=CARTESIAN_POINT('Origin',(59.5586600728479,782.515804719233,98.8790820269056));
#70952=CARTESIAN_POINT('',(59.5586600728479,780.852388087727,105.085977270394));
#70953=CARTESIAN_POINT('Origin',(59.5586600728479,780.380965857118,104.919360703127));
#70954=CARTESIAN_POINT('',(59.558660072848,779.380861865021,109.249489853121));
#70955=CARTESIAN_POINT('',(59.5586600728479,782.987226949842,99.0456985941727));
#70956=CARTESIAN_POINT('Ctrl Pts',(59.5586513681714,778.416331464684,108.977614565517));
#70957=CARTESIAN_POINT('Ctrl Pts',(59.497472789011,778.416545597769,108.977011897015));
#70958=CARTESIAN_POINT('Ctrl Pts',(59.4368314718854,778.427633987372,108.979335555447));
#70959=CARTESIAN_POINT('Ctrl Pts',(59.3183791845843,778.471987852838,108.990062024086));
#70960=CARTESIAN_POINT('Ctrl Pts',(59.2622836940566,778.506410872123,108.998802932055));
#70961=CARTESIAN_POINT('Ctrl Pts',(59.1669241754906,778.594167519378,109.02182532098));
#70962=CARTESIAN_POINT('Ctrl Pts',(59.1286095049931,778.646682464612,109.035897096814));
#70963=CARTESIAN_POINT('Ctrl Pts',(59.074886361842,778.763389551699,109.067824769961));
#70964=CARTESIAN_POINT('Ctrl Pts',(59.060231889012,778.826552703242,109.085407716669));
#70965=CARTESIAN_POINT('Ctrl Pts',(59.057321262279,778.954806178108,109.121715105653));
#70966=CARTESIAN_POINT('Ctrl Pts',(59.0692085890005,779.018633408671,109.140083886269));
#70967=CARTESIAN_POINT('Ctrl Pts',(59.1181801789798,779.137561600903,109.174798604849));
#70968=CARTESIAN_POINT('Ctrl Pts',(59.1546307622503,779.191532000205,109.190807514258));
#70969=CARTESIAN_POINT('Ctrl Pts',(59.2473241610817,779.282497734407,109.218149449029));
#70970=CARTESIAN_POINT('Ctrl Pts',(59.3026112008437,779.318612197079,109.229212283854));
#70971=CARTESIAN_POINT('Ctrl Pts',(59.4247318917649,779.367997348572,109.24469659038));
#70972=CARTESIAN_POINT('Ctrl Pts',(59.4903466069188,779.380766024055,109.248958240076));
#70973=CARTESIAN_POINT('Ctrl Pts',(59.6229829252642,779.380959468382,109.249992585328));
#70974=CARTESIAN_POINT('Ctrl Pts',(59.688676245608,779.368388609669,109.246758112561));
#70975=CARTESIAN_POINT('Ctrl Pts',(59.8112001817466,779.319349655604,109.233282829004));
#70976=CARTESIAN_POINT('Ctrl Pts',(59.8668001735035,779.283359637815,109.223177490479));
#70977=CARTESIAN_POINT('Ctrl Pts',(59.9603943689052,779.192424348506,109.197553856238));
#70978=CARTESIAN_POINT('Ctrl Pts',(59.99737193986,779.138308193386,109.182273464386));
#70979=CARTESIAN_POINT('Ctrl Pts',(60.04683244192,779.020164775574,109.149016356485));
#70980=CARTESIAN_POINT('Ctrl Pts',(60.0591832290489,778.957427159715,109.131403066181));
#70981=CARTESIAN_POINT('Ctrl Pts',(60.0581036627097,778.831005763246,109.096013690838));
#70982=CARTESIAN_POINT('Ctrl Pts',(60.0447172790343,778.768524164436,109.078572531174));
#70983=CARTESIAN_POINT('Ctrl Pts',(59.9938306790339,778.652266775422,109.046097033671));
#70984=CARTESIAN_POINT('Ctrl Pts',(59.9568864010481,778.599567405004,109.031359754466));
#70985=CARTESIAN_POINT('Ctrl Pts',(59.8641507641302,778.511006684921,109.00637202405));
#70986=CARTESIAN_POINT('Ctrl Pts',(59.8092933253543,778.475960331079,108.996348291178));
#70987=CARTESIAN_POINT('Ctrl Pts',(59.6886015082836,778.428265112025,108.982220333221));
#70988=CARTESIAN_POINT('Ctrl Pts',(59.6239434182865,778.416102933908,108.978257755708));
#70989=CARTESIAN_POINT('Ctrl Pts',(59.5586513681714,778.416331464684,108.977614565517));
#70990=CARTESIAN_POINT('Origin',(65.8523138277871,779.672231777069,97.874067134449));
#70991=CARTESIAN_POINT('',(65.8523138277871,774.942544771236,108.411058755856));
#70992=CARTESIAN_POINT('',(65.852313827786,776.834453268023,108.748340500639));
#70993=CARTESIAN_POINT('Ctrl Pts',(65.8523138277871,774.942544771236,108.411058755856));
#70994=CARTESIAN_POINT('Ctrl Pts',(65.7322417836214,774.944350535709,108.405949554955));
#70995=CARTESIAN_POINT('Ctrl Pts',(65.6135118178383,774.969019786884,108.404584777808));
#70996=CARTESIAN_POINT('Ctrl Pts',(65.3853653172308,775.063262639199,108.409857329762));
#70997=CARTESIAN_POINT('Ctrl Pts',(65.2791432926612,775.134129844452,108.416871158307));
#70998=CARTESIAN_POINT('Ctrl Pts',(65.0979365589389,775.314037132206,108.439338683121));
#70999=CARTESIAN_POINT('Ctrl Pts',(65.0255044176019,775.422226128488,108.454787173952));
#71000=CARTESIAN_POINT('Ctrl Pts',(64.9281324361108,775.658118649035,108.492073344462));
#71001=CARTESIAN_POINT('Ctrl Pts',(64.9035127580602,775.783470088651,108.513505234639));
#71002=CARTESIAN_POINT('Ctrl Pts',(64.9049679604501,776.033966376516,108.55933217769));
#71003=CARTESIAN_POINT('Ctrl Pts',(64.9303580011618,776.156810587794,108.583261877123));
#71004=CARTESIAN_POINT('Ctrl Pts',(65.0278868846264,776.384516462656,108.630174509819));
#71005=CARTESIAN_POINT('Ctrl Pts',(65.0987870954147,776.487254818492,108.652691131115));
#71006=CARTESIAN_POINT('Ctrl Pts',(65.2758838720473,776.657576442914,108.692440836573));
#71007=CARTESIAN_POINT('Ctrl Pts',(65.3796166526574,776.724077517478,108.709354965747));
#71008=CARTESIAN_POINT('Ctrl Pts',(65.6073879296887,776.813617520162,108.735323355696));
#71009=CARTESIAN_POINT('Ctrl Pts',(65.7290366671221,776.835873364083,108.744131991536));
#71010=CARTESIAN_POINT('Ctrl Pts',(65.8518246149033,776.834459028229,108.748323824041));
#71011=CARTESIAN_POINT('Ctrl Pts',(65.8519876882831,776.834457149864,108.748329391169));
#71012=CARTESIAN_POINT('Ctrl Pts',(65.8521507592488,776.834455229794,108.748334950035));
#71013=CARTESIAN_POINT('Ctrl Pts',(65.8523138277848,776.834453268023,108.748340500639));
#71014=CARTESIAN_POINT('',(65.852313813786,777.362147432391,107.255291135104));
#71015=CARTESIAN_POINT('',(65.8523138277871,780.566127949688,98.1900002875857));
#71016=CARTESIAN_POINT('Ctrl Pts',(65.8521676736201,775.46727685438,106.926390289016));
#71017=CARTESIAN_POINT('Ctrl Pts',(65.7938787655703,775.466892120574,106.92750581374));
#71018=CARTESIAN_POINT('Ctrl Pts',(65.7357126515191,775.471900601344,106.929492713395));
#71019=CARTESIAN_POINT('Ctrl Pts',(65.5552275269776,775.504466933521,106.938413702626));
#71020=CARTESIAN_POINT('Ctrl Pts',(65.4380309142196,775.550962449721,106.948301620205));
#71021=CARTESIAN_POINT('Ctrl Pts',(65.2435008496011,775.67720993831,106.972787148368));
#71022=CARTESIAN_POINT('Ctrl Pts',(65.1644084907303,775.750431692209,106.986348712562));
#71023=CARTESIAN_POINT('Ctrl Pts',(65.0290659387499,775.926769111364,107.018172304209));
#71024=CARTESIAN_POINT('Ctrl Pts',(64.976321495565,776.030372562027,107.036468342364));
#71025=CARTESIAN_POINT('Ctrl Pts',(64.9081731126887,776.259472346272,107.076464727966));
#71026=CARTESIAN_POINT('Ctrl Pts',(64.8965411565285,776.384020337214,107.097972551109));
#71027=CARTESIAN_POINT('Ctrl Pts',(64.9220490607854,776.632915868686,107.140648027606));
#71028=CARTESIAN_POINT('Ctrl Pts',(64.9599339375107,776.754973697645,107.161417845716));
#71029=CARTESIAN_POINT('Ctrl Pts',(65.0790786237519,776.972765128191,107.198024769879));
#71030=CARTESIAN_POINT('Ctrl Pts',(65.157423706574,777.06748124862,107.2137056887));
#71031=CARTESIAN_POINT('Ctrl Pts',(65.327869871706,777.207531871683,107.236126534395));
#71032=CARTESIAN_POINT('Ctrl Pts',(65.4133174380026,777.258017691905,107.243868632409));
#71033=CARTESIAN_POINT('Ctrl Pts',(65.5533429463574,777.313713915724,107.251634886811));
#71034=CARTESIAN_POINT('Ctrl Pts',(65.603046462404,777.328939096693,107.253564571878));
#71035=CARTESIAN_POINT('Ctrl Pts',(65.691202455759,777.34825438477,107.255572420587));
#71036=CARTESIAN_POINT('Ctrl Pts',(65.72910565202,777.354197115841,107.256001147787));
#71037=CARTESIAN_POINT('Ctrl Pts',(65.7851249769906,777.359548919515,107.255999937166));
#71038=CARTESIAN_POINT('Ctrl Pts',(65.8030275050721,777.360750787118,107.255905493694));
#71039=CARTESIAN_POINT('Ctrl Pts',(65.8642141912673,777.363126164254,107.255261695874));
#71040=CARTESIAN_POINT('Ctrl Pts',(65.9075288362554,777.3618553558,107.254258713131));
#71041=CARTESIAN_POINT('Ctrl Pts',(66.0215421744424,777.35069814177,107.25016831844));
#71042=CARTESIAN_POINT('Ctrl Pts',(66.0914119591671,777.335804392169,107.246164876582));
#71043=CARTESIAN_POINT('Ctrl Pts',(66.2777522215371,777.27351803522,107.23131969242));
#71044=CARTESIAN_POINT('Ctrl Pts',(66.3871548106612,777.210683193057,107.217750228743));
#71045=CARTESIAN_POINT('Ctrl Pts',(66.563117924055,777.056502548005,107.186360143025));
#71046=CARTESIAN_POINT('Ctrl Pts',(66.631886345624,776.970816324838,107.169518148369));
#71047=CARTESIAN_POINT('Ctrl Pts',(66.7411990064495,776.771970264116,107.131707116004));
#71048=CARTESIAN_POINT('Ctrl Pts',(66.7779141056529,776.658826566805,107.110842512559));
#71049=CARTESIAN_POINT('Ctrl Pts',(66.8088835662978,776.415907767078,107.067467884149));
#71050=CARTESIAN_POINT('Ctrl Pts',(66.7993393484381,776.287790441984,107.04536396087));
#71051=CARTESIAN_POINT('Ctrl Pts',(66.7311472726406,776.045441540949,107.005063032344));
#71052=CARTESIAN_POINT('Ctrl Pts',(66.6742419243611,775.933055037253,106.987133321718));
#71053=CARTESIAN_POINT('Ctrl Pts',(66.5213324548183,775.737620831312,106.95737404162));
#71054=CARTESIAN_POINT('Ctrl Pts',(66.4273149450998,775.655876932177,106.945712474531));
#71055=CARTESIAN_POINT('Ctrl Pts',(66.264699361539,775.562325212459,106.933579509576));
#71056=CARTESIAN_POINT('Ctrl Pts',(66.206184690539,775.536053303044,106.930454984566));
#71057=CARTESIAN_POINT('Ctrl Pts',(66.1075854805185,775.503247176792,106.927083624026));
#71058=CARTESIAN_POINT('Ctrl Pts',(66.0689740616965,775.493040979168,106.926199650991));
#71059=CARTESIAN_POINT('Ctrl Pts',(66.0125143587785,775.481867036827,106.92552098065));
#71060=CARTESIAN_POINT('Ctrl Pts',(65.9951093061857,775.478923975769,106.925393885891));
#71061=CARTESIAN_POINT('Ctrl Pts',(65.9607551680561,775.474097155938,106.925303286111));
#71062=CARTESIAN_POINT('Ctrl Pts',(65.943817948372,775.472181433331,106.925334324967));
#71063=CARTESIAN_POINT('Ctrl Pts',(65.9020012029613,775.468591689562,106.925596430788));
#71064=CARTESIAN_POINT('Ctrl Pts',(65.8770916458451,775.467441364147,106.925913297626));
#71065=CARTESIAN_POINT('Ctrl Pts',(65.8521676736201,775.46727685438,106.926390289016));
#71066=CARTESIAN_POINT('Ctrl Pts',(65.8523138277848,776.834453268023,108.748340500639));
#71067=CARTESIAN_POINT('Ctrl Pts',(65.9755932814574,776.832970173364,108.75253674477));
#71068=CARTESIAN_POINT('Ctrl Pts',(66.0974845196465,776.807660364505,108.752000220028));
#71069=CARTESIAN_POINT('Ctrl Pts',(66.3271173242504,776.711611238658,108.741919328901));
#71070=CARTESIAN_POINT('Ctrl Pts',(66.4321784934129,776.641010667136,108.732321657587));
#71071=CARTESIAN_POINT('Ctrl Pts',(66.6097011617382,776.463317298711,108.705744912834));
#71072=CARTESIAN_POINT('Ctrl Pts',(66.6801498205331,776.357660928064,108.688975507296));
#71073=CARTESIAN_POINT('Ctrl Pts',(66.7767014433819,776.124260080931,108.650642492643));
#71074=CARTESIAN_POINT('Ctrl Pts',(66.8012676906133,775.998380960927,108.629371044712));
#71075=CARTESIAN_POINT('Ctrl Pts',(66.7994991288181,775.74735913733,108.585763695408));
#71076=CARTESIAN_POINT('Ctrl Pts',(66.7741542057155,775.624422336652,108.56382675012));
#71077=CARTESIAN_POINT('Ctrl Pts',(66.6777954334382,775.397595837452,108.521749780387));
#71078=CARTESIAN_POINT('Ctrl Pts',(66.6084609820003,775.295441337757,108.501951703788));
#71079=CARTESIAN_POINT('Ctrl Pts',(66.4348223023411,775.124712757349,108.466479393225));
#71080=CARTESIAN_POINT('Ctrl Pts',(66.3326881832758,775.057397791066,108.451094710872));
#71081=CARTESIAN_POINT('Ctrl Pts',(66.1073521068603,774.965595399574,108.426235557521));
#71082=CARTESIAN_POINT('Ctrl Pts',(65.986522794371,774.942148754366,108.41703149008));
#71083=CARTESIAN_POINT('Ctrl Pts',(65.8602817427518,774.942450127446,108.411401868727));
#71084=CARTESIAN_POINT('Ctrl Pts',(65.8562970470197,774.942484867569,108.411228246327));
#71085=CARTESIAN_POINT('Ctrl Pts',(65.8523138277871,774.942544771236,108.411058755856));
#71086=CARTESIAN_POINT('Origin',(65.8523138277871,779.672231777069,97.874067134449));
#71087=CARTESIAN_POINT('',(65.8523138277871,778.008815145563,104.080962377937));
#71088=CARTESIAN_POINT('Origin',(65.8523138277871,777.537392914954,103.91434581067));
#71089=CARTESIAN_POINT('',(65.8523138277873,776.389806261283,108.661760026823));
#71090=CARTESIAN_POINT('',(65.8523138277871,780.143654007678,98.0406837017161));
#71091=CARTESIAN_POINT('Ctrl Pts',(65.8523236262048,775.392032337629,108.483943428478));
#71092=CARTESIAN_POINT('Ctrl Pts',(65.7878831210737,775.39295660244,108.481324538884));
#71093=CARTESIAN_POINT('Ctrl Pts',(65.7241978017977,775.406334757023,108.480843373498));
#71094=CARTESIAN_POINT('Ctrl Pts',(65.6030429989561,775.457117722179,108.484315352157));
#71095=CARTESIAN_POINT('Ctrl Pts',(65.547142292733,775.49486490529,108.488399771766));
#71096=CARTESIAN_POINT('Ctrl Pts',(65.4524055773241,775.590135292748,108.500900894481));
#71097=CARTESIAN_POINT('Ctrl Pts',(65.4147750191479,775.64705429602,108.509270128121));
#71098=CARTESIAN_POINT('Ctrl Pts',(65.3642116813439,775.771358807386,108.52915264891));
#71099=CARTESIAN_POINT('Ctrl Pts',(65.3515904232822,775.837563516921,108.540469630755));
#71100=CARTESIAN_POINT('Ctrl Pts',(65.3530953749288,775.97012946301,108.564479362415));
#71101=CARTESIAN_POINT('Ctrl Pts',(65.3670010612835,776.035275973097,108.57694019845));
#71102=CARTESIAN_POINT('Ctrl Pts',(65.4192307002952,776.154810754385,108.601026322507));
#71103=CARTESIAN_POINT('Ctrl Pts',(65.4565005520766,776.208278601099,108.612433029473));
#71104=CARTESIAN_POINT('Ctrl Pts',(65.5495777323318,776.297359004874,108.632697193855));
#71105=CARTESIAN_POINT('Ctrl Pts',(65.6042627705228,776.332258748866,108.641374072043));
#71106=CARTESIAN_POINT('Ctrl Pts',(65.7243323807721,776.379166233064,108.654827946433));
#71107=CARTESIAN_POINT('Ctrl Pts',(65.7884582310674,776.390729781173,108.65947181588));
#71108=CARTESIAN_POINT('Ctrl Pts',(65.9189746729532,776.388843611188,108.664149031545));
#71109=CARTESIAN_POINT('Ctrl Pts',(65.9839985847323,776.374979417501,108.66405355304));
#71110=CARTESIAN_POINT('Ctrl Pts',(66.105940596835,776.322870548642,108.659095610779));
#71111=CARTESIAN_POINT('Ctrl Pts',(66.1614612249993,776.284825042422,108.654220772858));
#71112=CARTESIAN_POINT('Ctrl Pts',(66.2547672156122,776.189536853153,108.640454625418));
#71113=CARTESIAN_POINT('Ctrl Pts',(66.291541390347,776.133108003367,108.631676658887));
#71114=CARTESIAN_POINT('Ctrl Pts',(66.3411916474218,776.00918888395,108.611441701454));
#71115=CARTESIAN_POINT('Ctrl Pts',(66.3534220149565,775.942748845708,108.600150043006));
#71116=CARTESIAN_POINT('Ctrl Pts',(66.351070325944,775.810535114789,108.5768357731));
#71117=CARTESIAN_POINT('Ctrl Pts',(66.3370086347315,775.745929364074,108.565033027938));
#71118=CARTESIAN_POINT('Ctrl Pts',(66.2848546751548,775.626960494077,108.542344463995));
#71119=CARTESIAN_POINT('Ctrl Pts',(66.2476407407646,775.573531554295,108.531650840516));
#71120=CARTESIAN_POINT('Ctrl Pts',(66.1548823701777,775.484555924095,108.512576100187));
#71121=CARTESIAN_POINT('Ctrl Pts',(66.1004778653315,775.44968513785,108.504355193393));
#71122=CARTESIAN_POINT('Ctrl Pts',(65.9808501232473,775.402702517939,108.491280639784));
#71123=CARTESIAN_POINT('Ctrl Pts',(65.9168825237981,775.391106374724,108.486567129591));
#71124=CARTESIAN_POINT('Ctrl Pts',(65.8523236262048,775.392032337629,108.483943428478));
#71125=CARTESIAN_POINT('Origin',(44.8921369270856,786.628267531093,100.332565533275));
#71126=CARTESIAN_POINT('',(44.8921369270856,784.225718511386,110.909518141625));
#71127=CARTESIAN_POINT('Origin',(44.8921369270856,783.038336934424,110.489857316266));
#71128=CARTESIAN_POINT('',(44.892136974638,784.857852423734,109.120968636072));
#71129=CARTESIAN_POINT('',(44.8921369270856,787.815649108055,100.752226358633));
#71130=CARTESIAN_POINT('Ctrl Pts',(44.8923073484297,782.422749479518,108.45237145031));
#71131=CARTESIAN_POINT('Ctrl Pts',(44.8162819691552,782.42299144979,108.451655950142));
#71132=CARTESIAN_POINT('Ctrl Pts',(44.7404232666641,782.429931891369,108.452646681253));
#71133=CARTESIAN_POINT('Ctrl Pts',(44.5603464969493,782.462552645622,108.459142731722));
#71134=CARTESIAN_POINT('Ctrl Pts',(44.4579575372025,782.494594811484,108.46629916939));
#71135=CARTESIAN_POINT('Ctrl Pts',(44.208852900756,782.608056538512,108.493019022734));
#71136=CARTESIAN_POINT('Ctrl Pts',(44.0725044195926,782.706041579602,108.517055867388));
#71137=CARTESIAN_POINT('Ctrl Pts',(43.85889975643,782.934951031857,108.575212430792));
#71138=CARTESIAN_POINT('Ctrl Pts',(43.7786615350378,783.059590779428,108.607576757387));
#71139=CARTESIAN_POINT('Ctrl Pts',(43.6637106530933,783.338132164978,108.681584485548));
#71140=CARTESIAN_POINT('Ctrl Pts',(43.6331172062892,783.49090718019,108.723031679013));
#71141=CARTESIAN_POINT('Ctrl Pts',(43.6324246149148,783.805991553284,108.810250709823));
#71142=CARTESIAN_POINT('Ctrl Pts',(43.6651931363107,783.965339218652,108.855280334504));
#71143=CARTESIAN_POINT('Ctrl Pts',(43.7923201765428,784.259766106586,108.939900381986));
#71144=CARTESIAN_POINT('Ctrl Pts',(43.8844794342416,784.392357994548,108.978738096277));
#71145=CARTESIAN_POINT('Ctrl Pts',(44.1057679513745,784.605258926542,109.041971711113));
#71146=CARTESIAN_POINT('Ctrl Pts',(44.2288314515859,784.687626790762,109.066871395095));
#71147=CARTESIAN_POINT('Ctrl Pts',(44.446078059077,784.783614759782,109.096393723432));
#71148=CARTESIAN_POINT('Ctrl Pts',(44.531919601865,784.811252398521,109.105054853075));
#71149=CARTESIAN_POINT('Ctrl Pts',(44.6575272967582,784.837700513626,109.113607669532));
#71150=CARTESIAN_POINT('Ctrl Pts',(44.6952917615232,784.843932240686,109.115672881431));
#71151=CARTESIAN_POINT('Ctrl Pts',(44.7676643818972,784.852630748071,109.118674765112));
#71152=CARTESIAN_POINT('Ctrl Pts',(44.8021976191136,784.855397046532,109.119699250864));
#71153=CARTESIAN_POINT('Ctrl Pts',(44.9118036736405,784.859814273518,109.121665797058));
#71154=CARTESIAN_POINT('Ctrl Pts',(44.9869414563982,784.856388765398,109.121112186209));
#71155=CARTESIAN_POINT('Ctrl Pts',(45.1659145638157,784.832726237737,109.115249535883));
#71156=CARTESIAN_POINT('Ctrl Pts',(45.2682965869261,784.806321184381,109.108122784627));
#71157=CARTESIAN_POINT('Ctrl Pts',(45.5212130708983,784.707055967686,109.080701233473));
#71158=CARTESIAN_POINT('Ctrl Pts',(45.6621889493315,784.617025423278,109.05540971265));
#71159=CARTESIAN_POINT('Ctrl Pts',(45.8868787027634,784.401100004618,108.994901346306));
#71160=CARTESIAN_POINT('Ctrl Pts',(45.973250561103,784.281702220923,108.961503594805));
#71161=CARTESIAN_POINT('Ctrl Pts',(46.1021019238818,784.011660239623,108.886550026756));
#71162=CARTESIAN_POINT('Ctrl Pts',(46.1406334213441,783.862007390482,108.845309057943));
#71163=CARTESIAN_POINT('Ctrl Pts',(46.1589399696531,783.547147245785,108.759302434206));
#71164=CARTESIAN_POINT('Ctrl Pts',(46.134740405625,783.384648516219,108.715324803664));
#71165=CARTESIAN_POINT('Ctrl Pts',(46.0227701768699,783.080537851574,108.633482615148));
#71166=CARTESIAN_POINT('Ctrl Pts',(45.9370116997564,782.941548162612,108.596303039931));
#71167=CARTESIAN_POINT('Ctrl Pts',(45.7159078965255,782.704871855997,108.532769262459));
#71168=CARTESIAN_POINT('Ctrl Pts',(45.5831741223873,782.609040411889,108.506898925147));
#71169=CARTESIAN_POINT('Ctrl Pts',(45.3471502485886,782.500099987671,108.476693369378));
#71170=CARTESIAN_POINT('Ctrl Pts',(45.2546051644565,782.469577723498,108.46798515072));
#71171=CARTESIAN_POINT('Ctrl Pts',(45.1243436765839,782.442489798182,108.459764223446));
#71172=CARTESIAN_POINT('Ctrl Pts',(45.0890639855754,782.436672235543,108.457924227011));
#71173=CARTESIAN_POINT('Ctrl Pts',(45.0270251652088,782.429074442781,108.455357726509));
#71174=CARTESIAN_POINT('Ctrl Pts',(45.0003760569042,782.426648194516,108.454468151232));
#71175=CARTESIAN_POINT('Ctrl Pts',(44.9465807318617,782.423430431719,108.453099584936));
#71176=CARTESIAN_POINT('Ctrl Pts',(44.9194473842637,782.422663099392,108.452626874227));
#71177=CARTESIAN_POINT('Ctrl Pts',(44.8923073484297,782.422749479518,108.45237145031));
#71178=CARTESIAN_POINT('Origin',(44.8921369270856,786.628267531093,100.332565533275));
#71179=CARTESIAN_POINT('',(44.8921369270856,784.964850899586,106.539460776763));
#71180=CARTESIAN_POINT('Origin',(44.8921369270856,784.493428668978,106.372844209496));
#71181=CARTESIAN_POINT('',(44.8921369270856,783.509759165033,110.656473883533));
#71182=CARTESIAN_POINT('',(44.8921369270856,787.099689761701,100.499182100542));
#71183=CARTESIAN_POINT('Origin',(44.8921369270856,783.038336934424,110.489857316266));
#71184=CARTESIAN_POINT('Origin',(49.0936533033807,782.22871327632,98.7776141969985));
#71185=CARTESIAN_POINT('',(49.0936533033807,777.622727263691,108.744570586988));
#71186=CARTESIAN_POINT('',(49.0936533033809,779.593263946518,109.299458278251));
#71187=CARTESIAN_POINT('Ctrl Pts',(49.0936533033807,777.622727263691,108.744570586988));
#71188=CARTESIAN_POINT('Ctrl Pts',(48.9632002870732,777.622428485583,108.745415944952));
#71189=CARTESIAN_POINT('Ctrl Pts',(48.833946065599,777.646453119096,108.752434741664));
#71190=CARTESIAN_POINT('Ctrl Pts',(48.5883527706715,777.741862477848,108.778574089776));
#71191=CARTESIAN_POINT('Ctrl Pts',(48.4749703105534,777.813617826965,108.79777836983));
#71192=CARTESIAN_POINT('Ctrl Pts',(48.2830436461297,777.995647923637,108.846516004725));
#71193=CARTESIAN_POINT('Ctrl Pts',(48.2064874701559,778.104274454239,108.875624111595));
#71194=CARTESIAN_POINT('Ctrl Pts',(48.1012232380387,778.343602206046,108.940563764105));
#71195=CARTESIAN_POINT('Ctrl Pts',(48.0735033741326,778.472013653152,108.97578880451));
#71196=CARTESIAN_POINT('Ctrl Pts',(48.0710564047158,778.732958464172,109.048553371529));
#71197=CARTESIAN_POINT('Ctrl Pts',(48.0969653472274,778.862958451878,109.08540613932));
#71198=CARTESIAN_POINT('Ctrl Pts',(48.1995298154465,779.103846631018,109.154765673716));
#71199=CARTESIAN_POINT('Ctrl Pts',(48.2745791925128,779.212586684015,109.186630601971));
#71200=CARTESIAN_POINT('Ctrl Pts',(48.4641597582515,779.395616161713,109.240795518626));
#71201=CARTESIAN_POINT('Ctrl Pts',(48.5767645661844,779.468158125872,109.262557898456));
#71202=CARTESIAN_POINT('Ctrl Pts',(48.8252757551249,779.5674830409,109.292254814351));
#71203=CARTESIAN_POINT('Ctrl Pts',(48.9587983910953,779.593131925164,109.299831817343));
#71204=CARTESIAN_POINT('Ctrl Pts',(49.0936533033811,779.593263946518,109.299458278251));
#71205=CARTESIAN_POINT('',(49.0936533269279,780.072861410571,107.94249294157));
#71206=CARTESIAN_POINT('',(49.0936533033807,783.191742416563,99.1179812800658));
#71207=CARTESIAN_POINT('Ctrl Pts',(49.0937056776217,778.048104433328,107.541015281665));
#71208=CARTESIAN_POINT('Ctrl Pts',(49.0271547441502,778.048321177872,107.540391787571));
#71209=CARTESIAN_POINT('Ctrl Pts',(48.9607903865118,778.055022080643,107.540940204712));
#71210=CARTESIAN_POINT('Ctrl Pts',(48.8117888491069,778.084877021327,107.544868878333));
#71211=CARTESIAN_POINT('Ctrl Pts',(48.7305237807704,778.112035075303,107.548991866279));
#71212=CARTESIAN_POINT('Ctrl Pts',(48.5304377372779,778.207843672871,107.564542383633));
#71213=CARTESIAN_POINT('Ctrl Pts',(48.4205566551283,778.290624354942,107.57871212594));
#71214=CARTESIAN_POINT('Ctrl Pts',(48.248797333885,778.483372358419,107.613207792825));
#71215=CARTESIAN_POINT('Ctrl Pts',(48.1846162168159,778.588357303446,107.63252937346));
#71216=CARTESIAN_POINT('Ctrl Pts',(48.0939316473472,778.822159595282,107.676842225506));
#71217=CARTESIAN_POINT('Ctrl Pts',(48.0707481447969,778.950081617404,107.701742704981));
#71218=CARTESIAN_POINT('Ctrl Pts',(48.073967176409,779.213418464044,107.754361930166));
#71219=CARTESIAN_POINT('Ctrl Pts',(48.1027752555812,779.346440990759,107.781666810885));
#71220=CARTESIAN_POINT('Ctrl Pts',(48.2106876020914,779.590992471309,107.833037117464));
#71221=CARTESIAN_POINT('Ctrl Pts',(48.2877948789974,779.700566598424,107.856657992685));
#71222=CARTESIAN_POINT('Ctrl Pts',(48.4740930495997,779.877463759995,107.895605643368));
#71223=CARTESIAN_POINT('Ctrl Pts',(48.5789813814141,779.945728191473,107.911061578461));
#71224=CARTESIAN_POINT('Ctrl Pts',(48.7673092303796,780.024177526603,107.92940720315));
#71225=CARTESIAN_POINT('Ctrl Pts',(48.8440766979462,780.046159153914,107.934755182649));
#71226=CARTESIAN_POINT('Ctrl Pts',(48.9564409588534,780.064664640844,107.939636414258));
#71227=CARTESIAN_POINT('Ctrl Pts',(48.9904403298714,780.068545523425,107.94074320737));
#71228=CARTESIAN_POINT('Ctrl Pts',(49.0557675827937,780.072739097664,107.942165936498));
#71229=CARTESIAN_POINT('Ctrl Pts',(49.0870359458949,780.073328819959,107.942541166276));
#71230=CARTESIAN_POINT('Ctrl Pts',(49.186430777403,780.070706768523,107.942764797524));
#71231=CARTESIAN_POINT('Ctrl Pts',(49.2542214653515,780.062191609398,107.941466692095));
#71232=CARTESIAN_POINT('Ctrl Pts',(49.4129475467574,780.026113842808,107.934975581307));
#71233=CARTESIAN_POINT('Ctrl Pts',(49.5017986747611,779.99260694913,107.928494380102));
#71234=CARTESIAN_POINT('Ctrl Pts',(49.7038721599177,779.882801061356,107.906730217753));
#71235=CARTESIAN_POINT('Ctrl Pts',(49.8086123473817,779.795323691912,107.889064186069));
#71236=CARTESIAN_POINT('Ctrl Pts',(49.9699044951568,779.594614101948,107.848576378668));
#71237=CARTESIAN_POINT('Ctrl Pts',(50.0285430722642,779.485966583569,107.826683787102));
#71238=CARTESIAN_POINT('Ctrl Pts',(50.1061786557834,779.246339681443,107.778767657688));
#71239=CARTESIAN_POINT('Ctrl Pts',(50.1218291289306,779.116500703771,107.752999600788));
#71240=CARTESIAN_POINT('Ctrl Pts',(50.1025559176442,778.852484042031,107.701053957671));
#71241=CARTESIAN_POINT('Ctrl Pts',(50.0656026602404,778.720801185339,107.675385835317));
#71242=CARTESIAN_POINT('Ctrl Pts',(49.9428080377817,778.48180386328,107.628961357646));
#71243=CARTESIAN_POINT('Ctrl Pts',(49.8590764708186,778.376243292557,107.608531686978));
#71244=CARTESIAN_POINT('Ctrl Pts',(49.6683817970023,778.214707142724,107.576927859538));
#71245=CARTESIAN_POINT('Ctrl Pts',(49.5674138549477,778.155205162263,107.56511209074));
#71246=CARTESIAN_POINT('Ctrl Pts',(49.385058364516,778.086339371718,107.550818021285));
#71247=CARTESIAN_POINT('Ctrl Pts',(49.3088046063118,778.067170383379,107.546599133708));
#71248=CARTESIAN_POINT('Ctrl Pts',(49.2085259745404,778.053932036756,107.543210601871));
#71249=CARTESIAN_POINT('Ctrl Pts',(49.1859256021635,778.051710488846,107.542584550007));
#71250=CARTESIAN_POINT('Ctrl Pts',(49.1401126226283,778.048741795942,107.54159245028));
#71251=CARTESIAN_POINT('Ctrl Pts',(49.1169122878013,778.04802885353,107.541232696863));
#71252=CARTESIAN_POINT('Ctrl Pts',(49.0937056776217,778.048104433328,107.541015281665));
#71253=CARTESIAN_POINT('Ctrl Pts',(49.093653303381,779.593263946518,109.299458278251));
#71254=CARTESIAN_POINT('Ctrl Pts',(49.0938253602664,779.593264114959,109.299457801665));
#71255=CARTESIAN_POINT('Ctrl Pts',(49.0939974193205,779.593264241851,109.299457312176));
#71256=CARTESIAN_POINT('Ctrl Pts',(49.0941694805274,779.59326432719,109.299456809783));
#71257=CARTESIAN_POINT('Ctrl Pts',(49.2265276323488,779.593329974147,109.299070344109));
#71258=CARTESIAN_POINT('Ctrl Pts',(49.3576186666871,779.568813570152,109.291030003779));
#71259=CARTESIAN_POINT('Ctrl Pts',(49.6047420471024,779.472477681339,109.260464064252));
#71260=CARTESIAN_POINT('Ctrl Pts',(49.7180437433462,779.400798422938,109.238004235613));
#71261=CARTESIAN_POINT('Ctrl Pts',(49.9087951730618,779.219487758016,109.182331489965));
#71262=CARTESIAN_POINT('Ctrl Pts',(49.9844406122878,779.111714188496,109.149707751261));
#71263=CARTESIAN_POINT('Ctrl Pts',(50.0882999563377,778.872938961531,109.079036770978));
#71264=CARTESIAN_POINT('Ctrl Pts',(50.1150962223982,778.744134562306,109.041666387846));
#71265=CARTESIAN_POINT('Ctrl Pts',(50.115027228245,778.484815561264,108.968211725716));
#71266=CARTESIAN_POINT('Ctrl Pts',(50.0887005288884,778.356819261407,108.932822778779));
#71267=CARTESIAN_POINT('Ctrl Pts',(49.9866264473733,778.117713653121,108.868221322591));
#71268=CARTESIAN_POINT('Ctrl Pts',(49.911937647475,778.008822967132,108.839593293666));
#71269=CARTESIAN_POINT('Ctrl Pts',(49.7239293003419,777.825088963006,108.792347678592));
#71270=CARTESIAN_POINT('Ctrl Pts',(49.6125313280592,777.751850570673,108.77412198634));
#71271=CARTESIAN_POINT('Ctrl Pts',(49.3672158233277,777.650964133216,108.749820142085));
#71272=CARTESIAN_POINT('Ctrl Pts',(49.2357088177524,777.624230107928,108.743950384203));
#71273=CARTESIAN_POINT('Ctrl Pts',(49.0996434064598,777.622753796935,108.744535038214));
#71274=CARTESIAN_POINT('Ctrl Pts',(49.0966480390014,777.62273412257,108.744551180586));
#71275=CARTESIAN_POINT('Ctrl Pts',(49.0936533033807,777.622727263691,108.744570586988));
#71276=CARTESIAN_POINT('Origin',(49.0936533033807,782.22871327632,98.7776141969985));
#71277=CARTESIAN_POINT('',(49.0936533033807,780.565296644814,104.984509440487));
#71278=CARTESIAN_POINT('Origin',(49.0936533033807,780.093874414205,104.81789287322));
#71279=CARTESIAN_POINT('',(49.0936533033808,779.093842445626,109.147818241034));
#71280=CARTESIAN_POINT('',(49.0936533033807,782.700135506929,98.9442307642656));
#71281=CARTESIAN_POINT('Ctrl Pts',(49.0936529529939,778.129187731554,108.876294684482));
#71282=CARTESIAN_POINT('Ctrl Pts',(49.0339299911541,778.129069875144,108.876628271105));
#71283=CARTESIAN_POINT('Ctrl Pts',(48.9746952099443,778.139320411379,108.879735639841));
#71284=CARTESIAN_POINT('Ctrl Pts',(48.8573329198357,778.18153746217,108.891789301062));
#71285=CARTESIAN_POINT('Ctrl Pts',(48.8010442575993,778.215116638054,108.901159973048));
#71286=CARTESIAN_POINT('Ctrl Pts',(48.7049742964704,778.301444764448,108.925117630472));
#71287=CARTESIAN_POINT('Ctrl Pts',(48.6661795247187,778.353406890188,108.939489958875));
#71288=CARTESIAN_POINT('Ctrl Pts',(48.6112999432858,778.469396243527,108.971680317644));
#71289=CARTESIAN_POINT('Ctrl Pts',(48.5960093741457,778.532414270852,108.989223232261));
#71290=CARTESIAN_POINT('Ctrl Pts',(48.5917898937807,778.66076063377,109.025170440976));
#71291=CARTESIAN_POINT('Ctrl Pts',(48.6030318506563,778.724832348016,109.04322517028));
#71292=CARTESIAN_POINT('Ctrl Pts',(48.6507951793941,778.844547241534,109.077148151531));
#71293=CARTESIAN_POINT('Ctrl Pts',(48.6866959785454,778.899058201511,109.09269200419));
#71294=CARTESIAN_POINT('Ctrl Pts',(48.778497345828,778.991364058649,109.119061017436));
#71295=CARTESIAN_POINT('Ctrl Pts',(48.8334672140009,779.028253422815,109.12962279123));
#71296=CARTESIAN_POINT('Ctrl Pts',(48.9553347524394,779.079321089152,109.144100974579));
#71297=CARTESIAN_POINT('Ctrl Pts',(49.0210330503128,779.0929322282,109.147851902656));
#71298=CARTESIAN_POINT('Ctrl Pts',(49.1541503834313,779.09466592974,109.147809453492));
#71299=CARTESIAN_POINT('Ctrl Pts',(49.2202266744672,779.082752256428,109.144010035709));
#71300=CARTESIAN_POINT('Ctrl Pts',(49.3434565507019,779.034810560724,109.129362668073));
#71301=CARTESIAN_POINT('Ctrl Pts',(49.3993906882173,778.999315633519,109.118679925339));
#71302=CARTESIAN_POINT('Ctrl Pts',(49.4934489760915,778.909406933719,109.092016312694));
#71303=CARTESIAN_POINT('Ctrl Pts',(49.530653525023,778.855912476024,109.076312562696));
#71304=CARTESIAN_POINT('Ctrl Pts',(49.5812722610349,778.737772260162,109.042098756154));
#71305=CARTESIAN_POINT('Ctrl Pts',(49.5940906052375,778.674262434235,109.023922964426));
#71306=CARTESIAN_POINT('Ctrl Pts',(49.5931995727275,778.546923013897,108.98797833082));
#71307=CARTESIAN_POINT('Ctrl Pts',(49.57987089725,778.484328380295,108.970551259103));
#71308=CARTESIAN_POINT('Ctrl Pts',(49.5290189689823,778.367655334965,108.938502065176));
#71309=CARTESIAN_POINT('Ctrl Pts',(49.492025321095,778.314666705199,108.924175652239));
#71310=CARTESIAN_POINT('Ctrl Pts',(49.3991635310428,778.225507085843,108.900409256669));
#71311=CARTESIAN_POINT('Ctrl Pts',(49.3442389574218,778.190136099238,108.891177247252));
#71312=CARTESIAN_POINT('Ctrl Pts',(49.2235176617433,778.141821358915,108.878883772904));
#71313=CARTESIAN_POINT('Ctrl Pts',(49.1589091968619,778.129316507261,108.87593019134));
#71314=CARTESIAN_POINT('Ctrl Pts',(49.0936529529939,778.129187731554,108.876294684482));
#71315=CARTESIAN_POINT('Origin',(54.622724097431,778.213544437116,97.3585176725896));
#71316=CARTESIAN_POINT('',(54.622724097431,773.482462218109,107.899456887669));
#71317=CARTESIAN_POINT('',(54.622724097431,775.377367353003,108.228259992878));
#71318=CARTESIAN_POINT('Ctrl Pts',(54.6227240974307,773.482462218109,107.899456887669));
#71319=CARTESIAN_POINT('Ctrl Pts',(54.5071908003515,773.482696433452,107.898794202553));
#71320=CARTESIAN_POINT('Ctrl Pts',(54.3927095887361,773.504165869956,107.90141402035));
#71321=CARTESIAN_POINT('Ctrl Pts',(54.1679886550712,773.590758299484,107.913586074231));
#71322=CARTESIAN_POINT('Ctrl Pts',(54.0614064897469,773.658443861292,107.923574140098));
#71323=CARTESIAN_POINT('Ctrl Pts',(53.8792311617861,773.831873819902,107.950262927227));
#71324=CARTESIAN_POINT('Ctrl Pts',(53.8059507901509,773.936483652477,107.966814225441));
#71325=CARTESIAN_POINT('Ctrl Pts',(53.7035028551231,774.16948192188,108.004940395586));
#71326=CARTESIAN_POINT('Ctrl Pts',(53.6761364981783,774.296106177837,108.026257726283));
#71327=CARTESIAN_POINT('Ctrl Pts',(53.6732822144116,774.550249009593,108.070375030963));
#71328=CARTESIAN_POINT('Ctrl Pts',(53.6971030856602,774.675439235575,108.092753169681));
#71329=CARTESIAN_POINT('Ctrl Pts',(53.7922038053258,774.907418348338,108.135309699879));
#71330=CARTESIAN_POINT('Ctrl Pts',(53.8619123252693,775.012258230956,108.155105398148));
#71331=CARTESIAN_POINT('Ctrl Pts',(54.0382646177959,775.188373499272,108.189078330288));
#71332=CARTESIAN_POINT('Ctrl Pts',(54.142876742799,775.25810793812,108.202938788058));
#71333=CARTESIAN_POINT('Ctrl Pts',(54.3737564245772,775.353177412434,108.222346328971));
#71334=CARTESIAN_POINT('Ctrl Pts',(54.4975757462634,775.377566653681,108.227689314813));
#71335=CARTESIAN_POINT('Ctrl Pts',(54.6227069807416,775.377367380385,108.228259914849));
#71336=CARTESIAN_POINT('Ctrl Pts',(54.6227126863074,775.377367371299,108.228259940867));
#71337=CARTESIAN_POINT('Ctrl Pts',(54.6227183918705,775.377367362191,108.22825996688));
#71338=CARTESIAN_POINT('Ctrl Pts',(54.622724097431,775.377367353003,108.228259992878));
#71339=CARTESIAN_POINT('',(54.6227240859897,775.748529403717,107.178100067398));
#71340=CARTESIAN_POINT('',(54.622724097431,779.107440609735,97.6744508257262));
#71341=CARTESIAN_POINT('Ctrl Pts',(54.622716580523,773.827866246708,106.922176294992));
#71342=CARTESIAN_POINT('Ctrl Pts',(54.5547214479639,773.827706518738,106.922629844528));
#71343=CARTESIAN_POINT('Ctrl Pts',(54.48695467043,773.835001109058,106.923941811772));
#71344=CARTESIAN_POINT('Ctrl Pts',(54.3341976754647,773.868608227771,106.92889428809));
#71345=CARTESIAN_POINT('Ctrl Pts',(54.2510658090552,773.899791884602,106.933087388114));
#71346=CARTESIAN_POINT('Ctrl Pts',(54.0627462365035,774.002529467038,106.946450719118));
#71347=CARTESIAN_POINT('Ctrl Pts',(53.965430143705,774.084527837828,106.956839943242));
#71348=CARTESIAN_POINT('Ctrl Pts',(53.813741224562,774.27409207907,106.980954385284));
#71349=CARTESIAN_POINT('Ctrl Pts',(53.758027625191,774.377889685351,106.994202828633));
#71350=CARTESIAN_POINT('Ctrl Pts',(53.6836643689704,774.607301028281,107.023918515021));
#71351=CARTESIAN_POINT('Ctrl Pts',(53.66837221503,774.732056379351,107.040308491224));
#71352=CARTESIAN_POINT('Ctrl Pts',(53.6858630334801,774.984738439568,107.074080228882));
#71353=CARTESIAN_POINT('Ctrl Pts',(53.7202694225296,775.110424799374,107.09118321926));
#71354=CARTESIAN_POINT('Ctrl Pts',(53.8349920837059,775.337509559787,107.122448519933));
#71355=CARTESIAN_POINT('Ctrl Pts',(53.912929941399,775.437441484146,107.136388643344));
#71356=CARTESIAN_POINT('Ctrl Pts',(54.0900558647598,775.58983252655,107.157590658501));
#71357=CARTESIAN_POINT('Ctrl Pts',(54.1833384098643,775.645864259133,107.165352934401));
#71358=CARTESIAN_POINT('Ctrl Pts',(54.3536483355174,775.711783249342,107.174173684347));
#71359=CARTESIAN_POINT('Ctrl Pts',(54.4260017437422,775.730362875771,107.176534938924));
#71360=CARTESIAN_POINT('Ctrl Pts',(54.532241205095,775.744561140108,107.178038880669));
#71361=CARTESIAN_POINT('Ctrl Pts',(54.5648533558934,775.747202740603,107.178243185922));
#71362=CARTESIAN_POINT('Ctrl Pts',(54.628232021751,775.749024807328,107.178141976805));
#71363=CARTESIAN_POINT('Ctrl Pts',(54.6589472785579,775.74840522504,107.177866856488));
#71364=CARTESIAN_POINT('Ctrl Pts',(54.7593635711179,775.741456415546,107.176226523946));
#71365=CARTESIAN_POINT('Ctrl Pts',(54.8283504852572,775.728864667926,107.17392188599));
#71366=CARTESIAN_POINT('Ctrl Pts',(54.9911292612032,775.679976819372,107.16562604374));
#71367=CARTESIAN_POINT('Ctrl Pts',(55.0816102887839,775.636136579799,107.158529661192));
#71368=CARTESIAN_POINT('Ctrl Pts',(55.2539895568943,775.515836505949,107.139718538326));
#71369=CARTESIAN_POINT('Ctrl Pts',(55.3325516100012,775.437401730338,107.127752856353));
#71370=CARTESIAN_POINT('Ctrl Pts',(55.4632320033908,775.251799922037,107.100265283793));
#71371=CARTESIAN_POINT('Ctrl Pts',(55.5122974996599,775.144706590069,107.084806196904));
#71372=CARTESIAN_POINT('Ctrl Pts',(55.5718394124838,774.910271451148,107.052025829815));
#71373=CARTESIAN_POINT('Ctrl Pts',(55.5787844982082,774.784042196732,107.034938701645));
#71374=CARTESIAN_POINT('Ctrl Pts',(55.5440059142545,774.532007887812,107.002014366974));
#71375=CARTESIAN_POINT('Ctrl Pts',(55.5010399322351,774.408502445413,106.986515261922));
#71376=CARTESIAN_POINT('Ctrl Pts',(55.3711866059429,774.188986879033,106.959985826081));
#71377=CARTESIAN_POINT('Ctrl Pts',(55.2868141078448,774.094130136453,106.949050756357));
#71378=CARTESIAN_POINT('Ctrl Pts',(55.10685794516,773.958321213211,106.934053534688));
#71379=CARTESIAN_POINT('Ctrl Pts',(55.0184126392753,773.911103993303,106.929122534429));
#71380=CARTESIAN_POINT('Ctrl Pts',(54.8565851010744,773.855460892064,106.923747053613));
#71381=CARTESIAN_POINT('Ctrl Pts',(54.7866558209677,773.840026945331,106.922445492453));
#71382=CARTESIAN_POINT('Ctrl Pts',(54.6847458860643,773.829564008447,106.921941855052));
#71383=CARTESIAN_POINT('Ctrl Pts',(54.6537438552632,773.827939133155,106.921969333031));
#71384=CARTESIAN_POINT('Ctrl Pts',(54.622716580523,773.827866246708,106.922176294992));
#71385=CARTESIAN_POINT('Ctrl Pts',(54.622724097431,775.377367353003,108.228259992878));
#71386=CARTESIAN_POINT('Ctrl Pts',(54.7413994181553,775.377176233909,108.228800742162));
#71387=CARTESIAN_POINT('Ctrl Pts',(54.8589252993588,775.354871874229,108.225040606538));
#71388=CARTESIAN_POINT('Ctrl Pts',(55.0856783861241,775.26607659639,108.209119800715));
#71389=CARTESIAN_POINT('Ctrl Pts',(55.1916913443785,775.198109872329,108.196676095123));
#71390=CARTESIAN_POINT('Ctrl Pts',(55.3716683219127,775.02490891286,108.165162909421));
#71391=CARTESIAN_POINT('Ctrl Pts',(55.4435478901821,774.921140142487,108.146374901502));
#71392=CARTESIAN_POINT('Ctrl Pts',(55.5433977550748,774.69045841209,108.105268754576));
#71393=CARTESIAN_POINT('Ctrl Pts',(55.5697381870677,774.565445575138,108.083306050231));
#71394=CARTESIAN_POINT('Ctrl Pts',(55.5718043512056,774.313882365095,108.039852320873));
#71395=CARTESIAN_POINT('Ctrl Pts',(55.5480284369105,774.189581291565,108.018739817575));
#71396=CARTESIAN_POINT('Ctrl Pts',(55.4541571370007,773.958887117895,107.980018294411));
#71397=CARTESIAN_POINT('Ctrl Pts',(55.3855739147925,773.854258479443,107.962689098121));
#71398=CARTESIAN_POINT('Ctrl Pts',(55.2130607587389,773.678553474488,107.933609686352));
#71399=CARTESIAN_POINT('Ctrl Pts',(55.1113512440305,773.608566369919,107.922029109468));
#71400=CARTESIAN_POINT('Ctrl Pts',(54.8870777334388,773.511594919478,107.905551238059));
#71401=CARTESIAN_POINT('Ctrl Pts',(54.7669522819423,773.48531221698,107.900770610043));
#71402=CARTESIAN_POINT('Ctrl Pts',(54.6375558568623,773.482519595948,107.899555498672));
#71403=CARTESIAN_POINT('Ctrl Pts',(54.6301378111837,773.482447188628,107.899499411841));
#71404=CARTESIAN_POINT('Ctrl Pts',(54.6227240974307,773.482462218109,107.899456887669));
#71405=CARTESIAN_POINT('Origin',(54.622724097431,778.213544437116,97.3585176725896));
#71406=CARTESIAN_POINT('',(54.622724097431,776.55012780561,103.565412916078));
#71407=CARTESIAN_POINT('Origin',(54.622724097431,776.078705575001,103.398796348811));
#71408=CARTESIAN_POINT('',(54.6227240974311,774.932139756061,108.143322231624));
#71409=CARTESIAN_POINT('',(54.622724097431,778.684966667725,97.5251342398567));
#71410=CARTESIAN_POINT('Ctrl Pts',(54.6227191556436,773.932781274095,107.969988956817));
#71411=CARTESIAN_POINT('Ctrl Pts',(54.561687772208,773.932899898407,107.969655133269));
#71412=CARTESIAN_POINT('Ctrl Pts',(54.50124623174,773.944221424331,107.97115222592));
#71413=CARTESIAN_POINT('Ctrl Pts',(54.3828385167216,773.989774403011,107.977947863272));
#71414=CARTESIAN_POINT('Ctrl Pts',(54.3267325112097,774.025310100391,107.98347519596));
#71415=CARTESIAN_POINT('Ctrl Pts',(54.2305902711695,774.11658962763,107.998107413849));
#71416=CARTESIAN_POINT('Ctrl Pts',(54.1918597388119,774.171805615782,108.007137886609));
#71417=CARTESIAN_POINT('Ctrl Pts',(54.1379246848474,774.294554828104,108.027653350482));
#71418=CARTESIAN_POINT('Ctrl Pts',(54.1235485762318,774.361091335508,108.038979723125));
#71419=CARTESIAN_POINT('Ctrl Pts',(54.1219744257417,774.495120721451,108.062235715201));
#71420=CARTESIAN_POINT('Ctrl Pts',(54.134587267002,774.561388536653,108.073949533389));
#71421=CARTESIAN_POINT('Ctrl Pts',(54.1850639422275,774.684427445897,108.096069747683));
#71422=CARTESIAN_POINT('Ctrl Pts',(54.2221935785743,774.740129991465,108.106277457678));
#71423=CARTESIAN_POINT('Ctrl Pts',(54.3151486312484,774.832544682185,108.123489914695));
#71424=CARTESIAN_POINT('Ctrl Pts',(54.3695203856928,774.86885143445,108.130406436861));
#71425=CARTESIAN_POINT('Ctrl Pts',(54.4891072638071,774.918557228744,108.140130263793));
#71426=CARTESIAN_POINT('Ctrl Pts',(54.5530376305238,774.931594169828,108.14286200799));
#71427=CARTESIAN_POINT('Ctrl Pts',(54.683310748962,774.932660053448,108.143730806839));
#71428=CARTESIAN_POINT('Ctrl Pts',(54.7482901945077,774.920352680989,108.141798928));
#71429=CARTESIAN_POINT('Ctrl Pts',(54.8706748106997,774.871194126728,108.133440911594));
#71430=CARTESIAN_POINT('Ctrl Pts',(54.9266391554852,774.834490789525,108.127037758269));
#71431=CARTESIAN_POINT('Ctrl Pts',(55.0212308234026,774.741354475557,108.110721338592));
#71432=CARTESIAN_POINT('Ctrl Pts',(55.0587548320678,774.685712231709,108.100949918147));
#71433=CARTESIAN_POINT('Ctrl Pts',(55.1100602100006,774.562690923574,108.079447781784));
#71434=CARTESIAN_POINT('Ctrl Pts',(55.1231033222687,774.49636817689,108.067904897197));
#71435=CARTESIAN_POINT('Ctrl Pts',(55.1223255313603,774.36219256659,108.044690970332));
#71436=CARTESIAN_POINT('Ctrl Pts',(55.1083339956401,774.295564275139,108.033232246365));
#71437=CARTESIAN_POINT('Ctrl Pts',(55.0556195402748,774.173902001322,108.012368859315));
#71438=CARTESIAN_POINT('Ctrl Pts',(55.0182397743535,774.119620555165,108.003088267979));
#71439=CARTESIAN_POINT('Ctrl Pts',(54.9251461528609,774.029090451328,107.987532467646));
#71440=CARTESIAN_POINT('Ctrl Pts',(54.8706037585573,773.993430164989,107.981356802045));
#71441=CARTESIAN_POINT('Ctrl Pts',(54.7509780106576,773.945032249884,107.972729045437));
#71442=CARTESIAN_POINT('Ctrl Pts',(54.6871837286973,773.932655976827,107.970341558893));
#71443=CARTESIAN_POINT('Ctrl Pts',(54.6227191556436,773.932781274095,107.969988956817));
#71444=CARTESIAN_POINT('Origin',(35.6544901166228,789.126363770955,101.215477269642));
#71445=CARTESIAN_POINT('',(35.6544901166228,786.723814751248,111.792429877991));
#71446=CARTESIAN_POINT('Origin',(35.6544901166228,785.536433174286,111.372769052633));
#71447=CARTESIAN_POINT('',(35.6544901166059,787.390150915315,109.907109072553));
#71448=CARTESIAN_POINT('',(35.6544901166228,790.313745347917,101.635138095));
#71449=CARTESIAN_POINT('Ctrl Pts',(35.6547954302602,784.997496551132,109.118408634909));
#71450=CARTESIAN_POINT('Ctrl Pts',(35.6023362552077,784.99746368276,109.118463466802));
#71451=CARTESIAN_POINT('Ctrl Pts',(35.5499276664424,785.000559817699,109.119501560811));
#71452=CARTESIAN_POINT('Ctrl Pts',(35.4748183637044,785.009515828586,109.122411075434));
#71453=CARTESIAN_POINT('Ctrl Pts',(35.451845283349,785.012873836572,109.12349567397));
#71454=CARTESIAN_POINT('Ctrl Pts',(35.3789035841627,785.025516809238,109.127563385561));
#71455=CARTESIAN_POINT('Ctrl Pts',(35.3294234991337,785.037086900285,109.131265659108));
#71456=CARTESIAN_POINT('Ctrl Pts',(35.2073924451325,785.073225428222,109.14279919142));
#71457=CARTESIAN_POINT('Ctrl Pts',(35.1362154876891,785.101338101937,109.151749240883));
#71458=CARTESIAN_POINT('Ctrl Pts',(34.9260028488811,785.206763856821,109.185308769177));
#71459=CARTESIAN_POINT('Ctrl Pts',(34.7994566209819,785.303343773512,109.216042429876));
#71460=CARTESIAN_POINT('Ctrl Pts',(34.6042763552335,785.521913936625,109.285961961862));
#71461=CARTESIAN_POINT('Ctrl Pts',(34.5317505805344,785.63769143293,109.323126754227));
#71462=CARTESIAN_POINT('Ctrl Pts',(34.4263153853796,785.895713696395,109.40648561012));
#71463=CARTESIAN_POINT('Ctrl Pts',(34.3973405094104,786.037171543863,109.45246585178));
#71464=CARTESIAN_POINT('Ctrl Pts',(34.3930164084478,786.332746671641,109.549353509024));
#71465=CARTESIAN_POINT('Ctrl Pts',(34.4215593604839,786.484350661742,109.599500429788));
#71466=CARTESIAN_POINT('Ctrl Pts',(34.5389873956959,786.773457383948,109.69605211633));
#71467=CARTESIAN_POINT('Ctrl Pts',(34.6286257756405,786.907518738343,109.741339307826));
#71468=CARTESIAN_POINT('Ctrl Pts',(34.8553936006824,787.13262266724,109.818025567516));
#71469=CARTESIAN_POINT('Ctrl Pts',(34.9894375292637,787.222324758519,109.84893812918));
#71470=CARTESIAN_POINT('Ctrl Pts',(35.2299877882829,787.324594196331,109.884326347562));
#71471=CARTESIAN_POINT('Ctrl Pts',(35.3268177589307,787.353138209337,109.894250096422));
#71472=CARTESIAN_POINT('Ctrl Pts',(35.4839021678214,787.380486101967,109.90375848326));
#71473=CARTESIAN_POINT('Ctrl Pts',(35.542263123963,787.386709856269,109.905923084951));
#71474=CARTESIAN_POINT('Ctrl Pts',(35.626202679431,787.390090766529,109.907091867684));
#71475=CARTESIAN_POINT('Ctrl Pts',(35.6515620585677,787.390388537154,109.907192438922));
#71476=CARTESIAN_POINT('Ctrl Pts',(35.7004714487293,787.389568306025,109.906899429126));
#71477=CARTESIAN_POINT('Ctrl Pts',(35.724012903159,787.38854914281,109.906540366245));
#71478=CARTESIAN_POINT('Ctrl Pts',(35.8018783737722,787.383107682481,109.904629781023));
#71479=CARTESIAN_POINT('Ctrl Pts',(35.8559278107591,787.375979306361,109.902133143967));
#71480=CARTESIAN_POINT('Ctrl Pts',(35.9917086189071,787.349495923221,109.892874204745));
#71481=CARTESIAN_POINT('Ctrl Pts',(36.0721871295654,787.325669420196,109.884554034847));
#71482=CARTESIAN_POINT('Ctrl Pts',(36.3031927842254,787.232397628624,109.852089575935));
#71483=CARTESIAN_POINT('Ctrl Pts',(36.4422395725919,787.142063105976,109.820751230696));
#71484=CARTESIAN_POINT('Ctrl Pts',(36.6612453160988,786.928442619778,109.747444288974));
#71485=CARTESIAN_POINT('Ctrl Pts',(36.7445262595779,786.811916635859,109.70773192335));
#71486=CARTESIAN_POINT('Ctrl Pts',(36.8684825246604,786.548578270246,109.618930130974));
#71487=CARTESIAN_POINT('Ctrl Pts',(36.9050534097343,786.40262360428,109.570192486408));
#71488=CARTESIAN_POINT('Ctrl Pts',(36.9202890269026,786.096231476617,109.469009300794));
#71489=CARTESIAN_POINT('Ctrl Pts',(36.8951923414051,785.93845968691,109.417510657593));
#71490=CARTESIAN_POINT('Ctrl Pts',(36.782221356325,785.641467927504,109.321522024938));
#71491=CARTESIAN_POINT('Ctrl Pts',(36.6956398814662,785.505082966989,109.277933140005));
#71492=CARTESIAN_POINT('Ctrl Pts',(36.4755872336333,785.275605637353,109.20510404788));
#71493=CARTESIAN_POINT('Ctrl Pts',(36.3456948455117,785.183375207323,109.176107924705));
#71494=CARTESIAN_POINT('Ctrl Pts',(36.0760626338526,785.059292373403,109.137303069111));
#71495=CARTESIAN_POINT('Ctrl Pts',(35.9418479810997,785.021839732685,109.125703610021));
#71496=CARTESIAN_POINT('Ctrl Pts',(35.7544543225039,785.000384650602,109.119192547212));
#71497=CARTESIAN_POINT('Ctrl Pts',(35.7046473858209,784.997527785947,109.118356528159));
#71498=CARTESIAN_POINT('Ctrl Pts',(35.6547954302602,784.997496551132,109.118408634909));
#71499=CARTESIAN_POINT('Origin',(35.6544901166228,789.126363770955,101.215477269642));
#71500=CARTESIAN_POINT('',(35.6544901166228,787.462947139449,107.42237251313));
#71501=CARTESIAN_POINT('Origin',(35.6544901166228,786.99152490884,107.255755945863));
#71502=CARTESIAN_POINT('',(35.6544901166228,786.007855404895,111.5393856199));
#71503=CARTESIAN_POINT('',(35.6544901166228,789.597786001564,101.382093836909));
#71504=CARTESIAN_POINT('Origin',(35.6544901166228,785.536433174286,111.372769052633));
#71505=CARTESIAN_POINT('Origin',(38.7940239657454,783.999333857892,99.403411420971));
#71506=CARTESIAN_POINT('',(38.7940239657454,779.394310614873,109.367643766138));
#71507=CARTESIAN_POINT('',(38.7940239657454,781.363295832901,109.926921146904));
#71508=CARTESIAN_POINT('Ctrl Pts',(38.7940239657453,779.394310614873,109.367643766138));
#71509=CARTESIAN_POINT('Ctrl Pts',(38.6635349461688,779.393207383636,109.370765230824));
#71510=CARTESIAN_POINT('Ctrl Pts',(38.5342083152401,779.416399346092,109.380182277251));
#71511=CARTESIAN_POINT('Ctrl Pts',(38.2888290241497,779.510170214757,109.410878727397));
#71512=CARTESIAN_POINT('Ctrl Pts',(38.1756822099265,779.580985895905,109.432143641909));
#71513=CARTESIAN_POINT('Ctrl Pts',(37.9838549896053,779.761485508096,109.484183819058));
#71514=CARTESIAN_POINT('Ctrl Pts',(37.9072551623842,779.869578073241,109.514504437028));
#71515=CARTESIAN_POINT('Ctrl Pts',(37.8017537134914,780.108411515024,109.58084224068));
#71516=CARTESIAN_POINT('Ctrl Pts',(37.7739374450261,780.236881950785,109.616244705413));
#71517=CARTESIAN_POINT('Ctrl Pts',(37.7713755000717,780.497798391027,109.688304510556));
#71518=CARTESIAN_POINT('Ctrl Pts',(37.7970878703195,780.627733019712,109.724281755939));
#71519=CARTESIAN_POINT('Ctrl Pts',(37.8994698608417,780.869972587616,109.791750369839));
#71520=CARTESIAN_POINT('Ctrl Pts',(37.9750248536947,780.979934395059,109.82258688857));
#71521=CARTESIAN_POINT('Ctrl Pts',(38.1654495596747,781.164254064518,109.8743032276));
#71522=CARTESIAN_POINT('Ctrl Pts',(38.2780994460044,781.237108238932,109.894745419256));
#71523=CARTESIAN_POINT('Ctrl Pts',(38.5263339759862,781.336877902731,109.921917474556));
#71524=CARTESIAN_POINT('Ctrl Pts',(38.6594853898809,781.362783466954,109.928351139963));
#71525=CARTESIAN_POINT('Ctrl Pts',(38.7939741509504,781.363295644351,109.926921676737));
#71526=CARTESIAN_POINT('Ctrl Pts',(38.7939907559017,781.363295707588,109.926921500245));
#71527=CARTESIAN_POINT('Ctrl Pts',(38.7940073608334,781.363295770438,109.926921323634));
#71528=CARTESIAN_POINT('Ctrl Pts',(38.7940239657454,781.363295832901,109.926921146904));
#71529=CARTESIAN_POINT('',(38.7940239785527,781.951092439748,108.263818899095));
#71530=CARTESIAN_POINT('',(38.7940239657454,784.962362998135,99.7437785040383));
#71531=CARTESIAN_POINT('Ctrl Pts',(38.7941252323501,779.956131957018,107.778035528783));
#71532=CARTESIAN_POINT('Ctrl Pts',(38.7717982570025,779.956215312796,107.77779304053));
#71533=CARTESIAN_POINT('Ctrl Pts',(38.7494784386769,779.957016493482,107.777716414688));
#71534=CARTESIAN_POINT('Ctrl Pts',(38.7071993034286,779.959896357852,107.77788640697));
#71535=CARTESIAN_POINT('Ctrl Pts',(38.6872412690192,779.961835607304,107.778100784944));
#71536=CARTESIAN_POINT('Ctrl Pts',(38.6234800619274,779.969892971348,107.779217291371));
#71537=CARTESIAN_POINT('Ctrl Pts',(38.5800189399609,779.978221365635,107.780635739443));
#71538=CARTESIAN_POINT('Ctrl Pts',(38.4733597888644,780.005786882482,107.785778436175));
#71539=CARTESIAN_POINT('Ctrl Pts',(38.4112650578069,780.028311812588,107.790282402133));
#71540=CARTESIAN_POINT('Ctrl Pts',(38.2304860384765,780.114081553115,107.808156405804));
#71541=CARTESIAN_POINT('Ctrl Pts',(38.1219923371333,780.194451284638,107.825696855367));
#71542=CARTESIAN_POINT('Ctrl Pts',(37.9547601499314,780.378227595285,107.867196662891));
#71543=CARTESIAN_POINT('Ctrl Pts',(37.8925536783812,780.475872236695,107.889709764016));
#71544=CARTESIAN_POINT('Ctrl Pts',(37.8011983956067,780.694807928319,107.941223168081));
#71545=CARTESIAN_POINT('Ctrl Pts',(37.7755572834675,780.815533665404,107.9701642364));
#71546=CARTESIAN_POINT('Ctrl Pts',(37.769954637119,781.068558963853,108.031937760385));
#71547=CARTESIAN_POINT('Ctrl Pts',(37.7935051652747,781.198683872671,108.064320940692));
#71548=CARTESIAN_POINT('Ctrl Pts',(37.8908118600368,781.441895243009,108.125910441481));
#71549=CARTESIAN_POINT('Ctrl Pts',(37.9634303911922,781.552718258361,108.154533590756));
#71550=CARTESIAN_POINT('Ctrl Pts',(38.1467671682822,781.738631312653,108.203399195271));
#71551=CARTESIAN_POINT('Ctrl Pts',(38.2549051097159,781.812684561484,108.22333946862));
#71552=CARTESIAN_POINT('Ctrl Pts',(38.449377361593,781.897268171814,108.246811960939));
#71553=CARTESIAN_POINT('Ctrl Pts',(38.5279083013846,781.920896627017,108.253607234217));
#71554=CARTESIAN_POINT('Ctrl Pts',(38.6568967577939,781.943672007042,108.260648257632));
#71555=CARTESIAN_POINT('Ctrl Pts',(38.7058364234343,781.948801804334,108.262417759953));
#71556=CARTESIAN_POINT('Ctrl Pts',(38.7968213338433,781.951914662628,108.264055971153));
#71557=CARTESIAN_POINT('Ctrl Pts',(38.838723164895,781.95084253162,108.264166302565));
#71558=CARTESIAN_POINT('Ctrl Pts',(38.9285392607002,781.943158445415,108.263020921169));
#71559=CARTESIAN_POINT('Ctrl Pts',(38.9762780876931,781.935735056933,108.261555365153));
#71560=CARTESIAN_POINT('Ctrl Pts',(39.0990243848424,781.907870141158,108.255546324818));
#71561=CARTESIAN_POINT('Ctrl Pts',(39.1724825034312,781.88234186469,108.249690030792));
#71562=CARTESIAN_POINT('Ctrl Pts',(39.3645106741623,781.790518890985,108.228062343069));
#71563=CARTESIAN_POINT('Ctrl Pts',(39.4734992058981,781.708941552887,108.208368670797));
#71564=CARTESIAN_POINT('Ctrl Pts',(39.6417942305272,781.520949901741,108.162743628668));
#71565=CARTESIAN_POINT('Ctrl Pts',(39.7041303056591,781.420051168054,108.138179679678));
#71566=CARTESIAN_POINT('Ctrl Pts',(39.7930469243524,781.194622883409,108.083395275582));
#71567=CARTESIAN_POINT('Ctrl Pts',(39.8161856608473,781.07090148787,108.053381528825));
#71568=CARTESIAN_POINT('Ctrl Pts',(39.8145910060359,780.813453807,107.991079118705));
#71569=CARTESIAN_POINT('Ctrl Pts',(39.7866483271373,780.682070359643,107.959366200801));
#71570=CARTESIAN_POINT('Ctrl Pts',(39.680502460119,780.439521693832,107.900731119095));
#71571=CARTESIAN_POINT('Ctrl Pts',(39.6040659813743,780.330365021441,107.874287509353));
#71572=CARTESIAN_POINT('Ctrl Pts',(39.4167249560214,780.151573518842,107.830468416537));
#71573=CARTESIAN_POINT('Ctrl Pts',(39.3093051606854,780.081890568166,107.813103271351));
#71574=CARTESIAN_POINT('Ctrl Pts',(39.1092107426472,779.999803301894,107.791801995607));
#71575=CARTESIAN_POINT('Ctrl Pts',(39.0228489620844,779.976801574484,107.785486260207));
#71576=CARTESIAN_POINT('Ctrl Pts',(38.8879679640875,779.958955767925,107.779787654166));
#71577=CARTESIAN_POINT('Ctrl Pts',(38.8410741021507,779.955956677588,107.778545429889));
#71578=CARTESIAN_POINT('Ctrl Pts',(38.7941252323501,779.956131957018,107.778035528783));
#71579=CARTESIAN_POINT('Ctrl Pts',(38.7940239657454,781.363295832901,109.926921146904));
#71580=CARTESIAN_POINT('Ctrl Pts',(38.9271033661578,781.36379643565,109.925504749551));
#71581=CARTESIAN_POINT('Ctrl Pts',(39.0589168714063,781.339426030814,109.916406030783));
#71582=CARTESIAN_POINT('Ctrl Pts',(39.3066501931785,781.243147914772,109.883523984144));
#71583=CARTESIAN_POINT('Ctrl Pts',(39.419915521759,781.171607115591,109.859889198305));
#71584=CARTESIAN_POINT('Ctrl Pts',(39.6103838098438,780.990699904101,109.801715818852));
#71585=CARTESIAN_POINT('Ctrl Pts',(39.6858212226316,780.883217206252,109.767797720514));
#71586=CARTESIAN_POINT('Ctrl Pts',(39.7890053443797,780.645542422123,109.694733020183));
#71587=CARTESIAN_POINT('Ctrl Pts',(39.8155355248429,780.517612882452,109.656308445813));
#71588=CARTESIAN_POINT('Ctrl Pts',(39.8153290314093,780.259446696781,109.581104571311));
#71589=CARTESIAN_POINT('Ctrl Pts',(39.7889372378603,780.131729598482,109.545052014377));
#71590=CARTESIAN_POINT('Ctrl Pts',(39.6867045289745,779.892704916431,109.479987305234));
#71591=CARTESIAN_POINT('Ctrl Pts',(39.6118483159403,779.78366064126,109.451584439574));
#71592=CARTESIAN_POINT('Ctrl Pts',(39.4234816594619,779.599339561651,109.405894216676));
#71593=CARTESIAN_POINT('Ctrl Pts',(39.3118682787941,779.525676509119,109.388982729106));
#71594=CARTESIAN_POINT('Ctrl Pts',(39.0663780401034,779.423854589174,109.368235081468));
#71595=CARTESIAN_POINT('Ctrl Pts',(38.9349087847057,779.396525332607,109.364541127432));
#71596=CARTESIAN_POINT('Ctrl Pts',(38.7992650647418,779.39436471664,109.36752095019));
#71597=CARTESIAN_POINT('Ctrl Pts',(38.7966442807793,779.394332768564,109.367581084842));
#71598=CARTESIAN_POINT('Ctrl Pts',(38.7940239657454,779.394310614874,109.367643766138));
#71599=CARTESIAN_POINT('Origin',(38.7940239657454,783.999333857892,99.403411420971));
#71600=CARTESIAN_POINT('',(38.7940239657454,782.335917226386,105.610306664459));
#71601=CARTESIAN_POINT('Origin',(38.7940239657454,781.864494995777,105.443690097192));
#71602=CARTESIAN_POINT('',(38.7940239657455,780.86401645488,109.774878989525));
#71603=CARTESIAN_POINT('',(38.7940239657454,784.470756088501,99.5700279882381));
#71604=CARTESIAN_POINT('Ctrl Pts',(38.7940134537644,779.900130022071,109.501181670678));
#71605=CARTESIAN_POINT('Ctrl Pts',(38.7331652254187,779.899685911755,109.502442068218));
#71606=CARTESIAN_POINT('Ctrl Pts',(38.6728198670922,779.909992103199,109.506617340839));
#71607=CARTESIAN_POINT('Ctrl Pts',(38.554769845173,779.952671412073,109.520882982605));
#71608=CARTESIAN_POINT('Ctrl Pts',(38.4987817926341,779.986234012438,109.531255916666));
#71609=CARTESIAN_POINT('Ctrl Pts',(38.4033499215098,780.072528529065,109.556908581401));
#71610=CARTESIAN_POINT('Ctrl Pts',(38.3649085626957,780.124480117025,109.571956667297));
#71611=CARTESIAN_POINT('Ctrl Pts',(38.3110385487116,780.239904350712,109.604916405902));
#71612=CARTESIAN_POINT('Ctrl Pts',(38.2961754871977,780.302280958421,109.622518437702));
#71613=CARTESIAN_POINT('Ctrl Pts',(38.2922864000264,780.429680183009,109.658246329906));
#71614=CARTESIAN_POINT('Ctrl Pts',(38.3035620976856,780.493479633859,109.676029847614));
#71615=CARTESIAN_POINT('Ctrl Pts',(38.3513481199104,780.613367305899,109.70928158051));
#71616=CARTESIAN_POINT('Ctrl Pts',(38.3874751602821,780.668243250305,109.724412540661));
#71617=CARTESIAN_POINT('Ctrl Pts',(38.4796635603617,780.760954307424,109.749677264535));
#71618=CARTESIAN_POINT('Ctrl Pts',(38.5347076160494,780.797957298672,109.759582328796));
#71619=CARTESIAN_POINT('Ctrl Pts',(38.6565040388531,780.849181732395,109.772649652012));
#71620=CARTESIAN_POINT('Ctrl Pts',(38.7220319881178,780.862905639468,109.775680761675));
#71621=CARTESIAN_POINT('Ctrl Pts',(38.8548068665812,780.865010636589,109.774218698247));
#71622=CARTESIAN_POINT('Ctrl Pts',(38.9207215027086,780.85334476714,109.769729672175));
#71623=CARTESIAN_POINT('Ctrl Pts',(39.0437830252023,780.805958802169,109.753726404538));
#71624=CARTESIAN_POINT('Ctrl Pts',(39.0996984050641,780.770725369361,109.742377051878));
#71625=CARTESIAN_POINT('Ctrl Pts',(39.1937617655332,780.681304018546,109.714429983369));
#71626=CARTESIAN_POINT('Ctrl Pts',(39.2309813150243,780.62802482522,109.698119994925));
#71627=CARTESIAN_POINT('Ctrl Pts',(39.2816007843049,780.510309578999,109.66286077316));
#71628=CARTESIAN_POINT('Ctrl Pts',(39.2944278342269,780.447020073884,109.644261590856));
#71629=CARTESIAN_POINT('Ctrl Pts',(39.2936060490897,780.319935487117,109.607738208716));
#71630=CARTESIAN_POINT('Ctrl Pts',(39.2803046369429,780.257381042135,109.590162038697));
#71631=CARTESIAN_POINT('Ctrl Pts',(39.2294872958762,780.140596593304,109.558184273771));
#71632=CARTESIAN_POINT('Ctrl Pts',(39.1924764666662,780.087469683158,109.544082686883));
#71633=CARTESIAN_POINT('Ctrl Pts',(39.099563435551,779.997919820937,109.521177493141));
#71634=CARTESIAN_POINT('Ctrl Pts',(39.0445971580782,779.962297891029,109.51257219115));
#71635=CARTESIAN_POINT('Ctrl Pts',(38.923852863808,779.913433836878,109.501856959151));
#71636=CARTESIAN_POINT('Ctrl Pts',(38.8592616191411,779.900606246017,109.499830133758));
#71637=CARTESIAN_POINT('Ctrl Pts',(38.7940134537644,779.900130022071,109.501181670678));
#71638=CARTESIAN_POINT('Origin',(43.3168648737812,778.988051266838,97.6322545923071));
#71639=CARTESIAN_POINT('',(43.3168648737812,774.257710238126,108.171096695511));
#71640=CARTESIAN_POINT('',(43.3168648737814,776.151024833139,108.504400048628));
#71641=CARTESIAN_POINT('Ctrl Pts',(43.3168648737811,774.257710238126,108.171096695511));
#71642=CARTESIAN_POINT('Ctrl Pts',(43.1997889459331,774.256411461088,108.174771434332));
#71643=CARTESIAN_POINT('Ctrl Pts',(43.0836809340222,774.276907434386,108.181853420389));
#71644=CARTESIAN_POINT('Ctrl Pts',(42.8587797518068,774.361923392078,108.202728140363));
#71645=CARTESIAN_POINT('Ctrl Pts',(42.7533149370578,774.427996104428,108.216658299341));
#71646=CARTESIAN_POINT('Ctrl Pts',(42.5725818214765,774.598386769129,108.249907769786));
#71647=CARTESIAN_POINT('Ctrl Pts',(42.4997983366597,774.701633843668,108.268988797232));
#71648=CARTESIAN_POINT('Ctrl Pts',(42.398003120726,774.931950151518,108.310324525063));
#71649=CARTESIAN_POINT('Ctrl Pts',(42.3707207599739,775.057192487492,108.33224420223));
#71650=CARTESIAN_POINT('Ctrl Pts',(42.3670375822734,775.310927938652,108.376041434313));
#71651=CARTESIAN_POINT('Ctrl Pts',(42.390728083664,775.437135635385,108.397529791516));
#71652=CARTESIAN_POINT('Ctrl Pts',(42.4858363338574,775.671275521423,108.436823330913));
#71653=CARTESIAN_POINT('Ctrl Pts',(42.5556801279478,775.777318844528,108.454316668448));
#71654=CARTESIAN_POINT('Ctrl Pts',(42.7322371250952,775.955721747957,108.48268721344));
#71655=CARTESIAN_POINT('Ctrl Pts',(42.8368789628639,776.026658532097,108.493338344764));
#71656=CARTESIAN_POINT('Ctrl Pts',(43.0677886888812,776.124200473689,108.505821338737));
#71657=CARTESIAN_POINT('Ctrl Pts',(43.1916145190988,776.149916964495,108.507534634318));
#71658=CARTESIAN_POINT('Ctrl Pts',(43.3168648737817,776.151024833139,108.504400048628));
#71659=CARTESIAN_POINT('',(43.3168650111487,776.615095621064,107.191365639192));
#71660=CARTESIAN_POINT('',(43.3168648737812,779.881947439457,97.9481877454437));
#71661=CARTESIAN_POINT('Ctrl Pts',(43.3169432955444,774.709698431335,106.892248594599));
#71662=CARTESIAN_POINT('Ctrl Pts',(43.2916025682699,774.709912156225,106.891637594698));
#71663=CARTESIAN_POINT('Ctrl Pts',(43.2662785675948,774.711151510538,106.891173520281));
#71664=CARTESIAN_POINT('Ctrl Pts',(43.1914778887744,774.717848091664,106.890238296377));
#71665=CARTESIAN_POINT('Ctrl Pts',(43.1423556364478,774.72620547009,106.89019199734));
#71666=CARTESIAN_POINT('Ctrl Pts',(43.0313357479768,774.754234755326,106.891415707021));
#71667=CARTESIAN_POINT('Ctrl Pts',(42.9703725212796,774.776475472245,106.893082917823));
#71668=CARTESIAN_POINT('Ctrl Pts',(42.8038921843578,774.857168113161,106.900603511246));
#71669=CARTESIAN_POINT('Ctrl Pts',(42.7066589318352,774.929552839227,106.908753210904));
#71670=CARTESIAN_POINT('Ctrl Pts',(42.5498762981391,775.099319630695,106.930126868861));
#71671=CARTESIAN_POINT('Ctrl Pts',(42.4892198667589,775.193263454763,106.942786202768));
#71672=CARTESIAN_POINT('Ctrl Pts',(42.3992430673852,775.404589368925,106.972970371438));
#71673=CARTESIAN_POINT('Ctrl Pts',(42.3732901755161,775.521580003357,106.990560624007));
#71674=CARTESIAN_POINT('Ctrl Pts',(42.3650763894248,775.766564702822,107.029159607396));
#71675=CARTESIAN_POINT('Ctrl Pts',(42.3859669946615,775.892605645028,107.049978821053));
#71676=CARTESIAN_POINT('Ctrl Pts',(42.4753790497857,776.126867070568,107.090377825187));
#71677=CARTESIAN_POINT('Ctrl Pts',(42.5422302186713,776.23318554235,107.109590038852));
#71678=CARTESIAN_POINT('Ctrl Pts',(42.7123975957046,776.411983125607,107.143434630939));
#71679=CARTESIAN_POINT('Ctrl Pts',(42.813289673547,776.483334619936,107.157809112372));
#71680=CARTESIAN_POINT('Ctrl Pts',(42.9976768306654,776.565590843421,107.175901933663));
#71681=CARTESIAN_POINT('Ctrl Pts',(43.0737952876244,776.588611330745,107.181514182836));
#71682=CARTESIAN_POINT('Ctrl Pts',(43.2050472441892,776.610831894175,107.18819191073));
#71683=CARTESIAN_POINT('Ctrl Pts',(43.2587849691808,776.615268834182,107.190126376709));
#71684=CARTESIAN_POINT('Ctrl Pts',(43.3368949521302,776.615048573204,107.191795193994));
#71685=CARTESIAN_POINT('Ctrl Pts',(43.3611452981077,776.614048983843,107.192153792773));
#71686=CARTESIAN_POINT('Ctrl Pts',(43.4380116491318,776.607922795436,107.192785236627));
#71687=CARTESIAN_POINT('Ctrl Pts',(43.4902448310117,776.599333853516,107.192458039042));
#71688=CARTESIAN_POINT('Ctrl Pts',(43.6143666224452,776.56814802355,107.189859135102));
#71689=CARTESIAN_POINT('Ctrl Pts',(43.6847685628978,776.54128895514,107.186834684274));
#71690=CARTESIAN_POINT('Ctrl Pts',(43.8636259881094,776.447702018633,107.17496477402));
#71691=CARTESIAN_POINT('Ctrl Pts',(43.9629224883099,776.367243756333,107.163671038405));
#71692=CARTESIAN_POINT('Ctrl Pts',(44.1160839257071,776.182866466268,107.136709568032));
#71693=CARTESIAN_POINT('Ctrl Pts',(44.172354506465,776.083624610569,107.121822623364));
#71694=CARTESIAN_POINT('Ctrl Pts',(44.2503317040309,775.863170793678,107.08831273556));
#71695=CARTESIAN_POINT('Ctrl Pts',(44.2687223641544,775.742707419449,107.069779404458));
#71696=CARTESIAN_POINT('Ctrl Pts',(44.259612352217,775.493922253699,107.031097509907));
#71697=CARTESIAN_POINT('Ctrl Pts',(44.2292053396555,775.367804321865,107.011264511283));
#71698=CARTESIAN_POINT('Ctrl Pts',(44.1217941034704,775.138808117992,106.974497329291));
#71699=CARTESIAN_POINT('Ctrl Pts',(44.0472299995365,775.037383156253,106.95781273974));
#71700=CARTESIAN_POINT('Ctrl Pts',(43.8645121774589,774.871228617837,106.92915962184));
#71701=CARTESIAN_POINT('Ctrl Pts',(43.7589390086845,774.807351301255,106.91736525756));
#71702=CARTESIAN_POINT('Ctrl Pts',(43.571472191739,774.739427657388,106.902928350702));
#71703=CARTESIAN_POINT('Ctrl Pts',(43.4962200622162,774.722243139992,106.898576271112));
#71704=CARTESIAN_POINT('Ctrl Pts',(43.3855168802414,774.710999060835,106.894170355902));
#71705=CARTESIAN_POINT('Ctrl Pts',(43.3512401635335,774.709409169933,106.893075539411));
#71706=CARTESIAN_POINT('Ctrl Pts',(43.3169432955444,774.709698431335,106.892248594599));
#71707=CARTESIAN_POINT('Ctrl Pts',(43.3168648737817,776.151024833139,108.504400048628));
#71708=CARTESIAN_POINT('Ctrl Pts',(43.3169501287949,776.151025587239,108.504397914989));
#71709=CARTESIAN_POINT('Ctrl Pts',(43.3170353844682,776.151026329935,108.504395779109));
#71710=CARTESIAN_POINT('Ctrl Pts',(43.3171206407995,776.151027061225,108.504393640989));
#71711=CARTESIAN_POINT('Ctrl Pts',(43.4355136039576,776.152042581919,108.501424496826));
#71712=CARTESIAN_POINT('Ctrl Pts',(43.5528642729635,776.131046769687,108.494177999891));
#71713=CARTESIAN_POINT('Ctrl Pts',(43.7797464004146,776.044763126869,108.471240762669));
#71714=CARTESIAN_POINT('Ctrl Pts',(43.8860081083987,775.977869599269,108.455327829206));
#71715=CARTESIAN_POINT('Ctrl Pts',(44.0658810353981,775.806796758588,108.417518461765));
#71716=CARTESIAN_POINT('Ctrl Pts',(44.1375564214189,775.704304443765,108.396013449576));
#71717=CARTESIAN_POINT('Ctrl Pts',(44.2370134195534,775.476452463699,108.350677577371));
#71718=CARTESIAN_POINT('Ctrl Pts',(44.263369533438,775.353125065724,108.327285004586));
#71719=CARTESIAN_POINT('Ctrl Pts',(44.2664140159794,775.101257501571,108.2820056959));
#71720=CARTESIAN_POINT('Ctrl Pts',(44.2423238519086,774.975022664943,108.260573808016));
#71721=CARTESIAN_POINT('Ctrl Pts',(44.1469186354503,774.741289399089,108.223349987931));
#71722=CARTESIAN_POINT('Ctrl Pts',(44.0774089508596,774.635485043324,108.207767424861));
#71723=CARTESIAN_POINT('Ctrl Pts',(43.9029192305033,774.45765507229,108.183950529821));
#71724=CARTESIAN_POINT('Ctrl Pts',(43.8001315532888,774.386653024556,108.17579414174));
#71725=CARTESIAN_POINT('Ctrl Pts',(43.5745041424813,774.288294926036,108.167394418138));
#71726=CARTESIAN_POINT('Ctrl Pts',(43.4541499450961,774.261311437038,108.167116988508));
#71727=CARTESIAN_POINT('Ctrl Pts',(43.3269438906221,774.257862392255,108.170786729149));
#71728=CARTESIAN_POINT('Ctrl Pts',(43.3219034854246,774.257766133759,108.170938545307));
#71729=CARTESIAN_POINT('Ctrl Pts',(43.3168648737811,774.257710238126,108.171096695511));
#71730=CARTESIAN_POINT('Origin',(43.3168648737812,778.988051266838,97.6322545923071));
#71731=CARTESIAN_POINT('',(43.3168648737812,777.324634635332,103.839149835795));
#71732=CARTESIAN_POINT('Origin',(43.3168648737812,776.853212404723,103.672533268528));
#71733=CARTESIAN_POINT('',(43.3168648737813,775.706104888437,108.418591821086));
#71734=CARTESIAN_POINT('',(43.3168648737812,779.459473497447,97.7988711595741));
#71735=CARTESIAN_POINT('Ctrl Pts',(43.3168503266343,774.70758740764,108.242879031684));
#71736=CARTESIAN_POINT('Ctrl Pts',(43.2550682844173,774.706935028639,108.244730256454));
#71737=CARTESIAN_POINT('Ctrl Pts',(43.193823506189,774.717759010054,108.248471851981));
#71738=CARTESIAN_POINT('Ctrl Pts',(43.0752989715982,774.762508820301,108.259670623897));
#71739=CARTESIAN_POINT('Ctrl Pts',(43.0197247862468,774.79724439007,108.267209108575));
#71740=CARTESIAN_POINT('Ctrl Pts',(42.9245342076126,774.886766279282,108.2852145568));
#71741=CARTESIAN_POINT('Ctrl Pts',(42.8861964492455,774.940962188479,108.295546493636));
#71742=CARTESIAN_POINT('Ctrl Pts',(42.8322758868149,775.062406211994,108.317906051551));
#71743=CARTESIAN_POINT('Ctrl Pts',(42.8178102587603,775.128756576984,108.329753951295));
#71744=CARTESIAN_POINT('Ctrl Pts',(42.8160129070241,775.262862992254,108.353142511379));
#71745=CARTESIAN_POINT('Ctrl Pts',(42.8285836005518,775.329393357407,108.364473180029));
#71746=CARTESIAN_POINT('Ctrl Pts',(42.8789928241664,775.453201577646,108.385013777053));
#71747=CARTESIAN_POINT('Ctrl Pts',(42.9161449838627,775.509428205282,108.394053274978));
#71748=CARTESIAN_POINT('Ctrl Pts',(43.0101178256596,775.603988858005,108.408505009329));
#71749=CARTESIAN_POINT('Ctrl Pts',(43.0658721367692,775.641536067018,108.413800454879));
#71750=CARTESIAN_POINT('Ctrl Pts',(43.1872698849458,775.692169429266,108.419674199264));
#71751=CARTESIAN_POINT('Ctrl Pts',(43.2513862686608,775.70540853512,108.420318980157));
#71752=CARTESIAN_POINT('Ctrl Pts',(43.3809545301484,775.706787231306,108.416901440254));
#71753=CARTESIAN_POINT('Ctrl Pts',(43.4450683019003,775.694967030789,108.41288325223));
#71754=CARTESIAN_POINT('Ctrl Pts',(43.5659481755348,775.647244426328,108.400577172761));
#71755=CARTESIAN_POINT('Ctrl Pts',(43.6212926952439,775.611458228687,108.39235270157));
#71756=CARTESIAN_POINT('Ctrl Pts',(43.7153285625206,775.520007538906,108.372796375814));
#71757=CARTESIAN_POINT('Ctrl Pts',(43.7527737650026,775.465010586555,108.361628112382));
#71758=CARTESIAN_POINT('Ctrl Pts',(43.8039815725099,775.343242807349,108.338041781264));
#71759=CARTESIAN_POINT('Ctrl Pts',(43.8170502786639,775.277577267703,108.325849305159));
#71760=CARTESIAN_POINT('Ctrl Pts',(43.8166738351301,775.144318022938,108.302185190506));
#71761=CARTESIAN_POINT('Ctrl Pts',(43.802996267905,775.077944109442,108.290940650918));
#71762=CARTESIAN_POINT('Ctrl Pts',(43.7508744080774,774.955503435521,108.271265687373));
#71763=CARTESIAN_POINT('Ctrl Pts',(43.7134089410029,774.900319559939,108.262951444371));
#71764=CARTESIAN_POINT('Ctrl Pts',(43.6199682076064,774.808010507736,108.250148038055));
#71765=CARTESIAN_POINT('Ctrl Pts',(43.5651553995317,774.771439202618,108.245711149419));
#71766=CARTESIAN_POINT('Ctrl Pts',(43.4452175081836,774.721463704055,108.241114382368));
#71767=CARTESIAN_POINT('Ctrl Pts',(43.3814051537084,774.708269065483,108.240944723743));
#71768=CARTESIAN_POINT('Ctrl Pts',(43.3168503266343,774.70758740764,108.242879031684));
#71769=CARTESIAN_POINT('Origin',(29.1099152851011,787.750281848153,100.729123357227));
#71770=CARTESIAN_POINT('',(29.1099152851011,783.147271975424,110.687659104939));
#71771=CARTESIAN_POINT('',(29.1099152851012,785.112934988763,111.256336278119));
#71772=CARTESIAN_POINT('Ctrl Pts',(29.1099152851011,783.147271975424,110.687659104939));
#71773=CARTESIAN_POINT('Ctrl Pts',(28.9787483332411,783.145433331028,110.692861335767));
#71774=CARTESIAN_POINT('Ctrl Pts',(28.8487346582336,783.168046709765,110.70469804998));
#71775=CARTESIAN_POINT('Ctrl Pts',(28.6032732367854,783.260735106295,110.74031249655));
#71776=CARTESIAN_POINT('Ctrl Pts',(28.4905625898534,783.330655829655,110.763922498915));
#71777=CARTESIAN_POINT('Ctrl Pts',(28.2993559915101,783.509432962389,110.820051965965));
#71778=CARTESIAN_POINT('Ctrl Pts',(28.2229742882335,783.6167202065,110.85206760072));
#71779=CARTESIAN_POINT('Ctrl Pts',(28.1175997654022,783.854467596885,110.920842468896));
#71780=CARTESIAN_POINT('Ctrl Pts',(28.0898122652965,783.98268545845,110.956961640161));
#71781=CARTESIAN_POINT('Ctrl Pts',(28.0872917990849,784.242317633029,111.029077359832));
#71782=CARTESIAN_POINT('Ctrl Pts',(28.1125710043552,784.371250162536,111.064400207693));
#71783=CARTESIAN_POINT('Ctrl Pts',(28.2140091567208,784.61408460271,111.130437573787));
#71784=CARTESIAN_POINT('Ctrl Pts',(28.2898721071226,784.725354188797,111.160436223417));
#71785=CARTESIAN_POINT('Ctrl Pts',(28.4810730060538,784.911526158526,111.209964033082));
#71786=CARTESIAN_POINT('Ctrl Pts',(28.5940093658696,784.985059931315,111.229130498158));
#71787=CARTESIAN_POINT('Ctrl Pts',(28.8424384690884,785.085710925819,111.253707018508));
#71788=CARTESIAN_POINT('Ctrl Pts',(28.975406862261,785.112001002839,111.258904477997));
#71789=CARTESIAN_POINT('Ctrl Pts',(29.1097268752779,785.112933697117,111.256339880534));
#71790=CARTESIAN_POINT('Ctrl Pts',(29.1097896788289,785.112934133213,111.256338681414));
#71791=CARTESIAN_POINT('Ctrl Pts',(29.1098524821037,785.112934563762,111.256337480609));
#71792=CARTESIAN_POINT('Ctrl Pts',(29.1099152851014,785.112934988763,111.256336278119));
#71793=CARTESIAN_POINT('',(29.1099152827985,785.751926387763,109.448384310331));
#71794=CARTESIAN_POINT('',(29.1099152851011,788.713310988396,101.069490440295));
#71795=CARTESIAN_POINT('Ctrl Pts',(29.1098761559961,783.783777209309,108.886741454917));
#71796=CARTESIAN_POINT('Ctrl Pts',(29.0202287505466,783.782651395279,108.889937120993));
#71797=CARTESIAN_POINT('Ctrl Pts',(28.9309471570873,783.792927405918,108.896289886262));
#71798=CARTESIAN_POINT('Ctrl Pts',(28.7990746032532,783.82557523518,108.910478138312));
#71799=CARTESIAN_POINT('Ctrl Pts',(28.7547021140882,783.839790686475,108.916140937024));
#71800=CARTESIAN_POINT('Ctrl Pts',(28.693668843277,783.864005294673,108.925208871393));
#71801=CARTESIAN_POINT('Ctrl Pts',(28.6760225836916,783.871586815564,108.927989911544));
#71802=CARTESIAN_POINT('Ctrl Pts',(28.6430773370826,783.886853839333,108.933487141561));
#71803=CARTESIAN_POINT('Ctrl Pts',(28.6277350233886,783.894438495488,108.936177399633));
#71804=CARTESIAN_POINT('Ctrl Pts',(28.5793647875507,783.919888781342,108.945080746947));
#71805=CARTESIAN_POINT('Ctrl Pts',(28.5471872541053,783.939173519489,108.951649044907));
#71806=CARTESIAN_POINT('Ctrl Pts',(28.4699608361721,783.991521328781,108.969076731593));
#71807=CARTESIAN_POINT('Ctrl Pts',(28.4265443682553,784.026590968006,108.980421608421));
#71808=CARTESIAN_POINT('Ctrl Pts',(28.3001221336293,784.147626083841,109.018661655491));
#71809=CARTESIAN_POINT('Ctrl Pts',(28.2301070425694,784.244716468015,109.048106650153));
#71810=CARTESIAN_POINT('Ctrl Pts',(28.132682303859,784.451124605322,109.108898530641));
#71811=CARTESIAN_POINT('Ctrl Pts',(28.1033621835979,784.55769513117,109.139553905886));
#71812=CARTESIAN_POINT('Ctrl Pts',(28.0815893348599,784.784169783905,109.203527275506));
#71813=CARTESIAN_POINT('Ctrl Pts',(28.0922331544423,784.902673246739,109.236368840142));
#71814=CARTESIAN_POINT('Ctrl Pts',(28.1584798739867,785.138465004452,109.300651731836));
#71815=CARTESIAN_POINT('Ctrl Pts',(28.2165006037512,785.252995534348,109.331270729447));
#71816=CARTESIAN_POINT('Ctrl Pts',(28.3766173930253,785.458603801005,109.384974672869));
#71817=CARTESIAN_POINT('Ctrl Pts',(28.4786090373902,785.546735662626,109.407239684852));
#71818=CARTESIAN_POINT('Ctrl Pts',(28.7084761035384,785.677932617153,109.438371460242));
#71819=CARTESIAN_POINT('Ctrl Pts',(28.8333423905459,785.721061493646,109.447326013261));
#71820=CARTESIAN_POINT('Ctrl Pts',(29.0806312716797,785.757873925994,109.450955844317));
#71821=CARTESIAN_POINT('Ctrl Pts',(29.200274304189,785.755550876228,109.446862986797));
#71822=CARTESIAN_POINT('Ctrl Pts',(29.3711115561848,785.723209312974,109.432419198064));
#71823=CARTESIAN_POINT('Ctrl Pts',(29.4245786574587,785.708632186141,109.426579559483));
#71824=CARTESIAN_POINT('Ctrl Pts',(29.5119641176442,785.67716942096,109.414763994875));
#71825=CARTESIAN_POINT('Ctrl Pts',(29.5466365298866,785.662506178878,109.409427815552));
#71826=CARTESIAN_POINT('Ctrl Pts',(29.5956714241808,785.638527670092,109.400916731226));
#71827=CARTESIAN_POINT('Ctrl Pts',(29.6107798755938,785.630666971371,109.398153735095));
#71828=CARTESIAN_POINT('Ctrl Pts',(29.6599117960034,785.603524165089,109.388698536729));
#71829=CARTESIAN_POINT('Ctrl Pts',(29.6929569172784,785.582698766549,109.381574653211));
#71830=CARTESIAN_POINT('Ctrl Pts',(29.7745389746346,785.524427593713,109.361950288889));
#71831=CARTESIAN_POINT('Ctrl Pts',(29.8208810640803,785.484435772604,109.348755521566));
#71832=CARTESIAN_POINT('Ctrl Pts',(29.9517215936083,785.348516600507,109.304700512644));
#71833=CARTESIAN_POINT('Ctrl Pts',(30.0208613487702,785.240743531152,109.270790110757));
#71834=CARTESIAN_POINT('Ctrl Pts',(30.1074039202553,785.018976884056,109.20297685208));
#71835=CARTESIAN_POINT('Ctrl Pts',(30.1291758558536,784.908726368771,109.170019179988));
#71836=CARTESIAN_POINT('Ctrl Pts',(30.1333197859797,784.677076963654,109.102504484767));
#71837=CARTESIAN_POINT('Ctrl Pts',(30.1125607153376,784.55741217819,109.068586766506));
#71838=CARTESIAN_POINT('Ctrl Pts',(30.024295720814,784.322417252564,109.004138224049));
#71839=CARTESIAN_POINT('Ctrl Pts',(29.954352866702,784.210271276886,108.974647794333));
#71840=CARTESIAN_POINT('Ctrl Pts',(29.7827806717245,784.027129496309,108.929036325172));
#71841=CARTESIAN_POINT('Ctrl Pts',(29.6862569985383,783.954587292616,108.91223455758));
#71842=CARTESIAN_POINT('Ctrl Pts',(29.5153336234898,783.867209843521,108.894253133582));
#71843=CARTESIAN_POINT('Ctrl Pts',(29.4483240993924,783.841142549999,108.889548585355));
#71844=CARTESIAN_POINT('Ctrl Pts',(29.2914060860322,783.797796476869,108.883536508149));
#71845=CARTESIAN_POINT('Ctrl Pts',(29.2008614875201,783.784919825343,108.883498095715));
#71846=CARTESIAN_POINT('Ctrl Pts',(29.1098761559961,783.783777209309,108.886741454917));
#71847=CARTESIAN_POINT('Ctrl Pts',(29.1099152851014,785.112934988763,111.256336278119));
#71848=CARTESIAN_POINT('Ctrl Pts',(29.2417187854962,785.113826929972,111.253812634032));
#71849=CARTESIAN_POINT('Ctrl Pts',(29.3723014451918,785.090289281962,111.243847695462));
#71850=CARTESIAN_POINT('Ctrl Pts',(29.6195013119506,784.995965598073,111.209284433721));
#71851=CARTESIAN_POINT('Ctrl Pts',(29.7332620403393,784.924991413875,111.184676204043));
#71852=CARTESIAN_POINT('Ctrl Pts',(29.9246539146689,784.745029752424,111.124318273611));
#71853=CARTESIAN_POINT('Ctrl Pts',(30.000521891227,784.63793575237,111.089210763936));
#71854=CARTESIAN_POINT('Ctrl Pts',(30.1041612235064,784.401495571549,111.013792466794));
#71855=CARTESIAN_POINT('Ctrl Pts',(30.1309721341953,784.274500123432,110.974249691163));
#71856=CARTESIAN_POINT('Ctrl Pts',(30.1316710389441,784.016053870509,110.896410747585));
#71857=CARTESIAN_POINT('Ctrl Pts',(30.105110186717,783.88715069737,110.858919261452));
#71858=CARTESIAN_POINT('Ctrl Pts',(30.0019418635203,783.64717626582,110.792216295676));
#71859=CARTESIAN_POINT('Ctrl Pts',(29.9268641669351,783.538233544062,110.763561784645));
#71860=CARTESIAN_POINT('Ctrl Pts',(29.7379565707489,783.353748398758,110.718399153832));
#71861=CARTESIAN_POINT('Ctrl Pts',(29.6259787794184,783.279879865624,110.702282096702));
#71862=CARTESIAN_POINT('Ctrl Pts',(29.3799365456471,783.177551001541,110.684210113816));
#71863=CARTESIAN_POINT('Ctrl Pts',(29.2482733293954,783.149880421077,110.682355112769));
#71864=CARTESIAN_POINT('Ctrl Pts',(29.1133855354354,783.147324894626,110.687522642653));
#71865=CARTESIAN_POINT('Ctrl Pts',(29.1116503093094,783.147296296281,110.687590291901));
#71866=CARTESIAN_POINT('Ctrl Pts',(29.1099152851011,783.147271975424,110.687659104939));
#71867=CARTESIAN_POINT('Origin',(29.1099152851011,787.750281848153,100.729123357227));
#71868=CARTESIAN_POINT('',(29.1099152851011,786.086865216647,106.936018600716));
#71869=CARTESIAN_POINT('Origin',(29.1099152851011,785.615442986038,106.769402033449));
#71870=CARTESIAN_POINT('',(29.1099152851012,784.6139997576,111.103320397167));
#71871=CARTESIAN_POINT('',(29.1099152851011,788.221704078762,100.895739924495));
#71872=CARTESIAN_POINT('Ctrl Pts',(29.1096415055408,783.651752382614,110.824985779127));
#71873=CARTESIAN_POINT('Ctrl Pts',(29.0494213811045,783.651046473984,110.827082017624));
#71874=CARTESIAN_POINT('Ctrl Pts',(28.9896823355468,783.660840914554,110.832115293449));
#71875=CARTESIAN_POINT('Ctrl Pts',(28.8721818261715,783.702224124192,110.848151793531));
#71876=CARTESIAN_POINT('Ctrl Pts',(28.8161719795131,783.735174074544,110.859463041959));
#71877=CARTESIAN_POINT('Ctrl Pts',(28.7205510696045,783.82032487939,110.886809468527));
#71878=CARTESIAN_POINT('Ctrl Pts',(28.681947966405,783.871751384858,110.902592576135));
#71879=CARTESIAN_POINT('Ctrl Pts',(28.6275938724069,783.98638894001,110.936708264004));
#71880=CARTESIAN_POINT('Ctrl Pts',(28.6124462165888,784.048514793948,110.954718856745));
#71881=CARTESIAN_POINT('Ctrl Pts',(28.6079643042431,784.175066905785,110.990715434349));
#71882=CARTESIAN_POINT('Ctrl Pts',(28.6186960189196,784.238278715916,111.008359168119));
#71883=CARTESIAN_POINT('Ctrl Pts',(28.6652534994828,784.358260734604,111.041294172221));
#71884=CARTESIAN_POINT('Ctrl Pts',(28.7010478762961,784.413712623193,111.056215116982));
#71885=CARTESIAN_POINT('Ctrl Pts',(28.792739146943,784.507606755541,111.080806383023));
#71886=CARTESIAN_POINT('Ctrl Pts',(28.8475916214523,784.545236136081,111.090267084053));
#71887=CARTESIAN_POINT('Ctrl Pts',(28.969089050239,784.597718776362,111.102322899475));
#71888=CARTESIAN_POINT('Ctrl Pts',(29.034495610272,784.612106187238,111.104810471845));
#71889=CARTESIAN_POINT('Ctrl Pts',(29.1672292978429,784.61557840484,111.102229458831));
#71890=CARTESIAN_POINT('Ctrl Pts',(29.2332258694233,784.604600092217,111.09717403284));
#71891=CARTESIAN_POINT('Ctrl Pts',(29.3567084403629,784.558499090403,111.0800019596));
#71892=CARTESIAN_POINT('Ctrl Pts',(29.412945752427,784.523824651056,111.068052336922));
#71893=CARTESIAN_POINT('Ctrl Pts',(29.5077136648204,784.435364605945,111.038885690367));
#71894=CARTESIAN_POINT('Ctrl Pts',(29.5453165048092,784.382491446767,111.021970912703));
#71895=CARTESIAN_POINT('Ctrl Pts',(29.5966542486413,784.265553629841,110.985598212997));
#71896=CARTESIAN_POINT('Ctrl Pts',(29.6098782986424,784.202659042162,110.966508949068));
#71897=CARTESIAN_POINT('Ctrl Pts',(29.6099522833995,784.075011066491,110.928847950516));
#71898=CARTESIAN_POINT('Ctrl Pts',(29.5966825891023,784.011526446793,110.91065924973));
#71899=CARTESIAN_POINT('Ctrl Pts',(29.5455296138344,783.893837807457,110.878130449407));
#71900=CARTESIAN_POINT('Ctrl Pts',(29.5085107025099,783.840634192522,110.864048011921));
#71901=CARTESIAN_POINT('Ctrl Pts',(29.4155234533503,783.750778963925,110.841586980028));
#71902=CARTESIAN_POINT('Ctrl Pts',(29.3604736528929,783.714946347179,110.833407470084));
#71903=CARTESIAN_POINT('Ctrl Pts',(29.2395914942158,783.665615214772,110.8239378139));
#71904=CARTESIAN_POINT('Ctrl Pts',(29.1749437335729,783.652517864365,110.822712634632));
#71905=CARTESIAN_POINT('Ctrl Pts',(29.1096415055408,783.651752382614,110.824985779127));
#71906=CARTESIAN_POINT('Origin',(32.4288564564431,781.96190260128,98.6833142766745));
#71907=CARTESIAN_POINT('',(32.4288564564431,777.234399375335,109.214127146458));
#71908=CARTESIAN_POINT('',(32.4288564564448,779.121595087564,109.564743167926));
#71909=CARTESIAN_POINT('Ctrl Pts',(32.4288564564431,777.234399375335,109.214127146458));
#71910=CARTESIAN_POINT('Ctrl Pts',(32.3101547171348,777.231595722789,109.222059755793));
#71911=CARTESIAN_POINT('Ctrl Pts',(32.1923352143316,777.251103332821,109.233757555294));
#71912=CARTESIAN_POINT('Ctrl Pts',(31.9671822172065,777.334478737508,109.263847146364));
#71913=CARTESIAN_POINT('Ctrl Pts',(31.8627895610585,777.398855105508,109.282112857103));
#71914=CARTESIAN_POINT('Ctrl Pts',(31.6837661754366,777.565695961093,109.323075248878));
#71915=CARTESIAN_POINT('Ctrl Pts',(31.6116352422431,777.667034631619,109.345412732826));
#71916=CARTESIAN_POINT('Ctrl Pts',(31.5103077358069,777.89417146595,109.39175065861));
#71917=CARTESIAN_POINT('Ctrl Pts',(31.4830297368684,778.018152703095,109.415323694428));
#71918=CARTESIAN_POINT('Ctrl Pts',(31.4787580499234,778.271183927327,109.46079925837));
#71919=CARTESIAN_POINT('Ctrl Pts',(31.5023951125465,778.397931822898,109.4822676082));
#71920=CARTESIAN_POINT('Ctrl Pts',(31.5975982095106,778.633539800542,109.519820243943));
#71921=CARTESIAN_POINT('Ctrl Pts',(31.6676565991942,778.740519737735,109.535640456385));
#71922=CARTESIAN_POINT('Ctrl Pts',(31.8445008416407,778.920733700444,109.55940470734));
#71923=CARTESIAN_POINT('Ctrl Pts',(31.949202460396,778.992660241787,109.567207699515));
#71924=CARTESIAN_POINT('Ctrl Pts',(32.1799990128611,779.09228918265,109.573273818901));
#71925=CARTESIAN_POINT('Ctrl Pts',(32.3036731310029,779.11920400299,109.57150846409));
#71926=CARTESIAN_POINT('Ctrl Pts',(32.4288564564465,779.121595087564,109.564743167926));
#71927=CARTESIAN_POINT('',(32.4288565295822,779.758468006617,107.762785193163));
#71928=CARTESIAN_POINT('',(32.4288564564431,782.855798773899,98.9992474298111));
#71929=CARTESIAN_POINT('Ctrl Pts',(32.4289098699438,777.886461794448,107.369192249501));
#71930=CARTESIAN_POINT('Ctrl Pts',(32.3637578802491,777.885807238946,107.371033223316));
#71931=CARTESIAN_POINT('Ctrl Pts',(32.2987643707776,777.891796036555,107.374231026386));
#71932=CARTESIAN_POINT('Ctrl Pts',(32.2096473094209,777.909320985861,107.38052044553));
#71933=CARTESIAN_POINT('Ctrl Pts',(32.1845614936939,777.915323247997,107.382509568572));
#71934=CARTESIAN_POINT('Ctrl Pts',(32.1431917498704,777.927021424797,107.386158045918));
#71935=CARTESIAN_POINT('Ctrl Pts',(32.1267554856739,777.932156741984,107.387707344574));
#71936=CARTESIAN_POINT('Ctrl Pts',(32.10308670609,777.940266420243,107.390084632186));
#71937=CARTESIAN_POINT('Ctrl Pts',(32.0957308859324,777.942888993599,107.390844370931));
#71938=CARTESIAN_POINT('Ctrl Pts',(32.0711923148809,777.9519818915,107.393449256827));
#71939=CARTESIAN_POINT('Ctrl Pts',(32.0541734470669,777.958858947601,107.395372687863));
#71940=CARTESIAN_POINT('Ctrl Pts',(32.0091600065378,777.978594060938,107.400776631465));
#71941=CARTESIAN_POINT('Ctrl Pts',(31.981595864868,777.992327796017,107.404423470151));
#71942=CARTESIAN_POINT('Ctrl Pts',(31.86030555755,778.060382594237,107.422034338184));
#71943=CARTESIAN_POINT('Ctrl Pts',(31.7760833968559,778.129138626915,107.438671915095));
#71944=CARTESIAN_POINT('Ctrl Pts',(31.6416384373393,778.284589931715,107.4746810714));
#71945=CARTESIAN_POINT('Ctrl Pts',(31.5898952076319,778.368154494824,107.493450566722));
#71946=CARTESIAN_POINT('Ctrl Pts',(31.5106696841909,778.557436045641,107.534958402962));
#71947=CARTESIAN_POINT('Ctrl Pts',(31.4868742502069,778.663182510197,107.557607942895));
#71948=CARTESIAN_POINT('Ctrl Pts',(31.4763124924462,778.886848161771,107.604564602141));
#71949=CARTESIAN_POINT('Ctrl Pts',(31.4928190226874,779.003232442255,107.628475197057));
#71950=CARTESIAN_POINT('Ctrl Pts',(31.5709857690768,779.232823306635,107.674597836214));
#71951=CARTESIAN_POINT('Ctrl Pts',(31.6352662925648,779.342931522523,107.696103966605));
#71952=CARTESIAN_POINT('Ctrl Pts',(31.8012862656198,779.52906909741,107.731049352303));
#71953=CARTESIAN_POINT('Ctrl Pts',(31.9002217088409,779.604351269389,107.744396594242));
#71954=CARTESIAN_POINT('Ctrl Pts',(32.1059129820279,779.705790038944,107.760427952354));
#71955=CARTESIAN_POINT('Ctrl Pts',(32.2080259836926,779.736725755301,107.764252910837));
#71956=CARTESIAN_POINT('Ctrl Pts',(32.4011468680326,779.761890836999,107.76429668748));
#71957=CARTESIAN_POINT('Ctrl Pts',(32.4902427056032,779.76115907177,107.761655079529));
#71958=CARTESIAN_POINT('Ctrl Pts',(32.6084649806787,779.743707004276,107.754577618871));
#71959=CARTESIAN_POINT('Ctrl Pts',(32.6388199915054,779.737709479938,107.752431875471));
#71960=CARTESIAN_POINT('Ctrl Pts',(32.6873290199313,779.725651121272,107.748466994289));
#71961=CARTESIAN_POINT('Ctrl Pts',(32.7056979419549,779.720494503792,107.746837721623));
#71962=CARTESIAN_POINT('Ctrl Pts',(32.7319460767755,779.712267143011,107.744323672343));
#71963=CARTESIAN_POINT('Ctrl Pts',(32.7399662388543,779.709635392808,107.743529986877));
#71964=CARTESIAN_POINT('Ctrl Pts',(32.7654359451088,779.700899982102,107.740927736297));
#71965=CARTESIAN_POINT('Ctrl Pts',(32.7827348481111,779.694396008882,107.739036758963));
#71966=CARTESIAN_POINT('Ctrl Pts',(32.8260733986865,779.676638522689,107.733983026282));
#71967=CARTESIAN_POINT('Ctrl Pts',(32.8518025663583,779.664717926169,107.730684761982));
#71968=CARTESIAN_POINT('Ctrl Pts',(32.9477030907431,779.614924131929,107.717234300634));
#71969=CARTESIAN_POINT('Ctrl Pts',(33.0133099159968,779.569450251953,107.705571309765));
#71970=CARTESIAN_POINT('Ctrl Pts',(33.1422003111067,779.453288462453,107.676912148343));
#71971=CARTESIAN_POINT('Ctrl Pts',(33.2019567319261,779.380150398644,107.659494344002));
#71972=CARTESIAN_POINT('Ctrl Pts',(33.3028562573453,779.209095036935,107.619979831064));
#71973=CARTESIAN_POINT('Ctrl Pts',(33.3401851525365,779.110475622494,107.597855895354));
#71974=CARTESIAN_POINT('Ctrl Pts',(33.3817915100074,778.895969171291,107.551083864768));
#71975=CARTESIAN_POINT('Ctrl Pts',(33.3825159827171,778.781052794483,107.52676400737));
#71976=CARTESIAN_POINT('Ctrl Pts',(33.340615761912,778.54767794391,107.478903837609));
#71977=CARTESIAN_POINT('Ctrl Pts',(33.2950359339541,778.431735421668,107.455999781223));
#71978=CARTESIAN_POINT('Ctrl Pts',(33.1602200989399,778.221636436189,107.416268778882));
#71979=CARTESIAN_POINT('Ctrl Pts',(33.0715905275148,778.129835781634,107.399915221269));
#71980=CARTESIAN_POINT('Ctrl Pts',(32.9032068320337,778.01331196114,107.380924465116));
#71981=CARTESIAN_POINT('Ctrl Pts',(32.8338108035281,777.976810683779,107.375501208513));
#71982=CARTESIAN_POINT('Ctrl Pts',(32.6546820911718,777.908854946885,107.366936997579));
#71983=CARTESIAN_POINT('Ctrl Pts',(32.5423259508394,777.887601239614,107.365987496492));
#71984=CARTESIAN_POINT('Ctrl Pts',(32.4289098699438,777.886461794448,107.369192249501));
#71985=CARTESIAN_POINT('Ctrl Pts',(32.4288564564465,779.121595087564,109.564743167926));
#71986=CARTESIAN_POINT('Ctrl Pts',(32.4290525561669,779.121598833199,109.564732570088));
#71987=CARTESIAN_POINT('Ctrl Pts',(32.4292486595918,779.121602518635,109.564721959994));
#71988=CARTESIAN_POINT('Ctrl Pts',(32.4294447666942,779.121606143867,109.564711337644));
#71989=CARTESIAN_POINT('Ctrl Pts',(32.5479650636094,779.123797107451,109.558291559722));
#71990=CARTESIAN_POINT('Ctrl Pts',(32.6655284664017,779.103957979382,109.547505888086));
#71991=CARTESIAN_POINT('Ctrl Pts',(32.8917401323626,779.020196791546,109.517398336627));
#71992=CARTESIAN_POINT('Ctrl Pts',(32.9973173386712,778.955090411697,109.498006966697));
#71993=CARTESIAN_POINT('Ctrl Pts',(33.1770386812934,778.787130123766,109.453481937324));
#71994=CARTESIAN_POINT('Ctrl Pts',(33.2489783367674,778.685696229256,109.428775728013));
#71995=CARTESIAN_POINT('Ctrl Pts',(33.3485088707922,778.460233422003,109.37799569508));
#71996=CARTESIAN_POINT('Ctrl Pts',(33.3749556280529,778.338418135868,109.352445590819));
#71997=CARTESIAN_POINT('Ctrl Pts',(33.3787327982746,778.089527534902,109.304228213008));
#71998=CARTESIAN_POINT('Ctrl Pts',(33.355459123767,777.964788289699,109.282066930245));
#71999=CARTESIAN_POINT('Ctrl Pts',(33.2610753639977,777.728947207022,109.244377166675));
#72000=CARTESIAN_POINT('Ctrl Pts',(33.1901692203057,777.620221547493,109.22928976029));
#72001=CARTESIAN_POINT('Ctrl Pts',(33.0127108190374,777.438787898314,109.208807515502));
#72002=CARTESIAN_POINT('Ctrl Pts',(32.9088501529068,777.36666055042,109.203300264579));
#72003=CARTESIAN_POINT('Ctrl Pts',(32.6815189326721,777.266530500913,109.20174319306));
#72004=CARTESIAN_POINT('Ctrl Pts',(32.5605210423891,777.238705364035,109.205534243894));
#72005=CARTESIAN_POINT('Ctrl Pts',(32.4348005148754,777.234553739407,109.213732320876));
#72006=CARTESIAN_POINT('Ctrl Pts',(32.4318282089087,777.234469566062,109.213928549946));
#72007=CARTESIAN_POINT('Ctrl Pts',(32.4288564564431,777.234399375335,109.214127146458));
#72008=CARTESIAN_POINT('Origin',(32.4288564564431,781.96190260128,98.6833142766745));
#72009=CARTESIAN_POINT('',(32.4288564564431,780.298485969774,104.890209520163));
#72010=CARTESIAN_POINT('Origin',(32.4288564564431,779.827063739165,104.723592952896));
#72011=CARTESIAN_POINT('',(32.4288564564431,778.677869419194,109.475555874173));
#72012=CARTESIAN_POINT('',(32.4288564564431,782.433324831889,98.8499308439416));
#72013=CARTESIAN_POINT('Ctrl Pts',(32.4290799508113,777.68259233814,109.290674899213));
#72014=CARTESIAN_POINT('Ctrl Pts',(32.3665334453012,777.681150919677,109.294669327409));
#72015=CARTESIAN_POINT('Ctrl Pts',(32.3044660597605,777.691430237481,109.300719408193));
#72016=CARTESIAN_POINT('Ctrl Pts',(32.1857666667416,777.735267561329,109.316547451625));
#72017=CARTESIAN_POINT('Ctrl Pts',(32.1306658993913,777.769142775006,109.326276325882));
#72018=CARTESIAN_POINT('Ctrl Pts',(32.0362583975027,777.856852174475,109.348218096714));
#72019=CARTESIAN_POINT('Ctrl Pts',(31.9982204294419,777.910059217511,109.36023628958));
#72020=CARTESIAN_POINT('Ctrl Pts',(31.9446687192663,778.029416818984,109.385193211902));
#72021=CARTESIAN_POINT('Ctrl Pts',(31.9301864927072,778.094613600829,109.397897869096));
#72022=CARTESIAN_POINT('Ctrl Pts',(31.9276892751721,778.227633723303,109.422265697251));
#72023=CARTESIAN_POINT('Ctrl Pts',(31.9399520972781,778.294234746654,109.433692986043));
#72024=CARTESIAN_POINT('Ctrl Pts',(31.989751865069,778.418596819799,109.453558877717));
#72025=CARTESIAN_POINT('Ctrl Pts',(32.0266601281827,778.475303485784,109.461840561142));
#72026=CARTESIAN_POINT('Ctrl Pts',(32.1201560115448,778.571116454262,109.47407505859));
#72027=CARTESIAN_POINT('Ctrl Pts',(32.1757253581395,778.609454002537,109.477942531954));
#72028=CARTESIAN_POINT('Ctrl Pts',(32.2970438717336,778.661951914601,109.48053467932));
#72029=CARTESIAN_POINT('Ctrl Pts',(32.361330718645,778.676188264655,109.479357549754));
#72030=CARTESIAN_POINT('Ctrl Pts',(32.4910841361272,778.679429649575,109.47205459791));
#72031=CARTESIAN_POINT('Ctrl Pts',(32.5552229102832,778.668592088853,109.466037804857));
#72032=CARTESIAN_POINT('Ctrl Pts',(32.675480520112,778.623066822056,109.449821046499));
#72033=CARTESIAN_POINT('Ctrl Pts',(32.7303336121286,778.588809263881,109.439782109346));
#72034=CARTESIAN_POINT('Ctrl Pts',(32.8246423274275,778.500017133566,109.416725069329));
#72035=CARTESIAN_POINT('Ctrl Pts',(32.8626062374142,778.44589451156,109.403881793554));
#72036=CARTESIAN_POINT('Ctrl Pts',(32.9147824306265,778.325695477516,109.37749955097));
#72037=CARTESIAN_POINT('Ctrl Pts',(32.9283833135647,778.260800967028,109.364230327539));
#72038=CARTESIAN_POINT('Ctrl Pts',(32.9293087524434,778.128738424644,109.339161010214));
#72039=CARTESIAN_POINT('Ctrl Pts',(32.9164313804879,778.062808208154,109.327612231577));
#72040=CARTESIAN_POINT('Ctrl Pts',(32.8655150618067,777.938880686931,109.307896134678));
#72041=CARTESIAN_POINT('Ctrl Pts',(32.8277569141518,777.88207133417,109.299933066946));
#72042=CARTESIAN_POINT('Ctrl Pts',(32.7335263655159,777.787373325686,109.288925300188));
#72043=CARTESIAN_POINT('Ctrl Pts',(32.6784224760383,777.749847132771,109.285847176004));
#72044=CARTESIAN_POINT('Ctrl Pts',(32.5579665365653,777.698144462057,109.284687314585));
#72045=CARTESIAN_POINT('Ctrl Pts',(32.493923646632,777.684086696613,109.28653376479));
#72046=CARTESIAN_POINT('Ctrl Pts',(32.4290799508113,777.68259233814,109.290674899213));
#72047=CARTESIAN_POINT('Origin',(20.4645692803024,793.317622820883,102.696810032682));
#72048=CARTESIAN_POINT('',(20.4645692803024,788.717535272518,112.647077402928));
#72049=CARTESIAN_POINT('',(20.4645692803045,790.678180117724,113.229952900161));
#72050=CARTESIAN_POINT('Ctrl Pts',(20.4645692803024,788.717535272518,112.647077402928));
#72051=CARTESIAN_POINT('Ctrl Pts',(20.3325219374791,788.715078477829,112.654028618235));
#72052=CARTESIAN_POINT('Ctrl Pts',(20.2016382854414,788.737261681635,112.668105133025));
#72053=CARTESIAN_POINT('Ctrl Pts',(19.955921009562,788.829133186696,112.708574079991));
#72054=CARTESIAN_POINT('Ctrl Pts',(19.843625220678,788.898242966989,112.73464303333));
#72055=CARTESIAN_POINT('Ctrl Pts',(19.653225199422,789.075233118174,112.795368281891));
#72056=CARTESIAN_POINT('Ctrl Pts',(19.5771916689324,789.181517184176,112.829456845998));
#72057=CARTESIAN_POINT('Ctrl Pts',(19.472166143186,789.417613506439,112.901588035092));
#72058=CARTESIAN_POINT('Ctrl Pts',(19.4444624805739,789.545202241544,112.938946875231));
#72059=CARTESIAN_POINT('Ctrl Pts',(19.4419466144868,789.804194947771,113.012522195203));
#72060=CARTESIAN_POINT('Ctrl Pts',(19.4672608066609,789.933106481549,113.048043093946));
#72061=CARTESIAN_POINT('Ctrl Pts',(19.5684801551307,790.175513753612,113.113318570561));
#72062=CARTESIAN_POINT('Ctrl Pts',(19.6438367318199,790.286513714994,113.142399952549));
#72063=CARTESIAN_POINT('Ctrl Pts',(19.8344868411345,790.473611921838,113.18989579132));
#72064=CARTESIAN_POINT('Ctrl Pts',(19.9477602472955,790.548015311287,113.207886612269));
#72065=CARTESIAN_POINT('Ctrl Pts',(20.1965535380417,790.649888329027,113.229885608953));
#72066=CARTESIAN_POINT('Ctrl Pts',(20.329457736696,790.676715811939,113.233770000985));
#72067=CARTESIAN_POINT('Ctrl Pts',(20.4637455691717,790.678171506983,113.229976266535));
#72068=CARTESIAN_POINT('Ctrl Pts',(20.4640201446788,790.678174483412,113.229968509566));
#72069=CARTESIAN_POINT('Ctrl Pts',(20.4642947150789,790.678177353655,113.229960720774));
#72070=CARTESIAN_POINT('Ctrl Pts',(20.4645692803066,790.678180117724,113.229952900161));
#72071=CARTESIAN_POINT('',(20.4645692794436,791.316321136848,111.424406983493));
#72072=CARTESIAN_POINT('',(20.4645692803024,794.280651961126,103.037177115749));
#72073=CARTESIAN_POINT('Ctrl Pts',(19.8034793393769,789.575990153271,110.94679009387));
#72074=CARTESIAN_POINT('Ctrl Pts',(19.7019570676491,789.657262245375,110.97551440113));
#72075=CARTESIAN_POINT('Ctrl Pts',(19.6182946642219,789.757180409438,111.008511950969));
#72076=CARTESIAN_POINT('Ctrl Pts',(19.4960576281591,789.982964085745,111.079459916268));
#72077=CARTESIAN_POINT('Ctrl Pts',(19.4586768930075,790.106625866136,111.116723594058));
#72078=CARTESIAN_POINT('Ctrl Pts',(19.4353986127253,790.361967455207,111.191117472984));
#72079=CARTESIAN_POINT('Ctrl Pts',(19.4499511871445,790.491225300991,111.227539736259));
#72080=CARTESIAN_POINT('Ctrl Pts',(19.5298918348331,790.738128191629,111.295038853781));
#72081=CARTESIAN_POINT('Ctrl Pts',(19.594740179245,790.853367006595,111.325455221171));
#72082=CARTESIAN_POINT('Ctrl Pts',(19.7666919636577,791.053765611051,111.376187043996));
#72083=CARTESIAN_POINT('Ctrl Pts',(19.8721962464135,791.13697621735,111.39600731711));
#72084=CARTESIAN_POINT('Ctrl Pts',(20.109020464352,791.259173362915,111.42198658606));
#72085=CARTESIAN_POINT('Ctrl Pts',(20.2378323791516,791.297408288582,111.428019856243));
#72086=CARTESIAN_POINT('Ctrl Pts',(20.5046047909829,791.324600450561,111.425226084446));
#72087=CARTESIAN_POINT('Ctrl Pts',(20.6400225102791,791.312656919593,111.416227096002));
#72088=CARTESIAN_POINT('Ctrl Pts',(20.8977666698177,791.238874182027,111.383658883735));
#72089=CARTESIAN_POINT('Ctrl Pts',(21.0175013272838,791.177693561985,111.36038410836));
#72090=CARTESIAN_POINT('Ctrl Pts',(21.2235374007743,791.014756398011,111.302700430138));
#72091=CARTESIAN_POINT('Ctrl Pts',(21.3081427937904,790.915002100251,111.268968630032));
#72092=CARTESIAN_POINT('Ctrl Pts',(21.4318962781407,790.689528973368,111.195459831531));
#72093=CARTESIAN_POINT('Ctrl Pts',(21.4698711405743,790.566028769384,111.156411579716));
#72094=CARTESIAN_POINT('Ctrl Pts',(21.493803531542,790.311774723019,111.078625656527));
#72095=CARTESIAN_POINT('Ctrl Pts',(21.4797057516203,790.183497254593,111.040646690727));
#72096=CARTESIAN_POINT('Ctrl Pts',(21.4008074653581,789.937495165339,110.97070432197));
#72097=CARTESIAN_POINT('Ctrl Pts',(21.3363466690085,789.822250663681,110.93947794166));
#72098=CARTESIAN_POINT('Ctrl Pts',(21.1641762306254,789.620197757338,110.888197260474));
#72099=CARTESIAN_POINT('Ctrl Pts',(21.0576463410307,789.535718445791,110.868780965762));
#72100=CARTESIAN_POINT('Ctrl Pts',(20.8184824018924,789.411663968598,110.844947561625));
#72101=CARTESIAN_POINT('Ctrl Pts',(20.688426054859,789.372795585845,110.840590505318));
#72102=CARTESIAN_POINT('Ctrl Pts',(20.4210873969079,789.345400767821,110.847052620977));
#72103=CARTESIAN_POINT('Ctrl Pts',(20.2864005190574,789.357080159282,110.857782569417));
#72104=CARTESIAN_POINT('Ctrl Pts',(20.093792436167,789.411996676071,110.884057017687));
#72105=CARTESIAN_POINT('Ctrl Pts',(20.0314202005905,789.43656544207,110.894506922721));
#72106=CARTESIAN_POINT('Ctrl Pts',(19.9121651831173,789.49768702915,110.918505283261));
#72107=CARTESIAN_POINT('Ctrl Pts',(19.8556631087487,789.53421523986,110.932025425981));
#72108=CARTESIAN_POINT('Ctrl Pts',(19.8034793393769,789.575990153271,110.94679009387));
#72109=CARTESIAN_POINT('Ctrl Pts',(20.4645692803066,790.678180117724,113.229952900161));
#72110=CARTESIAN_POINT('Ctrl Pts',(20.5946003758858,790.679489150697,113.22624914336));
#72111=CARTESIAN_POINT('Ctrl Pts',(20.7234710520815,790.656987854421,113.215398262081));
#72112=CARTESIAN_POINT('Ctrl Pts',(20.9698009034802,790.565163135047,113.179229742229));
#72113=CARTESIAN_POINT('Ctrl Pts',(21.0841491966429,790.494929565677,113.153699929834));
#72114=CARTESIAN_POINT('Ctrl Pts',(21.2769583706158,790.315968441955,113.091256578208));
#72115=CARTESIAN_POINT('Ctrl Pts',(21.3535542838551,790.209060509613,113.054978782971));
#72116=CARTESIAN_POINT('Ctrl Pts',(21.4581130112891,789.973151183668,112.977103531815));
#72117=CARTESIAN_POINT('Ctrl Pts',(21.4852877520556,789.846577752246,112.936315730743));
#72118=CARTESIAN_POINT('Ctrl Pts',(21.4866421167182,789.589763570253,112.856252698726));
#72119=CARTESIAN_POINT('Ctrl Pts',(21.4607577494378,789.462050385905,112.817787682342));
#72120=CARTESIAN_POINT('Ctrl Pts',(21.3583695124856,789.221166101082,112.748664112043));
#72121=CARTESIAN_POINT('Ctrl Pts',(21.2823071884363,789.110589209333,112.718802454285));
#72122=CARTESIAN_POINT('Ctrl Pts',(21.0915337930738,788.924847286338,112.672842408319));
#72123=CARTESIAN_POINT('Ctrl Pts',(20.9792448009946,788.850933017746,112.656971625891));
#72124=CARTESIAN_POINT('Ctrl Pts',(20.7325772743618,788.748297214449,112.640511611668));
#72125=CARTESIAN_POINT('Ctrl Pts',(20.6005809955413,788.720396088668,112.640014084162));
#72126=CARTESIAN_POINT('Ctrl Pts',(20.4663059453286,788.717568648235,112.64698629291));
#72127=CARTESIAN_POINT('Ctrl Pts',(20.4654375876425,788.717551427731,112.647031693631));
#72128=CARTESIAN_POINT('Ctrl Pts',(20.4645692803024,788.717535272518,112.647077402928));
#72129=CARTESIAN_POINT('Origin',(20.4645692803024,793.317622820883,102.696810032682));
#72130=CARTESIAN_POINT('',(20.4645692803024,791.654206189377,108.90370527617));
#72131=CARTESIAN_POINT('Origin',(20.4645692803024,791.182783958768,108.737088708903));
#72132=CARTESIAN_POINT('',(20.4645692803024,790.179862406587,113.075189817997));
#72133=CARTESIAN_POINT('',(20.4645692803024,793.789045051492,102.863426599949));
#72134=CARTESIAN_POINT('Ctrl Pts',(20.4639964622118,789.220082879986,112.789873469231));
#72135=CARTESIAN_POINT('Ctrl Pts',(20.4050339558016,789.219174851509,112.79264534018));
#72136=CARTESIAN_POINT('Ctrl Pts',(20.3465213477788,789.228291826247,112.798349454785));
#72137=CARTESIAN_POINT('Ctrl Pts',(20.2299791925496,789.267798967435,112.815878398925));
#72138=CARTESIAN_POINT('Ctrl Pts',(20.1737927019346,789.2999482079,112.828111760667));
#72139=CARTESIAN_POINT('Ctrl Pts',(20.0776751488463,789.383567300992,112.857245534214));
#72140=CARTESIAN_POINT('Ctrl Pts',(20.0387363811842,789.434255422457,112.873868829814));
#72141=CARTESIAN_POINT('Ctrl Pts',(19.9835030697374,789.547693532412,112.909441744593));
#72142=CARTESIAN_POINT('Ctrl Pts',(19.9678359233545,789.609367386774,112.928051657371));
#72143=CARTESIAN_POINT('Ctrl Pts',(19.9622134681862,789.735451156348,112.964932404433));
#72144=CARTESIAN_POINT('Ctrl Pts',(19.9723727478844,789.798644689578,112.982848956574));
#72145=CARTESIAN_POINT('Ctrl Pts',(20.0178714824198,789.919080901477,113.016025290741));
#72146=CARTESIAN_POINT('Ctrl Pts',(20.0532539728035,789.97498382296,113.03089898142));
#72147=CARTESIAN_POINT('Ctrl Pts',(20.1442906242766,790.069945619686,113.055092918069));
#72148=CARTESIAN_POINT('Ctrl Pts',(20.1988977292507,790.108193680832,113.06421575077));
#72149=CARTESIAN_POINT('Ctrl Pts',(20.3200200141217,790.161979710785,113.075418632704));
#72150=CARTESIAN_POINT('Ctrl Pts',(20.3852912578462,790.177072686822,113.077411380082));
#72151=CARTESIAN_POINT('Ctrl Pts',(20.5179768841985,790.182012331175,113.073774105504));
#72152=CARTESIAN_POINT('Ctrl Pts',(20.5840645289053,790.171777355984,113.068165953632));
#72153=CARTESIAN_POINT('Ctrl Pts',(20.7080517332299,790.127056361971,113.049829964805));
#72154=CARTESIAN_POINT('Ctrl Pts',(20.7646773179151,790.092962590222,113.037266694887));
#72155=CARTESIAN_POINT('Ctrl Pts',(20.8603329116298,790.005415513898,113.006807333327));
#72156=CARTESIAN_POINT('Ctrl Pts',(20.8984073744595,789.952857542019,112.989222595352));
#72157=CARTESIAN_POINT('Ctrl Pts',(20.9505461168486,789.836465323121,112.951552643713));
#72158=CARTESIAN_POINT('Ctrl Pts',(20.964152305626,789.773828708788,112.931856012379));
#72159=CARTESIAN_POINT('Ctrl Pts',(20.9649674299414,789.646774706997,112.893169870772));
#72160=CARTESIAN_POINT('Ctrl Pts',(20.9521660913145,789.583623642089,112.874570776244));
#72161=CARTESIAN_POINT('Ctrl Pts',(20.9015594798973,789.465059445714,112.841090127105));
#72162=CARTESIAN_POINT('Ctrl Pts',(20.8641227571364,789.410870859766,112.826565317502));
#72163=CARTESIAN_POINT('Ctrl Pts',(20.7703456159225,789.320112533352,112.803967063599));
#72164=CARTESIAN_POINT('Ctrl Pts',(20.7152216934108,789.28412977799,112.796004639445));
#72165=CARTESIAN_POINT('Ctrl Pts',(20.5941608260255,789.234412799054,112.787391251644));
#72166=CARTESIAN_POINT('Ctrl Pts',(20.5294013185598,789.221090121294,112.786798738656));
#72167=CARTESIAN_POINT('Ctrl Pts',(20.4639964622118,789.220082879986,112.789873469231));
#72168=CARTESIAN_POINT('Origin',(22.434557059716,787.005126867006,100.465760373941));
#72169=CARTESIAN_POINT('',(22.434557059716,782.282406564289,110.983040517812));
#72170=CARTESIAN_POINT('',(22.434557059716,784.159183512917,111.363135221129));
#72171=CARTESIAN_POINT('Ctrl Pts',(22.434557059716,782.282406564289,110.983040517812));
#72172=CARTESIAN_POINT('Ctrl Pts',(22.3145647956342,782.278220036892,110.994885810969));
#72173=CARTESIAN_POINT('Ctrl Pts',(22.1953761212331,782.296664917096,111.011054461859));
#72174=CARTESIAN_POINT('Ctrl Pts',(21.9699686706315,782.378103171931,111.050362783727));
#72175=CARTESIAN_POINT('Ctrl Pts',(21.8663333745128,782.440806687305,111.073167957544));
#72176=CARTESIAN_POINT('Ctrl Pts',(21.6888029197355,782.603965586086,111.122652988845));
#72177=CARTESIAN_POINT('Ctrl Pts',(21.6172849690108,782.703154860505,111.14884513235));
#72178=CARTESIAN_POINT('Ctrl Pts',(21.5165756055335,782.926141192785,111.201634645248));
#72179=CARTESIAN_POINT('Ctrl Pts',(21.489273406918,783.048043541804,111.227688637841));
#72180=CARTESIAN_POINT('Ctrl Pts',(21.4840352038534,783.298238922486,111.276558115142));
#72181=CARTESIAN_POINT('Ctrl Pts',(21.5070188487827,783.424204913184,111.298851887648));
#72182=CARTESIAN_POINT('Ctrl Pts',(21.6011223070221,783.660931494703,111.336591727571));
#72183=CARTESIAN_POINT('Ctrl Pts',(21.6715006688284,783.769520779225,111.351688252688));
#72184=CARTESIAN_POINT('Ctrl Pts',(21.8492291727829,783.952493435218,111.372363421747));
#72185=CARTESIAN_POINT('Ctrl Pts',(21.9544112999345,784.025697796313,111.377887946878));
#72186=CARTESIAN_POINT('Ctrl Pts',(22.1856973228963,784.127506336629,111.378346908484));
#72187=CARTESIAN_POINT('Ctrl Pts',(22.3093449109512,784.155565812865,111.37337108336));
#72188=CARTESIAN_POINT('Ctrl Pts',(22.434557059716,784.159183512917,111.363135221129));
#72189=CARTESIAN_POINT('',(22.4345565353571,784.811902018906,109.516343998021));
#72190=CARTESIAN_POINT('',(22.434557059716,787.899023039625,100.781693527078));
#72191=CARTESIAN_POINT('Ctrl Pts',(22.4341912064781,782.955910373024,109.077439905874));
#72192=CARTESIAN_POINT('Ctrl Pts',(22.3319455172926,782.953259645336,109.085058233456));
#72193=CARTESIAN_POINT('Ctrl Pts',(22.2302594739761,782.966838186319,109.096390842135));
#72194=CARTESIAN_POINT('Ctrl Pts',(22.0857147349296,783.010594491383,109.118060440226));
#72195=CARTESIAN_POINT('Ctrl Pts',(22.03964939657,783.028630720995,109.125897246329));
#72196=CARTESIAN_POINT('Ctrl Pts',(21.9638031770467,783.065544932245,109.140435804426));
#72197=CARTESIAN_POINT('Ctrl Pts',(21.9332233825504,783.082647231539,109.146800344347));
#72198=CARTESIAN_POINT('Ctrl Pts',(21.8745657646438,783.120006959674,109.160039888438));
#72199=CARTESIAN_POINT('Ctrl Pts',(21.8465144402259,783.140197898613,109.166897680218));
#72200=CARTESIAN_POINT('Ctrl Pts',(21.7829406417972,783.191690564646,109.183738895911));
#72201=CARTESIAN_POINT('Ctrl Pts',(21.748624641401,783.224249003488,109.193908821543));
#72202=CARTESIAN_POINT('Ctrl Pts',(21.6500854470938,783.333649529516,109.226727722468));
#72203=CARTESIAN_POINT('Ctrl Pts',(21.5961992886768,783.418421105743,109.250342260558));
#72204=CARTESIAN_POINT('Ctrl Pts',(21.5179717724287,783.603541053572,109.298860266041));
#72205=CARTESIAN_POINT('Ctrl Pts',(21.4946669617016,783.702832337023,109.323443667668));
#72206=CARTESIAN_POINT('Ctrl Pts',(21.481358554927,783.913726526315,109.373063675941));
#72207=CARTESIAN_POINT('Ctrl Pts',(21.4943742457734,784.024045980758,109.397591569015));
#72208=CARTESIAN_POINT('Ctrl Pts',(21.561203385517,784.243585087575,109.443685582558));
#72209=CARTESIAN_POINT('Ctrl Pts',(21.6173964599638,784.350248354268,109.46450956386));
#72210=CARTESIAN_POINT('Ctrl Pts',(21.770553698826,784.542666785869,109.498725550062));
#72211=CARTESIAN_POINT('Ctrl Pts',(21.8679207567976,784.625350123151,109.511387442897));
#72212=CARTESIAN_POINT('Ctrl Pts',(22.0861584324583,784.747450361711,109.525098704896));
#72213=CARTESIAN_POINT('Ctrl Pts',(22.2042453108566,784.786928099409,109.526342678263));
#72214=CARTESIAN_POINT('Ctrl Pts',(22.4498465842724,784.820054756526,109.517236101008));
#72215=CARTESIAN_POINT('Ctrl Pts',(22.5750169437994,784.812895137463,109.506847199228));
#72216=CARTESIAN_POINT('Ctrl Pts',(22.7483472112806,784.768498679961,109.484000899264));
#72217=CARTESIAN_POINT('Ctrl Pts',(22.8004886325275,784.750157708231,109.475905823453));
#72218=CARTESIAN_POINT('Ctrl Pts',(22.8838113679857,784.712317496645,109.46086572957));
#72219=CARTESIAN_POINT('Ctrl Pts',(22.9160638714698,784.695321524171,109.454464822773));
#72220=CARTESIAN_POINT('Ctrl Pts',(22.9611726951682,784.668041079933,109.4446457373));
#72221=CARTESIAN_POINT('Ctrl Pts',(22.9749311106217,784.659212428218,109.441525439157));
#72222=CARTESIAN_POINT('Ctrl Pts',(23.0186971033218,784.629453315632,109.431186098564));
#72223=CARTESIAN_POINT('Ctrl Pts',(23.0476449210594,784.60712631829,109.42369456889));
#72224=CARTESIAN_POINT('Ctrl Pts',(23.1167419282984,784.546887288026,109.404099395442));
#72225=CARTESIAN_POINT('Ctrl Pts',(23.1548544457957,784.506990149632,109.391645446958));
#72226=CARTESIAN_POINT('Ctrl Pts',(23.2609525475023,784.373336121114,109.351426617369));
#72227=CARTESIAN_POINT('Ctrl Pts',(23.3144028445643,784.27003570303,109.322325145207));
#72228=CARTESIAN_POINT('Ctrl Pts',(23.3759579552401,784.059388392483,109.266522815396));
#72229=CARTESIAN_POINT('Ctrl Pts',(23.3874433847075,783.954916956048,109.240273368974));
#72230=CARTESIAN_POINT('Ctrl Pts',(23.3736807622339,783.737700515715,109.188742314248));
#72231=CARTESIAN_POINT('Ctrl Pts',(23.3455640688954,783.626745545018,109.164131463533));
#72232=CARTESIAN_POINT('Ctrl Pts',(23.2468246171695,783.411393848005,109.120130746721));
#72233=CARTESIAN_POINT('Ctrl Pts',(23.1740611543256,783.31008566456,109.101678454116));
#72234=CARTESIAN_POINT('Ctrl Pts',(23.0069973980688,783.152118460831,109.077461305136));
#72235=CARTESIAN_POINT('Ctrl Pts',(22.9185796482836,783.092097603502,109.07037525928));
#72236=CARTESIAN_POINT('Ctrl Pts',(22.7668316838621,783.02154291635,109.065982529064));
#72237=CARTESIAN_POINT('Ctrl Pts',(22.7091762628634,783.000975149791,109.065805757572));
#72238=CARTESIAN_POINT('Ctrl Pts',(22.5793306231022,782.967876198178,109.068527071148));
#72239=CARTESIAN_POINT('Ctrl Pts',(22.5069179824542,782.957795820522,109.072021032885));
#72240=CARTESIAN_POINT('Ctrl Pts',(22.4341912064781,782.955910373024,109.077439905874));
#72241=CARTESIAN_POINT('Ctrl Pts',(22.434557059716,784.159183512916,111.363135221129));
#72242=CARTESIAN_POINT('Ctrl Pts',(22.4345899353016,784.159184462776,111.363132533611));
#72243=CARTESIAN_POINT('Ctrl Pts',(22.4346228109951,784.159185410951,111.363129845729));
#72244=CARTESIAN_POINT('Ctrl Pts',(22.4346556867964,784.15918635744,111.363127157485));
#72245=CARTESIAN_POINT('Ctrl Pts',(22.5528163031172,784.162588182837,111.35346520049));
#72246=CARTESIAN_POINT('Ctrl Pts',(22.6701261161492,784.144154849174,111.339290814618));
#72247=CARTESIAN_POINT('Ctrl Pts',(22.8972414404405,784.062970749404,111.30190779092));
#72248=CARTESIAN_POINT('Ctrl Pts',(23.0037970543271,783.998567263484,111.278611028557));
#72249=CARTESIAN_POINT('Ctrl Pts',(23.1840228811689,783.831951523415,111.2265530828));
#72250=CARTESIAN_POINT('Ctrl Pts',(23.2557926901844,783.73153169703,111.198354053641));
#72251=CARTESIAN_POINT('Ctrl Pts',(23.3548161962533,783.507967150304,111.141213130509));
#72252=CARTESIAN_POINT('Ctrl Pts',(23.3809709745847,783.387105574554,111.112876322306));
#72253=CARTESIAN_POINT('Ctrl Pts',(23.3841718939372,783.140133970266,111.060233344492));
#72254=CARTESIAN_POINT('Ctrl Pts',(23.360736107379,783.01643049486,111.036499466763));
#72255=CARTESIAN_POINT('Ctrl Pts',(23.2664302813607,782.782104439017,110.997192363948));
#72256=CARTESIAN_POINT('Ctrl Pts',(23.1957467150693,782.67389759727,110.982117502344));
#72257=CARTESIAN_POINT('Ctrl Pts',(23.018217947104,782.491565613827,110.963324471303));
#72258=CARTESIAN_POINT('Ctrl Pts',(22.9135927122306,782.418438310118,110.959561888858));
#72259=CARTESIAN_POINT('Ctrl Pts',(22.6847807346403,782.316346703612,110.963262832796));
#72260=CARTESIAN_POINT('Ctrl Pts',(22.5629895452002,782.287541742545,110.970489769422));
#72261=CARTESIAN_POINT('Ctrl Pts',(22.4378656680881,782.28252629713,110.982714739956));
#72262=CARTESIAN_POINT('Ctrl Pts',(22.4362112874469,782.282464280257,110.982877217181));
#72263=CARTESIAN_POINT('Ctrl Pts',(22.434557059716,782.282406564289,110.983040517812));
#72264=CARTESIAN_POINT('Origin',(22.434557059716,787.005126867006,100.465760373941));
#72265=CARTESIAN_POINT('',(22.434557059716,785.3417102355,106.672655617429));
#72266=CARTESIAN_POINT('Origin',(22.434557059716,784.870288004891,106.506039050162));
#72267=CARTESIAN_POINT('',(22.434557059716,783.717529955679,111.268085129529));
#72268=CARTESIAN_POINT('',(22.434557059716,787.476549097615,100.632376941208));
#72269=CARTESIAN_POINT('Ctrl Pts',(22.4343367025393,782.727746084943,111.067661749631));
#72270=CARTESIAN_POINT('Ctrl Pts',(22.3726006506608,782.725703330114,111.073523135672));
#72271=CARTESIAN_POINT('Ctrl Pts',(22.3112754249538,782.73500614065,111.081594388938));
#72272=CARTESIAN_POINT('Ctrl Pts',(22.1933973637207,782.77647171044,111.101696852075));
#72273=CARTESIAN_POINT('Ctrl Pts',(22.1383687395877,782.80910552941,111.113662513152));
#72274=CARTESIAN_POINT('Ctrl Pts',(22.0439914880774,782.894279111862,111.139852903109));
#72275=CARTESIAN_POINT('Ctrl Pts',(22.0058470515114,782.946124909647,111.15382062966));
#72276=CARTESIAN_POINT('Ctrl Pts',(21.9517697780768,783.062846215763,111.182106167447));
#72277=CARTESIAN_POINT('Ctrl Pts',(21.936799458975,783.126716842681,111.196133986485));
#72278=CARTESIAN_POINT('Ctrl Pts',(21.9327285656268,783.258661595137,111.222599196432));
#72279=CARTESIAN_POINT('Ctrl Pts',(21.9443532108643,783.325500261434,111.234727930421));
#72280=CARTESIAN_POINT('Ctrl Pts',(21.9931984200521,783.450943032292,111.255091508743));
#72281=CARTESIAN_POINT('Ctrl Pts',(22.0298801262911,783.508434903931,111.263156863517));
#72282=CARTESIAN_POINT('Ctrl Pts',(22.1230989462501,783.605896687254,111.274090436186));
#72283=CARTESIAN_POINT('Ctrl Pts',(22.1786153243142,783.645130577056,111.276903026751));
#72284=CARTESIAN_POINT('Ctrl Pts',(22.3010543292766,783.700005284196,111.276775953314));
#72285=CARTESIAN_POINT('Ctrl Pts',(22.3667029375574,783.715294105381,111.273878190394));
#72286=CARTESIAN_POINT('Ctrl Pts',(22.4978996032111,783.719620484652,111.26267793443));
#72287=CARTESIAN_POINT('Ctrl Pts',(22.5621006292266,783.70933723706,111.254636365592));
#72288=CARTESIAN_POINT('Ctrl Pts',(22.6821935273669,783.664944586968,111.234288495329));
#72289=CARTESIAN_POINT('Ctrl Pts',(22.7368752939048,783.631365466351,111.222203200013));
#72290=CARTESIAN_POINT('Ctrl Pts',(22.830343684457,783.544414068082,111.195303409615));
#72291=CARTESIAN_POINT('Ctrl Pts',(22.8678716260544,783.491661948801,111.180736044124));
#72292=CARTESIAN_POINT('Ctrl Pts',(22.9200963452349,783.373508134824,111.151123204493));
#72293=CARTESIAN_POINT('Ctrl Pts',(22.9338837698804,783.309167122121,111.13638881739));
#72294=CARTESIAN_POINT('Ctrl Pts',(22.9351871181484,783.177907773511,111.109036424678));
#72295=CARTESIAN_POINT('Ctrl Pts',(22.9224955483466,783.11226932585,111.096708180252));
#72296=CARTESIAN_POINT('Ctrl Pts',(22.8719994835884,782.988519520773,111.076266337587));
#72297=CARTESIAN_POINT('Ctrl Pts',(22.8344406021171,782.931627027859,111.068381887645));
#72298=CARTESIAN_POINT('Ctrl Pts',(22.7403204731203,782.835987918371,111.058395017031));
#72299=CARTESIAN_POINT('Ctrl Pts',(22.6849452223084,782.797760735205,111.056274121979));
#72300=CARTESIAN_POINT('Ctrl Pts',(22.5639127224996,782.744665805673,111.057868962667));
#72301=CARTESIAN_POINT('Ctrl Pts',(22.4995295038568,782.729903218508,111.061472170545));
#72302=CARTESIAN_POINT('Ctrl Pts',(22.4343367025393,782.727746084943,111.067661749631));
#72303=CARTESIAN_POINT('Origin',(13.2358290567306,800.458037260509,105.220474097608));
#72304=CARTESIAN_POINT('',(13.2358290567306,795.861581228149,115.160466514987));
#72305=CARTESIAN_POINT('',(13.2358290567306,797.815642116494,115.76197055367));
#72306=CARTESIAN_POINT('Ctrl Pts',(13.2358290567306,795.861581228149,115.160466514987));
#72307=CARTESIAN_POINT('Ctrl Pts',(13.1041212291136,795.858690928329,115.168644282725));
#72308=CARTESIAN_POINT('Ctrl Pts',(12.973562697341,795.880144614487,115.184392017813));
#72309=CARTESIAN_POINT('Ctrl Pts',(12.7282734162024,795.970123546666,115.228853097103));
#72310=CARTESIAN_POINT('Ctrl Pts',(12.616046168791,796.038139662565,115.257221950587));
#72311=CARTESIAN_POINT('Ctrl Pts',(12.4257398984536,796.212771683765,115.322601874734));
#72312=CARTESIAN_POINT('Ctrl Pts',(12.3496618273244,796.317767841094,115.358984279569));
#72313=CARTESIAN_POINT('Ctrl Pts',(12.2442054471236,796.551652098824,115.435220635439));
#72314=CARTESIAN_POINT('Ctrl Pts',(12.2161681956213,796.678332578655,115.474336159374));
#72315=CARTESIAN_POINT('Ctrl Pts',(12.2128246923721,796.93630278225,115.550549646238));
#72316=CARTESIAN_POINT('Ctrl Pts',(12.2377687821284,797.065077413602,115.586906141854));
#72317=CARTESIAN_POINT('Ctrl Pts',(12.3378734280937,797.30662427731,115.652500687538));
#72318=CARTESIAN_POINT('Ctrl Pts',(12.4120749207504,797.417086570966,115.681127350276));
#72319=CARTESIAN_POINT('Ctrl Pts',(12.6017910977174,797.606075689974,115.727617315544));
#72320=CARTESIAN_POINT('Ctrl Pts',(12.7160882481684,797.682172169096,115.744842792295));
#72321=CARTESIAN_POINT('Ctrl Pts',(12.9667210870214,797.786170619628,115.764616149613));
#72322=CARTESIAN_POINT('Ctrl Pts',(13.1002602974402,797.813718866267,115.767166354558));
#72323=CARTESIAN_POINT('Ctrl Pts',(13.235210494504,797.815633520053,115.761994314233));
#72324=CARTESIAN_POINT('Ctrl Pts',(13.2354166848091,797.815636445451,115.761986411876));
#72325=CARTESIAN_POINT('Ctrl Pts',(13.2356228722272,797.81563931093,115.761978491688));
#72326=CARTESIAN_POINT('Ctrl Pts',(13.2358290567306,797.815642116494,115.76197055367));
#72327=CARTESIAN_POINT('',(13.2358290558362,798.453583033059,113.956990803958));
#72328=CARTESIAN_POINT('',(13.2358290567306,801.421066400752,105.560841180675));
#72329=CARTESIAN_POINT('Ctrl Pts',(12.4273032040843,796.862039029937,113.521926296511));
#72330=CARTESIAN_POINT('Ctrl Pts',(12.3459211826545,796.961436378916,113.557056682833));
#72331=CARTESIAN_POINT('Ctrl Pts',(12.2859599712866,797.075587204588,113.59508453686));
#72332=CARTESIAN_POINT('Ctrl Pts',(12.215569609869,797.320459667716,113.672779125306));
#72333=CARTESIAN_POINT('Ctrl Pts',(12.20582869449,797.448791059769,113.711693201858));
#72334=CARTESIAN_POINT('Ctrl Pts',(12.2382675360023,797.703224865197,113.785766239328));
#72335=CARTESIAN_POINT('Ctrl Pts',(12.2803637546695,797.826868988588,113.820204423165));
#72336=CARTESIAN_POINT('Ctrl Pts',(12.4116340282938,798.052841521947,113.880306044229));
#72337=CARTESIAN_POINT('Ctrl Pts',(12.499762698849,798.152920781911,113.905364511945));
#72338=CARTESIAN_POINT('Ctrl Pts',(12.7107555953734,798.315370737971,113.942683998402));
#72339=CARTESIAN_POINT('Ctrl Pts',(12.8316392065375,798.376146995356,113.954575213524));
#72340=CARTESIAN_POINT('Ctrl Pts',(13.0890422797066,798.449367725707,113.963244560179));
#72341=CARTESIAN_POINT('Ctrl Pts',(13.2229524793323,798.46156769217,113.960076194865));
#72342=CARTESIAN_POINT('Ctrl Pts',(13.4890321484625,798.435955840218,113.938619697876));
#72343=CARTESIAN_POINT('Ctrl Pts',(13.618525917093,798.397760389817,113.920342392848));
#72344=CARTESIAN_POINT('Ctrl Pts',(13.8539178118326,798.275109375275,113.870502477999));
#72345=CARTESIAN_POINT('Ctrl Pts',(13.9574302937875,798.191805645498,113.839408647088));
#72346=CARTESIAN_POINT('Ctrl Pts',(14.1230271734505,797.992040790806,113.768708816872));
#72347=CARTESIAN_POINT('Ctrl Pts',(14.1838920191604,797.877870836644,113.729882036027));
#72348=CARTESIAN_POINT('Ctrl Pts',(14.2556491449628,797.633023205371,113.649525632122));
#72349=CARTESIAN_POINT('Ctrl Pts',(14.2658792373226,797.504746037582,113.608789039666));
#72350=CARTESIAN_POINT('Ctrl Pts',(14.2340583906279,797.251273713088,113.531279403436));
#72351=CARTESIAN_POINT('Ctrl Pts',(14.1924913567775,797.128512457711,113.495250053973));
#72352=CARTESIAN_POINT('Ctrl Pts',(14.0622479731902,796.903235669234,113.432632707769));
#72353=CARTESIAN_POINT('Ctrl Pts',(13.9744411469121,796.803080423965,113.406739381224));
#72354=CARTESIAN_POINT('Ctrl Pts',(13.7628720578125,796.639054932882,113.368898875281));
#72355=CARTESIAN_POINT('Ctrl Pts',(13.6407645383992,796.577232890325,113.357490426058));
#72356=CARTESIAN_POINT('Ctrl Pts',(13.3808574549199,796.502634827345,113.351136592103));
#72357=CARTESIAN_POINT('Ctrl Pts',(13.2457219745547,796.490046144811,113.35606767105));
#72358=CARTESIAN_POINT('Ctrl Pts',(12.9793028609075,796.515545091894,113.381224233002));
#72359=CARTESIAN_POINT('Ctrl Pts',(12.8505921104556,796.553326383922,113.401179476283));
#72360=CARTESIAN_POINT('Ctrl Pts',(12.6747785467436,796.644752360755,113.440357603061));
#72361=CARTESIAN_POINT('Ctrl Pts',(12.6193094711535,796.680998840812,113.454934807369));
#72362=CARTESIAN_POINT('Ctrl Pts',(12.516304707968,796.764145693389,113.486717641978));
#72363=CARTESIAN_POINT('Ctrl Pts',(12.4691346226,796.810947498522,113.503868820583));
#72364=CARTESIAN_POINT('Ctrl Pts',(12.4273032040843,796.862039029937,113.521926296511));
#72365=CARTESIAN_POINT('Ctrl Pts',(13.2358290567306,797.815642116494,115.76197055367));
#72366=CARTESIAN_POINT('Ctrl Pts',(13.3668381839024,797.817424765096,115.756926756439));
#72367=CARTESIAN_POINT('Ctrl Pts',(13.4966705402353,797.79501818008,115.744684286592));
#72368=CARTESIAN_POINT('Ctrl Pts',(13.7429834672164,797.703252865656,115.70589433082));
#72369=CARTESIAN_POINT('Ctrl Pts',(13.8565880736033,797.633581041091,115.679343320689));
#72370=CARTESIAN_POINT('Ctrl Pts',(14.0485151820788,797.455900294262,115.614936513227));
#72371=CARTESIAN_POINT('Ctrl Pts',(14.1248911380197,797.349587483375,115.577693034246));
#72372=CARTESIAN_POINT('Ctrl Pts',(14.2293664624442,797.11470288253,115.497676654686));
#72373=CARTESIAN_POINT('Ctrl Pts',(14.2565570706956,796.988489343664,115.455713402195));
#72374=CARTESIAN_POINT('Ctrl Pts',(14.2578921523234,796.73258620367,115.373250788514));
#72375=CARTESIAN_POINT('Ctrl Pts',(14.2320451601527,796.605413136226,115.333581681107));
#72376=CARTESIAN_POINT('Ctrl Pts',(14.1299427876524,796.365828693017,115.262335923215));
#72377=CARTESIAN_POINT('Ctrl Pts',(14.0542704661199,796.255947264145,115.23156063921));
#72378=CARTESIAN_POINT('Ctrl Pts',(13.8641237251078,796.070659717731,115.184267303577));
#72379=CARTESIAN_POINT('Ctrl Pts',(13.7519211761802,795.996662649226,115.16804993926));
#72380=CARTESIAN_POINT('Ctrl Pts',(13.5052398524324,795.893424010687,115.151906601647));
#72381=CARTESIAN_POINT('Ctrl Pts',(13.3731239816882,795.865071075193,115.152091801046));
#72382=CARTESIAN_POINT('Ctrl Pts',(13.2383415336434,795.861638576023,115.16031121011));
#72383=CARTESIAN_POINT('Ctrl Pts',(13.237085242904,795.861608794883,115.160388518114));
#72384=CARTESIAN_POINT('Ctrl Pts',(13.2358290567306,795.861581228149,115.160466514987));
#72385=CARTESIAN_POINT('Origin',(13.2358290567306,800.458037260509,105.220474097608));
#72386=CARTESIAN_POINT('',(13.2358290567306,798.794620629003,111.427369341096));
#72387=CARTESIAN_POINT('Origin',(13.2358290567306,798.323198398394,111.260752773829));
#72388=CARTESIAN_POINT('',(13.2358290567306,797.318300108841,115.604446831791));
#72389=CARTESIAN_POINT('',(13.2358290567306,800.929459491118,105.387090664875));
#72390=CARTESIAN_POINT('Ctrl Pts',(13.2354533120498,796.361757660371,115.309970985344));
#72391=CARTESIAN_POINT('Ctrl Pts',(13.1752379075312,796.360605246904,115.313367400001));
#72392=CARTESIAN_POINT('Ctrl Pts',(13.1154959366117,796.36985571648,115.319971852384));
#72393=CARTESIAN_POINT('Ctrl Pts',(12.9981428930495,796.409939133173,115.33961134581));
#72394=CARTESIAN_POINT('Ctrl Pts',(12.9422366428628,796.44208307235,115.352933503107));
#72395=CARTESIAN_POINT('Ctrl Pts',(12.8468224525815,796.525525714675,115.384236969571));
#72396=CARTESIAN_POINT('Ctrl Pts',(12.8082799589247,796.576029991166,115.401915191058));
#72397=CARTESIAN_POINT('Ctrl Pts',(12.7538475128707,796.689037826653,115.439382299639));
#72398=CARTESIAN_POINT('Ctrl Pts',(12.7385853584983,796.750464932062,115.458808831554));
#72399=CARTESIAN_POINT('Ctrl Pts',(12.7337447351938,796.87610395184,115.496952308307));
#72400=CARTESIAN_POINT('Ctrl Pts',(12.744301334523,796.93909251629,115.515296434828));
#72401=CARTESIAN_POINT('Ctrl Pts',(12.7901215243676,797.05798481727,115.54855854042));
#72402=CARTESIAN_POINT('Ctrl Pts',(12.8249689896076,797.112737150708,115.563156844004));
#72403=CARTESIAN_POINT('Ctrl Pts',(12.9153615496383,797.207392425631,115.586949603157));
#72404=CARTESIAN_POINT('Ctrl Pts',(12.9703955264301,797.2460467359,115.595799558701));
#72405=CARTESIAN_POINT('Ctrl Pts',(13.0922702046139,797.300271545736,115.606071285171));
#72406=CARTESIAN_POINT('Ctrl Pts',(13.1578123687506,797.315480168869,115.607445845313));
#72407=CARTESIAN_POINT('Ctrl Pts',(13.2906192914867,797.320495339603,115.602405918425));
#72408=CARTESIAN_POINT('Ctrl Pts',(13.356555221227,797.31035708358,115.596069310506));
#72409=CARTESIAN_POINT('Ctrl Pts',(13.4800532313852,797.266000197467,115.576293489835));
#72410=CARTESIAN_POINT('Ctrl Pts',(13.5363803104309,797.232231482656,115.563049591712));
#72411=CARTESIAN_POINT('Ctrl Pts',(13.6316289907162,797.145454251167,115.53126151422));
#72412=CARTESIAN_POINT('Ctrl Pts',(13.6695873623299,797.093309077365,115.513032813375));
#72413=CARTESIAN_POINT('Ctrl Pts',(13.7217020073133,796.977650458397,115.474076233999));
#72414=CARTESIAN_POINT('Ctrl Pts',(13.7353497047518,796.915302076225,115.453742496961));
#72415=CARTESIAN_POINT('Ctrl Pts',(13.7362840686973,796.788704020686,115.413854309931));
#72416=CARTESIAN_POINT('Ctrl Pts',(13.7235359348621,796.725719130352,115.394704459687));
#72417=CARTESIAN_POINT('Ctrl Pts',(13.6730191627257,796.607401935663,115.360333201665));
#72418=CARTESIAN_POINT('Ctrl Pts',(13.6356243685776,796.553297760889,115.345481743696));
#72419=CARTESIAN_POINT('Ctrl Pts',(13.5419009937708,796.462549287198,115.322568960372));
#72420=CARTESIAN_POINT('Ctrl Pts',(13.4867817211731,796.426508582014,115.314622935924));
#72421=CARTESIAN_POINT('Ctrl Pts',(13.3656941306241,796.376524780958,115.306448691272));
#72422=CARTESIAN_POINT('Ctrl Pts',(13.3008943237075,796.363010082466,115.306279823374));
#72423=CARTESIAN_POINT('Ctrl Pts',(13.2354533120498,796.361757660371,115.309970985344));
#72424=CARTESIAN_POINT('Origin',(13.7707655252052,793.897310963527,102.901691436531));
#72425=CARTESIAN_POINT('',(13.7707655252052,789.181066524569,113.400648875834));
#72426=CARTESIAN_POINT('',(13.7707655252132,791.043521315622,113.821266461007));
#72427=CARTESIAN_POINT('Ctrl Pts',(13.7707655252052,789.181066524569,113.400648875834));
#72428=CARTESIAN_POINT('Ctrl Pts',(13.6492784145032,789.175680293637,113.415888590839));
#72429=CARTESIAN_POINT('Ctrl Pts',(13.5285703655825,789.193261731801,113.436216379807));
#72430=CARTESIAN_POINT('Ctrl Pts',(13.3025153023418,789.273178909632,113.484449828108));
#72431=CARTESIAN_POINT('Ctrl Pts',(13.1993987229554,789.334524325493,113.511828328945));
#72432=CARTESIAN_POINT('Ctrl Pts',(13.0234167711003,789.494374366946,113.570254118077));
#72433=CARTESIAN_POINT('Ctrl Pts',(12.9526596650833,789.591384689429,113.600689697077));
#72434=CARTESIAN_POINT('Ctrl Pts',(12.8528934676997,789.810075625491,113.661124028342));
#72435=CARTESIAN_POINT('Ctrl Pts',(12.8257378275371,789.929805362413,113.690458608107));
#72436=CARTESIAN_POINT('Ctrl Pts',(12.8200631331498,790.176191048161,113.744419453954));
#72437=CARTESIAN_POINT('Ctrl Pts',(12.8424389481425,790.300465020687,113.768428489183));
#72438=CARTESIAN_POINT('Ctrl Pts',(12.9351494967828,790.536606222016,113.808198156768));
#72439=CARTESIAN_POINT('Ctrl Pts',(13.0054727532173,790.646007389772,113.82344242124));
#72440=CARTESIAN_POINT('Ctrl Pts',(13.1834024574027,790.830976922132,113.84264262536));
#72441=CARTESIAN_POINT('Ctrl Pts',(13.2889133176225,790.905326833515,113.846576875626));
#72442=CARTESIAN_POINT('Ctrl Pts',(13.5206220459066,791.009347472381,113.842562056751));
#72443=CARTESIAN_POINT('Ctrl Pts',(13.644390372637,791.038599593603,113.83479114981));
#72444=CARTESIAN_POINT('Ctrl Pts',(13.7697596530115,791.043482662353,113.821374226517));
#72445=CARTESIAN_POINT('Ctrl Pts',(13.7700949501014,791.043495722001,113.821338343282));
#72446=CARTESIAN_POINT('Ctrl Pts',(13.7704302408894,791.043508606022,113.821302421345));
#72447=CARTESIAN_POINT('Ctrl Pts',(13.7707655252212,791.043521315622,113.821266461007));
#72448=CARTESIAN_POINT('',(13.7707655251889,791.698900378754,111.966947500389));
#72449=CARTESIAN_POINT('',(13.7707655252052,794.791207136146,103.217624589667));
#72450=CARTESIAN_POINT('Ctrl Pts',(13.0869837155771,790.11503182315,111.63240064931));
#72451=CARTESIAN_POINT('Ctrl Pts',(13.0049672579053,790.195544742242,111.660856639139));
#72452=CARTESIAN_POINT('Ctrl Pts',(12.9397259231793,790.290827518569,111.6911850193));
#72453=CARTESIAN_POINT('Ctrl Pts',(12.8468751181743,790.506826171458,111.754248307119));
#72454=CARTESIAN_POINT('Ctrl Pts',(12.8225251034181,790.626429944291,111.786374964653));
#72455=CARTESIAN_POINT('Ctrl Pts',(12.8228358603533,790.867018868523,111.84620141651));
#72456=CARTESIAN_POINT('Ctrl Pts',(12.8466565698299,790.985687233574,111.87341329365));
#72457=CARTESIAN_POINT('Ctrl Pts',(12.9393638812806,791.210552717328,111.920654283523));
#72458=CARTESIAN_POINT('Ctrl Pts',(13.0081189415837,791.314463601038,111.94013481181));
#72459=CARTESIAN_POINT('Ctrl Pts',(13.1828765863515,791.492791454484,111.968569638707));
#72460=CARTESIAN_POINT('Ctrl Pts',(13.2877112181536,791.565178812335,111.977129194197));
#72461=CARTESIAN_POINT('Ctrl Pts',(13.5194529266911,791.666885982961,111.981620750733));
#72462=CARTESIAN_POINT('Ctrl Pts',(13.6441809396813,791.695125117343,111.977474984418));
#72463=CARTESIAN_POINT('Ctrl Pts',(13.8912599510332,791.702494156065,111.956926546054));
#72464=CARTESIAN_POINT('Ctrl Pts',(14.0111979117764,791.683573565169,111.941230694138));
#72465=CARTESIAN_POINT('Ctrl Pts',(14.2324367871271,791.603831820801,111.900581035401));
#72466=CARTESIAN_POINT('Ctrl Pts',(14.3322371818225,791.54513150621,111.876310508249));
#72467=CARTESIAN_POINT('Ctrl Pts',(14.5041670791584,791.394206690427,111.821363139156));
#72468=CARTESIAN_POINT('Ctrl Pts',(14.5745608791319,791.303183734224,111.791155249483));
#72469=CARTESIAN_POINT('Ctrl Pts',(14.6779001994751,791.09713949323,111.727783702372));
#72470=CARTESIAN_POINT('Ctrl Pts',(14.7088159254487,790.983527220993,111.695175601264));
#72471=CARTESIAN_POINT('Ctrl Pts',(14.72516982677,790.743922053886,111.631057305945));
#72472=CARTESIAN_POINT('Ctrl Pts',(14.7079659446061,790.620070837777,111.600365882178));
#72473=CARTESIAN_POINT('Ctrl Pts',(14.6257958682063,790.387589802217,111.547862325335));
#72474=CARTESIAN_POINT('Ctrl Pts',(14.5626944247314,790.280871314744,111.526365639337));
#72475=CARTESIAN_POINT('Ctrl Pts',(14.3977546066292,790.094402858652,111.494581682993));
#72476=CARTESIAN_POINT('Ctrl Pts',(14.2969248398132,790.016779155715,111.484749905825));
#72477=CARTESIAN_POINT('Ctrl Pts',(14.0703270086054,789.902563463259,111.478462642894));
#72478=CARTESIAN_POINT('Ctrl Pts',(13.9464808250464,789.867430435575,111.482184507875));
#72479=CARTESIAN_POINT('Ctrl Pts',(13.7064244472674,789.847328150563,111.501702484579));
#72480=CARTESIAN_POINT('Ctrl Pts',(13.5926681403926,789.857685050726,111.516042739114));
#72481=CARTESIAN_POINT('Ctrl Pts',(13.3699873528363,789.919062454618,111.554388960176));
#72482=CARTESIAN_POINT('Ctrl Pts',(13.2636782647354,789.971532393303,111.578482025435));
#72483=CARTESIAN_POINT('Ctrl Pts',(13.1413503420825,790.064891015258,111.614333873035));
#72484=CARTESIAN_POINT('Ctrl Pts',(13.113353216892,790.089145731674,111.623251628704));
#72485=CARTESIAN_POINT('Ctrl Pts',(13.0869837155771,790.11503182315,111.63240064931));
#72486=CARTESIAN_POINT('Ctrl Pts',(13.7707655252212,791.043521315622,113.821266461007));
#72487=CARTESIAN_POINT('Ctrl Pts',(13.8911012868655,791.04808287511,113.808360058089));
#72488=CARTESIAN_POINT('Ctrl Pts',(14.0106059580553,791.030100687515,113.790485308017));
#72489=CARTESIAN_POINT('Ctrl Pts',(14.2368210489679,790.949946485546,113.745783657447));
#72490=CARTESIAN_POINT('Ctrl Pts',(14.3410046451445,790.887881897924,113.719259733935));
#72491=CARTESIAN_POINT('Ctrl Pts',(14.5189034927078,790.726343959621,113.660593518157));
#72492=CARTESIAN_POINT('Ctrl Pts',(14.5904105476491,790.628171924739,113.629008416356));
#72493=CARTESIAN_POINT('Ctrl Pts',(14.6900521482705,790.408090704759,113.565126045315));
#72494=CARTESIAN_POINT('Ctrl Pts',(14.7167142995753,790.288290918272,113.533509985004));
#72495=CARTESIAN_POINT('Ctrl Pts',(14.7207463961015,790.043589576605,113.475233159204));
#72496=CARTESIAN_POINT('Ctrl Pts',(14.6979109393481,789.921159564621,113.449195572618));
#72497=CARTESIAN_POINT('Ctrl Pts',(14.6053240236367,789.689005947332,113.406546196425));
#72498=CARTESIAN_POINT('Ctrl Pts',(14.5359217725427,789.581678050486,113.390466256828));
#72499=CARTESIAN_POINT('Ctrl Pts',(14.3587046077869,789.39678406123,113.370879692966));
#72500=CARTESIAN_POINT('Ctrl Pts',(14.2519882513673,789.321358442444,113.367733513863));
#72501=CARTESIAN_POINT('Ctrl Pts',(14.0198183863037,789.216617046771,113.374961362592));
#72502=CARTESIAN_POINT('Ctrl Pts',(13.8970222289228,789.186910636597,113.384866626768));
#72503=CARTESIAN_POINT('Ctrl Pts',(13.7720311551946,789.181123259504,113.400490252153));
#72504=CARTESIAN_POINT('Ctrl Pts',(13.7713983296233,789.181094580473,113.400569494911));
#72505=CARTESIAN_POINT('Ctrl Pts',(13.7707655252052,789.181066524569,113.400648875834));
#72506=CARTESIAN_POINT('Origin',(13.7707655252052,793.897310963527,102.901691436531));
#72507=CARTESIAN_POINT('',(13.7707655252052,792.233894332021,109.108586680019));
#72508=CARTESIAN_POINT('Origin',(13.7707655252052,791.762472101412,108.941970112752));
#72509=CARTESIAN_POINT('',(13.7707655252051,790.604793599704,113.717938041125));
#72510=CARTESIAN_POINT('',(13.7707655252052,794.368733194136,103.068308003798));
#72511=CARTESIAN_POINT('Ctrl Pts',(13.7705656579046,789.622571644425,113.496119073646));
#72512=CARTESIAN_POINT('Ctrl Pts',(13.7079789944701,789.619914051806,113.503713500116));
#72513=CARTESIAN_POINT('Ctrl Pts',(13.6457874201933,789.628814405553,113.513869638531));
#72514=CARTESIAN_POINT('Ctrl Pts',(13.5274527452042,789.669636000176,113.538470417792));
#72515=CARTESIAN_POINT('Ctrl Pts',(13.4726695888231,789.701652930357,113.552754741715));
#72516=CARTESIAN_POINT('Ctrl Pts',(13.3790715125016,789.785315296323,113.583487719747));
#72517=CARTESIAN_POINT('Ctrl Pts',(13.3413318784207,789.836155196056,113.599616965602));
#72518=CARTESIAN_POINT('Ctrl Pts',(13.2878530989089,789.950824673352,113.631826576731));
#72519=CARTESIAN_POINT('Ctrl Pts',(13.2730365641952,790.013617018126,113.647559755922));
#72520=CARTESIAN_POINT('Ctrl Pts',(13.2689337098566,790.143331867244,113.676700604033));
#72521=CARTESIAN_POINT('Ctrl Pts',(13.2802379622306,790.208997031973,113.689759382511));
#72522=CARTESIAN_POINT('Ctrl Pts',(13.3281775282723,790.333634579579,113.711345037254));
#72523=CARTESIAN_POINT('Ctrl Pts',(13.3646690555538,790.391342894356,113.719614471265));
#72524=CARTESIAN_POINT('Ctrl Pts',(13.457598734647,790.489601360741,113.730056613978));
#72525=CARTESIAN_POINT('Ctrl Pts',(13.5130656544762,790.5293847229,113.732177343589));
#72526=CARTESIAN_POINT('Ctrl Pts',(13.6353884649001,790.585558085541,113.729928681215));
#72527=CARTESIAN_POINT('Ctrl Pts',(13.7010138313307,790.601612338272,113.725630069115));
#72528=CARTESIAN_POINT('Ctrl Pts',(13.8324207645165,790.607624549419,113.71114313671));
#72529=CARTESIAN_POINT('Ctrl Pts',(13.8968934152184,790.598176777658,113.70124278508));
#72530=CARTESIAN_POINT('Ctrl Pts',(14.0172914442885,790.555402151593,113.676949017842));
#72531=CARTESIAN_POINT('Ctrl Pts',(14.0720655339886,790.522704676629,113.662836096736));
#72532=CARTESIAN_POINT('Ctrl Pts',(14.1651508234348,790.437988080927,113.632043893543));
#72533=CARTESIAN_POINT('Ctrl Pts',(14.2024749867338,790.386827800339,113.615681598685));
#72534=CARTESIAN_POINT('Ctrl Pts',(14.2552963278157,790.271086038338,113.582449807667));
#72535=CARTESIAN_POINT('Ctrl Pts',(14.2695783894647,790.207416304052,113.565940175164));
#72536=CARTESIAN_POINT('Ctrl Pts',(14.2718152960103,790.077305573402,113.535577479682));
#72537=CARTESIAN_POINT('Ctrl Pts',(14.2596455275522,790.012186037977,113.522049402005));
#72538=CARTESIAN_POINT('Ctrl Pts',(14.210332779705,789.889083456448,113.499928736488));
#72539=CARTESIAN_POINT('Ctrl Pts',(14.1734685911125,789.832333077968,113.49158846207));
#72540=CARTESIAN_POINT('Ctrl Pts',(14.0796818308219,789.735083430543,113.48138693629));
#72541=CARTESIAN_POINT('Ctrl Pts',(14.0234642175206,789.695595617994,113.479667950468));
#72542=CARTESIAN_POINT('Ctrl Pts',(13.9010322090691,789.640799195777,113.48315987103));
#72543=CARTESIAN_POINT('Ctrl Pts',(13.836197853444,789.625358558263,113.488155094489));
#72544=CARTESIAN_POINT('Ctrl Pts',(13.7705656579046,789.622571644425,113.496119073646));
#72545=CARTESIAN_POINT('Origin',(7.73962524950056,808.859454792509,108.189819322485));
#72546=CARTESIAN_POINT('',(7.73962524950056,804.267101962135,118.118202206281));
#72547=CARTESIAN_POINT('',(7.73962524950039,806.213211761693,118.742202927456));
#72548=CARTESIAN_POINT('Ctrl Pts',(7.73962524950056,804.267101962135,118.118202206281));
#72549=CARTESIAN_POINT('Ctrl Pts',(7.73929993760265,804.267094191054,118.118224193655));
#72550=CARTESIAN_POINT('Ctrl Pts',(7.73897461814967,804.267086567046,118.118246231281));
#72551=CARTESIAN_POINT('Ctrl Pts',(7.60531324941621,804.264014660816,118.127321089998));
#72552=CARTESIAN_POINT('Ctrl Pts',(7.4732278130278,804.28571529985,118.144650731072));
#72553=CARTESIAN_POINT('Ctrl Pts',(7.22700336739817,804.376372539546,118.193171632574));
#72554=CARTESIAN_POINT('Ctrl Pts',(7.11513287093602,804.444293061202,118.223835269346));
#72555=CARTESIAN_POINT('Ctrl Pts',(6.92609483555976,804.618192584419,118.294059137281));
#72556=CARTESIAN_POINT('Ctrl Pts',(6.85077551572802,804.722462528698,118.332920483092));
#72557=CARTESIAN_POINT('Ctrl Pts',(6.74681866958897,804.954552184318,118.413770244575));
#72558=CARTESIAN_POINT('Ctrl Pts',(6.71943320781253,805.080146110677,118.45496182777));
#72559=CARTESIAN_POINT('Ctrl Pts',(6.71707351890575,805.336230349157,118.534550135433));
#72560=CARTESIAN_POINT('Ctrl Pts',(6.74240845697383,805.464196647438,118.572150775241));
#72561=CARTESIAN_POINT('Ctrl Pts',(6.84314685889307,805.704697604377,118.639200143135));
#72562=CARTESIAN_POINT('Ctrl Pts',(6.9176945787367,805.814870877432,118.667998289195));
#72563=CARTESIAN_POINT('Ctrl Pts',(7.10720753273267,806.002755049752,118.713620999227));
#72564=CARTESIAN_POINT('Ctrl Pts',(7.22068603978126,806.078348782568,118.729908655983));
#72565=CARTESIAN_POINT('Ctrl Pts',(7.47053559653812,806.18283418805,118.747546739802));
#72566=CARTESIAN_POINT('Ctrl Pts',(7.60437780516798,806.210886043958,118.748783275742));
#72567=CARTESIAN_POINT('Ctrl Pts',(7.73962524950022,806.213211761693,118.742202927456));
#72568=CARTESIAN_POINT('',(7.73962524873305,806.8511543926,116.937218327214));
#72569=CARTESIAN_POINT('',(7.73962524950056,809.822483932751,108.530186405553));
#72570=CARTESIAN_POINT('Ctrl Pts',(6.81899994463158,805.434810160941,116.55183368117));
#72571=CARTESIAN_POINT('Ctrl Pts',(6.76131495835045,805.547988625684,116.5918347801));
#72572=CARTESIAN_POINT('Ctrl Pts',(6.72767553170438,805.671414988733,116.633140922881));
#72573=CARTESIAN_POINT('Ctrl Pts',(6.71220824149641,805.924795682934,116.713842608071));
#72574=CARTESIAN_POINT('Ctrl Pts',(6.73053287063395,806.052276455167,116.752456046798));
#72575=CARTESIAN_POINT('Ctrl Pts',(6.81727110090787,806.29490017674,116.822355001029));
#72576=CARTESIAN_POINT('Ctrl Pts',(6.88507115706695,806.40765391491,116.852944154244));
#72577=CARTESIAN_POINT('Ctrl Pts',(7.06193391576527,806.603091405784,116.902253658114));
#72578=CARTESIAN_POINT('Ctrl Pts',(7.16949126667204,806.683778778631,116.920458376782));
#72579=CARTESIAN_POINT('Ctrl Pts',(7.41030387327418,806.801456189114,116.941953730715));
#72580=CARTESIAN_POINT('Ctrl Pts',(7.54128361897485,806.837273557006,116.945023629785));
#72581=CARTESIAN_POINT('Ctrl Pts',(7.80801579791962,806.858554084544,116.935335551326));
#72582=CARTESIAN_POINT('Ctrl Pts',(7.94117176407571,806.84428860958,116.92281340353));
#72583=CARTESIAN_POINT('Ctrl Pts',(8.19492973217388,806.767162435326,116.883150002009));
#72584=CARTESIAN_POINT('Ctrl Pts',(8.31284005106838,806.704449995406,116.856207563332));
#72585=CARTESIAN_POINT('Ctrl Pts',(8.51559192567223,806.538380271382,116.791022007443));
#72586=CARTESIAN_POINT('Ctrl Pts',(8.59835823994668,806.43661688178,116.753403908153));
#72587=CARTESIAN_POINT('Ctrl Pts',(8.71627854751855,806.208756339676,116.672774111363));
#72588=CARTESIAN_POINT('Ctrl Pts',(8.75074276010312,806.085139566965,116.630608505203));
#72589=CARTESIAN_POINT('Ctrl Pts',(8.76736739663133,805.831533572956,116.547156599559));
#72590=CARTESIAN_POINT('Ctrl Pts',(8.74940561479172,805.704022591982,116.506690803449));
#72591=CARTESIAN_POINT('Ctrl Pts',(8.66322225412873,805.462244124062,116.433314171803));
#72592=CARTESIAN_POINT('Ctrl Pts',(8.59600264518925,805.350263292758,116.401094988973));
#72593=CARTESIAN_POINT('Ctrl Pts',(8.42010642511699,805.155324004075,116.349199941691));
#72594=CARTESIAN_POINT('Ctrl Pts',(8.31279114856309,805.074504763307,116.330140613387));
#72595=CARTESIAN_POINT('Ctrl Pts',(8.07106999316088,804.955398951138,116.308176241868));
#72596=CARTESIAN_POINT('Ctrl Pts',(7.93872152846413,804.918792719516,116.305679913427));
#72597=CARTESIAN_POINT('Ctrl Pts',(7.66943048736669,804.896636574549,116.317860827714));
#72598=CARTESIAN_POINT('Ctrl Pts',(7.53512194261262,804.91074897204,116.332228971796));
#72599=CARTESIAN_POINT('Ctrl Pts',(7.28126616695447,804.98780557177,116.375607752691));
#72600=CARTESIAN_POINT('Ctrl Pts',(7.16415682131918,805.049946884604,116.404172651566));
#72601=CARTESIAN_POINT('Ctrl Pts',(7.01282167316582,805.173792299695,116.454808904763));
#72602=CARTESIAN_POINT('Ctrl Pts',(6.96668002233652,805.220108092428,116.472944944874));
#72603=CARTESIAN_POINT('Ctrl Pts',(6.88442731586288,805.321613394483,116.511216276703));
#72604=CARTESIAN_POINT('Ctrl Pts',(6.84865077857284,805.376634956608,116.531272595552));
#72605=CARTESIAN_POINT('Ctrl Pts',(6.81899994463153,805.434810160941,116.55183368117));
#72606=CARTESIAN_POINT('Ctrl Pts',(7.73962524950023,806.213211761693,118.742202927456));
#72607=CARTESIAN_POINT('Ctrl Pts',(7.73966507736922,806.213212446574,118.742200989665));
#72608=CARTESIAN_POINT('Ctrl Pts',(7.73970490535998,806.213213129224,118.742199051195));
#72609=CARTESIAN_POINT('Ctrl Pts',(7.73974473347228,806.213213809644,118.742197112044));
#72610=CARTESIAN_POINT('Ctrl Pts',(7.86972092356887,806.215434311411,118.735868832706));
#72611=CARTESIAN_POINT('Ctrl Pts',(7.99855463379575,806.193855978659,118.722427272111));
#72612=CARTESIAN_POINT('Ctrl Pts',(8.24422874222601,806.104026536541,118.68138442749));
#72613=CARTESIAN_POINT('Ctrl Pts',(8.35807038515727,806.035083011691,118.653698107887));
#72614=CARTESIAN_POINT('Ctrl Pts',(8.55091476656809,805.858369370529,118.586997037738));
#72615=CARTESIAN_POINT('Ctrl Pts',(8.62782091960456,805.752171957187,118.548577303902));
#72616=CARTESIAN_POINT('Ctrl Pts',(8.73310475984059,805.517085137047,118.466025251122));
#72617=CARTESIAN_POINT('Ctrl Pts',(8.76047806328709,805.390546161499,118.422718607167));
#72618=CARTESIAN_POINT('Ctrl Pts',(8.76156941761292,805.134638117182,118.337653443387));
#72619=CARTESIAN_POINT('Ctrl Pts',(8.73555670694445,805.007801765599,118.296741204908));
#72620=CARTESIAN_POINT('Ctrl Pts',(8.63347904356932,804.7699888555,118.223376934523));
#72621=CARTESIAN_POINT('Ctrl Pts',(8.55841972053927,804.661354389114,118.19166745545));
#72622=CARTESIAN_POINT('Ctrl Pts',(8.36795221021987,804.475801335955,118.142186475993));
#72623=CARTESIAN_POINT('Ctrl Pts',(8.25401916512692,804.40108967709,118.125073971573));
#72624=CARTESIAN_POINT('Ctrl Pts',(8.00520544493178,804.298210896697,118.108638494281));
#72625=CARTESIAN_POINT('Ctrl Pts',(7.87305008799637,804.270289227484,118.109184209061));
#72626=CARTESIAN_POINT('Ctrl Pts',(7.73962524950057,804.267101962135,118.118202206281));
#72627=CARTESIAN_POINT('Origin',(7.73962524950056,808.859454792509,108.189819322485));
#72628=CARTESIAN_POINT('',(7.73962524950056,807.196038161002,114.396714565974));
#72629=CARTESIAN_POINT('Origin',(7.73962524950056,806.724615930394,114.230097998707));
#72630=CARTESIAN_POINT('',(7.73962524950071,805.717276769695,118.580698218156));
#72631=CARTESIAN_POINT('',(7.73962524950056,809.330877023117,108.356435889752));
#72632=CARTESIAN_POINT('Ctrl Pts',(7.73942703132262,804.764632786182,118.275191812004));
#72633=CARTESIAN_POINT('Ctrl Pts',(7.6803069953167,804.763344197274,118.27890805784));
#72634=CARTESIAN_POINT('Ctrl Pts',(7.6216351072807,804.772026736497,118.285877779913));
#72635=CARTESIAN_POINT('Ctrl Pts',(7.50497069223838,804.810485868506,118.306576399115));
#72636=CARTESIAN_POINT('Ctrl Pts',(7.44878062387034,804.841967013201,118.320723743749));
#72637=CARTESIAN_POINT('Ctrl Pts',(7.35280716646198,804.924072931586,118.353854150928));
#72638=CARTESIAN_POINT('Ctrl Pts',(7.3139450565688,804.973877909452,118.372506437231));
#72639=CARTESIAN_POINT('Ctrl Pts',(7.25877394270037,805.085573767308,118.411883592206));
#72640=CARTESIAN_POINT('Ctrl Pts',(7.24306220635865,805.146384283711,118.432222756311));
#72641=CARTESIAN_POINT('Ctrl Pts',(7.23718461749696,805.271111529224,118.471992139086));
#72642=CARTESIAN_POINT('Ctrl Pts',(7.24717215376557,805.333806536062,118.491028612901));
#72643=CARTESIAN_POINT('Ctrl Pts',(7.29185694534469,805.452582953991,118.525369496033));
#72644=CARTESIAN_POINT('Ctrl Pts',(7.32618528592688,805.507493346813,118.540334741611));
#72645=CARTESIAN_POINT('Ctrl Pts',(7.41566526079609,805.602831926073,118.564508153228));
#72646=CARTESIAN_POINT('Ctrl Pts',(7.47033225120107,805.641998626575,118.573357622807));
#72647=CARTESIAN_POINT('Ctrl Pts',(7.5916655172645,805.69748301788,118.583323316583));
#72648=CARTESIAN_POINT('Ctrl Pts',(7.65704787848616,805.713424872029,118.584399185988));
#72649=CARTESIAN_POINT('Ctrl Pts',(7.78977309685976,805.720013409946,118.578574448473));
#72650=CARTESIAN_POINT('Ctrl Pts',(7.85579639670194,805.710696997823,118.571760280049));
#72651=CARTESIAN_POINT('Ctrl Pts',(7.97980651809698,805.667916211284,118.550908487762));
#72652=CARTESIAN_POINT('Ctrl Pts',(8.03654060555342,805.634850116953,118.537065832077));
#72653=CARTESIAN_POINT('Ctrl Pts',(8.13285433691024,805.549168836999,118.503954857943));
#72654=CARTESIAN_POINT('Ctrl Pts',(8.1714113386614,805.497367192946,118.485003329618));
#72655=CARTESIAN_POINT('Ctrl Pts',(8.22462677904391,805.382099483559,118.444530402764));
#72656=CARTESIAN_POINT('Ctrl Pts',(8.23875500815394,805.31980323468,118.423419601472));
#72657=CARTESIAN_POINT('Ctrl Pts',(8.24041517411517,805.193361333184,118.382075346817));
#72658=CARTESIAN_POINT('Ctrl Pts',(8.22800820244756,805.130490707571,118.36225839279));
#72659=CARTESIAN_POINT('Ctrl Pts',(8.17823550236331,805.012576685139,118.326773366923));
#72660=CARTESIAN_POINT('Ctrl Pts',(8.14138029080827,804.958704306977,118.311461483642));
#72661=CARTESIAN_POINT('Ctrl Pts',(8.04783721791141,804.867064539568,118.28756208062));
#72662=CARTESIAN_POINT('Ctrl Pts',(7.99198370064763,804.830288815083,118.279248410905));
#72663=CARTESIAN_POINT('Ctrl Pts',(7.8698833274836,804.779719352378,118.271028379672));
#72664=CARTESIAN_POINT('Ctrl Pts',(7.80497283984635,804.766061432163,118.271071646415));
#72665=CARTESIAN_POINT('Ctrl Pts',(7.73942703132262,804.764632786182,118.275191812004));
#72666=CARTESIAN_POINT('Origin',(6.8161311164539,802.337233373458,105.884645588114));
#72667=CARTESIAN_POINT('',(6.81613111645393,797.62882286912,116.361437819037));
#72668=CARTESIAN_POINT('',(6.81613111644524,799.473611621015,116.83203941074));
#72669=CARTESIAN_POINT('Ctrl Pts',(6.81613111645395,797.62882286912,116.361437819037));
#72670=CARTESIAN_POINT('Ctrl Pts',(6.81604355525754,797.628818358335,116.361450581781));
#72671=CARTESIAN_POINT('Ctrl Pts',(6.81595599336896,797.628813859282,116.361463347728));
#72672=CARTESIAN_POINT('Ctrl Pts',(6.69294816100052,797.622510078197,116.379401440403));
#72673=CARTESIAN_POINT('Ctrl Pts',(6.57085364087195,797.639445535317,116.403323434122));
#72674=CARTESIAN_POINT('Ctrl Pts',(6.34388761909424,797.718197941167,116.459742326899));
#72675=CARTESIAN_POINT('Ctrl Pts',(6.24095689020638,797.778570049065,116.491552034475));
#72676=CARTESIAN_POINT('Ctrl Pts',(6.06624785633576,797.935811287255,116.558993650833));
#72677=CARTESIAN_POINT('Ctrl Pts',(5.99624090564599,798.030950164683,116.59390349045));
#72678=CARTESIAN_POINT('Ctrl Pts',(5.89783051725714,798.245491134755,116.662757835106));
#72679=CARTESIAN_POINT('Ctrl Pts',(5.87106446850996,798.362848881483,116.695932839411));
#72680=CARTESIAN_POINT('Ctrl Pts',(5.86545622496071,798.605277690984,116.756533668511));
#72681=CARTESIAN_POINT('Ctrl Pts',(5.8876137635878,798.727906654488,116.783208304679));
#72682=CARTESIAN_POINT('Ctrl Pts',(5.97935436108149,798.961559238557,116.826681074512));
#72683=CARTESIAN_POINT('Ctrl Pts',(6.04891274062436,799.070074424253,116.84288196731));
#72684=CARTESIAN_POINT('Ctrl Pts',(6.22606528446883,799.255811493612,116.862470660604));
#72685=CARTESIAN_POINT('Ctrl Pts',(6.33215286282438,799.331286202517,116.865658921685));
#72686=CARTESIAN_POINT('Ctrl Pts',(6.56488788469013,799.437363932558,116.858520817398));
#72687=CARTESIAN_POINT('Ctrl Pts',(6.68912388985009,799.467641710427,116.848449614987));
#72688=CARTESIAN_POINT('Ctrl Pts',(6.81492901909246,799.47355585377,116.832194910747));
#72689=CARTESIAN_POINT('Ctrl Pts',(6.81532972689165,799.473574691185,116.832143137128));
#72690=CARTESIAN_POINT('Ctrl Pts',(6.81573042608588,799.473593280258,116.832091303782));
#72691=CARTESIAN_POINT('Ctrl Pts',(6.81613111643658,799.473611621015,116.83203941074));
#72692=CARTESIAN_POINT('',(6.81613111645102,800.132384730513,114.968117390021));
#72693=CARTESIAN_POINT('',(6.8161311164539,803.231129546077,106.200578741251));
#72694=CARTESIAN_POINT('Ctrl Pts',(6.01074779320954,798.702525949943,114.667511638846));
#72695=CARTESIAN_POINT('Ctrl Pts',(5.94827792768443,798.797357022413,114.701028148547));
#72696=CARTESIAN_POINT('Ctrl Pts',(5.9052416446383,798.90336977999,114.735148867139));
#72697=CARTESIAN_POINT('Ctrl Pts',(5.86113093765785,799.132940900446,114.803009124232));
#72698=CARTESIAN_POINT('Ctrl Pts',(5.86298459699158,799.254773993399,114.835923698928));
#72699=CARTESIAN_POINT('Ctrl Pts',(5.91459578159424,799.490217611791,114.893931625604));
#72700=CARTESIAN_POINT('Ctrl Pts',(5.96304364173721,799.601724382295,114.918612352913));
#72701=CARTESIAN_POINT('Ctrl Pts',(6.10107809442051,799.803724061892,114.957771793913));
#72702=CARTESIAN_POINT('Ctrl Pts',(6.19004984522366,799.892004700308,114.971728064651));
#72703=CARTESIAN_POINT('Ctrl Pts',(6.39791598941777,800.032415704775,114.98676179417));
#72704=CARTESIAN_POINT('Ctrl Pts',(6.51524274215751,800.082787547882,114.987540321836));
#72705=CARTESIAN_POINT('Ctrl Pts',(6.76216901966767,800.137060182909,114.975266908503));
#72706=CARTESIAN_POINT('Ctrl Pts',(6.88941986686158,800.140328981772,114.962295780724));
#72707=CARTESIAN_POINT('Ctrl Pts',(7.13112049099513,800.099261451316,114.92462821992));
#72708=CARTESIAN_POINT('Ctrl Pts',(7.243641089916,800.05730492707,114.900790689718));
#72709=CARTESIAN_POINT('Ctrl Pts',(7.44159738664962,799.93602222134,114.845459049661));
#72710=CARTESIAN_POINT('Ctrl Pts',(7.5260284388434,799.859065132993,114.814735960931));
#72711=CARTESIAN_POINT('Ctrl Pts',(7.66080878524161,799.677746268727,114.749046306696));
#72712=CARTESIAN_POINT('Ctrl Pts',(7.70972833342177,799.574899724096,114.714659560811));
#72713=CARTESIAN_POINT('Ctrl Pts',(7.76602834666594,799.35303571267,114.645696771555));
#72714=CARTESIAN_POINT('Ctrl Pts',(7.77173807031252,799.235793970228,114.611805892869));
#72715=CARTESIAN_POINT('Ctrl Pts',(7.73632287345495,798.998077719297,114.54835520444));
#72716=CARTESIAN_POINT('Ctrl Pts',(7.69309018749097,798.88021558252,114.519780523955));
#72717=CARTESIAN_POINT('Ctrl Pts',(7.56350523489464,798.66871882365,114.474693520515));
#72718=CARTESIAN_POINT('Ctrl Pts',(7.47937350020835,798.576590694492,114.458353560822));
#72719=CARTESIAN_POINT('Ctrl Pts',(7.27928281246208,798.426295646752,114.439354510948));
#72720=CARTESIAN_POINT('Ctrl Pts',(7.16475879310693,798.37001284635,114.437065330823));
#72721=CARTESIAN_POINT('Ctrl Pts',(6.9202875494757,798.302478660598,114.447276891869));
#72722=CARTESIAN_POINT('Ctrl Pts',(6.79251849366301,798.292279934721,114.459811382783));
#72723=CARTESIAN_POINT('Ctrl Pts',(6.5551195704484,798.319492011922,114.496051856014));
#72724=CARTESIAN_POINT('Ctrl Pts',(6.44687289501309,798.351848729651,114.518167590459));
#72725=CARTESIAN_POINT('Ctrl Pts',(6.24374667406768,798.455422307701,114.571427367212));
#72726=CARTESIAN_POINT('Ctrl Pts',(6.15171553339862,798.52754715734,114.602467143043));
#72727=CARTESIAN_POINT('Ctrl Pts',(6.05284563521359,798.642825807817,114.646066270405));
#72728=CARTESIAN_POINT('Ctrl Pts',(6.0308327767351,798.672036360887,114.656735586433));
#72729=CARTESIAN_POINT('Ctrl Pts',(6.01074779320959,798.702525949943,114.667511638846));
#72730=CARTESIAN_POINT('Ctrl Pts',(6.81613111643658,799.473611621015,116.83203941074));
#72731=CARTESIAN_POINT('Ctrl Pts',(6.93665525034905,799.479128359434,116.816430439957));
#72732=CARTESIAN_POINT('Ctrl Pts',(7.05637978296077,799.462177662245,116.795424117734));
#72733=CARTESIAN_POINT('Ctrl Pts',(7.28486648494508,799.383439235941,116.743426257329));
#72734=CARTESIAN_POINT('Ctrl Pts',(7.39079152683966,799.321029728914,116.712656173739));
#72735=CARTESIAN_POINT('Ctrl Pts',(7.56791944632267,799.16008888171,116.646186311464));
#72736=CARTESIAN_POINT('Ctrl Pts',(7.6380109240145,799.064003562227,116.611278377729));
#72737=CARTESIAN_POINT('Ctrl Pts',(7.73638929751765,798.847176413892,116.540457276636));
#72738=CARTESIAN_POINT('Ctrl Pts',(7.76266176660441,798.728252097948,116.505299866886));
#72739=CARTESIAN_POINT('Ctrl Pts',(7.76563629988533,798.485488138897,116.440662166943));
#72740=CARTESIAN_POINT('Ctrl Pts',(7.74229368430618,798.364173750922,116.411869578574));
#72741=CARTESIAN_POINT('Ctrl Pts',(7.64895664758895,798.134509339619,116.364886523339));
#72742=CARTESIAN_POINT('Ctrl Pts',(7.57953802933586,798.028539756959,116.347255576251));
#72743=CARTESIAN_POINT('Ctrl Pts',(7.40288190392766,797.845687558127,116.325994048102));
#72744=CARTESIAN_POINT('Ctrl Pts',(7.29677536501533,797.770950015637,116.322769350076));
#72745=CARTESIAN_POINT('Ctrl Pts',(7.06473329425217,797.665608558726,116.331537351354));
#72746=CARTESIAN_POINT('Ctrl Pts',(6.94113661840373,797.635262627994,116.343217269045));
#72747=CARTESIAN_POINT('Ctrl Pts',(6.81613111645396,797.62882286912,116.361437819037));
#72748=CARTESIAN_POINT('Origin',(6.8161311164539,802.337233373458,105.884645588114));
#72749=CARTESIAN_POINT('',(6.8161311164539,800.673816741952,112.091540831602));
#72750=CARTESIAN_POINT('Origin',(6.8161311164539,800.202394511343,111.924924264335));
#72751=CARTESIAN_POINT('',(6.8161311164541,799.038612298614,116.718161934316));
#72752=CARTESIAN_POINT('',(6.8161311164539,802.808655604067,106.051262155381));
#72753=CARTESIAN_POINT('Ctrl Pts',(6.81580794006168,798.065704838105,116.469988878972));
#72754=CARTESIAN_POINT('Ctrl Pts',(6.7543796153778,798.062661509509,116.47871877281));
#72755=CARTESIAN_POINT('Ctrl Pts',(6.69332155622728,798.070633238579,116.49025344683));
#72756=CARTESIAN_POINT('Ctrl Pts',(6.57572131339275,798.108967467512,116.518312508229));
#72757=CARTESIAN_POINT('Ctrl Pts',(6.52061302842095,798.139893322244,116.534754014128));
#72758=CARTESIAN_POINT('Ctrl Pts',(6.4266136932548,798.221243656218,116.569952156603));
#72759=CARTESIAN_POINT('Ctrl Pts',(6.3886468697899,798.270755429356,116.588332923346));
#72760=CARTESIAN_POINT('Ctrl Pts',(6.33456190763045,798.382768281265,116.624869201289));
#72761=CARTESIAN_POINT('Ctrl Pts',(6.31925762111652,798.444190102766,116.642626950885));
#72762=CARTESIAN_POINT('Ctrl Pts',(6.31381941331088,798.571424709535,116.675330894803));
#72763=CARTESIAN_POINT('Ctrl Pts',(6.32418796365442,798.635961269097,116.689882275963));
#72764=CARTESIAN_POINT('Ctrl Pts',(6.3701557089184,798.760009329424,116.713961899536));
#72765=CARTESIAN_POINT('Ctrl Pts',(6.40597239703097,798.818105205021,116.723108038333));
#72766=CARTESIAN_POINT('Ctrl Pts',(6.49792294837037,798.917744697554,116.734374023444));
#72767=CARTESIAN_POINT('Ctrl Pts',(6.55314738059275,798.95843843497,116.736417804411));
#72768=CARTESIAN_POINT('Ctrl Pts',(6.67518620580731,799.016665101815,116.733140858802));
#72769=CARTESIAN_POINT('Ctrl Pts',(6.74080209751259,799.03386033086,116.727909106));
#72770=CARTESIAN_POINT('Ctrl Pts',(6.87363166527902,799.04236903342,116.710754030943));
#72771=CARTESIAN_POINT('Ctrl Pts',(6.93955714260679,799.033781679734,116.69903933778));
#72772=CARTESIAN_POINT('Ctrl Pts',(7.06143948004197,798.99220535637,116.670801611149));
#72773=CARTESIAN_POINT('Ctrl Pts',(7.116420129854,798.960307081348,116.654695294223));
#72774=CARTESIAN_POINT('Ctrl Pts',(7.20970171777221,798.877245271801,116.619831929976));
#72775=CARTESIAN_POINT('Ctrl Pts',(7.24711464410287,798.827017237173,116.601442688545));
#72776=CARTESIAN_POINT('Ctrl Pts',(7.29989636346429,798.713693781464,116.564419428754));
#72777=CARTESIAN_POINT('Ctrl Pts',(7.31435912177347,798.651621065621,116.546181155725));
#72778=CARTESIAN_POINT('Ctrl Pts',(7.31762356009194,798.52358749062,116.512414208227));
#72779=CARTESIAN_POINT('Ctrl Pts',(7.305975167089,798.458935039213,116.497294475349));
#72780=CARTESIAN_POINT('Ctrl Pts',(7.25768541697495,798.336446873472,116.472618764187));
#72781=CARTESIAN_POINT('Ctrl Pts',(7.22137443733566,798.279868390151,116.463344637139));
#72782=CARTESIAN_POINT('Ctrl Pts',(7.12870284052068,798.18240642053,116.452059821675));
#72783=CARTESIAN_POINT('Ctrl Pts',(7.07303448450468,798.142563640943,116.450217458438));
#72784=CARTESIAN_POINT('Ctrl Pts',(6.94973861296488,798.085560492895,116.45439380324));
#72785=CARTESIAN_POINT('Ctrl Pts',(6.8831701538097,798.069042147929,116.460415689768));
#72786=CARTESIAN_POINT('Ctrl Pts',(6.81580794006168,798.065704838105,116.469988878972));
#72787=CARTESIAN_POINT('Origin',(4.21616833870003,818.154693156259,111.475071072488));
#72788=CARTESIAN_POINT('',(4.21616833870006,813.566663386125,121.391222359302));
#72789=CARTESIAN_POINT('',(4.21616833869997,815.503730966578,122.040806989507));
#72790=CARTESIAN_POINT('Ctrl Pts',(4.21616833870006,813.566663386125,121.391222359302));
#72791=CARTESIAN_POINT('Ctrl Pts',(4.21579739595471,813.566654326904,121.391247991317));
#72792=CARTESIAN_POINT('Ctrl Pts',(4.21542644360822,813.566645457546,121.391273692532));
#72793=CARTESIAN_POINT('Ctrl Pts',(4.08151962453409,813.563512416058,121.400576088745));
#72794=CARTESIAN_POINT('Ctrl Pts',(3.94927725818734,813.585048816235,121.4186585503));
#72795=CARTESIAN_POINT('Ctrl Pts',(3.70290827213485,813.675056767274,121.469733158647));
#72796=CARTESIAN_POINT('Ctrl Pts',(3.59101711651222,813.7424945632,121.502170135717));
#72797=CARTESIAN_POINT('Ctrl Pts',(3.40222886819611,813.915004724076,121.576569498705));
#72798=CARTESIAN_POINT('Ctrl Pts',(3.32706623318748,814.018333135414,121.61778141041));
#72799=CARTESIAN_POINT('Ctrl Pts',(3.22340449421018,814.24827939509,121.703389039361));
#72800=CARTESIAN_POINT('Ctrl Pts',(3.19605986775251,814.372671216344,121.746936556848));
#72801=CARTESIAN_POINT('Ctrl Pts',(3.19354318820913,814.626689524154,121.830781575904));
#72802=CARTESIAN_POINT('Ctrl Pts',(3.21870879655004,814.753790459032,121.87022216573));
#72803=CARTESIAN_POINT('Ctrl Pts',(3.3190825739423,814.99329705162,121.94007184856));
#72804=CARTESIAN_POINT('Ctrl Pts',(3.39352917219228,815.103278725567,121.969767839707));
#72805=CARTESIAN_POINT('Ctrl Pts',(3.5820490759131,815.290378121672,122.0158818445));
#72806=CARTESIAN_POINT('Ctrl Pts',(3.69433488590728,815.365693067524,122.03186961327));
#72807=CARTESIAN_POINT('Ctrl Pts',(3.94402218175684,815.471858923636,122.048509266252));
#72808=CARTESIAN_POINT('Ctrl Pts',(4.0793366716235,815.500912444094,122.048750602559));
#72809=CARTESIAN_POINT('Ctrl Pts',(4.21609103298932,815.503729376994,122.04081147827));
#72810=CARTESIAN_POINT('Ctrl Pts',(4.21611680160463,815.503729907789,122.040809982302));
#72811=CARTESIAN_POINT('Ctrl Pts',(4.21614257017483,815.50373043765,122.040808486047));
#72812=CARTESIAN_POINT('Ctrl Pts',(4.21616833869989,815.503730966578,122.040806989507));
#72813=CARTESIAN_POINT('',(4.21616833820598,816.141966729996,120.234993004862));
#72814=CARTESIAN_POINT('',(4.21616833870003,819.117722296501,111.815438155555));
#72815=CARTESIAN_POINT('Ctrl Pts',(3.22367932508172,814.919632311137,119.90409075603));
#72816=CARTESIAN_POINT('Ctrl Pts',(3.19221248465311,815.041645449644,119.947214327596));
#72817=CARTESIAN_POINT('Ctrl Pts',(3.18636504709321,815.168984840346,119.989903466751));
#72818=CARTESIAN_POINT('Ctrl Pts',(3.22649682289723,815.419921359348,120.069741297725));
#72819=CARTESIAN_POINT('Ctrl Pts',(3.27208612232692,815.541068456448,120.106116201354));
#72820=CARTESIAN_POINT('Ctrl Pts',(3.4093328644833,815.761495951288,120.16817025803));
#72821=CARTESIAN_POINT('Ctrl Pts',(3.49987357034009,815.858558603504,120.193213650547));
#72822=CARTESIAN_POINT('Ctrl Pts',(3.71459906287451,816.015190894562,120.228808083796));
#72823=CARTESIAN_POINT('Ctrl Pts',(3.8368843217803,816.073101566701,120.238962745765));
#72824=CARTESIAN_POINT('Ctrl Pts',(4.09699197200466,816.141139309507,120.242913761541));
#72825=CARTESIAN_POINT('Ctrl Pts',(4.23234340884442,816.150564070566,120.23665562034));
#72826=CARTESIAN_POINT('Ctrl Pts',(4.49674721742275,816.119210643793,120.208364921513));
#72827=CARTESIAN_POINT('Ctrl Pts',(4.62332939543466,816.079205911963,120.186745649431));
#72828=CARTESIAN_POINT('Ctrl Pts',(4.85367522162754,815.954106530113,120.130126893132));
#72829=CARTESIAN_POINT('Ctrl Pts',(4.95484884405447,815.869683540675,120.09551121166));
#72830=CARTESIAN_POINT('Ctrl Pts',(5.11609946869123,815.667542280614,120.017576754425));
#72831=CARTESIAN_POINT('Ctrl Pts',(5.17450233019456,815.551789456814,119.975014315745));
#72832=CARTESIAN_POINT('Ctrl Pts',(5.2395923823904,815.305793146957,119.887974724992));
#72833=CARTESIAN_POINT('Ctrl Pts',(5.24614971038165,815.178111264852,119.844372371625));
#72834=CARTESIAN_POINT('Ctrl Pts',(5.2069152812454,814.926745832242,119.761712356192));
#72835=CARTESIAN_POINT('Ctrl Pts',(5.16154664126315,814.805510702664,119.723464658313));
#72836=CARTESIAN_POINT('Ctrl Pts',(5.02476739304651,814.585827148372,119.657897116744));
#72837=CARTESIAN_POINT('Ctrl Pts',(4.93483302848475,814.489419795905,119.631182128276));
#72838=CARTESIAN_POINT('Ctrl Pts',(4.72097148078736,814.333104311715,119.592938040371));
#72839=CARTESIAN_POINT('Ctrl Pts',(4.59883794649819,814.275022747381,119.581914976267));
#72840=CARTESIAN_POINT('Ctrl Pts',(4.33752909919282,814.205765672262,119.577568835096));
#72841=CARTESIAN_POINT('Ctrl Pts',(4.20072395219808,814.195831741583,119.584499400288));
#72842=CARTESIAN_POINT('Ctrl Pts',(3.93381826417745,814.226811054965,119.615460183439));
#72843=CARTESIAN_POINT('Ctrl Pts',(3.80620658292549,814.266878946968,119.639001877507));
#72844=CARTESIAN_POINT('Ctrl Pts',(3.57600886078964,814.391903770064,119.699334251585));
#72845=CARTESIAN_POINT('Ctrl Pts',(3.47561916032804,814.475598574139,119.735516883545));
#72846=CARTESIAN_POINT('Ctrl Pts',(3.355376499897,814.62635652068,119.795664935966));
#72847=CARTESIAN_POINT('Ctrl Pts',(3.32057888538006,814.680693147426,119.816635810209));
#72848=CARTESIAN_POINT('Ctrl Pts',(3.26267307358109,814.796087730609,119.859816083944));
#72849=CARTESIAN_POINT('Ctrl Pts',(3.23985369072435,814.856915969473,119.881924678826));
#72850=CARTESIAN_POINT('Ctrl Pts',(3.22367932508172,814.919632311137,119.90409075603));
#72851=CARTESIAN_POINT('Ctrl Pts',(4.21616833869988,815.503730966578,122.040806989507));
#72852=CARTESIAN_POINT('Ctrl Pts',(4.347914315043,815.506435201059,122.033155672043));
#72853=CARTESIAN_POINT('Ctrl Pts',(4.47848121683415,815.484739441053,122.018051117122));
#72854=CARTESIAN_POINT('Ctrl Pts',(4.72499390664615,815.39419730065,121.973661824122));
#72855=CARTESIAN_POINT('Ctrl Pts',(4.83821063321016,815.325410607071,121.94454951115));
#72856=CARTESIAN_POINT('Ctrl Pts',(5.02957904846655,815.14947769508,121.875347618212));
#72857=CARTESIAN_POINT('Ctrl Pts',(5.10575399381212,815.043985810499,121.835898711131));
#72858=CARTESIAN_POINT('Ctrl Pts',(5.21013900292989,814.810264999246,121.751319288353));
#72859=CARTESIAN_POINT('Ctrl Pts',(5.2372210297118,814.68430473374,121.707007309095));
#72860=CARTESIAN_POINT('Ctrl Pts',(5.23792432954282,814.429332562611,121.619731263981));
#72861=CARTESIAN_POINT('Ctrl Pts',(5.21167957665196,814.302835549282,121.577632118039));
#72862=CARTESIAN_POINT('Ctrl Pts',(5.10914639550353,814.066009917319,121.501902354179));
#72863=CARTESIAN_POINT('Ctrl Pts',(5.03394315201209,813.957983982788,121.469023268446));
#72864=CARTESIAN_POINT('Ctrl Pts',(4.84358596990866,813.773904052068,121.417492551366));
#72865=CARTESIAN_POINT('Ctrl Pts',(4.73003738953763,813.699925994421,121.399478445952));
#72866=CARTESIAN_POINT('Ctrl Pts',(4.4816910942168,813.59771819199,121.381759167324));
#72867=CARTESIAN_POINT('Ctrl Pts',(4.34954949966834,813.569920841612,121.382005767238));
#72868=CARTESIAN_POINT('Ctrl Pts',(4.21616833870007,813.566663386125,121.391222359302));
#72869=CARTESIAN_POINT('Origin',(4.21616833870003,818.154693156259,111.475071072488));
#72870=CARTESIAN_POINT('',(4.21616833870003,816.491276524752,117.681966315976));
#72871=CARTESIAN_POINT('Origin',(4.21616833870003,816.019854294144,117.515349748709));
#72872=CARTESIAN_POINT('',(4.2161683387002,815.009671259245,121.873996379995));
#72873=CARTESIAN_POINT('',(4.21616833870003,818.626115386867,111.641687639755));
#72874=CARTESIAN_POINT('Ctrl Pts',(4.21591630885621,814.061445921076,121.555988002616));
#72875=CARTESIAN_POINT('Ctrl Pts',(4.15552196213932,814.06006265502,121.559993147844));
#72876=CARTESIAN_POINT('Ctrl Pts',(4.09561609080141,814.069024841709,121.567563518964));
#72877=CARTESIAN_POINT('Ctrl Pts',(3.97808181203072,814.108345878869,121.589863612151));
#72878=CARTESIAN_POINT('Ctrl Pts',(3.92213372965487,814.139987972191,121.604903509755));
#72879=CARTESIAN_POINT('Ctrl Pts',(3.82687081961698,814.222171178162,121.640013468081));
#72880=CARTESIAN_POINT('Ctrl Pts',(3.78843887181263,814.271878293051,121.659730173664));
#72881=CARTESIAN_POINT('Ctrl Pts',(3.7342215244729,814.383144228812,121.701216799812));
#72882=CARTESIAN_POINT('Ctrl Pts',(3.71899499190225,814.443619358232,121.72257857952));
#72883=CARTESIAN_POINT('Ctrl Pts',(3.71404760608176,814.567586012134,121.764179312166));
#72884=CARTESIAN_POINT('Ctrl Pts',(3.72447129863588,814.629856435003,121.784002021646));
#72885=CARTESIAN_POINT('Ctrl Pts',(3.76995848233187,814.747832107846,121.819548530303));
#72886=CARTESIAN_POINT('Ctrl Pts',(3.80466518948911,814.802353856866,121.83491178086));
#72887=CARTESIAN_POINT('Ctrl Pts',(3.89394549383036,814.896045752094,121.859198985713));
#72888=CARTESIAN_POINT('Ctrl Pts',(3.9476868533989,814.934292287786,121.867884107372));
#72889=CARTESIAN_POINT('Ctrl Pts',(4.06825440704684,814.989633510265,121.8775506611));
#72890=CARTESIAN_POINT('Ctrl Pts',(4.13411280462523,815.005766201399,121.878289859009));
#72891=CARTESIAN_POINT('Ctrl Pts',(4.26752485498035,815.012468557479,121.871423147378));
#72892=CARTESIAN_POINT('Ctrl Pts',(4.33374585310983,815.003161618151,121.863945434534));
#72893=CARTESIAN_POINT('Ctrl Pts',(4.45770354762203,814.960416980212,121.841647371366));
#72894=CARTESIAN_POINT('Ctrl Pts',(4.5142390171448,814.927495645059,121.827072175354));
#72895=CARTESIAN_POINT('Ctrl Pts',(4.61004378864544,814.842319992247,121.792524512427));
#72896=CARTESIAN_POINT('Ctrl Pts',(4.64834689317697,814.790915143196,121.772892696958));
#72897=CARTESIAN_POINT('Ctrl Pts',(4.70125386041098,814.676480271627,121.731066229657));
#72898=CARTESIAN_POINT('Ctrl Pts',(4.71530778575685,814.614593841588,121.709289011278));
#72899=CARTESIAN_POINT('Ctrl Pts',(4.7169515869088,814.488829597756,121.66660187769));
#72900=CARTESIAN_POINT('Ctrl Pts',(4.70454822428203,814.426216132537,121.646121994441));
#72901=CARTESIAN_POINT('Ctrl Pts',(4.65477641739308,814.308732600749,121.609400206655));
#72902=CARTESIAN_POINT('Ctrl Pts',(4.61790622062084,814.255038285866,121.593530522019));
#72903=CARTESIAN_POINT('Ctrl Pts',(4.52434712330669,814.163717598429,121.568741666655));
#72904=CARTESIAN_POINT('Ctrl Pts',(4.46850982709221,814.127074978406,121.560104934687));
#72905=CARTESIAN_POINT('Ctrl Pts',(4.34640555546615,814.076609567842,121.55157551949));
#72906=CARTESIAN_POINT('Ctrl Pts',(4.2814711554186,814.062947382702,121.551640630799));
#72907=CARTESIAN_POINT('Ctrl Pts',(4.21591630885621,814.061445921076,121.555988002616));
#72908=CARTESIAN_POINT('Origin',(1.87460472916284,811.956028988243,109.284253418465));
#72909=CARTESIAN_POINT('',(1.87460472916284,807.25641609678,119.736153825281));
#72910=CARTESIAN_POINT('',(1.87460472914096,809.080906302795,120.264187795611));
#72911=CARTESIAN_POINT('Ctrl Pts',(1.87460472916287,807.25641609678,119.736153825281));
#72912=CARTESIAN_POINT('Ctrl Pts',(1.75103549584412,807.24947860926,119.755782640683));
#72913=CARTESIAN_POINT('Ctrl Pts',(1.62836973988592,807.265718400088,119.78233157051));
#72914=CARTESIAN_POINT('Ctrl Pts',(1.40065186333159,807.342855758013,119.845485989263));
#72915=CARTESIAN_POINT('Ctrl Pts',(1.29742613189207,807.40234385158,119.881340847999));
#72916=CARTESIAN_POINT('Ctrl Pts',(1.12314017366551,807.557234499257,119.957439014239));
#72917=CARTESIAN_POINT('Ctrl Pts',(1.05351618053732,807.650714655165,119.996862573774));
#72918=CARTESIAN_POINT('Ctrl Pts',(0.956087033711997,807.861277422583,120.074560571483));
#72919=CARTESIAN_POINT('Ctrl Pts',(0.929579051060437,807.976212894383,120.111984351191));
#72920=CARTESIAN_POINT('Ctrl Pts',(0.923909377596282,808.214128449828,120.180375364673));
#72921=CARTESIAN_POINT('Ctrl Pts',(0.945672229366337,808.334631279297,120.210477268493));
#72922=CARTESIAN_POINT('Ctrl Pts',(1.03601846715911,808.564880083577,120.259459016282));
#72923=CARTESIAN_POINT('Ctrl Pts',(1.10451976956373,808.672072392336,120.277646302952));
#72924=CARTESIAN_POINT('Ctrl Pts',(1.28056330507626,808.858173895426,120.299796035088));
#72925=CARTESIAN_POINT('Ctrl Pts',(1.38723989220875,808.934688042217,120.303253530113));
#72926=CARTESIAN_POINT('Ctrl Pts',(1.62152018801628,809.042855486623,120.294711538717));
#72927=CARTESIAN_POINT('Ctrl Pts',(1.74674633614967,809.074099378817,120.282986895974));
#72928=CARTESIAN_POINT('Ctrl Pts',(1.8734622404411,809.080846138924,120.264355956543));
#72929=CARTESIAN_POINT('Ctrl Pts',(1.87384307751858,809.080866415908,120.264299962368));
#72930=CARTESIAN_POINT('Ctrl Pts',(1.87422390714615,809.080886470526,120.264243908713));
#72931=CARTESIAN_POINT('Ctrl Pts',(1.87460472911907,809.080906302795,120.264187795611));
#72932=CARTESIAN_POINT('',(1.87460472916012,809.743718201466,118.388838489889));
#72933=CARTESIAN_POINT('',(1.87460472916284,812.849925160862,109.600186571602));
#72934=CARTESIAN_POINT('Ctrl Pts',(0.982819008185952,808.489505833977,118.126561480607));
#72935=CARTESIAN_POINT('Ctrl Pts',(0.942625967695021,808.594510486907,118.163673677874));
#72936=CARTESIAN_POINT('Ctrl Pts',(0.923675628408658,808.706665929454,118.199965429178));
#72937=CARTESIAN_POINT('Ctrl Pts',(0.930232869014416,808.939958483743,118.269140966905));
#72938=CARTESIAN_POINT('Ctrl Pts',(0.958209188629994,809.05883551688,118.301010770041));
#72939=CARTESIAN_POINT('Ctrl Pts',(1.05886514447545,809.279189926667,118.35368565984));
#72940=CARTESIAN_POINT('Ctrl Pts',(1.129822751318,809.378863980049,118.374184304548));
#72941=CARTESIAN_POINT('Ctrl Pts',(1.307151577289,809.549612121828,118.402298394661));
#72942=CARTESIAN_POINT('Ctrl Pts',(1.41245152614895,809.6186410281,118.40945045186));
#72943=CARTESIAN_POINT('Ctrl Pts',(1.64434142181353,809.715473551999,118.409082071832));
#72944=CARTESIAN_POINT('Ctrl Pts',(1.76903255340026,809.741862161876,118.401384113382));
#72945=CARTESIAN_POINT('Ctrl Pts',(2.02035153667182,809.746760213165,118.371660051525));
#72946=CARTESIAN_POINT('Ctrl Pts',(2.14456374543044,809.725109791134,118.349881627919));
#72947=CARTESIAN_POINT('Ctrl Pts',(2.37032250526495,809.637718463314,118.295841669722));
#72948=CARTESIAN_POINT('Ctrl Pts',(2.47050805225589,809.574683409597,118.264554273995));
#72949=CARTESIAN_POINT('Ctrl Pts',(2.63653013030491,809.417331558491,118.196474577532));
#72950=CARTESIAN_POINT('Ctrl Pts',(2.70190179787091,809.325529478102,118.160504766322));
#72951=CARTESIAN_POINT('Ctrl Pts',(2.79364204544573,809.121763114752,118.08688140638));
#72952=CARTESIAN_POINT('Ctrl Pts',(2.81894932283529,809.011560918391,118.049894924289));
#72953=CARTESIAN_POINT('Ctrl Pts',(2.82574944824385,808.783443875928,117.978722102287));
#72954=CARTESIAN_POINT('Ctrl Pts',(2.80600362724193,808.667593067868,117.945322826876));
#72955=CARTESIAN_POINT('Ctrl Pts',(2.72036714624902,808.441872668529,117.886111878289));
#72956=CARTESIAN_POINT('Ctrl Pts',(2.65299513231454,808.334971119733,117.861411040457));
#72957=CARTESIAN_POINT('Ctrl Pts',(2.48165878776808,808.153294742417,117.826863568856));
#72958=CARTESIAN_POINT('Ctrl Pts',(2.38017372238493,808.079560671286,117.817024691649));
#72959=CARTESIAN_POINT('Ctrl Pts',(2.15367708819099,807.971539124383,117.81296652733));
#72960=CARTESIAN_POINT('Ctrl Pts',(2.03046406548969,807.938815338816,117.819003900188));
#72961=CARTESIAN_POINT('Ctrl Pts',(1.77880397588497,807.920446253038,117.846592071107));
#72962=CARTESIAN_POINT('Ctrl Pts',(1.65269616866143,807.935405948966,117.868018399543));
#72963=CARTESIAN_POINT('Ctrl Pts',(1.42833017212113,808.008377519518,117.920431826035));
#72964=CARTESIAN_POINT('Ctrl Pts',(1.33032402726732,808.061173261856,117.949771403349));
#72965=CARTESIAN_POINT('Ctrl Pts',(1.15562996349709,808.202187676284,118.01626403852));
#72966=CARTESIAN_POINT('Ctrl Pts',(1.08189897272091,808.290739046924,118.053109502678));
#72967=CARTESIAN_POINT('Ctrl Pts',(1.01080818798242,808.422860282031,118.102661369331));
#72968=CARTESIAN_POINT('Ctrl Pts',(0.995741663762431,808.455745288689,118.114629361585));
#72969=CARTESIAN_POINT('Ctrl Pts',(0.982819008185979,808.489505833977,118.126561480607));
#72970=CARTESIAN_POINT('Ctrl Pts',(1.87460472911908,809.080906302795,120.264187795611));
#72971=CARTESIAN_POINT('Ctrl Pts',(1.99072328499639,809.08695347077,120.247078036002));
#72972=CARTESIAN_POINT('Ctrl Pts',(2.10613151435791,809.072325787297,120.224449647386));
#72973=CARTESIAN_POINT('Ctrl Pts',(2.33134970731173,809.00036503431,120.168049079998));
#72974=CARTESIAN_POINT('Ctrl Pts',(2.43799701456852,808.940890665549,120.134168739612));
#72975=CARTESIAN_POINT('Ctrl Pts',(2.61920945920015,808.783876834124,120.060218809982));
#72976=CARTESIAN_POINT('Ctrl Pts',(2.69190568992126,808.688020815213,120.020918203225));
#72977=CARTESIAN_POINT('Ctrl Pts',(2.79289670773424,808.472524860687,119.941871820671));
#72978=CARTESIAN_POINT('Ctrl Pts',(2.82010327914144,808.355185743614,119.902969138478));
#72979=CARTESIAN_POINT('Ctrl Pts',(2.8249240987974,808.114954932764,119.831056598888));
#72980=CARTESIAN_POINT('Ctrl Pts',(2.80249149175379,807.99460496946,119.798816682038));
#72981=CARTESIAN_POINT('Ctrl Pts',(2.71086408106223,807.766515535603,119.745718689865));
#72982=CARTESIAN_POINT('Ctrl Pts',(2.64238875976384,807.661168277672,119.725471164478));
#72983=CARTESIAN_POINT('Ctrl Pts',(2.46772646343663,807.47885372346,119.700171889594));
#72984=CARTESIAN_POINT('Ctrl Pts',(2.36276911691211,807.404025681426,119.695569077496));
#72985=CARTESIAN_POINT('Ctrl Pts',(2.12960285019528,807.295668215198,119.703274012147));
#72986=CARTESIAN_POINT('Ctrl Pts',(2.00322961320662,807.263752966054,119.715757176099));
#72987=CARTESIAN_POINT('Ctrl Pts',(1.87519983982174,807.2564496419,119.736059333623));
#72988=CARTESIAN_POINT('Ctrl Pts',(1.87490228187681,807.256432802138,119.736106559411));
#72989=CARTESIAN_POINT('Ctrl Pts',(1.87460472916285,807.25641609678,119.736153825281));
#72990=CARTESIAN_POINT('Origin',(1.87460472916284,811.956028988243,109.284253418465));
#72991=CARTESIAN_POINT('',(1.87460472916284,810.292612356737,115.491148661954));
#72992=CARTESIAN_POINT('Origin',(1.87460472916284,809.821190126128,115.324532094686));
#72993=CARTESIAN_POINT('',(1.87460472916283,808.650347571495,120.137746182282));
#72994=CARTESIAN_POINT('',(1.87460472916284,812.427451218852,109.450869985732));
#72995=CARTESIAN_POINT('Ctrl Pts',(1.87415121283263,807.688135745084,119.859311375963));
#72996=CARTESIAN_POINT('Ctrl Pts',(1.81123905313606,807.684719945843,119.86914722499));
#72997=CARTESIAN_POINT('Ctrl Pts',(1.74876005479557,807.6927213796,119.882310692792));
#72998=CARTESIAN_POINT('Ctrl Pts',(1.63002655636162,807.73146338099,119.914217166966));
#72999=CARTESIAN_POINT('Ctrl Pts',(1.57503418290112,807.762342951292,119.93277936381));
#73000=CARTESIAN_POINT('Ctrl Pts',(1.48186889472678,807.843247470558,119.972450053152));
#73001=CARTESIAN_POINT('Ctrl Pts',(1.44446864217568,807.892267856135,119.99313112845));
#73002=CARTESIAN_POINT('Ctrl Pts',(1.39174295307579,808.002842937753,120.034135637593));
#73003=CARTESIAN_POINT('Ctrl Pts',(1.37706602145846,808.063263908712,120.054018864579));
#73004=CARTESIAN_POINT('Ctrl Pts',(1.37267743184874,808.188397163861,120.090588415092));
#73005=CARTESIAN_POINT('Ctrl Pts',(1.38340164071457,808.251816608146,120.106829571659));
#73006=CARTESIAN_POINT('Ctrl Pts',(1.42962580928306,808.373487772313,120.133572743112));
#73007=CARTESIAN_POINT('Ctrl Pts',(1.46517305774742,808.430358508466,120.143676182847));
#73008=CARTESIAN_POINT('Ctrl Pts',(1.55686256304649,808.529152863639,120.156235685135));
#73009=CARTESIAN_POINT('Ctrl Pts',(1.61245004635588,808.569888017684,120.158452324485));
#73010=CARTESIAN_POINT('Ctrl Pts',(1.73523469610953,808.628298955917,120.154543940035));
#73011=CARTESIAN_POINT('Ctrl Pts',(1.80125316755559,808.645590502154,120.148506330388));
#73012=CARTESIAN_POINT('Ctrl Pts',(1.93450917179671,808.654304616807,120.128978862922));
#73013=CARTESIAN_POINT('Ctrl Pts',(2.00049737710795,808.645885727578,120.115737376022));
#73014=CARTESIAN_POINT('Ctrl Pts',(2.12237961463586,808.60476778445,120.083969932862));
#73015=CARTESIAN_POINT('Ctrl Pts',(2.17733134395792,808.573117422367,120.065894989075));
#73016=CARTESIAN_POINT('Ctrl Pts',(2.27016201139863,808.490730810805,120.026935329761));
#73017=CARTESIAN_POINT('Ctrl Pts',(2.30724879376502,808.440993570416,120.006466421708));
#73018=CARTESIAN_POINT('Ctrl Pts',(2.35893381692117,808.329470149223,119.965558761407));
#73019=CARTESIAN_POINT('Ctrl Pts',(2.37297690792318,808.268834818019,119.945545079137));
#73020=CARTESIAN_POINT('Ctrl Pts',(2.37600694101095,808.142919188342,119.908165285883));
#73021=CARTESIAN_POINT('Ctrl Pts',(2.36426573934037,808.078918558869,119.891292908726));
#73022=CARTESIAN_POINT('Ctrl Pts',(2.31578907653539,807.957573271305,119.863643618579));
#73023=CARTESIAN_POINT('Ctrl Pts',(2.27941749384543,807.901516396578,119.853188989858));
#73024=CARTESIAN_POINT('Ctrl Pts',(2.18669906391868,807.804831068224,119.840287142195));
#73025=CARTESIAN_POINT('Ctrl Pts',(2.13106711651516,807.765275428406,119.838039605903));
#73026=CARTESIAN_POINT('Ctrl Pts',(2.00788629336271,807.708402984618,119.842281425572));
#73027=CARTESIAN_POINT('Ctrl Pts',(1.94137236530215,807.691785499959,119.848801847912));
#73028=CARTESIAN_POINT('Ctrl Pts',(1.87415121283263,807.688135745084,119.859311375963));
#73029=CARTESIAN_POINT('Origin',(-0.837845221469069,822.333310283414,112.951935752269));
#73030=CARTESIAN_POINT('',(-0.837845221469121,817.643030777277,123.37742842904));
#73031=CARTESIAN_POINT('',(-0.837845221469065,819.445433334314,123.967956837475));
#73032=CARTESIAN_POINT('Ctrl Pts',(-0.837845221469108,817.643030777277,
123.37742842904));
#73033=CARTESIAN_POINT('Ctrl Pts',(-0.838870544337092,817.642971214374,
123.377596955358));
#73034=CARTESIAN_POINT('Ctrl Pts',(-0.839895941276325,817.642913218051,
123.377766040561));
#73035=CARTESIAN_POINT('Ctrl Pts',(-0.965845396659871,817.635982543484,
123.398601934178));
#73036=CARTESIAN_POINT('Ctrl Pts',(-1.08962679456761,817.652486470228,123.427207421591));
#73037=CARTESIAN_POINT('Ctrl Pts',(-1.31856598867587,817.73013409283,123.496171760856));
#73038=CARTESIAN_POINT('Ctrl Pts',(-1.42199791702219,817.789827969577,123.535705754936));
#73039=CARTESIAN_POINT('Ctrl Pts',(-1.5953114515572,817.94447297846,123.620008575917));
#73040=CARTESIAN_POINT('Ctrl Pts',(-1.66405764291828,818.037361986833,123.663868162719));
#73041=CARTESIAN_POINT('Ctrl Pts',(-1.75888850861066,818.245520060921,123.750405240253));
#73042=CARTESIAN_POINT('Ctrl Pts',(-1.78412944892841,818.358527392692,123.792174138513));
#73043=CARTESIAN_POINT('Ctrl Pts',(-1.78756518092656,818.59188252935,123.8686854208));
#73044=CARTESIAN_POINT('Ctrl Pts',(-1.7651451040761,818.709747475906,123.902500385448));
#73045=CARTESIAN_POINT('Ctrl Pts',(-1.67415530367386,818.935425175148,123.95793561471));
#73046=CARTESIAN_POINT('Ctrl Pts',(-1.6056519868477,819.040614710209,123.978729192898));
#73047=CARTESIAN_POINT('Ctrl Pts',(-1.43041868743438,819.223396335037,124.004532279965));
#73048=CARTESIAN_POINT('Ctrl Pts',(-1.3246681546867,819.298638493162,124.008988335719));
#73049=CARTESIAN_POINT('Ctrl Pts',(-1.09143819615308,819.406436680195,124.000862648186));
#73050=CARTESIAN_POINT('Ctrl Pts',(-0.966039878408586,819.438016645367,
123.988356571581));
#73051=CARTESIAN_POINT('Ctrl Pts',(-0.839294955766421,819.445350508609,
123.968187856963));
#73052=CARTESIAN_POINT('Ctrl Pts',(-0.838811713835665,819.44537847052,123.968110959456));
#73053=CARTESIAN_POINT('Ctrl Pts',(-0.838328468930155,819.445406079099,
123.968033952939));
#73054=CARTESIAN_POINT('Ctrl Pts',(-0.837845221469056,819.445433334314,
123.967956837475));
#73055=CARTESIAN_POINT('',(-0.837845221469119,820.112801105241,122.079717220203));
#73056=CARTESIAN_POINT('',(-0.837845221469069,823.227206456033,113.267868905406));
#73057=CARTESIAN_POINT('Ctrl Pts',(-1.77705802490915,819.048233491177,121.858373098143));
#73058=CARTESIAN_POINT('Ctrl Pts',(-1.7932176116289,819.158822517368,121.897459001872));
#73059=CARTESIAN_POINT('Ctrl Pts',(-1.7872537863947,819.272264883798,121.934205595621));
#73060=CARTESIAN_POINT('Ctrl Pts',(-1.73031518108252,819.499265193667,122.001157241267));
#73061=CARTESIAN_POINT('Ctrl Pts',(-1.67743890059782,819.610129981052,122.030195245653));
#73062=CARTESIAN_POINT('Ctrl Pts',(-1.53213732178063,819.806110750292,122.07425566618));
#73063=CARTESIAN_POINT('Ctrl Pts',(-1.44177115614975,819.889798110493,122.089104072595));
#73064=CARTESIAN_POINT('Ctrl Pts',(-1.23289807750473,820.022274822958,122.103691744642));
#73065=CARTESIAN_POINT('Ctrl Pts',(-1.11587204363902,820.069271903309,122.103057009095));
#73066=CARTESIAN_POINT('Ctrl Pts',(-0.870093097674419,820.11876890377,122.085958653446));
#73067=CARTESIAN_POINT('Ctrl Pts',(-0.743487188025589,820.120254744304,
122.069459213704));
#73068=CARTESIAN_POINT('Ctrl Pts',(-0.498759344522085,820.075996069951,
122.022361501746));
#73069=CARTESIAN_POINT('Ctrl Pts',(-0.383014443759105,820.030566631178,
121.99217876904));
#73070=CARTESIAN_POINT('Ctrl Pts',(-0.183064289342193,819.900988850042,
121.923228690827));
#73071=CARTESIAN_POINT('Ctrl Pts',(-0.0995923834267395,819.819753903619,
121.885508837209));
#73072=CARTESIAN_POINT('Ctrl Pts',(0.0272395144654325,819.633381117852,
121.807172160489));
#73073=CARTESIAN_POINT('Ctrl Pts',(0.0706947418430991,819.530794624524,
121.767390772846));
#73074=CARTESIAN_POINT('Ctrl Pts',(0.11538540155723,819.313508374912,121.688989027642));
#73075=CARTESIAN_POINT('Ctrl Pts',(0.115974358696283,819.200739940794,121.651095550297));
#73076=CARTESIAN_POINT('Ctrl Pts',(0.0729773981583475,818.97620989415,121.581190493987));
#73077=CARTESIAN_POINT('Ctrl Pts',(0.0286390196368226,818.866709634554,
121.550035717279));
#73078=CARTESIAN_POINT('Ctrl Pts',(-0.103476020342342,818.662567745945,
121.498451344512));
#73079=CARTESIAN_POINT('Ctrl Pts',(-0.19204288195087,818.571119263489,121.479212143192));
#73080=CARTESIAN_POINT('Ctrl Pts',(-0.397642398028661,818.426796078826,
121.457866553751));
#73081=CARTESIAN_POINT('Ctrl Pts',(-0.512045409772581,818.374455856831,
121.455588986707));
#73082=CARTESIAN_POINT('Ctrl Pts',(-0.755049000647518,818.312960348412,
121.467974698637));
#73083=CARTESIAN_POINT('Ctrl Pts',(-0.881566026361287,818.304984047985,
121.482758670095));
#73084=CARTESIAN_POINT('Ctrl Pts',(-1.12941620842454,818.33611490466,121.52784179555));
#73085=CARTESIAN_POINT('Ctrl Pts',(-1.2483512507509,818.375357598635,121.557850557131));
#73086=CARTESIAN_POINT('Ctrl Pts',(-1.44987844994076,818.490533884236,121.625180557954));
#73087=CARTESIAN_POINT('Ctrl Pts',(-1.53336072539728,818.561314574774,121.660876624497));
#73088=CARTESIAN_POINT('Ctrl Pts',(-1.67198766313081,818.733378143591,121.738343081404));
#73089=CARTESIAN_POINT('Ctrl Pts',(-1.72419610591645,818.834409727487,121.779599475205));
#73090=CARTESIAN_POINT('Ctrl Pts',(-1.76440076878355,818.977560001563,121.833049377407));
#73091=CARTESIAN_POINT('Ctrl Pts',(-1.77186247933987,819.012677487488,121.845806403372));
#73092=CARTESIAN_POINT('Ctrl Pts',(-1.77705802490914,819.048233491177,121.858373098143));
#73093=CARTESIAN_POINT('Ctrl Pts',(-0.837845221469056,819.445433334314,
123.967956837475));
#73094=CARTESIAN_POINT('Ctrl Pts',(-0.837463437055385,819.445454867,123.967895913239));
#73095=CARTESIAN_POINT('Ctrl Pts',(-0.837081651046628,819.44547617913,123.967834921001));
#73096=CARTESIAN_POINT('Ctrl Pts',(-0.711701588183039,819.452402705841,
123.947782575134));
#73097=CARTESIAN_POINT('Ctrl Pts',(-0.587701893295878,819.435596050751,
123.920704421286));
#73098=CARTESIAN_POINT('Ctrl Pts',(-0.357004868804501,819.356342458806,
123.855293316923));
#73099=CARTESIAN_POINT('Ctrl Pts',(-0.252392382180456,819.294998403191,
123.81766184153));
#73100=CARTESIAN_POINT('Ctrl Pts',(-0.0777311002587548,819.136603506486,
123.736692949687));
#73101=CARTESIAN_POINT('Ctrl Pts',(-0.00884603348675146,819.041777621916,
123.69426066563));
#73102=CARTESIAN_POINT('Ctrl Pts',(0.0851971288872298,818.830539716007,
123.609334451121));
#73103=CARTESIAN_POINT('Ctrl Pts',(0.109637015562992,818.716408322916,123.567702195052));
#73104=CARTESIAN_POINT('Ctrl Pts',(0.110828055096987,818.481565818644,123.48987960165));
#73105=CARTESIAN_POINT('Ctrl Pts',(0.0868720204604159,818.363260089305,
123.454600933372));
#73106=CARTESIAN_POINT('Ctrl Pts',(-0.00744562183327744,818.138958151881,
123.395899461776));
#73107=CARTESIAN_POINT('Ctrl Pts',(-0.0772137185211807,818.035418763371,
123.373206376389));
#73108=CARTESIAN_POINT('Ctrl Pts',(-0.253364405911867,817.857499177711,
123.344247496048));
#73109=CARTESIAN_POINT('Ctrl Pts',(-0.358166509108883,817.78501276225,123.338355421415));
#73110=CARTESIAN_POINT('Ctrl Pts',(-0.588913932849431,817.680838923092,
123.344657928148));
#73111=CARTESIAN_POINT('Ctrl Pts',(-0.712830547148864,817.650293111087,
123.356880498781));
#73112=CARTESIAN_POINT('Ctrl Pts',(-0.837845221469107,817.643030777277,
123.37742842904));
#73113=CARTESIAN_POINT('Origin',(-0.837845221469069,822.333310283414,112.951935752269));
#73114=CARTESIAN_POINT('',(-0.837845221469069,820.669893651908,119.158830995758));
#73115=CARTESIAN_POINT('Origin',(-0.837845221469069,820.198471421299,118.992214428491));
#73116=CARTESIAN_POINT('',(-0.837845221469201,819.019888842168,123.827328016679));
#73117=CARTESIAN_POINT('',(-0.837845221469069,822.804732514023,113.118552319537));
#73118=CARTESIAN_POINT('Ctrl Pts',(-0.838127253371057,818.069328309183,
123.515926849969));
#73119=CARTESIAN_POINT('Ctrl Pts',(-0.903386802567897,818.065600594513,
123.52658445066));
#73120=CARTESIAN_POINT('Ctrl Pts',(-0.96810627933474,818.07400570268,123.541253699867));
#73121=CARTESIAN_POINT('Ctrl Pts',(-1.08869639284574,818.114227582888,123.576809526534));
#73122=CARTESIAN_POINT('Ctrl Pts',(-1.14354605159275,818.145532365327,123.59733483987));
#73123=CARTESIAN_POINT('Ctrl Pts',(-1.23565247345017,818.226895746216,123.641286165477));
#73124=CARTESIAN_POINT('Ctrl Pts',(-1.27227772680062,818.275879641158,123.664237576066));
#73125=CARTESIAN_POINT('Ctrl Pts',(-1.32296050700717,818.385686686851,123.709716037981));
#73126=CARTESIAN_POINT('Ctrl Pts',(-1.33658393458632,818.445317087223,123.731769586858));
#73127=CARTESIAN_POINT('Ctrl Pts',(-1.33895116164761,818.568338226321,123.772350546812));
#73128=CARTESIAN_POINT('Ctrl Pts',(-1.32742352957931,818.630432019446,123.790403742977));
#73129=CARTESIAN_POINT('Ctrl Pts',(-1.280059496147,818.749287811661,123.820213657924));
#73130=CARTESIAN_POINT('Ctrl Pts',(-1.24429665331102,818.804689147718,123.831544031392));
#73131=CARTESIAN_POINT('Ctrl Pts',(-1.1522982372719,818.901445669055,123.845948616437));
#73132=CARTESIAN_POINT('Ctrl Pts',(-1.09646639191691,818.941439069988,123.848661302589));
#73133=CARTESIAN_POINT('Ctrl Pts',(-0.973475719350933,818.998700737824,
123.844843178476));
#73134=CARTESIAN_POINT('Ctrl Pts',(-0.907483487113627,819.015558436254,
123.838392636998));
#73135=CARTESIAN_POINT('Ctrl Pts',(-0.774512181601959,819.023842503485,
123.817270075293));
#73136=CARTESIAN_POINT('Ctrl Pts',(-0.708732695548974,819.015384884699,
123.80284825954));
#73137=CARTESIAN_POINT('Ctrl Pts',(-0.58610711490321,818.974148875228,123.767809039508));
#73138=CARTESIAN_POINT('Ctrl Pts',(-0.530390937223295,818.941882381311,
123.747553670573));
#73139=CARTESIAN_POINT('Ctrl Pts',(-0.437826419359151,818.858565377267,
123.704221806289));
#73140=CARTESIAN_POINT('Ctrl Pts',(-0.401422293486539,818.80886555638,123.681659544998));
#73141=CARTESIAN_POINT('Ctrl Pts',(-0.351521899678847,818.697938420887,
123.636653869691));
#73142=CARTESIAN_POINT('Ctrl Pts',(-0.33842366126803,818.637910114495,123.61467090789));
#73143=CARTESIAN_POINT('Ctrl Pts',(-0.337301336556146,818.514783862232,
123.573950724408));
#73144=CARTESIAN_POINT('Ctrl Pts',(-0.349417725435632,818.452959187281,
123.555657405084));
#73145=CARTESIAN_POINT('Ctrl Pts',(-0.39809649811137,818.33437009056,123.524982773105));
#73146=CARTESIAN_POINT('Ctrl Pts',(-0.434792674234262,818.279047346598,
123.513103661662));
#73147=CARTESIAN_POINT('Ctrl Pts',(-0.527792894368055,818.183986419567,
123.498059527713));
#73148=CARTESIAN_POINT('Ctrl Pts',(-0.583239073177139,818.145239825183,
123.495075187514));
#73149=CARTESIAN_POINT('Ctrl Pts',(-0.705660969680285,818.089475828064,
123.498557023331));
#73150=CARTESIAN_POINT('Ctrl Pts',(-0.771587996691071,818.073129122493,
123.505060258999));
#73151=CARTESIAN_POINT('Ctrl Pts',(-0.838127253371057,818.069328309183,
123.515926849969));
#73152=CARTESIAN_POINT('Origin',(2.81945029875316,827.937505831762,114.932648081753));
#73153=CARTESIAN_POINT('',(2.81945029875317,823.353776244448,124.836632500591));
#73154=CARTESIAN_POINT('',(2.81945029874631,825.281064240076,125.513887330513));
#73155=CARTESIAN_POINT('Ctrl Pts',(2.81945029875317,823.353776244448,124.836632500591));
#73156=CARTESIAN_POINT('Ctrl Pts',(2.81791581258216,823.353739939602,124.836735220937));
#73157=CARTESIAN_POINT('Ctrl Pts',(2.81638116540465,823.353706863778,124.836839182085));
#73158=CARTESIAN_POINT('Ctrl Pts',(2.68102309435906,823.351074795614,124.846117234903));
#73159=CARTESIAN_POINT('Ctrl Pts',(2.54862698928472,823.373081668511,124.864568119099));
#73160=CARTESIAN_POINT('Ctrl Pts',(2.30214064245552,823.463765369885,124.917483105267));
#73161=CARTESIAN_POINT('Ctrl Pts',(2.19030299497781,823.531456705398,124.951390993351));
#73162=CARTESIAN_POINT('Ctrl Pts',(2.0021927260165,823.703984684317,125.029550081014));
#73163=CARTESIAN_POINT('Ctrl Pts',(1.92755636539819,823.807038105089,125.073003689809));
#73164=CARTESIAN_POINT('Ctrl Pts',(1.82531689718265,824.035726472811,125.163324160501));
#73165=CARTESIAN_POINT('Ctrl Pts',(1.7986825601708,824.159109076199,125.209294955413));
#73166=CARTESIAN_POINT('Ctrl Pts',(1.79742169351842,824.41077744021,125.297680541177));
#73167=CARTESIAN_POINT('Ctrl Pts',(1.82302350103118,824.536555735892,125.339193287099));
#73168=CARTESIAN_POINT('Ctrl Pts',(1.92397395762404,824.773806701183,125.412468330823));
#73169=CARTESIAN_POINT('Ctrl Pts',(1.99859537327238,824.882831159492,125.443455895961));
#73170=CARTESIAN_POINT('Ctrl Pts',(2.18740493361127,825.068660525225,125.491135776836));
#73171=CARTESIAN_POINT('Ctrl Pts',(2.29987719516671,825.143576314103,125.507343301605));
#73172=CARTESIAN_POINT('Ctrl Pts',(2.54883110033436,825.248869959957,125.523330091962));
#73173=CARTESIAN_POINT('Ctrl Pts',(2.6831123291743,825.277814208441,125.522816861722));
#73174=CARTESIAN_POINT('Ctrl Pts',(2.81878446568712,825.281048573515,125.513931005969));
#73175=CARTESIAN_POINT('Ctrl Pts',(2.8190064133322,825.281053864651,125.513916469493));
#73176=CARTESIAN_POINT('Ctrl Pts',(2.81922835769447,825.281059086836,125.513901911006));
#73177=CARTESIAN_POINT('Ctrl Pts',(2.81945029873946,825.281064240076,125.513887330513));
#73178=CARTESIAN_POINT('',(2.81945029873051,825.919929776281,123.70629147689));
#73179=CARTESIAN_POINT('',(2.81945029875316,828.900534972005,115.27301516482));
#73180=CARTESIAN_POINT('Ctrl Pts',(1.79847410877112,824.901973239337,123.432187801006));
#73181=CARTESIAN_POINT('Ctrl Pts',(1.7946006661164,825.027488491971,123.476549138201));
#73182=CARTESIAN_POINT('Ctrl Pts',(1.81680077872336,825.153207382516,123.518665537769));
#73183=CARTESIAN_POINT('Ctrl Pts',(1.91077766936289,825.390854142231,123.593806318141));
#73184=CARTESIAN_POINT('Ctrl Pts',(1.98163916793723,825.500461320881,123.626102624127));
#73185=CARTESIAN_POINT('Ctrl Pts',(2.16339608076163,825.689276527727,123.676983828598));
#73186=CARTESIAN_POINT('Ctrl Pts',(2.27272037300738,825.766533169006,123.695027106696));
#73187=CARTESIAN_POINT('Ctrl Pts',(2.51592406498725,825.877786076362,123.714582930294));
#73188=CARTESIAN_POINT('Ctrl Pts',(2.64759277928814,825.910530685313,123.715843054018));
#73189=CARTESIAN_POINT('Ctrl Pts',(2.91562752068664,825.926231130019,123.701296297768));
#73190=CARTESIAN_POINT('Ctrl Pts',(3.04943514138652,825.908983050468,123.685611072198));
#73191=CARTESIAN_POINT('Ctrl Pts',(3.29995486441188,825.826602274253,123.639285581525));
#73192=CARTESIAN_POINT('Ctrl Pts',(3.41443100569226,825.762709399156,123.609223431337));
#73193=CARTESIAN_POINT('Ctrl Pts',(3.61129747205381,825.595274583791,123.537641900378));
#73194=CARTESIAN_POINT('Ctrl Pts',(3.6913126252281,825.492896340028,123.496680224497));
#73195=CARTESIAN_POINT('Ctrl Pts',(3.80401457383471,825.26360721659,123.409150793774));
#73196=CARTESIAN_POINT('Ctrl Pts',(3.83550149727127,825.13894658962,123.36344003605));
#73197=CARTESIAN_POINT('Ctrl Pts',(3.84491654647323,824.885567051747,123.273790962698));
#73198=CARTESIAN_POINT('Ctrl Pts',(3.8232804031724,824.75937943419,123.230716732982));
#73199=CARTESIAN_POINT('Ctrl Pts',(3.72990164119277,824.521155563829,123.152701390303));
#73200=CARTESIAN_POINT('Ctrl Pts',(3.65910897033805,824.411431665406,123.118522151007));
#73201=CARTESIAN_POINT('Ctrl Pts',(3.47771174405423,824.223278428048,123.064098490298));
#73202=CARTESIAN_POINT('Ctrl Pts',(3.36899318715402,824.146556973427,123.044341164218));
#73203=CARTESIAN_POINT('Ctrl Pts',(3.12651308768783,824.035463552835,123.022080083715));
#73204=CARTESIAN_POINT('Ctrl Pts',(2.99489911717364,824.002527591301,123.019944326463));
#73205=CARTESIAN_POINT('Ctrl Pts',(2.72542302849062,823.985869682359,123.034188510356));
#73206=CARTESIAN_POINT('Ctrl Pts',(2.59014024058584,824.00289883509,123.050648741545));
#73207=CARTESIAN_POINT('Ctrl Pts',(2.33728496496612,824.085384872656,123.099813743796));
#73208=CARTESIAN_POINT('Ctrl Pts',(2.22194739003479,824.149528293997,123.131864544548));
#73209=CARTESIAN_POINT('Ctrl Pts',(2.02546846648917,824.31683546964,123.207140932675));
#73210=CARTESIAN_POINT('Ctrl Pts',(1.94618592283447,824.418335244401,123.249616443721));
#73211=CARTESIAN_POINT('Ctrl Pts',(1.86229093137326,824.589322608822,123.3169142569));
#73212=CARTESIAN_POINT('Ctrl Pts',(1.8403581759016,824.649281041984,123.339872067749));
#73213=CARTESIAN_POINT('Ctrl Pts',(1.80933002061679,824.773488709707,123.386167183759));
#73214=CARTESIAN_POINT('Ctrl Pts',(1.80046510872344,824.837456765419,123.409385496153));
#73215=CARTESIAN_POINT('Ctrl Pts',(1.79847410877112,824.901973239337,123.432187801006));
#73216=CARTESIAN_POINT('Ctrl Pts',(2.81945029873946,825.281064240076,125.513887330513));
#73217=CARTESIAN_POINT('Ctrl Pts',(2.95018225310641,825.284099699793,125.505298849708));
#73218=CARTESIAN_POINT('Ctrl Pts',(3.07976479896005,825.263206354084,125.489096445404));
#73219=CARTESIAN_POINT('Ctrl Pts',(3.32557482878724,825.174693257163,125.442353930516));
#73220=CARTESIAN_POINT('Ctrl Pts',(3.43897552087231,825.106775536387,125.411909442735));
#73221=CARTESIAN_POINT('Ctrl Pts',(3.63087432886115,824.932435262345,125.340134527275));
#73222=CARTESIAN_POINT('Ctrl Pts',(3.70738943235763,824.827654962982,125.299470901607));
#73223=CARTESIAN_POINT('Ctrl Pts',(3.81274670660058,824.594708319065,125.212386118258));
#73224=CARTESIAN_POINT('Ctrl Pts',(3.84026222369576,824.468742562579,125.166788721991));
#73225=CARTESIAN_POINT('Ctrl Pts',(3.84143550911825,824.213344401118,125.076788028346));
#73226=CARTESIAN_POINT('Ctrl Pts',(3.81510479130032,824.086454994449,125.033280863082));
#73227=CARTESIAN_POINT('Ctrl Pts',(3.71200697474968,823.849606391011,124.954883629206));
#73228=CARTESIAN_POINT('Ctrl Pts',(3.63655326772248,823.741883148951,124.920732856777));
#73229=CARTESIAN_POINT('Ctrl Pts',(3.44641415925407,823.559367339685,124.86698578621));
#73230=CARTESIAN_POINT('Ctrl Pts',(3.3336581971035,823.486322752695,124.847917398616));
#73231=CARTESIAN_POINT('Ctrl Pts',(3.08584832190646,823.384653308201,124.828176827905));
#73232=CARTESIAN_POINT('Ctrl Pts',(2.95326056976095,823.356942099808,124.827675080447));
#73233=CARTESIAN_POINT('Ctrl Pts',(2.81945029875316,823.353776244448,124.836632500591));
#73234=CARTESIAN_POINT('Origin',(2.81945029875316,827.937505831762,114.932648081753));
#73235=CARTESIAN_POINT('',(2.81945029875316,826.274089200256,121.139543325241));
#73236=CARTESIAN_POINT('Origin',(2.81945029875316,825.802666969647,120.972926757974));
#73237=CARTESIAN_POINT('',(2.81945029875316,824.789330259076,125.340496348389));
#73238=CARTESIAN_POINT('',(2.81945029875316,828.408928062371,115.09926464902));
#73239=CARTESIAN_POINT('Ctrl Pts',(2.81917054238824,823.845879038868,125.008980202828));
#73240=CARTESIAN_POINT('Ctrl Pts',(2.7598191810322,823.844516620611,125.012934660588));
#73241=CARTESIAN_POINT('Ctrl Pts',(2.70094339839517,823.853089617159,125.020489900141));
#73242=CARTESIAN_POINT('Ctrl Pts',(2.58398801401168,823.891174230767,125.043139335404));
#73243=CARTESIAN_POINT('Ctrl Pts',(2.5277096780785,823.922373774218,125.058708145184));
#73244=CARTESIAN_POINT('Ctrl Pts',(2.43182055000068,824.003656375447,125.095259561734));
#73245=CARTESIAN_POINT('Ctrl Pts',(2.39306971242166,824.052899522524,125.115870694418));
#73246=CARTESIAN_POINT('Ctrl Pts',(2.33827223814516,824.163183187804,125.15932074624));
#73247=CARTESIAN_POINT('Ctrl Pts',(2.32272841460622,824.223131749996,125.181729914033));
#73248=CARTESIAN_POINT('Ctrl Pts',(2.31709672244318,824.346106118589,125.225392637263));
#73249=CARTESIAN_POINT('Ctrl Pts',(2.32711354998336,824.407918514886,125.246210889237));
#73250=CARTESIAN_POINT('Ctrl Pts',(2.37173535253698,824.525276786811,125.283552464801));
#73251=CARTESIAN_POINT('Ctrl Pts',(2.40599117176568,824.579637174653,125.299692662541));
#73252=CARTESIAN_POINT('Ctrl Pts',(2.49446778498555,824.673421934029,125.32520988367));
#73253=CARTESIAN_POINT('Ctrl Pts',(2.54788723561534,824.711890374459,125.334323055125));
#73254=CARTESIAN_POINT('Ctrl Pts',(2.6679801840789,824.767975352769,125.344458703413));
#73255=CARTESIAN_POINT('Ctrl Pts',(2.7337029073108,824.784607576916,125.345220613515));
#73256=CARTESIAN_POINT('Ctrl Pts',(2.86700413355775,824.792473050555,125.338053006363));
#73257=CARTESIAN_POINT('Ctrl Pts',(2.9332601700801,824.783820174893,125.33025957484));
#73258=CARTESIAN_POINT('Ctrl Pts',(3.05748213479643,824.742442569745,125.307107502219));
#73259=CARTESIAN_POINT('Ctrl Pts',(3.11425445279668,824.710217417341,125.292002850164));
#73260=CARTESIAN_POINT('Ctrl Pts',(3.21080195129426,824.626295632984,125.256235997947));
#73261=CARTESIAN_POINT('Ctrl Pts',(3.24957772756914,824.575404495106,125.235917265404));
#73262=CARTESIAN_POINT('Ctrl Pts',(3.30355477045706,824.461635080464,125.192566698188));
#73263=CARTESIAN_POINT('Ctrl Pts',(3.31812602116394,824.399870523616,125.169961957814));
#73264=CARTESIAN_POINT('Ctrl Pts',(3.32060218684613,824.274098422348,125.12556746162));
#73265=CARTESIAN_POINT('Ctrl Pts',(3.30848418983936,824.211367414805,125.104228235675));
#73266=CARTESIAN_POINT('Ctrl Pts',(3.2590725721864,824.093792349117,125.065925050384));
#73267=CARTESIAN_POINT('Ctrl Pts',(3.22236516342835,824.040103744764,125.049334920485));
#73268=CARTESIAN_POINT('Ctrl Pts',(3.12928000770329,823.948993260361,125.023337325417));
#73269=CARTESIAN_POINT('Ctrl Pts',(3.07386495474634,823.912450896098,125.014181202832));
#73270=CARTESIAN_POINT('Ctrl Pts',(2.95145527750785,823.861359280484,125.004722558184));
#73271=CARTESIAN_POINT('Ctrl Pts',(2.88563042635011,823.84740463419,125.004552118992));
#73272=CARTESIAN_POINT('Ctrl Pts',(2.81917054238824,823.845879038868,125.008980202828));
#73273=CARTESIAN_POINT('Origin',(46.3540028286947,840.779950987597,119.47160273482));
#73274=CARTESIAN_POINT('',(46.3540028286947,838.188382810056,129.981749577168));
#73275=CARTESIAN_POINT('Origin',(46.3540028286947,837.190020390929,129.628894517811));
#73276=CARTESIAN_POINT('',(46.3540028286947,838.854849079124,128.096060654733));
#73277=CARTESIAN_POINT('',(46.3540028286947,841.778313406725,119.824457794176));
#73278=CARTESIAN_POINT('Origin',(46.3540028286947,837.856486659997,127.743205595376));
#73279=CARTESIAN_POINT('Origin',(46.3540028286947,840.779950987597,119.47160273482));
#73280=CARTESIAN_POINT('',(46.3540028286947,839.116534356091,125.678497978308));
#73281=CARTESIAN_POINT('Origin',(46.3540028286947,838.645112125482,125.511881411041));
#73282=CARTESIAN_POINT('',(46.3540028286947,837.661442621538,129.795511085078));
#73283=CARTESIAN_POINT('',(46.3540028286947,841.251373218206,119.638219302087));
#73284=CARTESIAN_POINT('Origin',(46.3540028286947,837.190020390929,129.628894517811));
#73285=CARTESIAN_POINT('Origin',(43.0684041447525,843.225670803329,120.336002870698));
#73286=CARTESIAN_POINT('',(43.0684041447525,840.857509486043,130.92510925662));
#73287=CARTESIAN_POINT('Origin',(43.0684041447525,839.63574020666,130.49329465369));
#73288=CARTESIAN_POINT('',(43.0684041447525,841.523975755111,129.039420334185));
#73289=CARTESIAN_POINT('',(43.0684041447525,844.447440082712,120.767817473629));
#73290=CARTESIAN_POINT('Origin',(43.0684041447525,840.302206475729,128.607605731254));
#73291=CARTESIAN_POINT('Origin',(43.0684041447525,843.225670803329,120.336002870698));
#73292=CARTESIAN_POINT('',(43.0684041447525,841.562254171823,126.542898114187));
#73293=CARTESIAN_POINT('Origin',(43.0684041447525,841.090831941214,126.37628154692));
#73294=CARTESIAN_POINT('',(43.0684041447525,840.107162437269,130.659911220957));
#73295=CARTESIAN_POINT('',(43.0684041447525,843.697093033938,120.502619437965));
#73296=CARTESIAN_POINT('Origin',(43.0684041447525,839.63574020666,130.49329465369));
#73297=CARTESIAN_POINT('Origin',(38.9324005984111,845.429042702751,121.114749052906));
#73298=CARTESIAN_POINT('',(38.9324005984111,843.353828508084,131.807392864075));
#73299=CARTESIAN_POINT('Origin',(38.9324005984111,841.839112106083,131.272040835897));
#73300=CARTESIAN_POINT('',(38.9324005984111,844.020294777152,129.92170394164));
#73301=CARTESIAN_POINT('',(38.9324005984111,846.943759104752,121.650101081084));
#73302=CARTESIAN_POINT('Origin',(38.9324005984111,842.505578375151,129.386351913462));
#73303=CARTESIAN_POINT('Origin',(38.9324005984111,845.429042702751,121.114749052906));
#73304=CARTESIAN_POINT('',(38.9324005984111,843.765626071245,127.321644296395));
#73305=CARTESIAN_POINT('Origin',(38.9324005984111,843.294203840636,127.155027729127));
#73306=CARTESIAN_POINT('',(38.9324005984111,842.310534336692,131.438657403165));
#73307=CARTESIAN_POINT('',(38.9324005984111,845.90046493336,121.281365620173));
#73308=CARTESIAN_POINT('Origin',(38.9324005984111,841.839112106083,131.272040835897));
#73309=CARTESIAN_POINT('Origin',(34.4222031106248,846.708386471252,121.566912428373));
#73310=CARTESIAN_POINT('',(34.4222031106248,844.84206801903,132.333387063086));
#73311=CARTESIAN_POINT('Origin',(34.4222031106248,843.118455874583,131.724204211364));
#73312=CARTESIAN_POINT('',(34.4222031106248,845.508534288098,130.447698140651));
#73313=CARTESIAN_POINT('',(34.4222031106248,848.431998615698,122.176095280095));
#73314=CARTESIAN_POINT('Origin',(34.4222031106248,843.784922143651,129.838515288929));
#73315=CARTESIAN_POINT('Origin',(34.4222031106248,846.708386471252,121.566912428373));
#73316=CARTESIAN_POINT('',(34.4222031106248,845.044969839745,127.773807671861));
#73317=CARTESIAN_POINT('Origin',(34.4222031106248,844.573547609136,127.607191104594));
#73318=CARTESIAN_POINT('',(34.4222031106248,843.589878105192,131.890820778631));
#73319=CARTESIAN_POINT('',(34.4222031106248,847.17980870186,121.73352899564));
#73320=CARTESIAN_POINT('Origin',(34.4222031106248,843.118455874583,131.724204211364));
#73321=CARTESIAN_POINT('Origin',(29.3744893768576,847.525235275903,121.855614434707));
#73322=CARTESIAN_POINT('',(29.3744893768576,845.687504076795,132.632192771945));
#73323=CARTESIAN_POINT('Origin',(29.3744893768576,843.935304679234,132.012906217698));
#73324=CARTESIAN_POINT('',(29.3744893768576,846.353970345864,130.74650384951));
#73325=CARTESIAN_POINT('',(29.3744893768576,849.277434673464,122.474900988954));
#73326=CARTESIAN_POINT('Origin',(29.3744893768576,844.601770948302,130.127217295263));
#73327=CARTESIAN_POINT('Origin',(29.3744893768576,847.525235275903,121.855614434707));
#73328=CARTESIAN_POINT('',(29.3744893768576,845.861818644396,128.062509678195));
#73329=CARTESIAN_POINT('Origin',(29.3744893768576,845.390396413787,127.895893110928));
#73330=CARTESIAN_POINT('',(29.3744893768576,844.406726909843,132.179522784965));
#73331=CARTESIAN_POINT('',(29.3744893768576,847.996657506511,122.022231001974));
#73332=CARTESIAN_POINT('Origin',(29.3744893768576,843.935304679234,132.012906217698));
#73333=CARTESIAN_POINT('Origin',(24.6354177384889,847.105053154204,121.707107855681));
#73334=CARTESIAN_POINT('',(24.6354177384889,845.224364905916,132.46850371825));
#73335=CARTESIAN_POINT('Origin',(24.6354177384889,843.515122557535,131.864399638672));
#73336=CARTESIAN_POINT('',(24.6354177384889,845.890831174984,130.582814795815));
#73337=CARTESIAN_POINT('',(24.6354177384889,848.814295502584,122.311211935259));
#73338=CARTESIAN_POINT('Origin',(24.6354177384889,844.181588826604,129.978710716237));
#73339=CARTESIAN_POINT('Origin',(24.6354177384889,847.105053154204,121.707107855681));
#73340=CARTESIAN_POINT('',(24.6354177384889,845.441636522697,127.914003099169));
#73341=CARTESIAN_POINT('Origin',(24.6354177384889,844.970214292089,127.747386531902));
#73342=CARTESIAN_POINT('',(24.6354177384889,843.986544788144,132.031016205939));
#73343=CARTESIAN_POINT('',(24.6354177384889,847.576475384813,121.873724422948));
#73344=CARTESIAN_POINT('Origin',(24.6354177384889,843.515122557535,131.864399638672));
#73345=CARTESIAN_POINT('Origin',(18.8286901708418,846.180691426412,121.380407144518));
#73346=CARTESIAN_POINT('',(18.8286901708418,844.392975979784,132.174662741008));
#73347=CARTESIAN_POINT('Origin',(18.8286901708418,842.590760829743,131.537698927509));
#73348=CARTESIAN_POINT('',(18.8286901708418,845.059442248852,130.288973818573));
#73349=CARTESIAN_POINT('',(18.8286901708418,847.982906576452,122.017370958017));
#73350=CARTESIAN_POINT('Origin',(18.8286901708418,843.257227098811,129.652010005074));
#73351=CARTESIAN_POINT('Origin',(18.8286901708418,846.180691426412,121.380407144518));
#73352=CARTESIAN_POINT('',(18.8286901708418,844.517274794905,127.587302388006));
#73353=CARTESIAN_POINT('Origin',(18.8286901708418,844.045852564297,127.420685820739));
#73354=CARTESIAN_POINT('',(18.8286901708418,843.062183060352,131.704315494776));
#73355=CARTESIAN_POINT('',(18.8286901708418,846.65211365702,121.547023711785));
#73356=CARTESIAN_POINT('Origin',(18.8286901708418,842.590760829743,131.537698927509));
#73357=CARTESIAN_POINT('Origin',(13.9747365845828,844.218509645117,120.686905710928));
#73358=CARTESIAN_POINT('',(13.9747365845828,842.089677864246,131.360599252937));
#73359=CARTESIAN_POINT('Origin',(13.9747365845828,840.628579048448,130.844197493919));
#73360=CARTESIAN_POINT('',(13.9747365845828,842.756144133314,129.474910330502));
#73361=CARTESIAN_POINT('',(13.9747365845828,845.679608460914,121.203307469945));
#73362=CARTESIAN_POINT('Origin',(13.9747365845828,841.295045317516,128.958508571484));
#73363=CARTESIAN_POINT('Origin',(13.9747365845828,844.218509645117,120.686905710928));
#73364=CARTESIAN_POINT('',(13.9747365845828,842.55509301361,126.893800954416));
#73365=CARTESIAN_POINT('Origin',(13.9747365845828,842.083670783002,126.727184387149));
#73366=CARTESIAN_POINT('',(13.9747365845828,841.100001279057,131.010814061186));
#73367=CARTESIAN_POINT('',(13.9747365845828,844.689931875726,120.853522278195));
#73368=CARTESIAN_POINT('Origin',(13.9747365845828,840.628579048448,130.844197493919));
#73369=CARTESIAN_POINT('Origin',(8.6903868869132,841.260133926098,119.641315632682));
#73370=CARTESIAN_POINT('',(8.6903868869132,838.857584906392,130.218268241032));
#73371=CARTESIAN_POINT('Origin',(8.6903868869132,837.67020332943,129.798607415673));
#73372=CARTESIAN_POINT('',(8.69038687124134,839.520801303739,128.341774453277));
#73373=CARTESIAN_POINT('',(8.6903868869132,842.44751550306,120.060976458041));
#73374=CARTESIAN_POINT('',(9.20983376921269,837.254998443755,127.530619307894));
#73375=CARTESIAN_POINT('Ctrl Pts',(8.69038687123737,839.520801303822,128.341774453042));
#73376=CARTESIAN_POINT('Ctrl Pts',(8.64508445351894,839.520560946243,128.342454515211));
#73377=CARTESIAN_POINT('Ctrl Pts',(8.59973500584719,839.518006330853,128.342347073248));
#73378=CARTESIAN_POINT('Ctrl Pts',(8.3885072590311,839.495195989871,128.338107439068));
#73379=CARTESIAN_POINT('Ctrl Pts',(8.22770820845667,839.446217715886,128.324053706448));
#73380=CARTESIAN_POINT('Ctrl Pts',(7.93598307619641,839.292425840023,128.275673458003));
#73381=CARTESIAN_POINT('Ctrl Pts',(7.80778813258912,839.189374835365,128.241898744099));
#73382=CARTESIAN_POINT('Ctrl Pts',(7.60164840112506,838.943588232457,128.158719926603));
#73383=CARTESIAN_POINT('Ctrl Pts',(7.52535695435235,838.803526026946,128.110226622501));
#73384=CARTESIAN_POINT('Ctrl Pts',(7.47983494279036,838.653883945332,128.057338047592));
#73385=CARTESIAN_POINT('Ctrl Pts',(7.46318547174112,838.599153026814,128.037994289121));
#73386=CARTESIAN_POINT('Ctrl Pts',(7.45073298503272,838.543405825278,128.01815863044));
#73387=CARTESIAN_POINT('Ctrl Pts',(7.42046193279149,838.33440932096,127.943319874755));
#73388=CARTESIAN_POINT('Ctrl Pts',(7.43016974680831,838.179445401286,127.886885132092));
#73389=CARTESIAN_POINT('Ctrl Pts',(7.51195492871686,837.882765369216,127.777376904774));
#73390=CARTESIAN_POINT('Ctrl Pts',(7.58300680585067,837.743796117878,127.725334933141));
#73391=CARTESIAN_POINT('Ctrl Pts',(7.77865108576784,837.498030616829,127.632340063583));
#73392=CARTESIAN_POINT('Ctrl Pts',(7.90188950339133,837.393924069373,127.59240811199));
#73393=CARTESIAN_POINT('Ctrl Pts',(8.17584855348552,837.240817866003,127.532976307217));
#73394=CARTESIAN_POINT('Ctrl Pts',(8.32216264264425,837.190204976988,127.512911156333));
#73395=CARTESIAN_POINT('Ctrl Pts',(8.62483087314532,837.141593624475,127.492538804799));
#73396=CARTESIAN_POINT('Ctrl Pts',(8.77849200804145,837.143199431036,127.492099195355));
#73397=CARTESIAN_POINT('Ctrl Pts',(9.02544731432327,837.188237595322,127.507157956335));
#73398=CARTESIAN_POINT('Ctrl Pts',(9.11997195076001,837.216636446791,127.517060880156));
#73399=CARTESIAN_POINT('Ctrl Pts',(9.20983376921266,837.254998443755,127.530619307894));
#73400=CARTESIAN_POINT('',(9.73894344514155,838.994312472096,128.145351736671));
#73401=CARTESIAN_POINT('Origin',(8.6903868869132,838.336669598498,127.912918493238));
#73402=CARTESIAN_POINT('Ctrl Pts',(9.73894344514147,838.994312472096,128.145351736671));
#73403=CARTESIAN_POINT('Ctrl Pts',(9.65588238431169,839.11204035232,128.186960752964));
#73404=CARTESIAN_POINT('Ctrl Pts',(9.551152040427,839.214779814469,128.22358824077));
#73405=CARTESIAN_POINT('Ctrl Pts',(9.30647723514233,839.381521455656,128.284220003819));
#73406=CARTESIAN_POINT('Ctrl Pts',(9.16812007029517,839.443556967977,128.307536040941));
#73407=CARTESIAN_POINT('Ctrl Pts',(8.91326191066645,839.507943838188,128.333650072219));
#73408=CARTESIAN_POINT('Ctrl Pts',(8.80196701421433,839.521393306068,128.340099455595));
#73409=CARTESIAN_POINT('Ctrl Pts',(8.69038687123737,839.520801303822,128.341774453042));
#73410=CARTESIAN_POINT('Origin',(8.6903868869132,841.260133926098,119.641315632682));
#73411=CARTESIAN_POINT('',(8.6903868869132,839.596717294592,125.84821087617));
#73412=CARTESIAN_POINT('Origin',(8.6903868869132,839.125295063983,125.681594308903));
#73413=CARTESIAN_POINT('',(8.6903868869132,838.141625560039,129.965223982941));
#73414=CARTESIAN_POINT('',(8.6903868869132,841.731556156707,119.807932199949));
#73415=CARTESIAN_POINT('Origin',(8.6903868869132,837.67020332943,129.798607415673));
#73416=CARTESIAN_POINT('Origin',(49.025689001695,841.80813580623,119.834998039228));
#73417=CARTESIAN_POINT('',(49.025689001695,839.216567628689,130.345144881576));
#73418=CARTESIAN_POINT('Origin',(49.025689001695,838.218205209562,129.992289822219));
#73419=CARTESIAN_POINT('',(49.025689001695,839.883033897757,128.45945595914));
#73420=CARTESIAN_POINT('',(49.025689001695,842.806498225357,120.187853098584));
#73421=CARTESIAN_POINT('Origin',(49.025689001695,838.88467147863,128.106600899784));
#73422=CARTESIAN_POINT('Origin',(49.025689001695,841.80813580623,119.834998039228));
#73423=CARTESIAN_POINT('',(49.025689001695,840.144719174724,126.041893282716));
#73424=CARTESIAN_POINT('Origin',(49.025689001695,839.673296944115,125.875276715449));
#73425=CARTESIAN_POINT('',(49.025689001695,838.68962744017,130.158906389486));
#73426=CARTESIAN_POINT('',(49.025689001695,842.279558036839,120.001614606495));
#73427=CARTESIAN_POINT('Origin',(49.025689001695,838.218205209562,129.992289822219));
#73428=CARTESIAN_POINT('Origin',(46.3512073306915,844.844481383473,120.908145303547));
#73429=CARTESIAN_POINT('',(46.3512073306915,842.476320066187,131.497251689469));
#73430=CARTESIAN_POINT('Origin',(46.3512073306915,841.254550786804,131.065437086538));
#73431=CARTESIAN_POINT('',(46.3512073306915,843.142786335256,129.611562767034));
#73432=CARTESIAN_POINT('',(46.3512073306915,846.066250662856,121.339959906477));
#73433=CARTESIAN_POINT('Origin',(46.3512073306915,841.921017055873,129.179748164103));
#73434=CARTESIAN_POINT('Origin',(46.3512073306915,844.844481383473,120.908145303547));
#73435=CARTESIAN_POINT('',(46.3512073306915,843.181064751967,127.115040547035));
#73436=CARTESIAN_POINT('Origin',(46.3512073306915,842.709642521358,126.948423979768));
#73437=CARTESIAN_POINT('',(46.3512073306915,841.725973017413,131.232053653805));
#73438=CARTESIAN_POINT('',(46.3512073306915,845.315903614082,121.074761870814));
#73439=CARTESIAN_POINT('Origin',(46.3512073306915,841.254550786804,131.065437086538));
#73440=CARTESIAN_POINT('Origin',(42.7914627445772,847.810478420552,121.956429013469));
#73441=CARTESIAN_POINT('',(42.7914627445772,845.735264225884,132.649072824638));
#73442=CARTESIAN_POINT('Origin',(42.7914627445772,844.220547823883,132.11372079646));
#73443=CARTESIAN_POINT('',(42.7914627445772,846.401730494952,130.763383902203));
#73444=CARTESIAN_POINT('',(42.7914627445772,849.325194822552,122.491781041647));
#73445=CARTESIAN_POINT('Origin',(42.7914627445772,844.887014092951,130.228031874025));
#73446=CARTESIAN_POINT('Origin',(42.7914627445772,847.810478420552,121.956429013469));
#73447=CARTESIAN_POINT('',(42.7914627445772,846.147061789045,128.163324256957));
#73448=CARTESIAN_POINT('Origin',(42.7914627445772,845.675639558437,127.99670768969));
#73449=CARTESIAN_POINT('',(42.7914627445772,844.691970054492,132.280337363727));
#73450=CARTESIAN_POINT('',(42.7914627445772,848.28190065116,122.123045580736));
#73451=CARTESIAN_POINT('Origin',(42.7914627445772,844.220547823883,132.11372079646));
#73452=CARTESIAN_POINT('Origin',(38.6619388515608,849.945992192791,122.711191837493));
#73453=CARTESIAN_POINT('',(38.6619388515608,848.079673740569,133.477666472207));
#73454=CARTESIAN_POINT('Origin',(38.6619388515608,846.356061596123,132.868483620484));
#73455=CARTESIAN_POINT('',(38.6619388515608,848.746140009638,131.591977549772));
#73456=CARTESIAN_POINT('',(38.6619388515608,851.669604337238,123.320374689216));
#73457=CARTESIAN_POINT('Origin',(38.6619388515608,847.022527865191,130.982794698049));
#73458=CARTESIAN_POINT('Origin',(38.6619388515608,849.945992192791,122.711191837493));
#73459=CARTESIAN_POINT('',(38.6619388515608,848.282575561285,128.918087080981));
#73460=CARTESIAN_POINT('Origin',(38.6619388515608,847.811153330676,128.751470513714));
#73461=CARTESIAN_POINT('',(38.6619388515608,846.827483826731,133.035100187751));
#73462=CARTESIAN_POINT('',(38.6619388515608,850.4174144234,122.87780840476));
#73463=CARTESIAN_POINT('Origin',(38.6619388515608,846.356061596123,132.868483620484));
#73464=CARTESIAN_POINT('Origin',(33.904657486265,851.734486067998,123.343306088194));
#73465=CARTESIAN_POINT('',(33.904657486265,849.896754868891,134.119884425433));
#73466=CARTESIAN_POINT('Origin',(33.904657486265,848.14455547133,133.500597871186));
#73467=CARTESIAN_POINT('',(33.904657486265,850.563221137959,132.234195502998));
#73468=CARTESIAN_POINT('',(33.904657486265,853.48668546556,123.962592642441));
#73469=CARTESIAN_POINT('Origin',(33.904657486265,848.811021740398,131.614908948751));
#73470=CARTESIAN_POINT('Origin',(33.904657486265,851.734486067998,123.343306088194));
#73471=CARTESIAN_POINT('',(33.904657486265,850.071069436492,129.550201331683));
#73472=CARTESIAN_POINT('Origin',(33.904657486265,849.599647205883,129.383584764416));
#73473=CARTESIAN_POINT('',(33.904657486265,848.615977701938,133.667214438453));
#73474=CARTESIAN_POINT('',(33.904657486265,852.205908298607,123.509922655461));
#73475=CARTESIAN_POINT('Origin',(33.904657486265,848.14455547133,133.500597871186));
#73476=CARTESIAN_POINT('Origin',(29.1764893194161,852.252478498716,123.526382139922));
#73477=CARTESIAN_POINT('',(29.1764893194161,850.371790250427,134.287778002492));
#73478=CARTESIAN_POINT('Origin',(29.1764893194161,848.662547902047,133.683673922913));
#73479=CARTESIAN_POINT('',(29.1764893194161,851.038256519496,132.402089080057));
#73480=CARTESIAN_POINT('',(29.1764893194161,853.961720847096,124.1304862195));
#73481=CARTESIAN_POINT('Origin',(29.1764893194161,849.329014171116,131.797985000478));
#73482=CARTESIAN_POINT('Origin',(29.1764893194161,852.252478498716,123.526382139922));
#73483=CARTESIAN_POINT('',(29.1764893194161,850.589061867209,129.73327738341));
#73484=CARTESIAN_POINT('Origin',(29.1764893194161,850.117639636601,129.566660816143));
#73485=CARTESIAN_POINT('',(29.1764893194161,849.133970132656,133.85029049018));
#73486=CARTESIAN_POINT('',(29.1764893194161,852.723900729324,123.692998707189));
#73487=CARTESIAN_POINT('Origin',(29.1764893194161,848.662547902047,133.683673922913));
#73488=CARTESIAN_POINT('Origin',(23.2928167169032,852.486599726132,123.609128503381));
#73489=CARTESIAN_POINT('',(23.2928167169032,850.698884279504,134.40338409987));
#73490=CARTESIAN_POINT('Origin',(23.2928167169032,848.896669129463,133.766420286372));
#73491=CARTESIAN_POINT('',(23.2928167169032,851.365350548572,132.517695177435));
#73492=CARTESIAN_POINT('',(23.2928167169032,854.288814876172,124.246092316879));
#73493=CARTESIAN_POINT('Origin',(23.2928167169032,849.563135398531,131.880731363937));
#73494=CARTESIAN_POINT('Origin',(23.2928167169032,852.486599726132,123.609128503381));
#73495=CARTESIAN_POINT('',(23.2928167169032,850.823183094625,129.816023746869));
#73496=CARTESIAN_POINT('Origin',(23.2928167169032,850.351760864016,129.649407179602));
#73497=CARTESIAN_POINT('',(23.2928167169032,849.368091360072,133.933036853639));
#73498=CARTESIAN_POINT('',(23.2928167169032,852.95802195674,123.775745070648));
#73499=CARTESIAN_POINT('Origin',(23.2928167169032,848.896669129463,133.766420286372));
#73500=CARTESIAN_POINT('Origin',(18.1122424300783,851.518809012321,123.267078519102));
#73501=CARTESIAN_POINT('',(18.1122424300783,849.38997723145,133.940772061111));
#73502=CARTESIAN_POINT('Origin',(18.1122424300783,847.928878415652,133.424370302094));
#73503=CARTESIAN_POINT('',(18.1122424300783,850.056443500518,132.055083138676));
#73504=CARTESIAN_POINT('',(18.1122424300783,852.979907828119,123.78348027812));
#73505=CARTESIAN_POINT('Origin',(18.1122424300783,848.595344684721,131.538681379659));
#73506=CARTESIAN_POINT('Origin',(18.1122424300783,851.518809012321,123.267078519102));
#73507=CARTESIAN_POINT('',(18.1122424300783,849.855392380815,129.473973762591));
#73508=CARTESIAN_POINT('Origin',(18.1122424300783,849.383970150206,129.307357195324));
#73509=CARTESIAN_POINT('',(18.1122424300783,848.400300646261,133.590986869361));
#73510=CARTESIAN_POINT('',(18.1122424300783,851.99023124293,123.43369508637));
#73511=CARTESIAN_POINT('Origin',(18.1122424300783,847.928878415652,133.424370302094));
#73512=CARTESIAN_POINT('Origin',(12.2910011493922,849.660963443569,122.610453033329));
#73513=CARTESIAN_POINT('',(12.2910011493922,847.258414423862,133.187405641679));
#73514=CARTESIAN_POINT('Origin',(12.2910011493922,846.0710328469,132.76774481632));
#73515=CARTESIAN_POINT('',(12.2910011421253,847.920148049266,131.315107184968));
#73516=CARTESIAN_POINT('',(12.2910011493922,850.848345020531,123.030113858687));
#73517=CARTESIAN_POINT('',(12.5605717611635,845.577638737166,130.472121991159));
#73518=CARTESIAN_POINT('Ctrl Pts',(12.2910011348584,847.920148049266,131.315107184968));
#73519=CARTESIAN_POINT('Ctrl Pts',(12.1670963424502,847.919423126756,131.317158264743));
#73520=CARTESIAN_POINT('Ctrl Pts',(12.0436279358354,847.901434025333,131.313177666126));
#73521=CARTESIAN_POINT('Ctrl Pts',(11.7655710010952,847.820082994309,131.289636036821));
#73522=CARTESIAN_POINT('Ctrl Pts',(11.6176364867692,847.744395575652,131.26553254008));
#73523=CARTESIAN_POINT('Ctrl Pts',(11.3620573685532,847.544363900691,131.198525062276));
#73524=CARTESIAN_POINT('Ctrl Pts',(11.2566171401221,847.422310749197,131.156396767216));
#73525=CARTESIAN_POINT('Ctrl Pts',(11.1790915154359,847.284862312556,131.107817839024));
#73526=CARTESIAN_POINT('Ctrl Pts',(11.1507368667833,847.234591164861,131.090050314461));
#73527=CARTESIAN_POINT('Ctrl Pts',(11.1262541876204,847.182504125465,131.071508280925));
#73528=CARTESIAN_POINT('Ctrl Pts',(11.0504903247229,846.984015357416,131.000383314775));
#73529=CARTESIAN_POINT('Ctrl Pts',(11.0256987007203,846.830546197247,130.944476870698));
#73530=CARTESIAN_POINT('Ctrl Pts',(11.0399519067323,846.524349054228,130.831604974351));
#73531=CARTESIAN_POINT('Ctrl Pts',(11.0786035845454,846.374508515622,130.775720721958));
#73532=CARTESIAN_POINT('Ctrl Pts',(11.2153525834717,846.095803855744,130.671084039146));
#73533=CARTESIAN_POINT('Ctrl Pts',(11.3127234995319,845.969835597046,130.62342541909));
#73534=CARTESIAN_POINT('Ctrl Pts',(11.546565107571,845.766407899241,130.546208295514));
#73535=CARTESIAN_POINT('Ctrl Pts',(11.6783701447436,845.688234254163,130.516402240896));
#73536=CARTESIAN_POINT('Ctrl Pts',(11.9634836843023,845.581375523282,130.475443294997));
#73537=CARTESIAN_POINT('Ctrl Pts',(12.1140712809063,845.552831209705,130.464347612941));
#73538=CARTESIAN_POINT('Ctrl Pts',(12.3655020970003,845.548480831299,130.461950791831));
#73539=CARTESIAN_POINT('Ctrl Pts',(12.4642142292712,845.557730509121,130.465085749757));
#73540=CARTESIAN_POINT('Ctrl Pts',(12.5605717611636,845.577638737166,130.47212199116));
#73541=CARTESIAN_POINT('',(13.461664589587,847.175224065062,131.036762701689));
#73542=CARTESIAN_POINT('Origin',(12.291001149392,846.737499115968,130.882055893885));
#73543=CARTESIAN_POINT('Ctrl Pts',(13.4616645895871,847.175224065062,131.036762701689));
#73544=CARTESIAN_POINT('Ctrl Pts',(13.4063794187397,847.306661634346,131.083217185975));
#73545=CARTESIAN_POINT('Ctrl Pts',(13.3266151996975,847.427683944249,131.126306450793));
#73546=CARTESIAN_POINT('Ctrl Pts',(13.1241739751137,847.638733418534,131.202598101252));
#73547=CARTESIAN_POINT('Ctrl Pts',(13.0026163741385,847.726525690388,131.235017448694));
#73548=CARTESIAN_POINT('Ctrl Pts',(12.7273317955889,847.858878443954,131.285730861966));
#73549=CARTESIAN_POINT('Ctrl Pts',(12.5750606879973,847.900659675509,131.303045913372));
#73550=CARTESIAN_POINT('Ctrl Pts',(12.3760093893508,847.918616263365,131.312991804535));
#73551=CARTESIAN_POINT('Ctrl Pts',(12.3334796188194,847.920396575643,131.314404009912));
#73552=CARTESIAN_POINT('Ctrl Pts',(12.2910011348584,847.920148049266,131.315107184968));
#73553=CARTESIAN_POINT('Origin',(12.2910011493922,849.660963443569,122.610453033329));
#73554=CARTESIAN_POINT('',(12.2910011493922,847.997546812062,128.817348276817));
#73555=CARTESIAN_POINT('Origin',(12.2910011493922,847.526124581453,128.65073170955));
#73556=CARTESIAN_POINT('',(12.2910011493922,846.542455077509,132.934361383587));
#73557=CARTESIAN_POINT('',(12.2910011493922,850.132385674177,122.777069600596));
#73558=CARTESIAN_POINT('Origin',(12.2910011493922,846.0710328469,132.76774481632));
#73559=CARTESIAN_POINT('Origin',(51.8657229726398,842.290125991002,120.005349679072));
#73560=CARTESIAN_POINT('',(51.8657229726398,839.69855781346,130.515496521419));
#73561=CARTESIAN_POINT('Origin',(51.8657229726398,838.700195394333,130.162641462063));
#73562=CARTESIAN_POINT('',(51.8657229726398,840.365024082528,128.629807598984));
#73563=CARTESIAN_POINT('',(51.8657229726398,843.288488410129,120.358204738428));
#73564=CARTESIAN_POINT('Origin',(51.8657229726398,839.366661663401,128.276952539628));
#73565=CARTESIAN_POINT('Origin',(51.8657229726398,842.290125991002,120.005349679072));
#73566=CARTESIAN_POINT('',(51.8657229726398,840.626709359495,126.21224492256));
#73567=CARTESIAN_POINT('Origin',(51.8657229726398,840.155287128887,126.045628355293));
#73568=CARTESIAN_POINT('',(51.8657229726398,839.171617624942,130.32925802933));
#73569=CARTESIAN_POINT('',(51.8657229726398,842.76154822161,120.171966246339));
#73570=CARTESIAN_POINT('Origin',(51.8657229726398,838.700195394333,130.162641462063));
#73571=CARTESIAN_POINT('Origin',(49.9192459971847,845.784394458028,121.240342386848));
#73572=CARTESIAN_POINT('',(49.9192459971847,843.416233140742,131.82944877277));
#73573=CARTESIAN_POINT('Origin',(49.9192459971847,842.194463861359,131.397634169839));
#73574=CARTESIAN_POINT('',(49.9192459971847,844.08269940981,129.943759850335));
#73575=CARTESIAN_POINT('',(49.9192459971847,847.006163737411,121.672156989779));
#73576=CARTESIAN_POINT('Origin',(49.9192459971847,842.860930130428,129.511945247404));
#73577=CARTESIAN_POINT('Origin',(49.9192459971847,845.784394458028,121.240342386848));
#73578=CARTESIAN_POINT('',(49.9192459971847,844.120977826522,127.447237630336));
#73579=CARTESIAN_POINT('Origin',(49.9192459971847,843.649555595913,127.280621063069));
#73580=CARTESIAN_POINT('',(49.9192459971847,842.665886091968,131.564250737106));
#73581=CARTESIAN_POINT('',(49.9192459971847,846.255816688637,121.406958954115));
#73582=CARTESIAN_POINT('Origin',(49.9192459971847,842.194463861359,131.397634169839));
#73583=CARTESIAN_POINT('Origin',(47.0913382912604,849.383388329809,122.512348596138));
#73584=CARTESIAN_POINT('',(47.0913382912604,847.308174135141,133.204992407307));
#73585=CARTESIAN_POINT('Origin',(47.0913382912604,845.793457733141,132.669640379129));
#73586=CARTESIAN_POINT('',(47.0913382912604,847.974640404209,131.319303484872));
#73587=CARTESIAN_POINT('',(47.0913382912604,850.89810473181,123.047700624315));
#73588=CARTESIAN_POINT('Origin',(47.0913382912604,846.459924002209,130.783951456694));
#73589=CARTESIAN_POINT('Origin',(47.0913382912604,849.383388329809,122.512348596138));
#73590=CARTESIAN_POINT('',(47.0913382912604,847.719971698303,128.719243839626));
#73591=CARTESIAN_POINT('Origin',(47.0913382912604,847.248549467694,128.552627272359));
#73592=CARTESIAN_POINT('',(47.0913382912604,846.264879963749,132.836256946396));
#73593=CARTESIAN_POINT('',(47.0913382912604,849.854810560418,122.678965163405));
#73594=CARTESIAN_POINT('Origin',(47.0913382912604,845.793457733141,132.669640379129));
#73595=CARTESIAN_POINT('Origin',(43.522968002793,852.281739906609,123.536724111556));
#73596=CARTESIAN_POINT('',(43.522968002793,850.415421454387,134.30319874627));
#73597=CARTESIAN_POINT('Origin',(43.522968002793,848.691809309941,133.694015894547));
#73598=CARTESIAN_POINT('',(43.522968002793,851.081887723456,132.417509823835));
#73599=CARTESIAN_POINT('',(43.522968002793,854.005352051056,124.145906963279));
#73600=CARTESIAN_POINT('Origin',(43.522968002793,849.358275579009,131.808326972112));
#73601=CARTESIAN_POINT('Origin',(43.522968002793,852.281739906609,123.536724111556));
#73602=CARTESIAN_POINT('',(43.522968002793,850.618323275103,129.743619355045));
#73603=CARTESIAN_POINT('Origin',(43.522968002793,850.146901044494,129.577002787777));
#73604=CARTESIAN_POINT('',(43.522968002793,849.16323154055,133.860632461815));
#73605=CARTESIAN_POINT('',(43.522968002793,852.753162137218,123.703340678823));
#73606=CARTESIAN_POINT('Origin',(43.522968002793,848.691809309941,133.694015894547));
#73607=CARTESIAN_POINT('Origin',(39.2640350296006,854.96371308788,124.484624180648));
#73608=CARTESIAN_POINT('',(39.2640350296006,853.125981888773,135.261202517887));
#73609=CARTESIAN_POINT('Origin',(39.2640350296006,851.373782491211,134.64191596364));
#73610=CARTESIAN_POINT('',(39.2640350296006,853.792448157841,133.375513595452));
#73611=CARTESIAN_POINT('',(39.2640350296006,856.715912485441,125.103910734895));
#73612=CARTESIAN_POINT('Origin',(39.2640350296006,852.04024876028,132.756227041205));
#73613=CARTESIAN_POINT('Origin',(39.2640350296006,854.96371308788,124.484624180648));
#73614=CARTESIAN_POINT('',(39.2640350296006,853.300296456374,130.691519424137));
#73615=CARTESIAN_POINT('Origin',(39.2640350296006,852.828874225765,130.52490285687));
#73616=CARTESIAN_POINT('',(39.2640350296006,851.84520472182,134.808532530907));
#73617=CARTESIAN_POINT('',(39.2640350296006,855.435135318489,124.651240747915));
#73618=CARTESIAN_POINT('Origin',(39.2640350296006,851.373782491211,134.64191596364));
#73619=CARTESIAN_POINT('Origin',(29.0499410597756,857.779613277735,125.479858586108));
#73620=CARTESIAN_POINT('',(29.0499410597756,855.991897831107,136.274114182598));
#73621=CARTESIAN_POINT('Origin',(29.0499410597756,854.189682681067,135.637150369099));
#73622=CARTESIAN_POINT('',(29.0499410597756,856.658364100176,134.388425260163));
#73623=CARTESIAN_POINT('',(29.0499410597756,859.581828427776,126.116822399607));
#73624=CARTESIAN_POINT('Origin',(29.0499410597756,854.856148950135,133.751461446664));
#73625=CARTESIAN_POINT('Origin',(29.0499410597756,857.779613277735,125.479858586108));
#73626=CARTESIAN_POINT('',(29.0499410597756,856.116196646229,131.686753829597));
#73627=CARTESIAN_POINT('Origin',(29.0499410597756,855.64477441562,131.520137262329));
#73628=CARTESIAN_POINT('',(29.0499410597756,854.661104911675,135.803766936367));
#73629=CARTESIAN_POINT('',(29.0499410597756,858.251035508344,125.646475153375));
#73630=CARTESIAN_POINT('Origin',(29.0499410597756,854.189682681067,135.637150369099));
#73631=CARTESIAN_POINT('Origin',(23.7691620278726,857.848510729578,125.504209276793));
#73632=CARTESIAN_POINT('',(23.7691620278726,855.719678948707,136.177902818801));
#73633=CARTESIAN_POINT('Origin',(23.7691620278726,854.258580132909,135.661501059784));
#73634=CARTESIAN_POINT('',(23.7691620278726,856.386145217775,134.292213896366));
#73635=CARTESIAN_POINT('',(23.7691620278726,859.309609545375,126.02061103581));
#73636=CARTESIAN_POINT('Origin',(23.7691620278726,854.925046401978,133.775812137349));
#73637=CARTESIAN_POINT('Origin',(23.7691620278726,857.848510729578,125.504209276793));
#73638=CARTESIAN_POINT('',(23.7691620278726,856.185094098072,131.711104520281));
#73639=CARTESIAN_POINT('Origin',(23.7691620278726,855.713671867463,131.544487953014));
#73640=CARTESIAN_POINT('',(23.7691620278726,854.730002363518,135.828117627051));
#73641=CARTESIAN_POINT('',(23.7691620278726,858.319932960187,125.67082584406));
#73642=CARTESIAN_POINT('Origin',(23.7691620278726,854.258580132909,135.661501059784));
#73643=CARTESIAN_POINT('Origin',(17.6654453415508,857.172392077378,125.265246068059));
#73644=CARTESIAN_POINT('',(17.6654453415508,854.769843057671,135.842198676409));
#73645=CARTESIAN_POINT('Origin',(17.6654453415508,853.582461480709,135.42253785105));
#73646=CARTESIAN_POINT('',(17.6654453366203,855.430023704928,133.974294191042));
#73647=CARTESIAN_POINT('',(17.6654453415508,858.35977365434,125.684906893417));
#73648=CARTESIAN_POINT('',(17.6733581535164,853.061569611098,133.117196387139));
#73649=CARTESIAN_POINT('Ctrl Pts',(17.6654453316897,855.430023704928,133.974294191042));
#73650=CARTESIAN_POINT('Ctrl Pts',(17.6295073639708,855.42981443297,133.974886300904));
#73651=CARTESIAN_POINT('Ctrl Pts',(17.59352668523,855.428157015281,133.974959520969));
#73652=CARTESIAN_POINT('Ctrl Pts',(17.3919526744461,855.410682439271,133.972410715024));
#73653=CARTESIAN_POINT('Ctrl Pts',(17.2307440375472,855.365630162799,133.959134714097));
#73654=CARTESIAN_POINT('Ctrl Pts',(16.9368955664509,855.220045084026,133.911370505633));
#73655=CARTESIAN_POINT('Ctrl Pts',(16.8069148003019,855.121321434135,133.877487645813));
#73656=CARTESIAN_POINT('Ctrl Pts',(16.7007738042995,855.002073798701,133.835341496605));
#73657=CARTESIAN_POINT('Ctrl Pts',(16.6619532122509,854.958459512211,133.819926732034));
#73658=CARTESIAN_POINT('Ctrl Pts',(16.6265103511939,854.912310910842,133.803483543428));
#73659=CARTESIAN_POINT('Ctrl Pts',(16.5085649220031,854.733018142063,133.739143092934));
#73660=CARTESIAN_POINT('Ctrl Pts',(16.4503573729137,854.587773946474,133.686143629637));
#73661=CARTESIAN_POINT('Ctrl Pts',(16.3964556695319,854.285505848461,133.574660390738));
#73662=CARTESIAN_POINT('Ctrl Pts',(16.4010178842328,854.131382945078,133.517262605736));
#73663=CARTESIAN_POINT('Ctrl Pts',(16.4728950147202,853.832004072906,133.405318956769));
#73664=CARTESIAN_POINT('Ctrl Pts',(16.5401428529477,853.689722598392,133.351894694273));
#73665=CARTESIAN_POINT('Ctrl Pts',(16.7236470185644,853.444937208962,133.260060363104));
#73666=CARTESIAN_POINT('Ctrl Pts',(16.8351824911558,853.342649262511,133.221731498453));
#73667=CARTESIAN_POINT('Ctrl Pts',(17.0902805099667,853.182257215964,133.161852067453));
#73668=CARTESIAN_POINT('Ctrl Pts',(17.2312131677073,853.124824135463,133.14054611769));
#73669=CARTESIAN_POINT('Ctrl Pts',(17.4761307604511,853.071287145555,133.120765083804));
#73670=CARTESIAN_POINT('Ctrl Pts',(17.5747161947025,853.060985237067,133.116989849583));
#73671=CARTESIAN_POINT('Ctrl Pts',(17.6733581535165,853.061569611098,133.117196387139));
#73672=CARTESIAN_POINT('',(18.9070520539092,854.447604093656,133.607067870924));
#73673=CARTESIAN_POINT('Origin',(17.6654453415506,854.248927749778,133.536848928615));
#73674=CARTESIAN_POINT('Ctrl Pts',(18.9070520539092,854.447604093656,133.607067870924));
#73675=CARTESIAN_POINT('Ctrl Pts',(18.8819590002978,854.587006899514,133.656337539326));
#73676=CARTESIAN_POINT('Ctrl Pts',(18.8306469852216,854.72101846392,133.704017646188));
#73677=CARTESIAN_POINT('Ctrl Pts',(18.6792869942737,854.967128558182,133.792700906052));
#73678=CARTESIAN_POINT('Ctrl Pts',(18.5798416076307,855.07682155118,133.832860709377));
#73679=CARTESIAN_POINT('Ctrl Pts',(18.3400311349627,855.260218651258,133.901614921833));
#73680=CARTESIAN_POINT('Ctrl Pts',(18.2004774636254,855.330918827193,133.929150906681));
#73681=CARTESIAN_POINT('Ctrl Pts',(17.9259064740675,855.412441796172,133.963152002444));
#73682=CARTESIAN_POINT('Ctrl Pts',(17.795957526262,855.43078369622,133.972143886994));
#73683=CARTESIAN_POINT('Ctrl Pts',(17.6654453316897,855.430023704928,133.974294191042));
#73684=CARTESIAN_POINT('Origin',(17.6654453415508,857.172392077378,125.265246068059));
#73685=CARTESIAN_POINT('',(17.6654453415508,855.508975445871,131.472141311547));
#73686=CARTESIAN_POINT('Origin',(17.6654453415508,855.037553215263,131.30552474428));
#73687=CARTESIAN_POINT('',(17.6654453415508,854.053883711318,135.589154418317));
#73688=CARTESIAN_POINT('',(17.6654453415508,857.643814307987,125.431862635326));
#73689=CARTESIAN_POINT('Origin',(17.6654453415508,853.582461480709,135.42253785105));
#73690=CARTESIAN_POINT('Origin',(54.7499816290036,842.204856257991,119.975212470252));
#73691=CARTESIAN_POINT('',(54.7499816290036,839.61328808045,130.4853593126));
#73692=CARTESIAN_POINT('Origin',(54.7499816290036,838.614925661323,130.132504253244));
#73693=CARTESIAN_POINT('',(54.7499816290036,840.279754349518,128.599670390165));
#73694=CARTESIAN_POINT('',(54.7499816290036,843.203218677118,120.328067529609));
#73695=CARTESIAN_POINT('Origin',(54.7499816290036,839.281391930391,128.246815330808));
#73696=CARTESIAN_POINT('Origin',(54.7499816290036,842.204856257991,119.975212470252));
#73697=CARTESIAN_POINT('',(54.7499816290036,840.541439626485,126.182107713741));
#73698=CARTESIAN_POINT('Origin',(54.7499816290036,840.070017395876,126.015491146474));
#73699=CARTESIAN_POINT('',(54.7499816290036,839.086347891931,130.299120820511));
#73700=CARTESIAN_POINT('',(54.7499816290036,842.6762784886,120.141829037519));
#73701=CARTESIAN_POINT('Origin',(54.7499816290036,838.614925661323,130.132504253244));
#73702=CARTESIAN_POINT('Origin',(53.6165797331573,846.004331315431,121.318075514004));
#73703=CARTESIAN_POINT('',(53.6165797331573,843.636169998145,131.907181899926));
#73704=CARTESIAN_POINT('Origin',(53.6165797331573,842.414400718763,131.475367296995));
#73705=CARTESIAN_POINT('',(53.6165797331573,844.302636267214,130.021492977491));
#73706=CARTESIAN_POINT('',(53.6165797331573,847.226100594814,121.749890116935));
#73707=CARTESIAN_POINT('Origin',(53.6165797331573,843.080866987831,129.58967837456));
#73708=CARTESIAN_POINT('Origin',(53.6165797331573,846.004331315431,121.318075514004));
#73709=CARTESIAN_POINT('',(53.6165797331573,844.340914683925,127.524970757492));
#73710=CARTESIAN_POINT('Origin',(53.6165797331573,843.869492453316,127.358354190225));
#73711=CARTESIAN_POINT('',(53.6165797331573,842.885822949371,131.641983864262));
#73712=CARTESIAN_POINT('',(53.6165797331573,846.47575354604,121.484692081271));
#73713=CARTESIAN_POINT('Origin',(53.6165797331573,842.414400718763,131.475367296995));
#73714=CARTESIAN_POINT('Origin',(51.6441020439785,850.07902871983,122.758211447552));
#73715=CARTESIAN_POINT('',(51.6441020439785,848.003814525162,133.450855258721));
#73716=CARTESIAN_POINT('Origin',(51.6441020439785,846.489098123162,132.915503230543));
#73717=CARTESIAN_POINT('',(51.6441020439785,848.67028079423,131.565166336286));
#73718=CARTESIAN_POINT('',(51.6441020439785,851.593745121831,123.29356347573));
#73719=CARTESIAN_POINT('Origin',(51.6441020439785,847.15556439223,131.029814308108));
#73720=CARTESIAN_POINT('Origin',(51.6441020439785,850.07902871983,122.758211447552));
#73721=CARTESIAN_POINT('',(51.6441020439785,848.415612088324,128.96510669104));
#73722=CARTESIAN_POINT('Origin',(51.6441020439785,847.944189857715,128.798490123773));
#73723=CARTESIAN_POINT('',(51.6441020439785,846.96052035377,133.08211979781));
#73724=CARTESIAN_POINT('',(51.6441020439785,850.550450950439,122.924828014819));
#73725=CARTESIAN_POINT('Origin',(51.6441020439785,846.489098123162,132.915503230543));
#73726=CARTESIAN_POINT('Origin',(48.7928402646065,853.613546229451,124.007429528842));
#73727=CARTESIAN_POINT('',(48.7928402646065,851.747227777229,134.773904163556));
#73728=CARTESIAN_POINT('Origin',(48.7928402646065,850.023615632782,134.164721311833));
#73729=CARTESIAN_POINT('',(48.7928402646065,852.413694046297,132.88821524112));
#73730=CARTESIAN_POINT('',(48.7928402646065,855.337158373898,124.616612380564));
#73731=CARTESIAN_POINT('Origin',(48.7928402646065,850.690081901851,132.279032389398));
#73732=CARTESIAN_POINT('Origin',(48.7928402646065,853.613546229451,124.007429528842));
#73733=CARTESIAN_POINT('',(48.7928402646065,851.950129597945,130.21432477233));
#73734=CARTESIAN_POINT('Origin',(48.7928402646065,851.478707367336,130.047708205063));
#73735=CARTESIAN_POINT('',(48.7928402646065,850.495037863391,134.3313378791));
#73736=CARTESIAN_POINT('',(48.7928402646065,854.08496846006,124.174046096109));
#73737=CARTESIAN_POINT('Origin',(48.7928402646065,850.023615632782,134.164721311833));
#73738=CARTESIAN_POINT('Origin',(45.2183914910739,857.071783619228,125.229687634777));
#73739=CARTESIAN_POINT('',(45.2183914910739,855.234052420121,136.006265972015));
#73740=CARTESIAN_POINT('Origin',(45.2183914910739,853.48185302256,135.386979417768));
#73741=CARTESIAN_POINT('',(45.2183914910739,855.900518689189,134.12057704958));
#73742=CARTESIAN_POINT('',(45.2183914910739,858.82398301679,125.848974189024));
#73743=CARTESIAN_POINT('Origin',(45.2183914910739,854.148319291628,133.501290495333));
#73744=CARTESIAN_POINT('Origin',(45.2183914910739,857.071783619228,125.229687634777));
#73745=CARTESIAN_POINT('',(45.2183914910739,855.408366987722,131.436582878265));
#73746=CARTESIAN_POINT('Origin',(45.2183914910739,854.936944757113,131.269966310998));
#73747=CARTESIAN_POINT('',(45.2183914910739,853.953275253168,135.553595985035));
#73748=CARTESIAN_POINT('',(45.2183914910739,857.543205849837,125.396304202044));
#73749=CARTESIAN_POINT('Origin',(45.2183914910739,853.48185302256,135.386979417768));
#73750=CARTESIAN_POINT('Origin',(41.1224533261868,859.358195582718,126.037782985357));
#73751=CARTESIAN_POINT('',(41.1224533261868,857.47750733443,136.799178847926));
#73752=CARTESIAN_POINT('Origin',(41.1224533261868,855.76826498605,136.195074768348));
#73753=CARTESIAN_POINT('',(41.1224533261868,858.143973603498,134.913489925491));
#73754=CARTESIAN_POINT('',(41.1224533261868,861.067437931099,126.641887064935));
#73755=CARTESIAN_POINT('Origin',(41.1224533261868,856.434731255118,134.309385845913));
#73756=CARTESIAN_POINT('Origin',(41.1224533261868,859.358195582718,126.037782985357));
#73757=CARTESIAN_POINT('',(41.1224533261868,857.694778951212,132.244678228845));
#73758=CARTESIAN_POINT('Origin',(41.1224533261868,857.223356720603,132.078061661578));
#73759=CARTESIAN_POINT('',(41.1224533261868,856.239687216658,136.361691335615));
#73760=CARTESIAN_POINT('',(41.1224533261868,859.829617813327,126.204399552624));
#73761=CARTESIAN_POINT('Origin',(41.1224533261868,855.76826498605,136.195074768348));
#73762=CARTESIAN_POINT('Origin',(35.8484492399277,861.828401990321,126.910837511327));
#73763=CARTESIAN_POINT('',(35.8484492399277,860.040686543693,137.705093107816));
#73764=CARTESIAN_POINT('Origin',(35.8484492399277,858.238471393652,137.068129294318));
#73765=CARTESIAN_POINT('',(35.8484492399277,860.707152812761,135.819404185381));
#73766=CARTESIAN_POINT('',(35.8484492399277,863.630617140361,127.547801324825));
#73767=CARTESIAN_POINT('Origin',(35.8484492399277,858.90493766272,135.182440371883));
#73768=CARTESIAN_POINT('Origin',(35.8484492399277,861.828401990321,126.910837511327));
#73769=CARTESIAN_POINT('',(35.8484492399277,860.164985358814,133.117732754815));
#73770=CARTESIAN_POINT('Origin',(35.8484492399277,859.693563128206,132.951116187548));
#73771=CARTESIAN_POINT('',(35.8484492399277,858.709893624261,137.234745861585));
#73772=CARTESIAN_POINT('',(35.8484492399277,862.299824220929,127.077454078594));
#73773=CARTESIAN_POINT('Origin',(35.8484492399277,858.238471393652,137.068129294318));
#73774=CARTESIAN_POINT('Origin',(30.69826084663,862.930976458564,127.300524634944));
#73775=CARTESIAN_POINT('',(30.69826084663,860.802144677693,137.974218176952));
#73776=CARTESIAN_POINT('Origin',(30.69826084663,859.341045861896,137.457816417935));
#73777=CARTESIAN_POINT('',(30.69826084663,861.468610946762,136.088529254517));
#73778=CARTESIAN_POINT('',(30.69826084663,864.392075274362,127.816926393961));
#73779=CARTESIAN_POINT('Origin',(30.69826084663,860.007512130964,135.5721274955));
#73780=CARTESIAN_POINT('Origin',(30.69826084663,862.930976458564,127.300524634944));
#73781=CARTESIAN_POINT('',(30.69826084663,861.267559827058,133.507419878432));
#73782=CARTESIAN_POINT('Origin',(30.69826084663,860.796137596449,133.340803311165));
#73783=CARTESIAN_POINT('',(30.69826084663,859.812468092504,137.624432985202));
#73784=CARTESIAN_POINT('',(30.69826084663,863.402398689173,127.467141202211));
#73785=CARTESIAN_POINT('Origin',(30.69826084663,859.341045861896,137.457816417935));
#73786=CARTESIAN_POINT('Origin',(24.5788304627471,863.466134352395,127.489667542144));
#73787=CARTESIAN_POINT('',(24.5788304627471,861.063585332689,138.066620150493));
#73788=CARTESIAN_POINT('Origin',(24.5788304627471,859.876203755726,137.646959325135));
#73789=CARTESIAN_POINT('',(24.5788304719421,861.72230180781,136.202858370173));
#73790=CARTESIAN_POINT('',(24.5788304627471,864.653515929357,127.909328367502));
#73791=CARTESIAN_POINT('',(24.3247396470537,859.379707374474,135.350240052251));
#73792=CARTESIAN_POINT('Ctrl Pts',(24.5788304811371,861.72230180781,136.202858370173));
#73793=CARTESIAN_POINT('Ctrl Pts',(24.4650951106064,861.721713023236,136.204524272744));
#73794=CARTESIAN_POINT('Ctrl Pts',(24.3516351742477,861.706668449823,136.200851948056));
#73795=CARTESIAN_POINT('Ctrl Pts',(24.0825158145281,861.635167682745,136.17869189312));
#73796=CARTESIAN_POINT('Ctrl Pts',(23.9336752938585,861.564074370878,136.154574529653));
#73797=CARTESIAN_POINT('Ctrl Pts',(23.8035577973859,861.46823923053,136.120703148391));
#73798=CARTESIAN_POINT('Ctrl Pts',(23.7559679080946,861.433187958849,136.10831484299));
#73799=CARTESIAN_POINT('Ctrl Pts',(23.7111138882448,861.394996533156,136.094683989506));
#73800=CARTESIAN_POINT('Ctrl Pts',(23.5561416739836,861.242749069374,136.039902264898));
#73801=CARTESIAN_POINT('Ctrl Pts',(23.4670621490132,861.11210057302,135.992061415569));
#73802=CARTESIAN_POINT('Ctrl Pts',(23.3473612993245,860.827035957846,135.8866584696));
#73803=CARTESIAN_POINT('Ctrl Pts',(23.3176346602385,860.67540677207,135.830142048776));
#73804=CARTESIAN_POINT('Ctrl Pts',(23.3214985467804,860.368522196417,135.715545630238));
#73805=CARTESIAN_POINT('Ctrl Pts',(23.3556842539537,860.216188967325,135.658568737564));
#73806=CARTESIAN_POINT('Ctrl Pts',(23.4808309645594,859.940817218659,135.555924152126));
#73807=CARTESIAN_POINT('Ctrl Pts',(23.5672222372109,859.81891533621,135.510663058839));
#73808=CARTESIAN_POINT('Ctrl Pts',(23.7811557277566,859.612043699473,135.43435616799));
#73809=CARTESIAN_POINT('Ctrl Pts',(23.9062740132204,859.528245783003,135.403731993118));
#73810=CARTESIAN_POINT('Ctrl Pts',(24.1339743085658,859.427873803726,135.367397889288));
#73811=CARTESIAN_POINT('Ctrl Pts',(24.2281243882554,859.398472394407,135.356872245226));
#73812=CARTESIAN_POINT('Ctrl Pts',(24.3247396470539,859.379707374475,135.350240052252));
#73813=CARTESIAN_POINT('',(25.8371162760489,860.493614653875,135.743932574787));
#73814=CARTESIAN_POINT('Origin',(24.5788304627464,860.542670024794,135.7612704027));
#73815=CARTESIAN_POINT('Ctrl Pts',(25.8371162760488,860.493614653875,135.743932574787));
#73816=CARTESIAN_POINT('Ctrl Pts',(25.8433120265261,860.634890124764,135.793864106374));
#73817=CARTESIAN_POINT('Ctrl Pts',(25.8226947966971,860.776029657672,135.844063478485));
#73818=CARTESIAN_POINT('Ctrl Pts',(25.7290311972954,861.046420841452,135.941328496956));
#73819=CARTESIAN_POINT('Ctrl Pts',(25.6560442655738,861.173201350605,135.987527606661));
#73820=CARTESIAN_POINT('Ctrl Pts',(25.4621887671792,861.399573424031,136.071470628793));
#73821=CARTESIAN_POINT('Ctrl Pts',(25.3414516971849,861.496067617522,136.108123092207));
#73822=CARTESIAN_POINT('Ctrl Pts',(25.0599300905018,861.646292595752,136.167054480677));
#73823=CARTESIAN_POINT('Ctrl Pts',(24.8999449549518,861.695586151695,136.187733337864));
#73824=CARTESIAN_POINT('Ctrl Pts',(24.6825627254731,861.719835765023,136.200231380237));
#73825=CARTESIAN_POINT('Ctrl Pts',(24.6306679924485,861.722570159924,136.202099096756));
#73826=CARTESIAN_POINT('Ctrl Pts',(24.5788304811371,861.72230180781,136.202858370173));
#73827=CARTESIAN_POINT('Origin',(24.5788304627471,863.466134352395,127.489667542144));
#73828=CARTESIAN_POINT('',(24.5788304627471,861.802717720889,133.696562785632));
#73829=CARTESIAN_POINT('Origin',(24.5788304627471,861.33129549028,133.529946218365));
#73830=CARTESIAN_POINT('',(24.5788304627471,860.347625986335,137.813575892402));
#73831=CARTESIAN_POINT('',(24.5788304627471,863.937556583004,127.656284109411));
#73832=CARTESIAN_POINT('Origin',(24.5788304627471,859.876203755726,137.646959325135));
#73833=CARTESIAN_POINT('Origin',(57.5524090272951,841.556053303701,119.74590355341));
#73834=CARTESIAN_POINT('',(57.5524090272951,838.96448512616,130.256050395757));
#73835=CARTESIAN_POINT('Origin',(57.5524090272951,837.966122707033,129.903195336401));
#73836=CARTESIAN_POINT('',(57.5524090272951,839.630951395229,128.370361473322));
#73837=CARTESIAN_POINT('',(57.5524090272951,842.554415722829,120.098758612766));
#73838=CARTESIAN_POINT('Origin',(57.5524090272951,838.632588976101,128.017506413966));
#73839=CARTESIAN_POINT('Origin',(57.5524090272951,841.556053303701,119.74590355341));
#73840=CARTESIAN_POINT('',(57.5524090272951,839.892636672195,125.952798796898));
#73841=CARTESIAN_POINT('Origin',(57.5524090272951,839.421214441586,125.786182229631));
#73842=CARTESIAN_POINT('',(57.5524090272951,838.437544937642,130.069811903668));
#73843=CARTESIAN_POINT('',(57.5524090272951,842.02747553431,119.912520120677));
#73844=CARTESIAN_POINT('Origin',(57.5524090272951,837.966122707033,129.903195336401));
#73845=CARTESIAN_POINT('Origin',(57.2816173125715,845.494679659641,121.137947374353));
#73846=CARTESIAN_POINT('',(57.2816173125715,843.126518342356,131.727053760275));
#73847=CARTESIAN_POINT('Origin',(57.2816173125715,841.904749062973,131.295239157344));
#73848=CARTESIAN_POINT('',(57.2816173125715,843.792984611424,129.84136483784));
#73849=CARTESIAN_POINT('',(57.2816173125715,846.716448939024,121.569761977284));
#73850=CARTESIAN_POINT('Origin',(57.2816173125715,842.571215332041,129.409550234909));
#73851=CARTESIAN_POINT('Origin',(57.2816173125715,845.494679659641,121.137947374353));
#73852=CARTESIAN_POINT('',(57.2816173125715,843.831263028135,127.344842617841));
#73853=CARTESIAN_POINT('Origin',(57.2816173125715,843.359840797526,127.178226050574));
#73854=CARTESIAN_POINT('',(57.2816173125715,842.376171293582,131.461855724611));
#73855=CARTESIAN_POINT('',(57.2816173125715,845.96610189025,121.30456394162));
#73856=CARTESIAN_POINT('Origin',(57.2816173125715,841.904749062973,131.295239157344));
#73857=CARTESIAN_POINT('Origin',(56.2507763801536,849.866996767518,122.683272181324));
#73858=CARTESIAN_POINT('',(56.2507763801536,847.79178257285,133.375915992493));
#73859=CARTESIAN_POINT('Origin',(56.2507763801536,846.277066170849,132.840563964316));
#73860=CARTESIAN_POINT('',(56.2507763801536,848.458248841918,131.490227070058));
#73861=CARTESIAN_POINT('',(56.2507763801536,851.381713169518,123.218624209502));
#73862=CARTESIAN_POINT('Origin',(56.2507763801536,846.943532439917,130.95487504188));
#73863=CARTESIAN_POINT('Origin',(56.2507763801536,849.866996767518,122.683272181324));
#73864=CARTESIAN_POINT('',(56.2507763801536,848.203580136011,128.890167424813));
#73865=CARTESIAN_POINT('Origin',(56.2507763801536,847.732157905402,128.723550857546));
#73866=CARTESIAN_POINT('',(56.2507763801536,846.748488401458,133.007180531583));
#73867=CARTESIAN_POINT('',(56.2507763801536,850.338418998126,122.849888748591));
#73868=CARTESIAN_POINT('Origin',(56.2507763801536,846.277066170849,132.840563964316));
#73869=CARTESIAN_POINT('Origin',(54.2412369315076,853.883204834292,124.10273600392));
#73870=CARTESIAN_POINT('',(54.2412369315076,852.01688638207,134.869210638633));
#73871=CARTESIAN_POINT('Origin',(54.2412369315076,850.293274237623,134.260027786911));
#73872=CARTESIAN_POINT('',(54.2412369315076,852.683352651138,132.983521716198));
#73873=CARTESIAN_POINT('',(54.2412369315076,855.606816978739,124.711918855642));
#73874=CARTESIAN_POINT('Origin',(54.2412369315076,850.959740506692,132.374338864476));
#73875=CARTESIAN_POINT('Origin',(54.2412369315076,853.883204834292,124.10273600392));
#73876=CARTESIAN_POINT('',(54.2412369315076,852.219788202786,130.309631247408));
#73877=CARTESIAN_POINT('Origin',(54.2412369315076,851.748365972177,130.143014680141));
#73878=CARTESIAN_POINT('',(54.2412369315076,850.764696468232,134.426644354178));
#73879=CARTESIAN_POINT('',(54.2412369315076,854.354627064901,124.269352571187));
#73880=CARTESIAN_POINT('Origin',(54.2412369315076,850.293274237623,134.260027786911));
#73881=CARTESIAN_POINT('Origin',(51.5074929211464,857.966564864178,125.545933602422));
#73882=CARTESIAN_POINT('',(51.5074929211464,856.128833665071,136.32251193966));
#73883=CARTESIAN_POINT('Origin',(51.5074929211464,854.37663426751,135.703225385413));
#73884=CARTESIAN_POINT('',(51.5074929211464,856.795299934139,134.436823017225));
#73885=CARTESIAN_POINT('',(51.5074929211464,859.71876426174,126.165220156669));
#73886=CARTESIAN_POINT('Origin',(51.5074929211464,855.043100536578,133.817536462978));
#73887=CARTESIAN_POINT('Origin',(51.5074929211464,857.966564864178,125.545933602422));
#73888=CARTESIAN_POINT('',(51.5074929211464,856.303148232672,131.75282884591));
#73889=CARTESIAN_POINT('Origin',(51.5074929211464,855.831726002063,131.586212278643));
#73890=CARTESIAN_POINT('',(51.5074929211464,854.848056498118,135.869841952681));
#73891=CARTESIAN_POINT('',(51.5074929211464,858.437987094787,125.712550169689));
#73892=CARTESIAN_POINT('Origin',(51.5074929211464,854.37663426751,135.703225385413));
#73893=CARTESIAN_POINT('Origin',(48.0052498018394,861.005933388624,126.620149278566));
#73894=CARTESIAN_POINT('',(48.0052498018394,859.125245140336,137.381545141136));
#73895=CARTESIAN_POINT('Origin',(48.0052498018394,857.416002791956,136.777441061558));
#73896=CARTESIAN_POINT('',(48.0052498018394,859.791711409404,135.495856218701));
#73897=CARTESIAN_POINT('',(48.0052498018394,862.715175737005,127.224253358145));
#73898=CARTESIAN_POINT('Origin',(48.0052498018394,858.082469061024,134.891752139123));
#73899=CARTESIAN_POINT('Origin',(48.0052498018394,861.005933388624,126.620149278566));
#73900=CARTESIAN_POINT('',(48.0052498018394,859.342516757118,132.827044522055));
#73901=CARTESIAN_POINT('Origin',(48.0052498018394,858.871094526509,132.660427954788));
#73902=CARTESIAN_POINT('',(48.0052498018394,857.887425022564,136.944057628825));
#73903=CARTESIAN_POINT('',(48.0052498018394,861.477355619233,126.786765845834));
#73904=CARTESIAN_POINT('Origin',(48.0052498018394,857.416002791956,136.777441061558));
#73905=CARTESIAN_POINT('Origin',(43.3912138270256,864.456014368904,127.839524633406));
#73906=CARTESIAN_POINT('',(43.3912138270256,862.668298922276,138.633780229895));
#73907=CARTESIAN_POINT('Origin',(43.3912138270256,860.866083772235,137.996816416397));
#73908=CARTESIAN_POINT('',(43.3912138270256,863.334765191344,136.74809130746));
#73909=CARTESIAN_POINT('',(43.3912138270256,866.258229518945,128.476488446904));
#73910=CARTESIAN_POINT('Origin',(43.3912138270256,861.532550041304,136.111127493962));
#73911=CARTESIAN_POINT('Origin',(43.3912138270256,864.456014368904,127.839524633406));
#73912=CARTESIAN_POINT('',(43.3912138270256,862.792597737398,134.046419876894));
#73913=CARTESIAN_POINT('Origin',(43.3912138270256,862.321175506789,133.879803309627));
#73914=CARTESIAN_POINT('',(43.3912138270256,861.337506002844,138.163432983664));
#73915=CARTESIAN_POINT('',(43.3912138270256,864.927436599513,128.006141200673));
#73916=CARTESIAN_POINT('Origin',(43.3912138270256,860.866083772235,137.996816416397));
#73917=CARTESIAN_POINT('Origin',(38.5967040184659,866.544078058546,128.577516992727));
#73918=CARTESIAN_POINT('',(38.5967040184659,864.415246277675,139.251210534735));
#73919=CARTESIAN_POINT('Origin',(38.5967040184659,862.954147461878,138.734808775718));
#73920=CARTESIAN_POINT('',(38.5967040184659,865.081712546744,137.3655216123));
#73921=CARTESIAN_POINT('',(38.5967040184659,868.005176874344,129.093918751744));
#73922=CARTESIAN_POINT('Origin',(38.5967040184659,863.620613730946,136.849119853283));
#73923=CARTESIAN_POINT('Origin',(38.5967040184659,866.544078058546,128.577516992727));
#73924=CARTESIAN_POINT('',(38.5967040184659,864.88066142704,134.784412236215));
#73925=CARTESIAN_POINT('Origin',(38.5967040184659,864.409239196431,134.617795668948));
#73926=CARTESIAN_POINT('',(38.5967040184659,863.425569692487,138.901425342985));
#73927=CARTESIAN_POINT('',(38.5967040184659,867.015500289155,128.744133559994));
#73928=CARTESIAN_POINT('Origin',(38.5967040184659,862.954147461878,138.734808775718));
#73929=CARTESIAN_POINT('Origin',(32.7290084090824,868.267123530476,129.186499563207));
#73930=CARTESIAN_POINT('',(32.7290084090824,865.864574510769,139.763452171557));
#73931=CARTESIAN_POINT('Origin',(32.7290084090824,864.677192933807,139.343791346199));
#73932=CARTESIAN_POINT('',(32.7290084119901,866.522075296429,137.90313004341));
#73933=CARTESIAN_POINT('',(32.7290084090824,869.454505107438,129.606160388566));
#73934=CARTESIAN_POINT('',(32.224018953637,864.255919089243,137.073658262999));
#73935=CARTESIAN_POINT('Ctrl Pts',(32.7290084148977,866.522075296429,137.90313004341));
#73936=CARTESIAN_POINT('Ctrl Pts',(32.7031571054404,866.521973103398,137.903419187084));
#73937=CARTESIAN_POINT('Ctrl Pts',(32.6772788326208,866.521125940755,137.903427495176));
#73938=CARTESIAN_POINT('Ctrl Pts',(32.4866202194529,866.50936005611,137.901396400289));
#73939=CARTESIAN_POINT('Ctrl Pts',(32.3254249892325,866.468990340329,137.888137795238));
#73940=CARTESIAN_POINT('Ctrl Pts',(32.1770177512588,866.40075615057,137.864021523816));
#73941=CARTESIAN_POINT('Ctrl Pts',(32.1227384712491,866.375799802465,137.855201105976));
#73942=CARTESIAN_POINT('Ctrl Pts',(32.0704336285077,866.347236523339,137.844973165265));
#73943=CARTESIAN_POINT('Ctrl Pts',(31.8852076585773,866.228701660669,137.802106614585));
#73944=CARTESIAN_POINT('Ctrl Pts',(31.7691493604183,866.118381696111,137.761450556226));
#73945=CARTESIAN_POINT('Ctrl Pts',(31.5888808659421,865.863043126858,137.666553800691));
#73946=CARTESIAN_POINT('Ctrl Pts',(31.5261645698418,865.720574753644,137.613275120991));
#73947=CARTESIAN_POINT('Ctrl Pts',(31.4618463420553,865.419681018586,137.500796068224));
#73948=CARTESIAN_POINT('Ctrl Pts',(31.4614758387299,865.263996806062,137.442634824622));
#73949=CARTESIAN_POINT('Ctrl Pts',(31.5227955825501,864.970146801218,137.333459398223));
#73950=CARTESIAN_POINT('Ctrl Pts',(31.5802669420954,864.833988571264,137.283159629352));
#73951=CARTESIAN_POINT('Ctrl Pts',(31.743685984272,864.589722450943,137.19363626273));
#73952=CARTESIAN_POINT('Ctrl Pts',(31.8475216280003,864.483235899298,137.154993156499));
#73953=CARTESIAN_POINT('Ctrl Pts',(32.0480530304138,864.340427466563,137.103660574143));
#73954=CARTESIAN_POINT('Ctrl Pts',(32.1336529452771,864.293213381728,137.086839327847));
#73955=CARTESIAN_POINT('Ctrl Pts',(32.2240189536389,864.255919089247,137.073658263001));
#73956=CARTESIAN_POINT('',(33.9489801953611,865.049016072261,137.353965571905));
#73957=CARTESIAN_POINT('Origin',(32.7290084090817,865.343659202875,137.458102423763));
#73958=CARTESIAN_POINT('Ctrl Pts',(33.948980195361,865.049016072261,137.353965571905));
#73959=CARTESIAN_POINT('Ctrl Pts',(33.9861939659006,865.185989792186,137.402376719148));
#73960=CARTESIAN_POINT('Ctrl Pts',(33.9971725931947,865.32808448117,137.452913675735));
#73961=CARTESIAN_POINT('Ctrl Pts',(33.9652989340809,865.610916023887,137.554575537985));
#73962=CARTESIAN_POINT('Ctrl Pts',(33.9219603364262,865.749224037751,137.604848857897));
#73963=CARTESIAN_POINT('Ctrl Pts',(33.7825322278083,866.008623498807,137.700464876327));
#73964=CARTESIAN_POINT('Ctrl Pts',(33.6858885484776,866.126659460691,137.744730929575));
#73965=CARTESIAN_POINT('Ctrl Pts',(33.4440501715648,866.328747814992,137.82199258999));
#73966=CARTESIAN_POINT('Ctrl Pts',(33.2986567258858,866.408303455729,137.853367091886));
#73967=CARTESIAN_POINT('Ctrl Pts',(33.0082071907687,866.501334098523,137.891757634516));
#73968=CARTESIAN_POINT('Ctrl Pts',(32.8690031975687,866.522628710994,137.901564219218));
#73969=CARTESIAN_POINT('Ctrl Pts',(32.7290084148977,866.522075296429,137.90313004341));
#73970=CARTESIAN_POINT('Origin',(32.7290084090824,868.267123530476,129.186499563207));
#73971=CARTESIAN_POINT('',(32.7290084090824,866.603706898969,135.393394806696));
#73972=CARTESIAN_POINT('Origin',(32.7290084090824,866.132284668361,135.226778239429));
#73973=CARTESIAN_POINT('',(32.7290084090824,865.148615164416,139.510407913466));
#73974=CARTESIAN_POINT('',(32.7290084090824,868.738545761084,129.353116130474));
#73975=CARTESIAN_POINT('Origin',(32.7290084090824,864.677192933807,139.343791346199));
#73976=CARTESIAN_POINT('Origin',(60.1505256426703,840.372072930537,119.327444828556));
#73977=CARTESIAN_POINT('',(60.1505256426703,837.780504752995,129.837591670903));
#73978=CARTESIAN_POINT('Origin',(60.1505256426703,836.782142333868,129.484736611547));
#73979=CARTESIAN_POINT('',(60.1505256426703,838.446971022064,127.951902748468));
#73980=CARTESIAN_POINT('',(60.1505256426703,841.370435349664,119.680299887912));
#73981=CARTESIAN_POINT('Origin',(60.1505256426703,837.448608602936,127.599047689112));
#73982=CARTESIAN_POINT('Origin',(60.1505256426703,840.372072930537,119.327444828556));
#73983=CARTESIAN_POINT('',(60.1505256426703,838.70865629903,125.534340072044));
#73984=CARTESIAN_POINT('Origin',(60.1505256426703,838.237234068422,125.367723504777));
#73985=CARTESIAN_POINT('',(60.1505256426703,837.253564564477,129.651353178814));
#73986=CARTESIAN_POINT('',(60.1505256426703,840.843495161145,119.494061395823));
#73987=CARTESIAN_POINT('Origin',(60.1505256426703,836.782142333868,129.484736611547));
#73988=CARTESIAN_POINT('Origin',(60.7541790064059,844.277713713595,120.707830431948));
#73989=CARTESIAN_POINT('',(60.7541790064059,841.909552396309,131.29693681787));
#73990=CARTESIAN_POINT('Origin',(60.7541790064059,840.687783116927,130.865122214939));
#73991=CARTESIAN_POINT('',(60.7541790064059,842.576018665377,129.411247895435));
#73992=CARTESIAN_POINT('',(60.7541790064059,845.499482992978,121.139645034879));
#73993=CARTESIAN_POINT('Origin',(60.7541790064059,841.354249385995,128.979433292504));
#73994=CARTESIAN_POINT('Origin',(60.7541790064059,844.277713713595,120.707830431948));
#73995=CARTESIAN_POINT('',(60.7541790064059,842.614297082089,126.914725675436));
#73996=CARTESIAN_POINT('Origin',(60.7541790064059,842.14287485148,126.748109108169));
#73997=CARTESIAN_POINT('',(60.7541790064059,841.159205347535,131.031738782206));
#73998=CARTESIAN_POINT('',(60.7541790064059,844.749135944204,120.874446999215));
#73999=CARTESIAN_POINT('Origin',(60.7541790064059,840.687783116927,130.865122214939));
#74000=CARTESIAN_POINT('Origin',(60.710027526019,848.756559286629,122.290806002987));
#74001=CARTESIAN_POINT('',(60.710027526019,846.681345091961,132.983449814156));
#74002=CARTESIAN_POINT('Origin',(60.710027526019,845.166628689961,132.448097785978));
#74003=CARTESIAN_POINT('',(60.710027526019,847.34781136103,131.097760891721));
#74004=CARTESIAN_POINT('',(60.710027526019,850.27127568863,122.826158031165));
#74005=CARTESIAN_POINT('Origin',(60.710027526019,845.833094959029,130.562408863543));
#74006=CARTESIAN_POINT('Origin',(60.710027526019,848.756559286629,122.290806002987));
#74007=CARTESIAN_POINT('',(60.710027526019,847.093142655123,128.497701246475));
#74008=CARTESIAN_POINT('Origin',(60.710027526019,846.621720424514,128.331084679208));
#74009=CARTESIAN_POINT('',(60.710027526019,845.63805092057,132.614714353245));
#74010=CARTESIAN_POINT('',(60.710027526019,849.227981517238,122.457422570254));
#74011=CARTESIAN_POINT('Origin',(60.710027526019,845.166628689961,132.448097785978));
#74012=CARTESIAN_POINT('Origin',(59.6300369248449,853.078930346135,123.818478186497));
#74013=CARTESIAN_POINT('',(59.6300369248449,851.212611893914,134.584952821211));
#74014=CARTESIAN_POINT('Origin',(59.6300369248449,849.488999749467,133.975769969489));
#74015=CARTESIAN_POINT('',(59.6300369248449,851.879078162982,132.699263898776));
#74016=CARTESIAN_POINT('',(59.6300369248449,854.802542490582,124.42766103822));
#74017=CARTESIAN_POINT('Origin',(59.6300369248449,850.155466018535,132.090081047054));
#74018=CARTESIAN_POINT('Origin',(59.6300369248449,853.078930346135,123.818478186497));
#74019=CARTESIAN_POINT('',(59.6300369248449,851.415513714629,130.025373429986));
#74020=CARTESIAN_POINT('Origin',(59.6300369248449,850.94409148402,129.858756862719));
#74021=CARTESIAN_POINT('',(59.6300369248449,849.960421980075,134.142386536756));
#74022=CARTESIAN_POINT('',(59.6300369248449,853.550352576744,123.985094753765));
#74023=CARTESIAN_POINT('Origin',(59.6300369248449,849.488999749467,133.975769969489));
#74024=CARTESIAN_POINT('Origin',(57.8564754088671,857.60895058869,125.419540617283));
#74025=CARTESIAN_POINT('',(57.8564754088671,855.771219389582,136.196118954521));
#74026=CARTESIAN_POINT('Origin',(57.8564754088671,854.019019992021,135.576832400274));
#74027=CARTESIAN_POINT('',(57.8564754088671,856.437685658651,134.310430032086));
#74028=CARTESIAN_POINT('',(57.8564754088671,859.361149986251,126.03882717153));
#74029=CARTESIAN_POINT('Origin',(57.8564754088671,854.685486261089,133.691143477839));
#74030=CARTESIAN_POINT('Origin',(57.8564754088671,857.60895058869,125.419540617283));
#74031=CARTESIAN_POINT('',(57.8564754088671,855.945533957183,131.626435860771));
#74032=CARTESIAN_POINT('Origin',(57.8564754088671,855.474111726575,131.459819293504));
#74033=CARTESIAN_POINT('',(57.8564754088671,854.49044222263,135.743448967541));
#74034=CARTESIAN_POINT('',(57.8564754088671,858.080372819298,125.58615718455));
#74035=CARTESIAN_POINT('Origin',(57.8564754088671,854.019019992021,135.576832400274));
#74036=CARTESIAN_POINT('Origin',(55.1009921650808,861.268440685064,126.712928239285));
#74037=CARTESIAN_POINT('',(55.1009921650808,859.387752436776,137.474324101854));
#74038=CARTESIAN_POINT('Origin',(55.1009921650808,857.678510088396,136.870220022276));
#74039=CARTESIAN_POINT('',(55.1009921650808,860.054218705844,135.588635179419));
#74040=CARTESIAN_POINT('',(55.1009921650808,862.977683033444,127.317032318863));
#74041=CARTESIAN_POINT('Origin',(55.1009921650808,858.344976357464,134.984531099841));
#74042=CARTESIAN_POINT('Origin',(55.1009921650808,861.268440685064,126.712928239285));
#74043=CARTESIAN_POINT('',(55.1009921650808,859.605024053558,132.919823482773));
#74044=CARTESIAN_POINT('Origin',(55.1009921650808,859.133601822949,132.753206915506));
#74045=CARTESIAN_POINT('',(55.1009921650808,858.149932319004,137.036836589543));
#74046=CARTESIAN_POINT('',(55.1009921650808,861.739862915673,126.879544806552));
#74047=CARTESIAN_POINT('Origin',(55.1009921650808,857.678510088396,136.870220022276));
#74048=CARTESIAN_POINT('Origin',(51.3485798144127,865.547611143858,128.225331868775));
#74049=CARTESIAN_POINT('',(51.3485798144127,863.75989569723,139.019587465264));
#74050=CARTESIAN_POINT('Origin',(51.3485798144127,861.957680547189,138.382623651766));
#74051=CARTESIAN_POINT('',(51.3485798144127,864.426361966298,137.133898542829));
#74052=CARTESIAN_POINT('',(51.3485798144127,867.349826293898,128.862295682273));
#74053=CARTESIAN_POINT('Origin',(51.3485798144127,862.624146816258,136.496934729331));
#74054=CARTESIAN_POINT('Origin',(51.3485798144127,865.547611143858,128.225331868775));
#74055=CARTESIAN_POINT('',(51.3485798144127,863.884194512352,134.432227112263));
#74056=CARTESIAN_POINT('Origin',(51.3485798144127,863.412772281743,134.265610544996));
#74057=CARTESIAN_POINT('',(51.3485798144127,862.429102777798,138.549240219033));
#74058=CARTESIAN_POINT('',(51.3485798144127,866.019033374467,128.391948436042));
#74059=CARTESIAN_POINT('Origin',(51.3485798144127,861.957680547189,138.382623651766));
#74060=CARTESIAN_POINT('Origin',(47.119291675836,868.529905652021,129.279375656417));
#74061=CARTESIAN_POINT('',(47.119291675836,866.40107387115,139.953069198425));
#74062=CARTESIAN_POINT('Origin',(47.119291675836,864.939975055353,139.436667439408));
#74063=CARTESIAN_POINT('',(47.119291675836,867.067540140218,138.06738027599));
#74064=CARTESIAN_POINT('',(47.119291675836,869.991004467819,129.795777415434));
#74065=CARTESIAN_POINT('Origin',(47.119291675836,865.606441324421,137.550978516973));
#74066=CARTESIAN_POINT('Origin',(47.119291675836,868.529905652021,129.279375656417));
#74067=CARTESIAN_POINT('',(47.119291675836,866.866489020515,135.486270899905));
#74068=CARTESIAN_POINT('Origin',(47.119291675836,866.395066789906,135.319654332638));
#74069=CARTESIAN_POINT('',(47.119291675836,865.411397285961,139.603284006675));
#74070=CARTESIAN_POINT('',(47.119291675836,869.00132788263,129.445992223684));
#74071=CARTESIAN_POINT('Origin',(47.119291675836,864.939975055353,139.436667439408));
#74072=CARTESIAN_POINT('Origin',(41.7597772954093,871.365533346835,130.281582429626));
#74073=CARTESIAN_POINT('',(41.7597772954093,868.962984327129,140.858535037976));
#74074=CARTESIAN_POINT('Origin',(41.7597772954093,867.775602750167,140.438874212617));
#74075=CARTESIAN_POINT('',(41.7597773059811,869.619655531143,139.000560114769));
#74076=CARTESIAN_POINT('',(41.7597772954093,872.552914923797,130.701243254984));
#74077=CARTESIAN_POINT('',(41.0259596626274,867.477090904821,138.212129373697));
#74078=CARTESIAN_POINT('Ctrl Pts',(41.7597773059816,869.619655531119,139.000560114837));
#74079=CARTESIAN_POINT('Ctrl Pts',(41.6573369345889,869.619422397947,139.001219740658));
#74080=CARTESIAN_POINT('Ctrl Pts',(41.555042709061,869.607515464247,138.997398768683));
#74081=CARTESIAN_POINT('Ctrl Pts',(41.4551932856153,869.584049900572,138.989105244503));
#74082=CARTESIAN_POINT('Ctrl Pts',(41.3965968798861,869.57027918821,138.984238208811));
#74083=CARTESIAN_POINT('Ctrl Pts',(41.339127186869,869.552594230335,138.977855034907));
#74084=CARTESIAN_POINT('Ctrl Pts',(41.1317427249637,869.472965862453,138.948739355919));
#74085=CARTESIAN_POINT('Ctrl Pts',(40.9937779581549,869.387818807864,138.91698025569));
#74086=CARTESIAN_POINT('Ctrl Pts',(40.7608204171255,869.173429676768,138.836556417158));
#74087=CARTESIAN_POINT('Ctrl Pts',(40.6678554670967,869.046388839606,138.788730350703));
#74088=CARTESIAN_POINT('Ctrl Pts',(40.5381661401692,868.764720660735,138.683046260005));
#74089=CARTESIAN_POINT('Ctrl Pts',(40.503255619118,868.612532689981,138.626120706543));
#74090=CARTESIAN_POINT('Ctrl Pts',(40.4980684291032,868.313120120479,138.51497928158));
#74091=CARTESIAN_POINT('Ctrl Pts',(40.5241081013521,868.168686202312,138.46175460448));
#74092=CARTESIAN_POINT('Ctrl Pts',(40.6298704988454,867.89774502338,138.362803369572));
#74093=CARTESIAN_POINT('Ctrl Pts',(40.7078853849485,867.773237639588,138.317791091509));
#74094=CARTESIAN_POINT('Ctrl Pts',(40.8724837098879,867.594245965953,138.253670127529));
#74095=CARTESIAN_POINT('Ctrl Pts',(40.9457923328914,867.53128453031,138.231283234632));
#74096=CARTESIAN_POINT('Ctrl Pts',(41.0259596626275,867.477090904821,138.212129373697));
#74097=CARTESIAN_POINT('',(42.8881164335297,867.914715447588,138.366800694508));
#74098=CARTESIAN_POINT('Origin',(41.7597772954084,868.442069019235,138.553185290182));
#74099=CARTESIAN_POINT('Ctrl Pts',(42.88811643353,867.914715447588,138.366800694508));
#74100=CARTESIAN_POINT('Ctrl Pts',(42.9547218037881,868.041401007716,138.41157565797));
#74101=CARTESIAN_POINT('Ctrl Pts',(42.9968164695112,868.178236295445,138.460253764197));
#74102=CARTESIAN_POINT('Ctrl Pts',(43.0281257825353,868.461123763136,138.561935392225));
#74103=CARTESIAN_POINT('Ctrl Pts',(43.0163296236268,868.604895462998,138.614139763637));
#74104=CARTESIAN_POINT('Ctrl Pts',(42.9374225821821,868.885931270645,138.717402799037));
#74105=CARTESIAN_POINT('Ctrl Pts',(42.8690960860492,869.02031527311,138.767446802976));
#74106=CARTESIAN_POINT('Ctrl Pts',(42.677510436449,869.265354624792,138.859888799149));
#74107=CARTESIAN_POINT('Ctrl Pts',(42.5530630718917,869.371650665748,138.900714263267));
#74108=CARTESIAN_POINT('Ctrl Pts',(42.2676632709367,869.532017614981,138.963368373441));
#74109=CARTESIAN_POINT('Ctrl Pts',(42.1096748558595,869.584750951896,138.984653116944));
#74110=CARTESIAN_POINT('Ctrl Pts',(41.8836861993185,869.615671233301,138.998125913844));
#74111=CARTESIAN_POINT('Ctrl Pts',(41.8217050457295,869.619796465891,139.000161354703));
#74112=CARTESIAN_POINT('Ctrl Pts',(41.7597773059816,869.619655531119,139.000560114837));
#74113=CARTESIAN_POINT('Origin',(41.7597772954093,871.365533346835,130.281582429626));
#74114=CARTESIAN_POINT('',(41.7597772954093,869.702116715329,136.488477673114));
#74115=CARTESIAN_POINT('Origin',(41.7597772954093,869.23069448472,136.321861105847));
#74116=CARTESIAN_POINT('',(41.7597772954093,868.247024980775,140.605490779884));
#74117=CARTESIAN_POINT('',(41.7597772954093,871.836955577444,130.448198996893));
#74118=CARTESIAN_POINT('Origin',(41.7597772954093,867.775602750167,140.438874212617));
#74119=CARTESIAN_POINT('Origin',(62.4307813118898,838.704660762172,118.738124949954));
#74120=CARTESIAN_POINT('',(62.4307813118898,836.113092584631,129.248271792302));
#74121=CARTESIAN_POINT('Origin',(62.4307813118898,835.114730165504,128.895416732946));
#74122=CARTESIAN_POINT('',(62.4307813118898,836.779558853699,127.362582869867));
#74123=CARTESIAN_POINT('',(62.4307813118898,839.703023181299,119.090980009311));
#74124=CARTESIAN_POINT('Origin',(62.4307813118898,835.781196434572,127.009727810511));
#74125=CARTESIAN_POINT('Origin',(62.4307813118898,838.704660762172,118.738124949954));
#74126=CARTESIAN_POINT('',(62.4307813118898,837.041244130666,124.945020193443));
#74127=CARTESIAN_POINT('Origin',(62.4307813118898,836.569821900057,124.778403626176));
#74128=CARTESIAN_POINT('',(62.4307813118898,835.586152396113,129.062033300213));
#74129=CARTESIAN_POINT('',(62.4307813118898,839.176082992781,118.904741517222));
#74130=CARTESIAN_POINT('Origin',(62.4307813118898,835.114730165504,128.895416732946));
#74131=CARTESIAN_POINT('Origin',(63.8824972054392,842.406620728786,120.046522861103));
#74132=CARTESIAN_POINT('',(63.8824972054392,840.0384594115,130.635629247025));
#74133=CARTESIAN_POINT('Origin',(63.8824972054392,838.816690132118,130.203814644094));
#74134=CARTESIAN_POINT('',(63.8824972054392,840.704925680569,128.74994032459));
#74135=CARTESIAN_POINT('',(63.8824972054392,843.628390008169,120.478337464034));
#74136=CARTESIAN_POINT('Origin',(63.8824972054392,839.483156401186,128.318125721659));
#74137=CARTESIAN_POINT('Origin',(63.8824972054392,842.406620728786,120.046522861103));
#74138=CARTESIAN_POINT('',(63.8824972054392,840.74320409728,126.253418104591));
#74139=CARTESIAN_POINT('Origin',(63.8824972054392,840.271781866671,126.086801537324));
#74140=CARTESIAN_POINT('',(63.8824972054392,839.288112362726,130.370431211361));
#74141=CARTESIAN_POINT('',(63.8824972054392,842.878042959395,120.21313942837));
#74142=CARTESIAN_POINT('Origin',(63.8824972054392,838.816690132118,130.203814644094));
#74143=CARTESIAN_POINT('Origin',(64.8269648086385,846.796247723552,121.597965567795));
#74144=CARTESIAN_POINT('',(64.8269648086385,844.721033528884,132.290609378964));
#74145=CARTESIAN_POINT('Origin',(64.8269648086385,843.206317126883,131.755257350787));
#74146=CARTESIAN_POINT('',(64.8269648086385,845.387499797952,130.404920456529));
#74147=CARTESIAN_POINT('',(64.8269648086385,848.310964125552,122.133317595973));
#74148=CARTESIAN_POINT('Origin',(64.8269648086385,843.872783395951,129.869568428351));
#74149=CARTESIAN_POINT('Origin',(64.8269648086385,846.796247723552,121.597965567795));
#74150=CARTESIAN_POINT('',(64.8269648086385,845.132831092045,127.804860811284));
#74151=CARTESIAN_POINT('Origin',(64.8269648086385,844.661408861436,127.638244244017));
#74152=CARTESIAN_POINT('',(64.8269648086385,843.677739357492,131.921873918054));
#74153=CARTESIAN_POINT('',(64.8269648086385,847.26766995416,121.764582135062));
#74154=CARTESIAN_POINT('Origin',(64.8269648086385,843.206317126883,131.755257350787));
#74155=CARTESIAN_POINT('Origin',(64.7237238265774,851.23587341945,123.167079507217));
#74156=CARTESIAN_POINT('',(64.7237238265774,849.369554967228,133.933554141931));
#74157=CARTESIAN_POINT('Origin',(64.7237238265774,847.645942822782,133.324371290208));
#74158=CARTESIAN_POINT('',(64.7237238265774,850.036021236297,132.047865219495));
#74159=CARTESIAN_POINT('',(64.7237238265774,852.959485563897,123.776262358939));
#74160=CARTESIAN_POINT('Origin',(64.7237238265774,848.31240909185,131.438682367773));
#74161=CARTESIAN_POINT('Origin',(64.7237238265774,851.23587341945,123.167079507217));
#74162=CARTESIAN_POINT('',(64.7237238265774,849.572456787944,129.373974750705));
#74163=CARTESIAN_POINT('Origin',(64.7237238265774,849.101034557335,129.207358183438));
#74164=CARTESIAN_POINT('',(64.7237238265774,848.117365053391,133.490987857475));
#74165=CARTESIAN_POINT('',(64.7237238265774,851.707295650059,123.333696074484));
#74166=CARTESIAN_POINT('Origin',(64.7237238265774,847.645942822782,133.324371290208));
#74167=CARTESIAN_POINT('Origin',(63.9878579537236,856.014570252624,124.85603265931));
#74168=CARTESIAN_POINT('',(63.9878579537236,854.176839053517,135.632610996548));
#74169=CARTESIAN_POINT('Origin',(63.9878579537236,852.424639655956,135.013324442301));
#74170=CARTESIAN_POINT('',(63.9878579537236,854.843305322585,133.746922074113));
#74171=CARTESIAN_POINT('',(63.9878579537236,857.766769650186,125.475319213557));
#74172=CARTESIAN_POINT('Origin',(63.9878579537236,853.091105925024,133.127635519866));
#74173=CARTESIAN_POINT('Origin',(63.9878579537236,856.014570252624,124.85603265931));
#74174=CARTESIAN_POINT('',(63.9878579537236,854.351153621118,131.062927902798));
#74175=CARTESIAN_POINT('Origin',(63.9878579537236,853.879731390509,130.896311335531));
#74176=CARTESIAN_POINT('',(63.9878579537236,852.896061886564,135.179941009568));
#74177=CARTESIAN_POINT('',(63.9878579537236,856.485992483233,125.022649226577));
#74178=CARTESIAN_POINT('Origin',(63.9878579537236,852.424639655956,135.013324442301));
#74179=CARTESIAN_POINT('Origin',(62.0995624254871,860.134244643534,126.312064981726));
#74180=CARTESIAN_POINT('',(62.0995624254871,858.253556395246,137.073460844295));
#74181=CARTESIAN_POINT('Origin',(62.0995624254871,856.544314046866,136.469356764717));
#74182=CARTESIAN_POINT('',(62.0995624254871,858.920022664315,135.18777192186));
#74183=CARTESIAN_POINT('',(62.0995624254871,861.843486991915,126.916169061304));
#74184=CARTESIAN_POINT('Origin',(62.0995624254871,857.210780315934,134.583667842282));
#74185=CARTESIAN_POINT('Origin',(62.0995624254871,860.134244643534,126.312064981726));
#74186=CARTESIAN_POINT('',(62.0995624254871,858.470828012028,132.518960225214));
#74187=CARTESIAN_POINT('Origin',(62.0995624254871,857.999405781419,132.352343657947));
#74188=CARTESIAN_POINT('',(62.0995624254871,857.015736277475,136.635973331984));
#74189=CARTESIAN_POINT('',(62.0995624254871,860.605666874143,126.478681548993));
#74190=CARTESIAN_POINT('Origin',(62.0995624254871,856.544314046866,136.469356764717));
#74191=CARTESIAN_POINT('Origin',(59.3727721247612,865.055484298055,128.05139758994));
#74192=CARTESIAN_POINT('',(59.3727721247612,863.267768851427,138.845653186429));
#74193=CARTESIAN_POINT('Origin',(59.3727721247612,861.465553701386,138.208689372931));
#74194=CARTESIAN_POINT('',(59.3727721247612,863.934235120495,136.959964263994));
#74195=CARTESIAN_POINT('',(59.3727721247612,866.857699448095,128.688361403438));
#74196=CARTESIAN_POINT('Origin',(59.3727721247612,862.132019970455,136.323000450496));
#74197=CARTESIAN_POINT('Origin',(59.3727721247612,865.055484298055,128.05139758994));
#74198=CARTESIAN_POINT('',(59.3727721247612,863.392067666549,134.258292833428));
#74199=CARTESIAN_POINT('Origin',(59.3727721247612,862.92064543594,134.091676266161));
#74200=CARTESIAN_POINT('',(59.3727721247612,861.936975931995,138.375305940198));
#74201=CARTESIAN_POINT('',(59.3727721247612,865.526906528664,128.218014157207));
#74202=CARTESIAN_POINT('Origin',(59.3727721247612,861.465553701386,138.208689372931));
#74203=CARTESIAN_POINT('Origin',(55.8935458421992,868.801669044095,129.37542603452));
#74204=CARTESIAN_POINT('',(55.8935458421992,866.672837263224,140.049119576529));
#74205=CARTESIAN_POINT('Origin',(55.8935458421992,865.211738447427,139.532717817511));
#74206=CARTESIAN_POINT('',(55.8935458421992,867.339303532293,138.163430654094));
#74207=CARTESIAN_POINT('',(55.8935458421992,870.262767859893,129.891827793537));
#74208=CARTESIAN_POINT('Origin',(55.8935458421992,865.878204716495,137.647028895076));
#74209=CARTESIAN_POINT('Origin',(55.8935458421992,868.801669044095,129.37542603452));
#74210=CARTESIAN_POINT('',(55.8935458421992,867.138252412589,135.582321278008));
#74211=CARTESIAN_POINT('Origin',(55.8935458421992,866.66683018198,135.415704710741));
#74212=CARTESIAN_POINT('',(55.8935458421992,865.683160678035,139.699334384778));
#74213=CARTESIAN_POINT('',(55.8935458421992,869.273091274704,129.542042601787));
#74214=CARTESIAN_POINT('Origin',(55.8935458421992,865.211738447427,139.532717817511));
#74215=CARTESIAN_POINT('Origin',(51.2764491869573,872.62594842468,130.727055765347));
#74216=CARTESIAN_POINT('',(51.2764491869573,870.223399404973,141.304008373696));
#74217=CARTESIAN_POINT('Origin',(51.2764491869573,869.036017828011,140.884347548338));
#74218=CARTESIAN_POINT('',(51.2764491871435,870.879723090442,139.447016713862));
#74219=CARTESIAN_POINT('',(51.2764491869573,873.813330001642,131.146716590705));
#74220=CARTESIAN_POINT('',(50.3458747286375,868.902442155958,138.715896733814));
#74221=CARTESIAN_POINT('Ctrl Pts',(51.2764491873298,870.879723090442,139.447016713862));
#74222=CARTESIAN_POINT('Ctrl Pts',(51.2618354165802,870.879718220088,139.447030493977));
#74223=CARTESIAN_POINT('Ctrl Pts',(51.2472113783088,870.879475947816,139.446952641435));
#74224=CARTESIAN_POINT('Ctrl Pts',(51.232583607977,870.878995268524,139.446782753109));
#74225=CARTESIAN_POINT('Ctrl Pts',(51.172231020632,870.877012038113,139.446081812378));
#74226=CARTESIAN_POINT('Ctrl Pts',(51.1121081786909,870.870980141333,139.443817224556));
#74227=CARTESIAN_POINT('Ctrl Pts',(50.8916289209462,870.833751761404,139.429687135951));
#74228=CARTESIAN_POINT('Ctrl Pts',(50.7377874078257,870.777521818001,139.408148321249));
#74229=CARTESIAN_POINT('Ctrl Pts',(50.4623221826389,870.613515830349,139.345531590367));
#74230=CARTESIAN_POINT('Ctrl Pts',(50.3431715930928,870.507494995374,139.305134703914));
#74231=CARTESIAN_POINT('Ctrl Pts',(50.1537792129284,870.257446839222,139.210626199135));
#74232=CARTESIAN_POINT('Ctrl Pts',(50.085854431441,870.115449532897,139.157302371292));
#74233=CARTESIAN_POINT('Ctrl Pts',(50.0143870126858,869.823633201028,139.048845713734));
#74234=CARTESIAN_POINT('Ctrl Pts',(50.0078569390086,869.677265941222,138.994937728282));
#74235=CARTESIAN_POINT('Ctrl Pts',(50.0513403675436,869.391534956718,138.890759275659));
#74236=CARTESIAN_POINT('Ctrl Pts',(50.1001248711416,869.254462140642,138.841305948666));
#74237=CARTESIAN_POINT('Ctrl Pts',(50.2215963819772,869.047121819918,138.767165613604));
#74238=CARTESIAN_POINT('Ctrl Pts',(50.2794097745223,868.971166592971,138.740186275205));
#74239=CARTESIAN_POINT('Ctrl Pts',(50.3458747286374,868.902442155957,138.715896733814));
#74240=CARTESIAN_POINT('',(52.2638418422125,868.965467966003,138.738172187616));
#74241=CARTESIAN_POINT('Origin',(51.2764491869568,869.70248409708,138.998658625903));
#74242=CARTESIAN_POINT('Ctrl Pts',(52.2638418422126,868.965467966004,138.738172187616));
#74243=CARTESIAN_POINT('Ctrl Pts',(52.3569278379003,869.076328599452,138.77735408654));
#74244=CARTESIAN_POINT('Ctrl Pts',(52.4282988031681,869.201919789666,138.822058148252));
#74245=CARTESIAN_POINT('Ctrl Pts',(52.5214227211125,869.472476304179,138.919381600198));
#74246=CARTESIAN_POINT('Ctrl Pts',(52.5416845496989,869.615409082029,138.971289468186));
#74247=CARTESIAN_POINT('Ctrl Pts',(52.5267471917766,869.905744583059,139.07783932989));
#74248=CARTESIAN_POINT('Ctrl Pts',(52.48972407459,870.050568410474,139.131573121207));
#74249=CARTESIAN_POINT('Ctrl Pts',(52.3567643645195,870.327769216161,139.235382063435));
#74250=CARTESIAN_POINT('Ctrl Pts',(52.2587020280801,870.456115288957,139.284000754887));
#74251=CARTESIAN_POINT('Ctrl Pts',(52.0153162405214,870.668883275139,139.365175164552));
#74252=CARTESIAN_POINT('Ctrl Pts',(51.8725921545554,870.751416302552,139.396992126975));
#74253=CARTESIAN_POINT('Ctrl Pts',(51.5758456035277,870.854733983497,139.437035579406));
#74254=CARTESIAN_POINT('Ctrl Pts',(51.4266900107678,870.879773161437,139.446875043663));
#74255=CARTESIAN_POINT('Ctrl Pts',(51.2764491873298,870.879723090442,139.447016713862));
#74256=CARTESIAN_POINT('Origin',(51.2764491869573,872.62594842468,130.727055765347));
#74257=CARTESIAN_POINT('',(51.2764491869573,870.962531793174,136.933951008835));
#74258=CARTESIAN_POINT('Origin',(51.2764491869573,870.491109562565,136.767334441568));
#74259=CARTESIAN_POINT('',(51.2764491869573,869.50744005862,141.050964115605));
#74260=CARTESIAN_POINT('',(51.2764491869573,873.097370655289,130.893672332614));
#74261=CARTESIAN_POINT('Origin',(51.2764491869573,869.036017828011,140.884347548338));
#74262=CARTESIAN_POINT('Origin',(64.2935179203293,836.626690711497,118.003700024172));
#74263=CARTESIAN_POINT('',(64.2935179203293,834.035122533956,128.513846866519));
#74264=CARTESIAN_POINT('Origin',(64.2935179203293,833.036760114829,128.160991807163));
#74265=CARTESIAN_POINT('',(64.2935179203293,834.701588803024,126.628157944084));
#74266=CARTESIAN_POINT('',(64.2935179203293,837.625053130624,118.356555083528));
#74267=CARTESIAN_POINT('Origin',(64.2935179203293,833.703226383897,126.275302884728));
#74268=CARTESIAN_POINT('Origin',(64.2935179203293,836.626690711497,118.003700024172));
#74269=CARTESIAN_POINT('',(64.2935179203293,834.963274079991,124.21059526766));
#74270=CARTESIAN_POINT('Origin',(64.2935179203293,834.491851849382,124.043978700393));
#74271=CARTESIAN_POINT('',(64.2935179203293,833.508182345437,128.32760837443));
#74272=CARTESIAN_POINT('',(64.2935179203293,837.098112942106,118.170316591439));
#74273=CARTESIAN_POINT('Origin',(64.2935179203293,833.036760114829,128.160991807163));
#74274=CARTESIAN_POINT('Origin',(66.5298493930383,839.963176447151,119.182926975969));
#74275=CARTESIAN_POINT('',(66.5298493930383,837.595015129865,129.772033361891));
#74276=CARTESIAN_POINT('Origin',(66.5298493930383,836.373245850482,129.34021875896));
#74277=CARTESIAN_POINT('',(66.5298493930383,838.261481398933,127.886344439456));
#74278=CARTESIAN_POINT('',(66.5298493930383,841.184945726533,119.6147415789));
#74279=CARTESIAN_POINT('Origin',(66.5298493930383,837.03971211955,127.454529836525));
#74280=CARTESIAN_POINT('Origin',(66.5298493930383,839.963176447151,119.182926975969));
#74281=CARTESIAN_POINT('',(66.5298493930383,838.299759815644,125.389822219457));
#74282=CARTESIAN_POINT('Origin',(66.5298493930383,837.828337585036,125.22320565219));
#74283=CARTESIAN_POINT('',(66.5298493930383,836.844668081091,129.506835326227));
#74284=CARTESIAN_POINT('',(66.5298493930383,840.434598677759,119.349543543236));
#74285=CARTESIAN_POINT('Origin',(66.5298493930383,836.373245850482,129.34021875896));
#74286=CARTESIAN_POINT('Origin',(68.4216583135058,844.071737100209,120.635031327384));
#74287=CARTESIAN_POINT('',(68.4216583135058,841.996522905541,131.327675138553));
#74288=CARTESIAN_POINT('Origin',(68.4216583135058,840.48180650354,130.792323110376));
#74289=CARTESIAN_POINT('',(68.4216583135058,842.662989174609,129.441986216118));
#74290=CARTESIAN_POINT('',(68.4216583135058,845.586453502209,121.170383355562));
#74291=CARTESIAN_POINT('Origin',(68.4216583135058,841.148272772608,128.906634187941));
#74292=CARTESIAN_POINT('Origin',(68.4216583135058,844.071737100209,120.635031327384));
#74293=CARTESIAN_POINT('',(68.4216583135058,842.408320468702,126.841926570873));
#74294=CARTESIAN_POINT('Origin',(68.4216583135058,841.936898238093,126.675310003606));
#74295=CARTESIAN_POINT('',(68.4216583135058,840.953228734149,130.958939677643));
#74296=CARTESIAN_POINT('',(68.4216583135058,844.543159330817,120.801647894651));
#74297=CARTESIAN_POINT('Origin',(68.4216583135058,840.48180650354,130.792323110376));
#74298=CARTESIAN_POINT('Origin',(69.2996790768792,848.434584485902,122.17700921412));
#74299=CARTESIAN_POINT('',(69.2996790768792,846.56826603368,132.943483848834));
#74300=CARTESIAN_POINT('Origin',(69.2996790768792,844.844653889233,132.334300997111));
#74301=CARTESIAN_POINT('',(69.2996790768792,847.234732302748,131.057794926399));
#74302=CARTESIAN_POINT('',(69.2996790768792,850.158196630348,122.786192065843));
#74303=CARTESIAN_POINT('Origin',(69.2996790768792,845.511120158302,130.448612074676));
#74304=CARTESIAN_POINT('Origin',(69.2996790768792,848.434584485902,122.17700921412));
#74305=CARTESIAN_POINT('',(69.2996790768792,846.771167854396,128.383904457608));
#74306=CARTESIAN_POINT('Origin',(69.2996790768792,846.299745623787,128.217287890341));
#74307=CARTESIAN_POINT('',(69.2996790768792,845.316076119842,132.500917564379));
#74308=CARTESIAN_POINT('',(69.2996790768792,848.906006716511,122.343625781387));
#74309=CARTESIAN_POINT('Origin',(69.2996790768792,844.844653889233,132.334300997111));
#74310=CARTESIAN_POINT('Origin',(69.6336697168692,853.253105927354,123.880037730278));
#74311=CARTESIAN_POINT('',(69.6336697168692,851.415374728247,134.656616067516));
#74312=CARTESIAN_POINT('Origin',(69.6336697168692,849.663175330685,134.03732951327));
#74313=CARTESIAN_POINT('',(69.6336697168692,852.081840997315,132.770927145081));
#74314=CARTESIAN_POINT('',(69.6336697168692,855.005305324915,124.499324284525));
#74315=CARTESIAN_POINT('Origin',(69.6336697168692,850.329641599754,132.151640590834));
#74316=CARTESIAN_POINT('Origin',(69.6336697168692,853.253105927354,123.880037730278));
#74317=CARTESIAN_POINT('',(69.6336697168692,851.589689295848,130.086932973767));
#74318=CARTESIAN_POINT('Origin',(69.6336697168692,851.118267065239,129.9203164065));
#74319=CARTESIAN_POINT('',(69.6336697168692,850.134597561294,134.203946080537));
#74320=CARTESIAN_POINT('',(69.6336697168692,853.724528157963,124.046654297545));
#74321=CARTESIAN_POINT('Origin',(69.6336697168692,849.663175330685,134.03732951327));
#74322=CARTESIAN_POINT('Origin',(67.1130950497633,863.001142136143,127.325323559515));
#74323=CARTESIAN_POINT('',(67.1130950497633,861.213426689515,138.119579156005));
#74324=CARTESIAN_POINT('Origin',(67.1130950497633,859.411211539474,137.482615342506));
#74325=CARTESIAN_POINT('',(67.1130950497633,861.879892958583,136.23389023357));
#74326=CARTESIAN_POINT('',(67.1130950497633,864.803357286184,127.962287373014));
#74327=CARTESIAN_POINT('Origin',(67.1130950497633,860.077677808543,135.596926420071));
#74328=CARTESIAN_POINT('Origin',(67.1130950497633,863.001142136143,127.325323559515));
#74329=CARTESIAN_POINT('',(67.1130950497633,861.337725504637,133.532218803004));
#74330=CARTESIAN_POINT('Origin',(67.1130950497633,860.866303274028,133.365602235737));
#74331=CARTESIAN_POINT('',(67.1130950497633,859.882633770083,137.649231909774));
#74332=CARTESIAN_POINT('',(67.1130950497633,863.472564366752,127.491940126782));
#74333=CARTESIAN_POINT('Origin',(67.1130950497633,859.411211539474,137.482615342506));
#74334=CARTESIAN_POINT('Origin',(64.535989506944,867.34749087047,128.861470264612));
#74335=CARTESIAN_POINT('',(64.535989506944,865.218659089599,139.535163806621));
#74336=CARTESIAN_POINT('Origin',(64.535989506944,863.757560273801,139.018762047603));
#74337=CARTESIAN_POINT('',(64.535989506944,865.885125358667,137.649474884186));
#74338=CARTESIAN_POINT('',(64.535989506944,868.808589686267,129.377872023629));
#74339=CARTESIAN_POINT('Origin',(64.535989506944,864.424026542869,137.133073125168));
#74340=CARTESIAN_POINT('Origin',(64.535989506944,867.34749087047,128.861470264612));
#74341=CARTESIAN_POINT('',(64.535989506944,865.684074238963,135.068365508101));
#74342=CARTESIAN_POINT('Origin',(64.535989506944,865.212652008354,134.901748940833));
#74343=CARTESIAN_POINT('',(64.535989506944,864.22898250441,139.185378614871));
#74344=CARTESIAN_POINT('',(64.535989506944,867.818913101078,129.028086831879));
#74345=CARTESIAN_POINT('Origin',(64.535989506944,863.757560273801,139.018762047603));
#74346=CARTESIAN_POINT('Origin',(60.8630998560088,871.993282576964,130.50345024798));
#74347=CARTESIAN_POINT('',(60.8630998560088,869.590733557258,141.080402856329));
#74348=CARTESIAN_POINT('Origin',(60.8630998560088,868.403351980296,140.660742030971));
#74349=CARTESIAN_POINT('',(60.8630998553805,870.247232404664,139.222915596134));
#74350=CARTESIAN_POINT('',(60.8630998560088,873.180664153927,130.923111073338));
#74351=CARTESIAN_POINT('',(59.7764391413702,868.469678153389,138.56294329237));
#74352=CARTESIAN_POINT('Ctrl Pts',(60.8630998547522,870.247232404664,139.222915596134));
#74353=CARTESIAN_POINT('Ctrl Pts',(60.7125947473751,870.247480485245,139.222213680484));
#74354=CARTESIAN_POINT('Ctrl Pts',(60.5631969146961,870.222538914215,139.211814297784));
#74355=CARTESIAN_POINT('Ctrl Pts',(60.2693839823579,870.120362912388,139.171234662913));
#74356=CARTESIAN_POINT('Ctrl Pts',(60.1292552058059,870.040035870772,139.139918832405));
#74357=CARTESIAN_POINT('Ctrl Pts',(59.8884371282248,869.83262025715,139.060478110665));
#74358=CARTESIAN_POINT('Ctrl Pts',(59.7904667251912,869.707062656979,139.012964631227));
#74359=CARTESIAN_POINT('Ctrl Pts',(59.655842546834,869.435669372995,138.911726169822));
#74360=CARTESIAN_POINT('Ctrl Pts',(59.6170281227853,869.293795614435,138.859406339753));
#74361=CARTESIAN_POINT('Ctrl Pts',(59.5963321478785,869.005806462867,138.754429774482));
#74362=CARTESIAN_POINT('Ctrl Pts',(59.6137541520704,868.86217278406,138.702657616607));
#74363=CARTESIAN_POINT('Ctrl Pts',(59.6867899608931,868.63555738197,138.621704815602));
#74364=CARTESIAN_POINT('Ctrl Pts',(59.7265814003054,868.549929814254,138.591306944703));
#74365=CARTESIAN_POINT('Ctrl Pts',(59.7764391413706,868.469678153389,138.562943292371));
#74366=CARTESIAN_POINT('',(61.6663922313285,868.155350700384,138.451849334943));
#74367=CARTESIAN_POINT('Origin',(60.8630998560082,869.069818249365,138.775053108536));
#74368=CARTESIAN_POINT('Ctrl Pts',(61.6663922313285,868.155350700384,138.451849334943));
#74369=CARTESIAN_POINT('Ctrl Pts',(61.7818905477588,868.245541265504,138.483725732331));
#74370=CARTESIAN_POINT('Ctrl Pts',(61.8794185589124,868.35439508296,138.522514240186));
#74371=CARTESIAN_POINT('Ctrl Pts',(62.0302871197043,868.600772687965,138.611292047399));
#74372=CARTESIAN_POINT('Ctrl Pts',(62.0817213966495,868.736600600712,138.66068881566));
#74373=CARTESIAN_POINT('Ctrl Pts',(62.1314065564681,869.023492700691,138.766021662923));
#74374=CARTESIAN_POINT('Ctrl Pts',(62.1273049061047,869.172391866978,138.821195816889));
#74375=CARTESIAN_POINT('Ctrl Pts',(62.0587821129058,869.469558973426,138.932061525383));
#74376=CARTESIAN_POINT('Ctrl Pts',(61.9913905992417,869.614301017483,138.98647510785));
#74377=CARTESIAN_POINT('Ctrl Pts',(61.8006559518915,869.870089012991,139.082854244429));
#74378=CARTESIAN_POINT('Ctrl Pts',(61.6794339224592,869.978778294368,139.123915712022));
#74379=CARTESIAN_POINT('Ctrl Pts',(61.399851307555,870.145341289405,139.186475194636));
#74380=CARTESIAN_POINT('Ctrl Pts',(61.2444721746654,870.201953729592,139.207493364977));
#74381=CARTESIAN_POINT('Ctrl Pts',(61.0818698441341,870.228996928008,139.217051346327));
#74382=CARTESIAN_POINT('Ctrl Pts',(61.0223987728464,870.238887856235,139.220547135031));
#74383=CARTESIAN_POINT('Ctrl Pts',(60.9622504386777,870.244774465707,139.222494950591));
#74384=CARTESIAN_POINT('Ctrl Pts',(60.8889550432104,870.24700405361,139.222964720184));
#74385=CARTESIAN_POINT('Ctrl Pts',(60.8760233670833,870.247211102579,139.222975867947));
#74386=CARTESIAN_POINT('Ctrl Pts',(60.8630998547522,870.247232404664,139.222915596135));
#74387=CARTESIAN_POINT('Origin',(60.8630998560088,871.993282576964,130.50345024798));
#74388=CARTESIAN_POINT('',(60.8630998560088,870.329865945458,136.710345491468));
#74389=CARTESIAN_POINT('Origin',(60.8630998560088,869.858443714849,136.543728924201));
#74390=CARTESIAN_POINT('',(60.8630998560088,868.874774210905,140.827358598238));
#74391=CARTESIAN_POINT('',(60.8630998560088,872.464704807573,130.670066815247));
#74392=CARTESIAN_POINT('Origin',(60.8630998560088,868.403351980296,140.660742030971));
#74393=CARTESIAN_POINT('Origin',(65.6573249397971,834.228980040933,117.156267944625));
#74394=CARTESIAN_POINT('',(65.6573249397971,831.637411863391,127.666414786973));
#74395=CARTESIAN_POINT('Origin',(65.6573249397971,830.639049444264,127.313559727617));
#74396=CARTESIAN_POINT('',(65.6573249397971,832.30387813246,125.780725864538));
#74397=CARTESIAN_POINT('',(65.6573249397971,835.22734246006,117.509123003982));
#74398=CARTESIAN_POINT('Origin',(65.6573249397971,831.305515713332,125.427870805181));
#74399=CARTESIAN_POINT('Origin',(65.6573249397971,834.228980040933,117.156267944625));
#74400=CARTESIAN_POINT('',(65.6573249397971,832.565563409427,123.363163188114));
#74401=CARTESIAN_POINT('Origin',(65.6573249397971,832.094141178818,123.196546620847));
#74402=CARTESIAN_POINT('',(65.6573249397971,831.110471674873,127.480176294884));
#74403=CARTESIAN_POINT('',(65.6573249397971,834.700402271542,117.322884511892));
#74404=CARTESIAN_POINT('Origin',(65.6573249397971,830.639049444264,127.313559727617));
#74405=CARTESIAN_POINT('Origin',(68.5805335751996,837.054171108743,118.154786060719));
#74406=CARTESIAN_POINT('',(68.5805335751996,834.686009791457,128.743892446641));
#74407=CARTESIAN_POINT('Origin',(68.5805335751996,833.464240512074,128.31207784371));
#74408=CARTESIAN_POINT('',(68.5805335751996,835.352476060525,126.858203524206));
#74409=CARTESIAN_POINT('',(68.5805335751996,838.275940388125,118.58660066365));
#74410=CARTESIAN_POINT('Origin',(68.5805335751996,834.130706781142,126.426388921275));
#74411=CARTESIAN_POINT('Origin',(68.5805335751996,837.054171108743,118.154786060719));
#74412=CARTESIAN_POINT('',(68.5805335751996,835.390754477236,124.361681304207));
#74413=CARTESIAN_POINT('Origin',(68.5805335751996,834.919332246628,124.19506473694));
#74414=CARTESIAN_POINT('',(68.5805335751996,833.935662742683,128.478694410977));
#74415=CARTESIAN_POINT('',(68.5805335751996,837.525593339351,118.321402627986));
#74416=CARTESIAN_POINT('Origin',(68.5805335751996,833.464240512074,128.31207784371));
#74417=CARTESIAN_POINT('Origin',(71.3370026852042,840.702101604493,119.444088128731));
#74418=CARTESIAN_POINT('',(71.3370026852042,838.626887409825,130.1367319399));
#74419=CARTESIAN_POINT('Origin',(71.3370026852042,837.112171007824,129.601379911722));
#74420=CARTESIAN_POINT('',(71.3370026852042,839.293353678893,128.251043017465));
#74421=CARTESIAN_POINT('',(71.3370026852042,842.216818006494,119.979440156909));
#74422=CARTESIAN_POINT('Origin',(71.3370026852042,837.778637276893,127.715690989287));
#74423=CARTESIAN_POINT('Origin',(71.3370026852042,840.702101604493,119.444088128731));
#74424=CARTESIAN_POINT('',(71.3370026852042,839.038684972987,125.650983372219));
#74425=CARTESIAN_POINT('Origin',(71.3370026852042,838.567262742378,125.484366804952));
#74426=CARTESIAN_POINT('',(71.3370026852042,837.583593238433,129.76799647899));
#74427=CARTESIAN_POINT('',(71.3370026852042,841.173523835102,119.610704695998));
#74428=CARTESIAN_POINT('Origin',(71.3370026852042,837.112171007824,129.601379911722));
#74429=CARTESIAN_POINT('Origin',(73.1579114734415,844.797493313962,120.8915381299));
#74430=CARTESIAN_POINT('',(73.1579114734415,842.93117486174,131.658012764614));
#74431=CARTESIAN_POINT('Origin',(73.1579114734415,841.207562717293,131.048829912891));
#74432=CARTESIAN_POINT('',(73.1579114734415,843.597641130808,129.772323842179));
#74433=CARTESIAN_POINT('',(73.1579114734415,846.521105458408,121.500720981622));
#74434=CARTESIAN_POINT('Origin',(73.1579114734415,841.874028986361,129.163140990456));
#74435=CARTESIAN_POINT('Origin',(73.1579114734415,844.797493313962,120.8915381299));
#74436=CARTESIAN_POINT('',(73.1579114734415,843.134076682455,127.098433373388));
#74437=CARTESIAN_POINT('Origin',(73.1579114734415,842.662654451847,126.931816806121));
#74438=CARTESIAN_POINT('',(73.1579114734415,841.678984947902,131.215446480159));
#74439=CARTESIAN_POINT('',(73.1579114734415,845.268915544571,121.058154697167));
#74440=CARTESIAN_POINT('Origin',(73.1579114734415,841.207562717293,131.048829912891));
#74441=CARTESIAN_POINT('Origin',(74.547161632643,849.445246854869,122.53421149193));
#74442=CARTESIAN_POINT('',(74.547161632643,847.607515655762,133.310789829168));
#74443=CARTESIAN_POINT('Origin',(74.547161632643,845.855316258201,132.691503274921));
#74444=CARTESIAN_POINT('',(74.547161632643,848.27398192483,131.425100906733));
#74445=CARTESIAN_POINT('',(74.547161632643,851.197446252431,123.153498046176));
#74446=CARTESIAN_POINT('Origin',(74.547161632643,846.521782527269,130.805814352486));
#74447=CARTESIAN_POINT('Origin',(74.547161632643,849.445246854869,122.53421149193));
#74448=CARTESIAN_POINT('',(74.547161632643,847.781830223363,128.741106735418));
#74449=CARTESIAN_POINT('Origin',(74.547161632643,847.310407992754,128.574490168151));
#74450=CARTESIAN_POINT('',(74.547161632643,846.32673848881,132.858119842188));
#74451=CARTESIAN_POINT('',(74.547161632643,849.916669085478,122.700828059197));
#74452=CARTESIAN_POINT('Origin',(74.547161632643,845.855316258201,132.691503274921));
#74453=CARTESIAN_POINT('Origin',(74.5993171469355,853.932897983989,124.120299244432));
#74454=CARTESIAN_POINT('',(74.5993171469355,852.052209735701,134.881695107002));
#74455=CARTESIAN_POINT('Origin',(74.5993171469355,850.342967387321,134.277591027424));
#74456=CARTESIAN_POINT('',(74.5993171469355,852.718676004769,132.996006184567));
#74457=CARTESIAN_POINT('',(74.5993171469355,855.64214033237,124.724403324011));
#74458=CARTESIAN_POINT('Origin',(74.5993171469355,851.009433656389,132.391902104989));
#74459=CARTESIAN_POINT('Origin',(74.5993171469355,853.932897983989,124.120299244432));
#74460=CARTESIAN_POINT('',(74.5993171469355,852.269481352483,130.327194487921));
#74461=CARTESIAN_POINT('Origin',(74.5993171469355,851.798059121874,130.160577920654));
#74462=CARTESIAN_POINT('',(74.5993171469355,850.814389617929,134.444207594691));
#74463=CARTESIAN_POINT('',(74.5993171469355,854.404320214598,124.2869158117));
#74464=CARTESIAN_POINT('Origin',(74.5993171469355,850.342967387321,134.277591027424));
#74465=CARTESIAN_POINT('Origin',(74.2312593354051,859.474369268425,126.07884269672));
#74466=CARTESIAN_POINT('',(74.2312593354051,857.686653821797,136.87309829321));
#74467=CARTESIAN_POINT('Origin',(74.2312593354051,855.884438671756,136.236134479712));
#74468=CARTESIAN_POINT('',(74.2312593354051,858.353120090865,134.987409370775));
#74469=CARTESIAN_POINT('',(74.2312593354051,861.276584418465,126.715806510219));
#74470=CARTESIAN_POINT('Origin',(74.2312593354051,856.550904940825,134.350445557277));
#74471=CARTESIAN_POINT('Origin',(74.2312593354051,859.474369268425,126.07884269672));
#74472=CARTESIAN_POINT('',(74.2312593354051,857.810952636918,132.285737940209));
#74473=CARTESIAN_POINT('Origin',(74.2312593354051,857.33953040631,132.119121372942));
#74474=CARTESIAN_POINT('',(74.2312593354051,856.355860902365,136.402751046979));
#74475=CARTESIAN_POINT('',(74.2312593354051,859.945791499033,126.245459263987));
#74476=CARTESIAN_POINT('Origin',(74.2312593354051,855.884438671756,136.236134479712));
#74477=CARTESIAN_POINT('Origin',(72.6689064108742,864.230925695252,127.759970680072));
#74478=CARTESIAN_POINT('',(72.6689064108742,862.102093914381,138.43366422208));
#74479=CARTESIAN_POINT('Origin',(72.6689064108742,860.640995098584,137.917262463063));
#74480=CARTESIAN_POINT('',(72.6689064108742,862.76856018345,136.547975299645));
#74481=CARTESIAN_POINT('',(72.6689064108742,865.69202451105,128.276372439089));
#74482=CARTESIAN_POINT('Origin',(72.6689064108742,861.307461367652,136.031573540628));
#74483=CARTESIAN_POINT('Origin',(72.6689064108742,864.230925695252,127.759970680072));
#74484=CARTESIAN_POINT('',(72.6689064108742,862.567509063746,133.96686592356));
#74485=CARTESIAN_POINT('Origin',(72.6689064108742,862.096086833137,133.800249356293));
#74486=CARTESIAN_POINT('',(72.6689064108742,861.112417329193,138.08387903033));
#74487=CARTESIAN_POINT('',(72.6689064108742,864.702347925861,127.926587247339));
#74488=CARTESIAN_POINT('Origin',(72.6689064108742,860.640995098584,137.917262463063));
#74489=CARTESIAN_POINT('Origin',(70.1007466664717,869.495186337102,129.620538511613));
#74490=CARTESIAN_POINT('',(70.1007466664717,867.092637317396,140.197491119963));
#74491=CARTESIAN_POINT('Origin',(70.1007466664717,865.905255740434,139.777830294604));
#74492=CARTESIAN_POINT('',(70.1007466531591,867.749813505509,138.338087402883));
#74493=CARTESIAN_POINT('',(70.1007466664717,870.682567914064,130.040199336972));
#74494=CARTESIAN_POINT('',(68.9054919831167,866.197712760658,137.759953848708));
#74495=CARTESIAN_POINT('Ctrl Pts',(70.1007466531577,867.749813505464,138.338087403012));
#74496=CARTESIAN_POINT('Ctrl Pts',(70.0385698236016,867.750027222959,138.337482712201));
#74497=CARTESIAN_POINT('Ctrl Pts',(69.976342079479,867.745935464751,138.335242039916));
#74498=CARTESIAN_POINT('Ctrl Pts',(69.7533901561324,867.715524071811,138.321283246897));
#74499=CARTESIAN_POINT('Ctrl Pts',(69.5984074925223,867.664441672665,138.300303462554));
#74500=CARTESIAN_POINT('Ctrl Pts',(69.3166886230872,867.508807874702,138.23916418655));
#74501=CARTESIAN_POINT('Ctrl Pts',(69.1929543752343,867.405220528364,138.199415738199));
#74502=CARTESIAN_POINT('Ctrl Pts',(69.0010571598675,867.166184517323,138.109613431888));
#74503=CARTESIAN_POINT('Ctrl Pts',(68.9316547620308,867.035034715326,138.061083810922));
#74504=CARTESIAN_POINT('Ctrl Pts',(68.8476838970957,866.757417727942,137.959773119425));
#74505=CARTESIAN_POINT('Ctrl Pts',(68.8329819766983,866.613514497137,137.907905692754));
#74506=CARTESIAN_POINT('Ctrl Pts',(68.8543900681979,866.37753999295,137.823645068394));
#74507=CARTESIAN_POINT('Ctrl Pts',(68.874420477635,866.285984262706,137.791151984273));
#74508=CARTESIAN_POINT('Ctrl Pts',(68.9054919831215,866.197712760659,137.759953848709));
#74509=CARTESIAN_POINT('',(70.6848310304297,865.51976966261,137.52034581908));
#74510=CARTESIAN_POINT('Origin',(70.1007466664716,866.571722009503,137.892141372169));
#74511=CARTESIAN_POINT('Ctrl Pts',(70.6848310304297,865.51976966261,137.52034581908));
#74512=CARTESIAN_POINT('Ctrl Pts',(70.8176938369516,865.585348398922,137.543523563405));
#74513=CARTESIAN_POINT('Ctrl Pts',(70.937116451913,865.672703071882,137.574713546154));
#74514=CARTESIAN_POINT('Ctrl Pts',(71.1391359754987,865.884110545421,137.651131725662));
#74515=CARTESIAN_POINT('Ctrl Pts',(71.2194947760908,866.006878166671,137.695912545002));
#74516=CARTESIAN_POINT('Ctrl Pts',(71.3316309737503,866.277734264315,137.795577726448));
#74517=CARTESIAN_POINT('Ctrl Pts',(71.3606300520131,866.424166171532,137.849879867578));
#74518=CARTESIAN_POINT('Ctrl Pts',(71.3595389505574,866.728231802344,137.963183747999));
#74519=CARTESIAN_POINT('Ctrl Pts',(71.325763592196,866.882999174463,138.021140620618));
#74520=CARTESIAN_POINT('Ctrl Pts',(71.1960161043892,867.170545970834,138.128744392009));
#74521=CARTESIAN_POINT('Ctrl Pts',(71.1015941158648,867.300604915829,138.177358621785));
#74522=CARTESIAN_POINT('Ctrl Pts',(70.8651064396571,867.518308900674,138.257993060595));
#74523=CARTESIAN_POINT('Ctrl Pts',(70.7256765621508,867.604136013465,138.289336684738));
#74524=CARTESIAN_POINT('Ctrl Pts',(70.5725909234467,867.662462925543,138.309951389007));
#74525=CARTESIAN_POINT('Ctrl Pts',(70.5166005394062,867.683795731382,138.317491124404));
#74526=CARTESIAN_POINT('Ctrl Pts',(70.4590554838378,867.70134539635,138.323561058407));
#74527=CARTESIAN_POINT('Ctrl Pts',(70.3021079592237,867.737816799193,138.335750016227));
#74528=CARTESIAN_POINT('Ctrl Pts',(70.2014941359312,867.749467210873,138.339067206542));
#74529=CARTESIAN_POINT('Ctrl Pts',(70.1007466531577,867.749813505464,138.338087403012));
#74530=CARTESIAN_POINT('Origin',(70.1007466664717,869.495186337102,129.620538511613));
#74531=CARTESIAN_POINT('',(70.1007466664717,867.831769705596,135.827433755101));
#74532=CARTESIAN_POINT('Origin',(70.1007466664717,867.360347474987,135.660817187834));
#74533=CARTESIAN_POINT('',(70.1007466664717,866.376677971043,139.944446861871));
#74534=CARTESIAN_POINT('',(70.1007466664717,869.966608567711,129.78715507888));
#74535=CARTESIAN_POINT('Origin',(70.1007466664717,865.905255740434,139.777830294604));
#74536=CARTESIAN_POINT('Origin',(66.4625974592707,831.616320212274,116.232865559622));
#74537=CARTESIAN_POINT('',(66.4625974592707,829.024752034733,126.74301240197));
#74538=CARTESIAN_POINT('Origin',(66.4625974592707,828.026389615606,126.390157342613));
#74539=CARTESIAN_POINT('',(66.4625974592707,829.691218303801,124.857323479535));
#74540=CARTESIAN_POINT('',(66.4625974592707,832.614682631402,116.585720618979));
#74541=CARTESIAN_POINT('Origin',(66.4625974592707,828.692855884674,124.504468420178));
#74542=CARTESIAN_POINT('Origin',(66.4625974592707,831.616320212274,116.232865559622));
#74543=CARTESIAN_POINT('',(66.4625974592707,829.952903580768,122.43976080311));
#74544=CARTESIAN_POINT('Origin',(66.4625974592707,829.481481350159,122.273144235843));
#74545=CARTESIAN_POINT('',(66.4625974592707,828.497811846215,126.55677390988));
#74546=CARTESIAN_POINT('',(66.4625974592707,832.087742442883,116.399482126889));
#74547=CARTESIAN_POINT('Origin',(66.4625974592707,828.026389615606,126.390157342613));
#74548=CARTESIAN_POINT('Origin',(69.9449250128882,833.806742205807,117.007034806917));
#74549=CARTESIAN_POINT('',(69.9449250128882,831.438580888521,127.59614119284));
#74550=CARTESIAN_POINT('Origin',(69.9449250128882,830.216811609138,127.164326589909));
#74551=CARTESIAN_POINT('',(69.9449250128882,832.105047157589,125.710452270404));
#74552=CARTESIAN_POINT('',(69.9449250128882,835.028511485189,117.438849409848));
#74553=CARTESIAN_POINT('Origin',(69.9449250128882,830.883277878207,125.278637667474));
#74554=CARTESIAN_POINT('Origin',(69.9449250128882,833.806742205807,117.007034806917));
#74555=CARTESIAN_POINT('',(69.9449250128882,832.1433255743,123.213930050406));
#74556=CARTESIAN_POINT('Origin',(69.9449250128882,831.671903343692,123.047313483139));
#74557=CARTESIAN_POINT('',(69.9449250128882,830.688233839747,127.330943157176));
#74558=CARTESIAN_POINT('',(69.9449250128882,834.278164436415,117.173651374185));
#74559=CARTESIAN_POINT('Origin',(69.9449250128882,830.216811609138,127.164326589909));
#74560=CARTESIAN_POINT('Origin',(73.4455833853166,836.834610476873,118.077185904396));
#74561=CARTESIAN_POINT('',(73.4455833853166,834.759396282205,128.769829715565));
#74562=CARTESIAN_POINT('Origin',(73.4455833853166,833.244679880204,128.234477687388));
#74563=CARTESIAN_POINT('',(73.4455833853166,835.425862551273,126.88414079313));
#74564=CARTESIAN_POINT('',(73.4455833853166,838.349326878873,118.612537932574));
#74565=CARTESIAN_POINT('Origin',(73.4455833853166,833.911146149272,126.348788764952));
#74566=CARTESIAN_POINT('Origin',(73.4455833853166,836.834610476873,118.077185904396));
#74567=CARTESIAN_POINT('',(73.4455833853166,835.171193845366,124.284081147885));
#74568=CARTESIAN_POINT('Origin',(73.4455833853166,834.699771614758,124.117464580618));
#74569=CARTESIAN_POINT('',(73.4455833853166,833.716102110813,128.401094254655));
#74570=CARTESIAN_POINT('',(73.4455833853166,837.306032707481,118.243802471663));
#74571=CARTESIAN_POINT('Origin',(73.4455833853166,833.244679880204,128.234477687388));
#74572=CARTESIAN_POINT('Origin',(76.129797746682,840.483558240543,119.366847509312));
#74573=CARTESIAN_POINT('',(76.129797746682,838.617239788321,130.133322144025));
#74574=CARTESIAN_POINT('Origin',(76.129797746682,836.893627643875,129.524139292303));
#74575=CARTESIAN_POINT('',(76.129797746682,839.28370605739,128.24763322159));
#74576=CARTESIAN_POINT('',(76.129797746682,842.20717038499,119.976030361034));
#74577=CARTESIAN_POINT('Origin',(76.129797746682,837.560093912943,127.638450369868));
#74578=CARTESIAN_POINT('Origin',(76.129797746682,840.483558240543,119.366847509312));
#74579=CARTESIAN_POINT('',(76.129797746682,838.820141609037,125.5737427528));
#74580=CARTESIAN_POINT('Origin',(76.129797746682,838.348719378428,125.407126185533));
#74581=CARTESIAN_POINT('',(76.129797746682,837.365049874483,129.69075585957));
#74582=CARTESIAN_POINT('',(76.129797746682,840.954980471152,119.533464076579));
#74583=CARTESIAN_POINT('Origin',(76.129797746682,836.893627643875,129.524139292303));
#74584=CARTESIAN_POINT('Origin',(78.5135905267759,844.757414748773,120.87737300887));
#74585=CARTESIAN_POINT('',(78.5135905267759,842.919683549666,131.653951346109));
#74586=CARTESIAN_POINT('Origin',(78.5135905267759,841.167484152104,131.034664791862));
#74587=CARTESIAN_POINT('',(78.5135905267759,843.586149818734,129.768262423673));
#74588=CARTESIAN_POINT('',(78.5135905267759,846.509614146334,121.496659563117));
#74589=CARTESIAN_POINT('Origin',(78.5135905267759,841.833950421173,129.148975869426));
#74590=CARTESIAN_POINT('Origin',(78.5135905267759,844.757414748773,120.87737300887));
#74591=CARTESIAN_POINT('',(78.5135905267759,843.093998117266,127.084268252359));
#74592=CARTESIAN_POINT('Origin',(78.5135905267759,842.622575886658,126.917651685091));
#74593=CARTESIAN_POINT('',(78.5135905267759,841.638906382713,131.201281359129));
#74594=CARTESIAN_POINT('',(78.5135905267759,845.228836979382,121.043989576137));
#74595=CARTESIAN_POINT('Origin',(78.5135905267759,841.167484152104,131.034664791862));
#74596=CARTESIAN_POINT('Origin',(79.5542023461718,849.136775972358,122.425187444677));
#74597=CARTESIAN_POINT('',(79.5542023461718,847.25608772407,133.186583307246));
#74598=CARTESIAN_POINT('Origin',(79.5542023461718,845.54684537569,132.582479227668));
#74599=CARTESIAN_POINT('',(79.5542023461718,847.922553993138,131.300894384811));
#74600=CARTESIAN_POINT('',(79.5542023461718,850.846018320739,123.029291524255));
#74601=CARTESIAN_POINT('Origin',(79.5542023461718,846.213311644758,130.696790305233));
#74602=CARTESIAN_POINT('Origin',(79.5542023461718,849.136775972358,122.425187444677));
#74603=CARTESIAN_POINT('',(79.5542023461718,847.473359340852,128.632082688165));
#74604=CARTESIAN_POINT('Origin',(79.5542023461718,847.001937110243,128.465466120898));
#74605=CARTESIAN_POINT('',(79.5542023461718,846.018267606298,132.749095794935));
#74606=CARTESIAN_POINT('',(79.5542023461718,849.608198202967,122.591804011944));
#74607=CARTESIAN_POINT('Origin',(79.5542023461718,845.54684537569,132.582479227668));
#74608=CARTESIAN_POINT('Origin',(80.4161670456629,854.629302592554,124.366432196538));
#74609=CARTESIAN_POINT('',(80.4161670456629,852.841587145926,135.160687793028));
#74610=CARTESIAN_POINT('Origin',(80.4161670456629,851.039371995885,134.523723979529));
#74611=CARTESIAN_POINT('',(80.4161670456629,853.508053414994,133.274998870593));
#74612=CARTESIAN_POINT('',(80.4161670456629,856.431517742594,125.003396010037));
#74613=CARTESIAN_POINT('Origin',(80.4161670456629,851.705838264953,132.638035057094));
#74614=CARTESIAN_POINT('Origin',(80.4161670456629,854.629302592554,124.366432196538));
#74615=CARTESIAN_POINT('',(80.4161670456629,852.965885961047,130.573327440026));
#74616=CARTESIAN_POINT('Origin',(80.4161670456629,852.494463730438,130.406710872759));
#74617=CARTESIAN_POINT('',(80.4161670456629,851.510794226494,134.690340546796));
#74618=CARTESIAN_POINT('',(80.4161670456629,855.100724823162,124.533048763805));
#74619=CARTESIAN_POINT('Origin',(80.4161670456629,851.039371995885,134.523723979529));
#74620=CARTESIAN_POINT('Origin',(79.9368490592233,859.58818237154,126.119068098324));
#74621=CARTESIAN_POINT('',(79.9368490592233,857.459350590669,136.792761640332));
#74622=CARTESIAN_POINT('Origin',(79.9368490592233,855.998251774872,136.276359881315));
#74623=CARTESIAN_POINT('',(79.9368490592233,858.125816859737,134.907072717897));
#74624=CARTESIAN_POINT('',(79.9368490592233,861.049281187338,126.635469857341));
#74625=CARTESIAN_POINT('Origin',(79.9368490592233,856.66471804394,134.39067095888));
#74626=CARTESIAN_POINT('Origin',(79.9368490592233,859.58818237154,126.119068098324));
#74627=CARTESIAN_POINT('',(79.9368490592233,857.924765740034,132.325963341812));
#74628=CARTESIAN_POINT('Origin',(79.9368490592233,857.453343509425,132.159346774545));
#74629=CARTESIAN_POINT('',(79.9368490592233,856.46967400548,136.442976448582));
#74630=CARTESIAN_POINT('',(79.9368490592233,860.059604602149,126.285684665591));
#74631=CARTESIAN_POINT('Origin',(79.9368490592233,855.998251774872,136.276359881315));
#74632=CARTESIAN_POINT('Origin',(78.5856601255815,865.24083849797,128.116908035806));
#74633=CARTESIAN_POINT('',(78.5856601255815,862.838289478264,138.693860644156));
#74634=CARTESIAN_POINT('Origin',(78.5856601255815,861.650907901302,138.274199818797));
#74635=CARTESIAN_POINT('',(78.5856601240841,863.496566482291,136.831342296269));
#74636=CARTESIAN_POINT('',(78.5856601255815,866.428220074932,128.536568861164));
#74637=CARTESIAN_POINT('',(77.3340498386503,862.185841767529,136.342022894688));
#74638=CARTESIAN_POINT('Ctrl Pts',(78.5856601225867,863.496566482291,136.831342296269));
#74639=CARTESIAN_POINT('Ctrl Pts',(78.4486937731582,863.497227928007,136.829470811441));
#74640=CARTESIAN_POINT('Ctrl Pts',(78.3124648687431,863.476938862574,136.819817687594));
#74641=CARTESIAN_POINT('Ctrl Pts',(78.0264738654205,863.387571443878,136.782579786376));
#74642=CARTESIAN_POINT('Ctrl Pts',(77.8823835531221,863.310524693534,136.752211682673));
#74643=CARTESIAN_POINT('Ctrl Pts',(77.6416001298824,863.114366012403,136.677563675543));
#74644=CARTESIAN_POINT('Ctrl Pts',(77.5446429760725,862.999701933924,136.634860667076));
#74645=CARTESIAN_POINT('Ctrl Pts',(77.4010671508439,862.744634128623,136.541519619498));
#74646=CARTESIAN_POINT('Ctrl Pts',(77.3548838503261,862.606764437272,136.49178464982));
#74647=CARTESIAN_POINT('Ctrl Pts',(77.3237285881768,862.371755847929,136.407865412448));
#74648=CARTESIAN_POINT('Ctrl Pts',(77.3231225426296,862.278275222544,136.374692005254));
#74649=CARTESIAN_POINT('Ctrl Pts',(77.3340498386502,862.185841767529,136.342022894688));
#74650=CARTESIAN_POINT('',(78.9250091887252,861.173912390952,135.984372813519));
#74651=CARTESIAN_POINT('Origin',(78.5856601255815,862.317374170371,136.388510896363));
#74652=CARTESIAN_POINT('Ctrl Pts',(78.9250091887252,861.173912390953,135.984372813519));
#74653=CARTESIAN_POINT('Ctrl Pts',(79.0694297431482,861.212013193,135.997838926136));
#74654=CARTESIAN_POINT('Ctrl Pts',(79.2055276205897,861.274046565504,136.020079504536));
#74655=CARTESIAN_POINT('Ctrl Pts',(79.4498688843905,861.441221048167,136.080864248408));
#74656=CARTESIAN_POINT('Ctrl Pts',(79.5556401434395,861.545543748934,136.11912600875));
#74657=CARTESIAN_POINT('Ctrl Pts',(79.7253264890131,861.78847209321,136.208920577197));
#74658=CARTESIAN_POINT('Ctrl Pts',(79.786158897029,861.926001974476,136.260076441147));
#74659=CARTESIAN_POINT('Ctrl Pts',(79.8525471736859,862.223596854638,136.371093339346));
#74660=CARTESIAN_POINT('Ctrl Pts',(79.8538641158598,862.381580756675,136.430187042472));
#74661=CARTESIAN_POINT('Ctrl Pts',(79.7907743754111,862.688237133456,136.544544786168));
#74662=CARTESIAN_POINT('Ctrl Pts',(79.72727912178,862.83394519488,136.598689943191));
#74663=CARTESIAN_POINT('Ctrl Pts',(79.5442220305133,863.093224784922,136.694018607624));
#74664=CARTESIAN_POINT('Ctrl Pts',(79.4268351630958,863.204501652834,136.734357036341));
#74665=CARTESIAN_POINT('Ctrl Pts',(79.2899567932164,863.291563112634,136.765127502032));
#74666=CARTESIAN_POINT('Ctrl Pts',(79.2398941448767,863.323405450102,136.776381661506));
#74667=CARTESIAN_POINT('Ctrl Pts',(79.1874673629681,863.351852988318,136.786303272653));
#74668=CARTESIAN_POINT('Ctrl Pts',(78.9856966443786,863.443980354888,136.817891881721));
#74669=CARTESIAN_POINT('Ctrl Pts',(78.8258553722391,863.483846736233,136.830316759686));
#74670=CARTESIAN_POINT('Ctrl Pts',(78.6368967142923,863.495587022015,136.831770148258));
#74671=CARTESIAN_POINT('Ctrl Pts',(78.6112655323327,863.496442827184,136.831692164219));
#74672=CARTESIAN_POINT('Ctrl Pts',(78.5856601225867,863.496566482291,136.831342296269));
#74673=CARTESIAN_POINT('Origin',(78.5856601255815,865.24083849797,128.116908035806));
#74674=CARTESIAN_POINT('',(78.5856601255815,863.577421866464,134.323803279294));
#74675=CARTESIAN_POINT('Origin',(78.5856601255815,863.105999635855,134.157186712027));
#74676=CARTESIAN_POINT('',(78.5856601255815,862.122330131911,138.440816386064));
#74677=CARTESIAN_POINT('',(78.5856601255815,865.712260728579,128.283524603073));
#74678=CARTESIAN_POINT('Origin',(78.5856601255815,861.650907901302,138.274199818797));
#74679=CARTESIAN_POINT('Origin',(66.6741412055227,828.902896996967,115.273849984363));
#74680=CARTESIAN_POINT('',(66.6741412055227,826.311328819426,125.783996826711));
#74681=CARTESIAN_POINT('Origin',(66.6741412055227,825.312966400299,125.431141767354));
#74682=CARTESIAN_POINT('',(66.6741412055227,826.977795088494,123.898307904275));
#74683=CARTESIAN_POINT('',(66.6741412055227,829.901259416094,115.626705043719));
#74684=CARTESIAN_POINT('Origin',(66.6741412055227,825.979432669367,123.545452844919));
#74685=CARTESIAN_POINT('Origin',(66.6741412055227,828.902896996967,115.273849984363));
#74686=CARTESIAN_POINT('',(66.6741412055227,827.239480365461,121.480745227851));
#74687=CARTESIAN_POINT('Origin',(66.6741412055227,826.768058134852,121.314128660584));
#74688=CARTESIAN_POINT('',(66.6741412055227,825.784388630908,125.597758334621));
#74689=CARTESIAN_POINT('',(66.6741412055227,829.374319227576,115.44046655163));
#74690=CARTESIAN_POINT('Origin',(66.6741412055227,825.312966400299,125.431141767354));
#74691=CARTESIAN_POINT('Origin',(70.5633932532005,830.362817964294,115.789835451877));
#74692=CARTESIAN_POINT('',(70.5633932532005,827.994656647008,126.378941837799));
#74693=CARTESIAN_POINT('Origin',(70.5633932532005,826.772887367626,125.947127234868));
#74694=CARTESIAN_POINT('',(70.5633932532005,828.661122916077,124.493252915364));
#74695=CARTESIAN_POINT('',(70.5633932532005,831.584587243677,116.221650054808));
#74696=CARTESIAN_POINT('Origin',(70.5633932532005,827.439353636694,124.061438312433));
#74697=CARTESIAN_POINT('Origin',(70.5633932532005,830.362817964294,115.789835451877));
#74698=CARTESIAN_POINT('',(70.5633932532005,828.699401332788,121.996730695365));
#74699=CARTESIAN_POINT('Origin',(70.5633932532005,828.227979102179,121.830114128098));
#74700=CARTESIAN_POINT('',(70.5633932532005,827.244309598234,126.113743802135));
#74701=CARTESIAN_POINT('',(70.5633932532005,830.834240194903,115.956452019144));
#74702=CARTESIAN_POINT('Origin',(70.5633932532005,826.772887367626,125.947127234868));
#74703=CARTESIAN_POINT('Origin',(74.6552453191549,832.638291637906,116.594064840708));
#74704=CARTESIAN_POINT('',(74.6552453191549,830.563077443238,127.286708651877));
#74705=CARTESIAN_POINT('Origin',(74.6552453191549,829.048361041238,126.751356623699));
#74706=CARTESIAN_POINT('',(74.6552453191549,831.229543712306,125.401019729442));
#74707=CARTESIAN_POINT('',(74.6552453191549,834.153008039907,117.129416868886));
#74708=CARTESIAN_POINT('Origin',(74.6552453191549,829.714827310306,124.865667701264));
#74709=CARTESIAN_POINT('Origin',(74.6552453191549,832.638291637906,116.594064840708));
#74710=CARTESIAN_POINT('',(74.6552453191549,830.9748750064,122.800960084196));
#74711=CARTESIAN_POINT('Origin',(74.6552453191549,830.503452775791,122.634343516929));
#74712=CARTESIAN_POINT('',(74.6552453191549,829.519783271846,126.917973190966));
#74713=CARTESIAN_POINT('',(74.6552453191549,833.109713868515,116.760681407975));
#74714=CARTESIAN_POINT('Origin',(74.6552453191549,829.048361041238,126.751356623699));
#74715=CARTESIAN_POINT('Origin',(78.0854522057672,835.681318928912,117.669573648752));
#74716=CARTESIAN_POINT('',(78.0854522057672,833.81500047669,128.436048283466));
#74717=CARTESIAN_POINT('Origin',(78.0854522057672,832.091388332243,127.826865431743));
#74718=CARTESIAN_POINT('',(78.0854522057672,834.481466745758,126.55035936103));
#74719=CARTESIAN_POINT('',(78.0854522057672,837.404931073359,118.278756500474));
#74720=CARTESIAN_POINT('Origin',(78.0854522057672,832.757854601311,125.941176509308));
#74721=CARTESIAN_POINT('Origin',(78.0854522057672,835.681318928912,117.669573648752));
#74722=CARTESIAN_POINT('',(78.0854522057672,834.017902297405,123.87646889224));
#74723=CARTESIAN_POINT('Origin',(78.0854522057672,833.546480066797,123.709852324973));
#74724=CARTESIAN_POINT('',(78.0854522057672,832.562810562852,127.99348199901));
#74725=CARTESIAN_POINT('',(78.0854522057672,836.152741159521,117.836190216019));
#74726=CARTESIAN_POINT('Origin',(78.0854522057672,832.091388332243,127.826865431743));
#74727=CARTESIAN_POINT('Origin',(81.3596044235566,839.394490366815,118.981934073203));
#74728=CARTESIAN_POINT('',(81.3596044235566,837.556759167708,129.758512410442));
#74729=CARTESIAN_POINT('Origin',(81.3596044235566,835.804559770147,129.139225856195));
#74730=CARTESIAN_POINT('',(81.3596044235566,838.223225436777,127.872823488007));
#74731=CARTESIAN_POINT('',(81.3596044235566,841.146689764377,119.601220627451));
#74732=CARTESIAN_POINT('Origin',(81.3596044235566,836.471026039215,127.25353693376));
#74733=CARTESIAN_POINT('Origin',(81.3596044235566,839.394490366815,118.981934073203));
#74734=CARTESIAN_POINT('',(81.3596044235566,837.731073735309,125.188829316692));
#74735=CARTESIAN_POINT('Origin',(81.3596044235566,837.2596515047,125.022212749425));
#74736=CARTESIAN_POINT('',(81.3596044235566,836.275982000755,129.305842423462));
#74737=CARTESIAN_POINT('',(81.3596044235566,839.865912597424,119.148550640471));
#74738=CARTESIAN_POINT('Origin',(81.3596044235566,835.804559770147,129.139225856195));
#74739=CARTESIAN_POINT('Origin',(83.343192818139,843.474162584889,120.423828274231));
#74740=CARTESIAN_POINT('',(83.343192818139,841.5934743366,131.185224136801));
#74741=CARTESIAN_POINT('Origin',(83.343192818139,839.88423198822,130.581120057222));
#74742=CARTESIAN_POINT('',(83.343192818139,842.259940605669,129.299535214366));
#74743=CARTESIAN_POINT('',(83.343192818139,845.183404933269,121.027932353809));
#74744=CARTESIAN_POINT('Origin',(83.343192818139,840.550698257288,128.695431134787));
#74745=CARTESIAN_POINT('Origin',(83.343192818139,843.474162584889,120.423828274231));
#74746=CARTESIAN_POINT('',(83.343192818139,841.810745953382,126.630723517719));
#74747=CARTESIAN_POINT('Origin',(83.343192818139,841.339323722773,126.464106950452));
#74748=CARTESIAN_POINT('',(83.343192818139,840.355654218829,130.747736624489));
#74749=CARTESIAN_POINT('',(83.343192818139,843.945584815497,120.590444841498));
#74750=CARTESIAN_POINT('Origin',(83.343192818139,839.88423198822,130.581120057222));
#74751=CARTESIAN_POINT('Origin',(85.3975080351181,848.677694771475,122.262932614884));
#74752=CARTESIAN_POINT('',(85.3975080351181,846.889979324847,133.057188211373));
#74753=CARTESIAN_POINT('Origin',(85.3975080351181,845.087764174806,132.420224397875));
#74754=CARTESIAN_POINT('',(85.3975080351181,847.556445593915,131.171499288938));
#74755=CARTESIAN_POINT('',(85.3975080351181,850.479909921515,122.899896428382));
#74756=CARTESIAN_POINT('Origin',(85.3975080351181,845.754230443874,130.53453547544));
#74757=CARTESIAN_POINT('Origin',(85.3975080351181,848.677694771475,122.262932614884));
#74758=CARTESIAN_POINT('',(85.3975080351181,847.014278139968,128.469827858372));
#74759=CARTESIAN_POINT('Origin',(85.3975080351181,846.542855909359,128.303211291105));
#74760=CARTESIAN_POINT('',(85.3975080351181,845.559186405414,132.586840965142));
#74761=CARTESIAN_POINT('',(85.3975080351181,849.149117002083,122.429549182151));
#74762=CARTESIAN_POINT('Origin',(85.3975080351181,845.087764174806,132.420224397875));
#74763=CARTESIAN_POINT('Origin',(86.0221734828003,853.622171060933,124.010477836116));
#74764=CARTESIAN_POINT('',(86.0221734828003,851.493339280062,134.684171378124));
#74765=CARTESIAN_POINT('Origin',(86.0221734828003,850.032240464264,134.167769619107));
#74766=CARTESIAN_POINT('',(86.0221734828003,852.15980554913,132.798482455689));
#74767=CARTESIAN_POINT('',(86.0221734828003,855.08326987673,124.526879595133));
#74768=CARTESIAN_POINT('Origin',(86.0221734828003,850.698706733332,132.282080696672));
#74769=CARTESIAN_POINT('Origin',(86.0221734828003,853.622171060933,124.010477836116));
#74770=CARTESIAN_POINT('',(86.0221734828003,851.958754429426,130.217373079604));
#74771=CARTESIAN_POINT('Origin',(86.0221734828003,851.487332198818,130.050756512337));
#74772=CARTESIAN_POINT('',(86.0221734828003,850.503662694873,134.334386186374));
#74773=CARTESIAN_POINT('',(86.0221734828003,854.093593291541,124.177094403383));
#74774=CARTESIAN_POINT('Origin',(86.0221734828003,850.032240464264,134.167769619107));
#74775=CARTESIAN_POINT('Origin',(85.9470088000432,859.416174474765,126.058274687571));
#74776=CARTESIAN_POINT('',(85.9470088000432,857.013625455059,136.635227295921));
#74777=CARTESIAN_POINT('Origin',(85.9470088000432,855.826243878096,136.215566470562));
#74778=CARTESIAN_POINT('',(85.9470087966831,857.673301053105,134.768751788653));
#74779=CARTESIAN_POINT('',(85.9470088000432,860.603556051727,126.477935512929));
#74780=CARTESIAN_POINT('',(84.6937442849622,856.609403187493,134.371120816987));
#74781=CARTESIAN_POINT('Ctrl Pts',(85.9470087933229,857.673301053105,134.768751788653));
#74782=CARTESIAN_POINT('Ctrl Pts',(85.898177953993,857.673578244451,134.767967507141));
#74783=CARTESIAN_POINT('Ctrl Pts',(85.8492938279539,857.671185445707,134.76621509686));
#74784=CARTESIAN_POINT('Ctrl Pts',(85.6371334459491,857.649028772594,134.754384637898));
#74785=CARTESIAN_POINT('Ctrl Pts',(85.4789845072744,857.601933009003,134.734602226331));
#74786=CARTESIAN_POINT('Ctrl Pts',(85.1998382671642,857.457297769682,134.678164346876));
#74787=CARTESIAN_POINT('Ctrl Pts',(85.0795638502545,857.364160676451,134.64306970338));
#74788=CARTESIAN_POINT('Ctrl Pts',(84.8826580172478,857.142833563675,134.561653758185));
#74789=CARTESIAN_POINT('Ctrl Pts',(84.8070117684544,857.017036808601,134.516185772685));
#74790=CARTESIAN_POINT('Ctrl Pts',(84.7246547871115,856.79327693593,134.436242212395));
#74791=CARTESIAN_POINT('Ctrl Pts',(84.7034387736784,856.701958809946,134.40383310566));
#74792=CARTESIAN_POINT('Ctrl Pts',(84.6937442849618,856.609403187493,134.371120816987));
#74793=CARTESIAN_POINT('',(86.0267913799356,855.307713701921,133.911059709021));
#74794=CARTESIAN_POINT('Origin',(85.9470088000436,856.492710147166,134.329877548128));
#74795=CARTESIAN_POINT('Ctrl Pts',(86.0267913799356,855.307713701921,133.911059709021));
#74796=CARTESIAN_POINT('Ctrl Pts',(86.1764578110232,855.316671381824,133.914225656189));
#74797=CARTESIAN_POINT('Ctrl Pts',(86.3232828206312,855.350667960248,133.926557082913));
#74798=CARTESIAN_POINT('Ctrl Pts',(86.5992669389399,855.466279786581,133.969117839372));
#74799=CARTESIAN_POINT('Ctrl Pts',(86.7258279448786,855.547579069414,133.999242344799));
#74800=CARTESIAN_POINT('Ctrl Pts',(86.9456483308198,855.751908486123,134.075394746216));
#74801=CARTESIAN_POINT('Ctrl Pts',(87.0356554004524,855.874490635807,134.121267576057));
#74802=CARTESIAN_POINT('Ctrl Pts',(87.1666215689656,856.15252829316,134.225372289979));
#74803=CARTESIAN_POINT('Ctrl Pts',(87.2029732549826,856.30677934918,134.283146679019));
#74804=CARTESIAN_POINT('Ctrl Pts',(87.2092985862878,856.619060905553,134.399492551516));
#74805=CARTESIAN_POINT('Ctrl Pts',(87.1795051148179,856.774013594738,134.456905072789));
#74806=CARTESIAN_POINT('Ctrl Pts',(87.0578790817858,857.063486351916,134.5629050241));
#74807=CARTESIAN_POINT('Ctrl Pts',(86.9676655938481,857.195335781048,134.610514492041));
#74808=CARTESIAN_POINT('Ctrl Pts',(86.8529767343722,857.307326785008,134.650095902151));
#74809=CARTESIAN_POINT('Ctrl Pts',(86.8110297996916,857.348286991164,134.66457262493));
#74810=CARTESIAN_POINT('Ctrl Pts',(86.7660125933822,857.386390931025,134.677907135151));
#74811=CARTESIAN_POINT('Ctrl Pts',(86.5888991837206,857.516064557618,134.722765862921));
#74812=CARTESIAN_POINT('Ctrl Pts',(86.4412266028949,857.586404622667,134.745961171809));
#74813=CARTESIAN_POINT('Ctrl Pts',(86.1737258624385,857.65758596838,134.767165773978));
#74814=CARTESIAN_POINT('Ctrl Pts',(86.0605112696524,857.672656749122,134.770574773776));
#74815=CARTESIAN_POINT('Ctrl Pts',(85.9470087933229,857.673301053105,134.768751788653));
#74816=CARTESIAN_POINT('Origin',(85.9470088000432,859.416174474765,126.058274687571));
#74817=CARTESIAN_POINT('',(85.9470088000432,857.752757843259,132.265169931059));
#74818=CARTESIAN_POINT('Origin',(85.9470088000432,857.28133561265,132.098553363792));
#74819=CARTESIAN_POINT('',(85.9470088000432,856.297666108705,136.382183037829));
#74820=CARTESIAN_POINT('',(85.9470088000432,859.887596705374,126.224891254838));
#74821=CARTESIAN_POINT('Origin',(85.9470088000432,855.826243878096,136.215566470562));
#74822=CARTESIAN_POINT('Origin',(66.2827107017424,826.207300009971,114.321134801354));
#74823=CARTESIAN_POINT('',(66.2827107017424,823.61573183243,124.831281643702));
#74824=CARTESIAN_POINT('Origin',(66.2827107017424,822.617369413302,124.478426584345));
#74825=CARTESIAN_POINT('',(66.2827107017424,824.282198101498,122.945592721267));
#74826=CARTESIAN_POINT('',(66.2827107017424,827.205662429098,114.67398986071));
#74827=CARTESIAN_POINT('Origin',(66.2827107017424,823.283835682371,122.59273766191));
#74828=CARTESIAN_POINT('Origin',(66.2827107017424,826.207300009971,114.321134801354));
#74829=CARTESIAN_POINT('',(66.2827107017424,824.543883378465,120.528030044842));
#74830=CARTESIAN_POINT('Origin',(66.2827107017424,824.072461147856,120.361413477575));
#74831=CARTESIAN_POINT('',(66.2827107017424,823.088791643911,124.645043151612));
#74832=CARTESIAN_POINT('',(66.2827107017424,826.67872224058,114.487751368621));
#74833=CARTESIAN_POINT('Origin',(66.2827107017424,822.617369413302,124.478426584345));
#74834=CARTESIAN_POINT('Origin',(70.4089082662952,826.872914399342,114.556385448183));
#74835=CARTESIAN_POINT('',(70.4089082662952,824.504753082056,125.145491834106));
#74836=CARTESIAN_POINT('Origin',(70.4089082662952,823.282983802673,124.713677231175));
#74837=CARTESIAN_POINT('',(70.4089082662952,825.171219351124,123.259802911671));
#74838=CARTESIAN_POINT('',(70.4089082662952,828.094683678724,114.988200051114));
#74839=CARTESIAN_POINT('Origin',(70.4089082662952,823.949450071741,122.82798830874));
#74840=CARTESIAN_POINT('Origin',(70.4089082662952,826.872914399342,114.556385448183));
#74841=CARTESIAN_POINT('',(70.4089082662952,825.209497767835,120.763280691672));
#74842=CARTESIAN_POINT('Origin',(70.4089082662952,824.738075537226,120.596664124405));
#74843=CARTESIAN_POINT('',(70.4089082662952,823.754406033282,124.880293798442));
#74844=CARTESIAN_POINT('',(70.4089082662952,827.34433662995,114.723002015451));
#74845=CARTESIAN_POINT('Origin',(70.4089082662952,823.282983802673,124.713677231175));
#74846=CARTESIAN_POINT('Origin',(74.9131204556088,828.296544357029,115.059544444954));
#74847=CARTESIAN_POINT('',(74.9131204556088,826.22133016236,125.752188256123));
#74848=CARTESIAN_POINT('Origin',(74.9131204556088,824.70661376036,125.216836227945));
#74849=CARTESIAN_POINT('',(74.9131204556088,826.887796431429,123.866499333688));
#74850=CARTESIAN_POINT('',(74.9131204556088,829.811260759029,115.594896473132));
#74851=CARTESIAN_POINT('Origin',(74.9131204556088,825.373080029428,123.33114730551));
#74852=CARTESIAN_POINT('Origin',(74.9131204556088,828.296544357029,115.059544444954));
#74853=CARTESIAN_POINT('',(74.9131204556088,826.633127725522,121.266439688442));
#74854=CARTESIAN_POINT('Origin',(74.9131204556088,826.161705494914,121.099823121175));
#74855=CARTESIAN_POINT('',(74.9131204556088,825.178035990969,125.383452795212));
#74856=CARTESIAN_POINT('',(74.9131204556088,828.767966587637,115.226161012221));
#74857=CARTESIAN_POINT('Origin',(74.9131204556088,824.70661376036,125.216836227945));
#74858=CARTESIAN_POINT('Origin',(78.9394033665642,830.600656280688,115.873895560351));
#74859=CARTESIAN_POINT('',(78.9394033665642,828.734337828466,126.640370195065));
#74860=CARTESIAN_POINT('Origin',(78.9394033665642,827.010725684019,126.031187343342));
#74861=CARTESIAN_POINT('',(78.9394033665642,829.400804097534,124.754681272629));
#74862=CARTESIAN_POINT('',(78.9394033665642,832.324268425134,116.483078412073));
#74863=CARTESIAN_POINT('Origin',(78.9394033665642,827.677191953087,124.145498420907));
#74864=CARTESIAN_POINT('Origin',(78.9394033665642,830.600656280688,115.873895560351));
#74865=CARTESIAN_POINT('',(78.9394033665642,828.937239649181,122.080790803839));
#74866=CARTESIAN_POINT('Origin',(78.9394033665642,828.465817418573,121.914174236572));
#74867=CARTESIAN_POINT('',(78.9394033665642,827.482147914628,126.197803910609));
#74868=CARTESIAN_POINT('',(78.9394033665642,831.072078511296,116.040512127618));
#74869=CARTESIAN_POINT('Origin',(78.9394033665642,827.010725684019,126.031187343342));
#74870=CARTESIAN_POINT('Origin',(82.9608188590062,833.590859238655,116.930734461743));
#74871=CARTESIAN_POINT('',(82.9608188590062,831.753128039548,127.707312798981));
#74872=CARTESIAN_POINT('Origin',(82.9608188590062,830.000928641986,127.088026244734));
#74873=CARTESIAN_POINT('',(82.9608188590062,832.419594308616,125.821623876546));
#74874=CARTESIAN_POINT('',(82.9608188590062,835.343058636216,117.55002101599));
#74875=CARTESIAN_POINT('Origin',(82.9608188590062,830.667394911054,125.202337322299));
#74876=CARTESIAN_POINT('Origin',(82.9608188590062,833.590859238655,116.930734461743));
#74877=CARTESIAN_POINT('',(82.9608188590062,831.927442607148,123.137629705231));
#74878=CARTESIAN_POINT('Origin',(82.9608188590062,831.45602037654,122.971013137964));
#74879=CARTESIAN_POINT('',(82.9608188590062,830.472350872595,127.254642812001));
#74880=CARTESIAN_POINT('',(82.9608188590062,834.062281469263,117.09735102901));
#74881=CARTESIAN_POINT('Origin',(82.9608188590062,830.000928641986,127.088026244734));
#74882=CARTESIAN_POINT('Origin',(85.8006914976185,837.192541198847,118.203690732431));
#74883=CARTESIAN_POINT('',(85.8006914976185,835.311852950559,128.965086595));
#74884=CARTESIAN_POINT('Origin',(85.8006914976185,833.602610602179,128.360982515422));
#74885=CARTESIAN_POINT('',(85.8006914976185,835.978319219627,127.079397672565));
#74886=CARTESIAN_POINT('',(85.8006914976185,838.901783547228,118.807794812009));
#74887=CARTESIAN_POINT('Origin',(85.8006914976185,834.269076871247,126.475293592987));
#74888=CARTESIAN_POINT('Origin',(85.8006914976185,837.192541198847,118.203690732431));
#74889=CARTESIAN_POINT('',(85.8006914976185,835.529124567341,124.410585975919));
#74890=CARTESIAN_POINT('Origin',(85.8006914976185,835.057702336732,124.243969408652));
#74891=CARTESIAN_POINT('',(85.8006914976185,834.074032832787,128.527599082689));
#74892=CARTESIAN_POINT('',(85.8006914976185,837.663963429456,118.370307299698));
#74893=CARTESIAN_POINT('Origin',(85.8006914976185,833.602610602179,128.360982515422));
#74894=CARTESIAN_POINT('Origin',(88.9575737994055,841.879659625952,119.860276977186));
#74895=CARTESIAN_POINT('',(88.9575737994055,840.091944179324,130.654532573676));
#74896=CARTESIAN_POINT('Origin',(88.9575737994055,838.289729029283,130.017568760178));
#74897=CARTESIAN_POINT('',(88.9575737994055,840.758410448393,128.768843651241));
#74898=CARTESIAN_POINT('',(88.9575737994055,843.681874775993,120.497240790685));
#74899=CARTESIAN_POINT('Origin',(88.9575737994055,838.956195298352,128.131879837743));
#74900=CARTESIAN_POINT('Origin',(88.9575737994055,841.879659625952,119.860276977186));
#74901=CARTESIAN_POINT('',(88.9575737994055,840.216242994446,126.067172220675));
#74902=CARTESIAN_POINT('Origin',(88.9575737994055,839.744820763837,125.900555653408));
#74903=CARTESIAN_POINT('',(88.9575737994055,838.761151259892,130.184185327445));
#74904=CARTESIAN_POINT('',(88.9575737994055,842.351081856561,120.026893544454));
#74905=CARTESIAN_POINT('Origin',(88.9575737994055,838.289729029283,130.017568760178));
#74906=CARTESIAN_POINT('Origin',(90.6589218036684,846.593635085803,121.526355406045));
#74907=CARTESIAN_POINT('',(90.6589218036684,844.464803304932,132.200048948054));
#74908=CARTESIAN_POINT('Origin',(90.6589218036684,843.003704489134,131.683647189036));
#74909=CARTESIAN_POINT('',(90.6589218036684,845.131269574,130.314360025618));
#74910=CARTESIAN_POINT('',(90.6589218036684,848.054733901601,122.042757165062));
#74911=CARTESIAN_POINT('Origin',(90.6589218036684,843.670170758203,129.797958266601));
#74912=CARTESIAN_POINT('Origin',(90.6589218036684,846.593635085803,121.526355406045));
#74913=CARTESIAN_POINT('',(90.6589218036684,844.930218454297,127.733250649533));
#74914=CARTESIAN_POINT('Origin',(90.6589218036684,844.458796223688,127.566634082266));
#74915=CARTESIAN_POINT('',(90.6589218036684,843.475126719743,131.850263756303));
#74916=CARTESIAN_POINT('',(90.6589218036684,847.065057316412,121.692971973312));
#74917=CARTESIAN_POINT('Origin',(90.6589218036684,843.003704489134,131.683647189036));
#74918=CARTESIAN_POINT('Origin',(91.8630664291128,852.27576003514,123.534610622645));
#74919=CARTESIAN_POINT('',(91.8630664291128,849.873211015433,134.111563230994));
#74920=CARTESIAN_POINT('Origin',(91.8630664291128,848.685829438471,133.691902405636));
#74921=CARTESIAN_POINT('',(91.8630664387515,850.534428209482,132.240725956837));
#74922=CARTESIAN_POINT('',(91.8630664291128,853.463141612102,123.954271448003));
#74923=CARTESIAN_POINT('',(90.662921359021,849.712114145219,131.933385493838));
#74924=CARTESIAN_POINT('Ctrl Pts',(91.8630664483903,850.534428209482,132.240725956837));
#74925=CARTESIAN_POINT('Ctrl Pts',(91.737992335004,850.53516728595,132.238634831534));
#74926=CARTESIAN_POINT('Ctrl Pts',(91.6133872467039,850.518326302074,132.230365038877));
#74927=CARTESIAN_POINT('Ctrl Pts',(91.3454402966626,850.442220816991,132.198798790733));
#74928=CARTESIAN_POINT('Ctrl Pts',(91.2071051858126,850.374711138186,132.17276174262));
#74929=CARTESIAN_POINT('Ctrl Pts',(90.9654750747892,850.196841598205,132.106705174074));
#74930=CARTESIAN_POINT('Ctrl Pts',(90.8636719817834,850.088629530986,132.067452212255));
#74931=CARTESIAN_POINT('Ctrl Pts',(90.7337126765244,849.885909553918,131.994944862974));
#74932=CARTESIAN_POINT('Ctrl Pts',(90.6928139367984,849.800746810279,131.964711276631));
#74933=CARTESIAN_POINT('Ctrl Pts',(90.6629213590209,849.712114145219,131.933385493838));
#74934=CARTESIAN_POINT('',(91.6797956441728,848.17755462737,131.391020237111));
#74935=CARTESIAN_POINT('Origin',(91.8630664291131,849.35229570754,131.806213483201));
#74936=CARTESIAN_POINT('Ctrl Pts',(91.6797956441728,848.17755462737,131.391020237111));
#74937=CARTESIAN_POINT('Ctrl Pts',(91.8281668107091,848.156977691535,131.383747651749));
#74938=CARTESIAN_POINT('Ctrl Pts',(91.9793019950186,848.161447324691,131.385643256946));
#74939=CARTESIAN_POINT('Ctrl Pts',(92.2748671375464,848.220420364746,131.408185949913));
#74940=CARTESIAN_POINT('Ctrl Pts',(92.416686567108,848.275123966036,131.428910641595));
#74941=CARTESIAN_POINT('Ctrl Pts',(92.6770337877353,848.431870239332,131.488245550114));
#74942=CARTESIAN_POINT('Ctrl Pts',(92.7922817781397,848.534112239401,131.526929482854));
#74943=CARTESIAN_POINT('Ctrl Pts',(92.9821019884994,848.780360946266,131.619798906068));
#74944=CARTESIAN_POINT('Ctrl Pts',(93.051899675246,848.924092923618,131.673855496785));
#74945=CARTESIAN_POINT('Ctrl Pts',(93.1273636309746,849.228269411424,131.787336763809));
#74946=CARTESIAN_POINT('Ctrl Pts',(93.1325740593341,849.385658205106,131.845610286839));
#74947=CARTESIAN_POINT('Ctrl Pts',(93.0776947258065,849.692622105076,131.95779219984));
#74948=CARTESIAN_POINT('Ctrl Pts',(93.0185973796637,849.83926778188,132.010631162352));
#74949=CARTESIAN_POINT('Ctrl Pts',(92.9311104840889,849.971293785735,132.057293619326));
#74950=CARTESIAN_POINT('Ctrl Pts',(92.8991125453979,850.019581703019,132.074360203157));
#74951=CARTESIAN_POINT('Ctrl Pts',(92.8634723826217,850.065678541835,132.090519674315));
#74952=CARTESIAN_POINT('Ctrl Pts',(92.7187569877708,850.227244420114,132.146650202932));
#74953=CARTESIAN_POINT('Ctrl Pts',(92.5897070986527,850.325006836843,132.179537498763));
#74954=CARTESIAN_POINT('Ctrl Pts',(92.2999886674533,850.468659422292,132.225657717503));
#74955=CARTESIAN_POINT('Ctrl Pts',(92.1421864000932,850.513398291368,132.238544411543));
#74956=CARTESIAN_POINT('Ctrl Pts',(91.9410083713401,850.532263460595,132.241428886593));
#74957=CARTESIAN_POINT('Ctrl Pts',(91.9020146658181,850.534198060251,132.241377135573));
#74958=CARTESIAN_POINT('Ctrl Pts',(91.8630664483903,850.534428209482,132.240725956837));
#74959=CARTESIAN_POINT('Origin',(91.8630664291128,852.27576003514,123.534610622645));
#74960=CARTESIAN_POINT('',(91.8630664291128,850.612343403633,129.741505866133));
#74961=CARTESIAN_POINT('Origin',(91.8630664291128,850.140921173025,129.574889298866));
#74962=CARTESIAN_POINT('',(91.8630664291128,849.15725166908,133.858518972903));
#74963=CARTESIAN_POINT('',(91.8630664291128,852.747182265749,123.701227189912));
#74964=CARTESIAN_POINT('Origin',(91.8630664291128,848.685829438471,133.691902405636));
#74965=CARTESIAN_POINT('Origin',(65.305413339237,823.647339774524,113.416358235727));
#74966=CARTESIAN_POINT('',(65.305413339237,821.055771596983,123.926505078075));
#74967=CARTESIAN_POINT('Origin',(65.305413339237,820.057409177856,123.573650018718));
#74968=CARTESIAN_POINT('',(65.305413339237,821.722237866051,122.04081615564));
#74969=CARTESIAN_POINT('',(65.305413339237,824.645702193652,113.769213295084));
#74970=CARTESIAN_POINT('Origin',(65.305413339237,820.723875446924,121.687961096283));
#74971=CARTESIAN_POINT('Origin',(65.305413339237,823.647339774524,113.416358235727));
#74972=CARTESIAN_POINT('',(65.305413339237,821.983923143018,119.623253479215));
#74973=CARTESIAN_POINT('Origin',(65.305413339237,821.512500912409,119.456636911948));
#74974=CARTESIAN_POINT('',(65.305413339237,820.528831408465,123.740266585986));
#74975=CARTESIAN_POINT('',(65.305413339237,824.118762005133,113.582974802994));
#74976=CARTESIAN_POINT('Origin',(65.305413339237,820.057409177856,123.573650018718));
#74977=CARTESIAN_POINT('Origin',(69.488221787401,823.489557043151,113.360592479748));
#74978=CARTESIAN_POINT('',(69.488221787401,821.121395725865,123.94969886567));
#74979=CARTESIAN_POINT('Origin',(69.488221787401,819.899626446483,123.517884262739));
#74980=CARTESIAN_POINT('',(69.488221787401,821.787861994934,122.064009943235));
#74981=CARTESIAN_POINT('',(69.488221787401,824.711326322534,113.792407082679));
#74982=CARTESIAN_POINT('Origin',(69.488221787401,820.566092715551,121.632195340304));
#74983=CARTESIAN_POINT('Origin',(69.488221787401,823.489557043151,113.360592479748));
#74984=CARTESIAN_POINT('',(69.488221787401,821.826140411645,119.567487723236));
#74985=CARTESIAN_POINT('Origin',(69.488221787401,821.354718181036,119.400871155969));
#74986=CARTESIAN_POINT('',(69.488221787401,820.371048677091,123.684500830006));
#74987=CARTESIAN_POINT('',(69.488221787401,823.96097927376,113.527209047015));
#74988=CARTESIAN_POINT('Origin',(69.488221787401,819.899626446483,123.517884262739));
#74989=CARTESIAN_POINT('Origin',(74.2079384137928,823.999123824428,113.540690621874));
#74990=CARTESIAN_POINT('',(74.2079384137928,821.92390962976,124.233334433043));
#74991=CARTESIAN_POINT('Origin',(74.2079384137928,820.409193227759,123.697982404865));
#74992=CARTESIAN_POINT('',(74.2079384137928,822.590375898829,122.347645510608));
#74993=CARTESIAN_POINT('',(74.2079384137928,825.513840226429,114.076042650052));
#74994=CARTESIAN_POINT('Origin',(74.2079384137928,821.075659496828,121.81229348243));
#74995=CARTESIAN_POINT('Origin',(74.2079384137928,823.999123824428,113.540690621874));
#74996=CARTESIAN_POINT('',(74.2079384137928,822.335707192922,119.747585865362));
#74997=CARTESIAN_POINT('Origin',(74.2079384137928,821.864284962313,119.580969298095));
#74998=CARTESIAN_POINT('',(74.2079384137928,820.880615458369,123.864598972132));
#74999=CARTESIAN_POINT('',(74.2079384137928,824.470546055037,113.707307189141));
#75000=CARTESIAN_POINT('Origin',(74.2079384137928,820.409193227759,123.697982404865));
#75001=CARTESIAN_POINT('Origin',(78.6543294656336,825.463619633321,114.058292993191));
#75002=CARTESIAN_POINT('',(78.6543294656336,823.597301181099,124.824767627905));
#75003=CARTESIAN_POINT('Origin',(78.6543294656336,821.873689036652,124.215584776183));
#75004=CARTESIAN_POINT('',(78.6543294656336,824.263767450167,122.93907870547));
#75005=CARTESIAN_POINT('',(78.6543294656336,827.187231777768,114.667475844914));
#75006=CARTESIAN_POINT('Origin',(78.6543294656336,822.540155305721,122.329895853747));
#75007=CARTESIAN_POINT('Origin',(78.6543294656336,825.463619633321,114.058292993191));
#75008=CARTESIAN_POINT('',(78.6543294656336,823.800203001815,120.26518823668));
#75009=CARTESIAN_POINT('Origin',(78.6543294656336,823.328780771206,120.098571669412));
#75010=CARTESIAN_POINT('',(78.6543294656336,822.345111267261,124.38220134345));
#75011=CARTESIAN_POINT('',(78.6543294656336,825.93504186393,114.224909560458));
#75012=CARTESIAN_POINT('Origin',(78.6543294656336,821.873689036652,124.215584776183));
#75013=CARTESIAN_POINT('Origin',(83.2472530788159,827.600167893503,114.813421440257));
#75014=CARTESIAN_POINT('',(83.2472530788159,825.762436694396,125.589999777496));
#75015=CARTESIAN_POINT('Origin',(83.2472530788159,824.010237296834,124.970713223248));
#75016=CARTESIAN_POINT('',(83.2472530788159,826.428902963464,123.70431085506));
#75017=CARTESIAN_POINT('',(83.2472530788159,829.352367291064,115.432707994504));
#75018=CARTESIAN_POINT('Origin',(83.2472530788159,824.676703565902,123.085024300813));
#75019=CARTESIAN_POINT('Origin',(83.2472530788159,827.600167893503,114.813421440257));
#75020=CARTESIAN_POINT('',(83.2472530788159,825.936751261997,121.020316683746));
#75021=CARTESIAN_POINT('Origin',(83.2472530788159,825.465329031388,120.853700116478));
#75022=CARTESIAN_POINT('',(83.2472530788159,824.481659527443,125.137329790516));
#75023=CARTESIAN_POINT('',(83.2472530788159,828.071590124112,114.980038007524));
#75024=CARTESIAN_POINT('Origin',(83.2472530788159,824.010237296834,124.970713223248));
#75025=CARTESIAN_POINT('Origin',(90.940772381535,834.532303912436,117.263472864034));
#75026=CARTESIAN_POINT('',(90.940772381535,832.744588465808,128.057728460524));
#75027=CARTESIAN_POINT('Origin',(90.940772381535,830.942373315767,127.420764647026));
#75028=CARTESIAN_POINT('',(90.940772381535,833.411054734876,126.172039538089));
#75029=CARTESIAN_POINT('',(90.940772381535,836.334519062477,117.900436677533));
#75030=CARTESIAN_POINT('Origin',(90.940772381535,831.608839584836,125.53507572459));
#75031=CARTESIAN_POINT('Origin',(90.940772381535,834.532303912436,117.263472864034));
#75032=CARTESIAN_POINT('',(90.940772381535,832.86888728093,123.470368107523));
#75033=CARTESIAN_POINT('Origin',(90.940772381535,832.397465050321,123.303751540255));
#75034=CARTESIAN_POINT('',(90.940772381535,831.413795546376,127.587381214293));
#75035=CARTESIAN_POINT('',(90.940772381535,835.003726143045,117.430089431301));
#75036=CARTESIAN_POINT('Origin',(90.940772381535,830.942373315767,127.420764647026));
#75037=CARTESIAN_POINT('Origin',(93.6444458706187,838.80975519492,118.775268878447));
#75038=CARTESIAN_POINT('',(93.6444458706187,836.680923414049,129.448962420455));
#75039=CARTESIAN_POINT('Origin',(93.6444458706187,835.219824598252,128.932560661438));
#75040=CARTESIAN_POINT('',(93.6444458706187,837.347389683118,127.56327349802));
#75041=CARTESIAN_POINT('',(93.6444458706187,840.270854010718,119.291670637464));
#75042=CARTESIAN_POINT('Origin',(93.6444458706187,835.88629086732,127.046871739003));
#75043=CARTESIAN_POINT('Origin',(93.6444458706187,838.80975519492,118.775268878447));
#75044=CARTESIAN_POINT('',(93.6444458706187,837.146338563414,124.982164121935));
#75045=CARTESIAN_POINT('Origin',(93.6444458706187,836.674916332805,124.815547554668));
#75046=CARTESIAN_POINT('',(93.6444458706187,835.691246828861,129.099177228705));
#75047=CARTESIAN_POINT('',(93.6444458706187,839.281177425529,118.941885445714));
#75048=CARTESIAN_POINT('Origin',(93.6444458706187,835.219824598252,128.932560661438));
#75049=CARTESIAN_POINT('Origin',(96.0752729060054,844.131665553615,120.656212070548));
#75050=CARTESIAN_POINT('',(96.0752729060054,841.729116533909,131.233164678898));
#75051=CARTESIAN_POINT('Origin',(96.0752729060054,840.541734956947,130.813503853539));
#75052=CARTESIAN_POINT('',(96.075272915159,842.391856517098,129.358018849683));
#75053=CARTESIAN_POINT('',(96.0752729060054,845.319047130577,121.075872895907));
#75054=CARTESIAN_POINT('',(94.9806993794011,841.795419268718,129.135357656415));
#75055=CARTESIAN_POINT('Ctrl Pts',(96.0752729243125,842.391856517098,129.358018849683));
#75056=CARTESIAN_POINT('Ctrl Pts',(96.0381869450381,842.392062128276,129.357437098348));
#75057=CARTESIAN_POINT('Ctrl Pts',(96.0010576020752,842.390718482093,129.356322901975));
#75058=CARTESIAN_POINT('Ctrl Pts',(95.8098139198172,842.375727679237,129.347827179232));
#75059=CARTESIAN_POINT('Ctrl Pts',(95.6594640231771,842.336825803051,129.331901096533));
#75060=CARTESIAN_POINT('Ctrl Pts',(95.3836700294588,842.210231411673,129.283966900442));
#75061=CARTESIAN_POINT('Ctrl Pts',(95.2601593759105,842.124347248646,129.252605375448));
#75062=CARTESIAN_POINT('Ctrl Pts',(95.0882775919892,841.951538801714,129.190669772999));
#75063=CARTESIAN_POINT('Ctrl Pts',(95.0294835971499,841.876255303615,129.163927846303));
#75064=CARTESIAN_POINT('Ctrl Pts',(94.9806993794009,841.795419268718,129.135357656415));
#75065=CARTESIAN_POINT('',(95.6369585689663,840.095057333157,128.534392215203));
#75066=CARTESIAN_POINT('Origin',(96.0752729060063,841.208201226016,128.927814931105));
#75067=CARTESIAN_POINT('Ctrl Pts',(95.6369585689663,840.095057333157,128.534392215203));
#75068=CARTESIAN_POINT('Ctrl Pts',(95.7775499390088,840.045845092418,128.516998944188));
#75069=CARTESIAN_POINT('Ctrl Pts',(95.9263899652387,840.020588098312,128.508388153485));
#75070=CARTESIAN_POINT('Ctrl Pts',(96.2286185169781,840.020321608885,128.509993592314));
#75071=CARTESIAN_POINT('Ctrl Pts',(96.3794981805657,840.046019623926,128.520466728387));
#75072=CARTESIAN_POINT('Ctrl Pts',(96.6689938130533,840.14827814966,128.560543823279));
#75073=CARTESIAN_POINT('Ctrl Pts',(96.8044458340276,840.225676544221,128.590447185228));
#75074=CARTESIAN_POINT('Ctrl Pts',(97.0448240321836,840.429293902598,128.668249247419));
#75075=CARTESIAN_POINT('Ctrl Pts',(97.1450172258218,840.556180302845,128.716352041202));
#75076=CARTESIAN_POINT('Ctrl Pts',(97.286321668992,840.838875704314,128.822241165483));
#75077=CARTESIAN_POINT('Ctrl Pts',(97.3263082764593,840.991785609775,128.878931697869));
#75078=CARTESIAN_POINT('Ctrl Pts',(97.3405741326517,841.302774181318,128.992536065982));
#75079=CARTESIAN_POINT('Ctrl Pts',(97.315175765911,841.457793125225,129.048334424406));
#75080=CARTESIAN_POINT('Ctrl Pts',(97.2587144313823,841.604083959076,129.100038554963));
#75081=CARTESIAN_POINT('Ctrl Pts',(97.2380639521442,841.657589173793,129.118949108238));
#75082=CARTESIAN_POINT('Ctrl Pts',(97.2133584790335,841.709666080833,129.137222137847));
#75083=CARTESIAN_POINT('Ctrl Pts',(97.1073658561724,841.896076358022,129.20213351767));
#75084=CARTESIAN_POINT('Ctrl Pts',(97.0025787581668,842.017011306053,129.243210770125));
#75085=CARTESIAN_POINT('Ctrl Pts',(96.7505467043735,842.214349710098,129.308305373662));
#75086=CARTESIAN_POINT('Ctrl Pts',(96.6058557131205,842.289064737309,129.331786656256));
#75087=CARTESIAN_POINT('Ctrl Pts',(96.3286812613534,842.372289415152,129.355764731473));
#75088=CARTESIAN_POINT('Ctrl Pts',(96.2022312191795,842.39115263803,129.360010388238));
#75089=CARTESIAN_POINT('Ctrl Pts',(96.0752729243125,842.391856517098,129.358018849683));
#75090=CARTESIAN_POINT('Origin',(96.0752729060054,844.131665553615,120.656212070548));
#75091=CARTESIAN_POINT('',(96.0752729060054,842.468248922109,126.863107314036));
#75092=CARTESIAN_POINT('Origin',(96.0752729060054,841.9968266915,126.696490746769));
#75093=CARTESIAN_POINT('',(96.0752729060054,841.013157187555,130.980120420807));
#75094=CARTESIAN_POINT('',(96.0752729060054,844.603087784224,120.822828637815));
#75095=CARTESIAN_POINT('Origin',(96.0752729060054,840.541734956947,130.813503853539));
#75096=CARTESIAN_POINT('Origin',(63.7849617023409,821.33489883697,112.599063365));
#75097=CARTESIAN_POINT('',(63.7849617023409,818.743330659428,123.109210207348));
#75098=CARTESIAN_POINT('Origin',(63.7849617023409,817.744968240301,122.756355147991));
#75099=CARTESIAN_POINT('',(63.7849617023409,819.409796928497,121.223521284913));
#75100=CARTESIAN_POINT('',(63.7849617023409,822.333261256097,112.951918424357));
#75101=CARTESIAN_POINT('Origin',(63.7849617023409,818.41143450937,120.870666225556));
#75102=CARTESIAN_POINT('Origin',(63.7849617023409,821.33489883697,112.599063365));
#75103=CARTESIAN_POINT('',(63.7849617023409,819.671482205463,118.805958608488));
#75104=CARTESIAN_POINT('Origin',(63.7849617023409,819.200059974855,118.639342041221));
#75105=CARTESIAN_POINT('',(63.7849617023409,818.21639047091,122.922971715259));
#75106=CARTESIAN_POINT('',(63.7849617023409,821.806321067579,112.765679932267));
#75107=CARTESIAN_POINT('Origin',(63.7849617023409,817.744968240301,122.756355147991));
#75108=CARTESIAN_POINT('Origin',(67.8415722335897,820.36061484734,112.254718437342));
#75109=CARTESIAN_POINT('',(67.8415722335897,817.992453530053,122.843824823264));
#75110=CARTESIAN_POINT('Origin',(67.8415722335897,816.770684250671,122.412010220333));
#75111=CARTESIAN_POINT('',(67.8415722335897,818.658919799122,120.958135900829));
#75112=CARTESIAN_POINT('',(67.8415722335897,821.582384126722,112.686533040273));
#75113=CARTESIAN_POINT('Origin',(67.8415722335897,817.437150519739,120.526321297898));
#75114=CARTESIAN_POINT('Origin',(67.8415722335897,820.36061484734,112.254718437342));
#75115=CARTESIAN_POINT('',(67.8415722335897,818.697198215833,118.46161368083));
#75116=CARTESIAN_POINT('Origin',(67.8415722335897,818.225775985225,118.294997113563));
#75117=CARTESIAN_POINT('',(67.8415722335897,817.24210648128,122.5786267876));
#75118=CARTESIAN_POINT('',(67.8415722335897,820.832037077948,112.421335004609));
#75119=CARTESIAN_POINT('Origin',(67.8415722335897,816.770684250671,122.412010220333));
#75120=CARTESIAN_POINT('Origin',(72.5705190327731,819.933847938692,112.103884571806));
#75121=CARTESIAN_POINT('',(72.5705190327731,817.858633744024,122.796528382975));
#75122=CARTESIAN_POINT('Origin',(72.5705190327731,816.343917342023,122.261176354798));
#75123=CARTESIAN_POINT('',(72.5705190327731,818.525100013092,120.91083946054));
#75124=CARTESIAN_POINT('',(72.5705190327731,821.448564340692,112.639236599984));
#75125=CARTESIAN_POINT('Origin',(72.5705190327731,817.010383611091,120.375487432362));
#75126=CARTESIAN_POINT('Origin',(72.5705190327731,819.933847938692,112.103884571806));
#75127=CARTESIAN_POINT('',(72.5705190327731,818.270431307185,118.310779815295));
#75128=CARTESIAN_POINT('Origin',(72.5705190327731,817.799009076576,118.144163248028));
#75129=CARTESIAN_POINT('',(72.5705190327731,816.815339572632,122.427792922065));
#75130=CARTESIAN_POINT('',(72.5705190327731,820.4052701693,112.270501139073));
#75131=CARTESIAN_POINT('Origin',(72.5705190327731,816.343917342023,122.261176354798));
#75132=CARTESIAN_POINT('Origin',(77.2426896003823,820.494722138539,112.302116491685));
#75133=CARTESIAN_POINT('',(77.2426896003823,818.628403686317,123.068591126399));
#75134=CARTESIAN_POINT('Origin',(77.2426896003823,816.904791541871,122.459408274677));
#75135=CARTESIAN_POINT('',(77.2426896003823,819.294869955385,121.182902203964));
#75136=CARTESIAN_POINT('',(77.2426896003823,822.218334282986,112.911299343408));
#75137=CARTESIAN_POINT('Origin',(77.2426896003823,817.571257810939,120.573719352242));
#75138=CARTESIAN_POINT('Origin',(77.2426896003823,820.494722138539,112.302116491685));
#75139=CARTESIAN_POINT('',(77.2426896003823,818.831305507033,118.509011735174));
#75140=CARTESIAN_POINT('Origin',(77.2426896003823,818.359883276424,118.342395167907));
#75141=CARTESIAN_POINT('',(77.2426896003823,817.376213772479,122.626024841944));
#75142=CARTESIAN_POINT('',(77.2426896003823,820.966144369148,112.468733058952));
#75143=CARTESIAN_POINT('Origin',(77.2426896003823,816.904791541871,122.459408274677));
#75144=CARTESIAN_POINT('Origin',(82.2063885331164,821.68423828967,112.72253174778));
#75145=CARTESIAN_POINT('',(82.2063885331164,819.846507090563,123.499110085019));
#75146=CARTESIAN_POINT('Origin',(82.2063885331164,818.094307693001,122.879823530771));
#75147=CARTESIAN_POINT('',(82.2063885331164,820.512973359631,121.613421162583));
#75148=CARTESIAN_POINT('',(82.2063885331164,823.436437687231,113.341818302027));
#75149=CARTESIAN_POINT('Origin',(82.2063885331164,818.760773962069,120.994134608336));
#75150=CARTESIAN_POINT('Origin',(82.2063885331164,821.68423828967,112.72253174778));
#75151=CARTESIAN_POINT('',(82.2063885331164,820.020821658163,118.929426991268));
#75152=CARTESIAN_POINT('Origin',(82.2063885331164,819.549399427555,118.762810424001));
#75153=CARTESIAN_POINT('',(82.2063885331164,818.56572992361,123.046440098039));
#75154=CARTESIAN_POINT('',(82.2063885331164,822.155660520279,112.889148315047));
#75155=CARTESIAN_POINT('Origin',(82.2063885331164,818.094307693001,122.879823530771));
#75156=CARTESIAN_POINT('Origin',(86.354482212296,823.885477455299,113.500524149703));
#75157=CARTESIAN_POINT('',(86.354482212296,822.004789207011,124.261920012272));
#75158=CARTESIAN_POINT('Origin',(86.354482212296,820.29554685863,123.657815932694));
#75159=CARTESIAN_POINT('',(86.354482212296,822.671255476079,122.376231089837));
#75160=CARTESIAN_POINT('',(86.354482212296,825.594719803679,114.104628229281));
#75161=CARTESIAN_POINT('Origin',(86.354482212296,820.962013127699,121.772127010259));
#75162=CARTESIAN_POINT('Origin',(86.354482212296,823.885477455299,113.500524149703));
#75163=CARTESIAN_POINT('',(86.354482212296,822.222060823793,119.707419393191));
#75164=CARTESIAN_POINT('Origin',(86.354482212296,821.750638593184,119.540802825924));
#75165=CARTESIAN_POINT('',(86.354482212296,820.766969089239,123.824432499961));
#75166=CARTESIAN_POINT('',(86.354482212296,824.356899685908,113.66714071697));
#75167=CARTESIAN_POINT('Origin',(86.354482212296,820.29554685863,123.657815932694));
#75168=CARTESIAN_POINT('Origin',(91.2604284870247,826.956742332132,114.586013076021));
#75169=CARTESIAN_POINT('',(91.2604284870247,825.169026885505,125.380268672511));
#75170=CARTESIAN_POINT('Origin',(91.2604284870247,823.366811735464,124.743304859012));
#75171=CARTESIAN_POINT('',(91.2604284870247,825.835493154573,123.494579750075));
#75172=CARTESIAN_POINT('',(91.2604284870247,828.758957482173,115.222976889519));
#75173=CARTESIAN_POINT('Origin',(91.2604284870247,824.033278004532,122.857615936577));
#75174=CARTESIAN_POINT('Origin',(91.2604284870247,826.956742332132,114.586013076021));
#75175=CARTESIAN_POINT('',(91.2604284870247,825.293325700626,120.792908319509));
#75176=CARTESIAN_POINT('Origin',(91.2604284870247,824.821903470017,120.626291752242));
#75177=CARTESIAN_POINT('',(91.2604284870247,823.838233966072,124.909921426279));
#75178=CARTESIAN_POINT('',(91.2604284870247,827.428164562741,114.752629643288));
#75179=CARTESIAN_POINT('Origin',(91.2604284870247,823.366811735464,124.743304859012));
#75180=CARTESIAN_POINT('Origin',(94.8482639557915,830.610724290717,115.877453935755));
#75181=CARTESIAN_POINT('',(94.8482639557915,828.481892509846,126.551147477763));
#75182=CARTESIAN_POINT('Origin',(94.8482639557915,827.020793694048,126.034745718746));
#75183=CARTESIAN_POINT('',(94.8482639557915,829.148358778914,124.665458555328));
#75184=CARTESIAN_POINT('',(94.8482639557915,832.071823106514,116.393855694772));
#75185=CARTESIAN_POINT('Origin',(94.8482639557915,827.687259963117,124.149056796311));
#75186=CARTESIAN_POINT('Origin',(94.8482639557915,830.610724290717,115.877453935755));
#75187=CARTESIAN_POINT('',(94.8482639557915,828.94730765921,122.084349179243));
#75188=CARTESIAN_POINT('Origin',(94.8482639557915,828.475885428602,121.917732611976));
#75189=CARTESIAN_POINT('',(94.8482639557915,827.492215924657,126.201362286013));
#75190=CARTESIAN_POINT('',(94.8482639557915,831.082146521326,116.044070503022));
#75191=CARTESIAN_POINT('Origin',(94.8482639557915,827.020793694048,126.034745718746));
#75192=CARTESIAN_POINT('Origin',(98.399534595272,835.339827038736,117.548878860097));
#75193=CARTESIAN_POINT('',(98.399534595272,832.937278019029,128.125831468446));
#75194=CARTESIAN_POINT('Origin',(98.399534595272,831.749896442067,127.706170643088));
#75195=CARTESIAN_POINT('',(98.3995346119163,833.601376047008,126.246843209188));
#75196=CARTESIAN_POINT('',(98.399534595272,836.527208615697,117.968539685455));
#75197=CARTESIAN_POINT('',(97.4583707276143,833.205316112613,126.099324547641));
#75198=CARTESIAN_POINT('Ctrl Pts',(98.3995346119195,833.601376047086,126.246843208968));
#75199=CARTESIAN_POINT('Ctrl Pts',(98.2960201644212,833.601860815876,126.245471616071));
#75200=CARTESIAN_POINT('Ctrl Pts',(98.1927006143714,833.590245389903,126.240034939902));
#75201=CARTESIAN_POINT('Ctrl Pts',(97.9441465608869,833.532056193237,126.216806144848));
#75202=CARTESIAN_POINT('Ctrl Pts',(97.8043263550253,833.472267314184,126.194667576166));
#75203=CARTESIAN_POINT('Ctrl Pts',(97.5980341511791,833.336934754523,126.145977220307));
#75204=CARTESIAN_POINT('Ctrl Pts',(97.5239144809264,833.274822594726,126.12389049023));
#75205=CARTESIAN_POINT('Ctrl Pts',(97.4583707276145,833.205316112613,126.099324547641));
#75206=CARTESIAN_POINT('',(97.7253331459279,831.413465735163,125.466023995477));
#75207=CARTESIAN_POINT('Origin',(98.3995345952731,832.416362711137,125.820481720653));
#75208=CARTESIAN_POINT('Ctrl Pts',(97.7253331459279,831.413465735163,125.466023995477));
#75209=CARTESIAN_POINT('Ctrl Pts',(97.8520002019731,831.337769000587,125.439270208214));
#75210=CARTESIAN_POINT('Ctrl Pts',(97.9920400467637,831.283884893482,125.420541627155));
#75211=CARTESIAN_POINT('Ctrl Pts',(98.2877231697512,831.22436718307,125.401205679672));
#75212=CARTESIAN_POINT('Ctrl Pts',(98.4410689020655,831.21991739046,125.401023560445));
#75213=CARTESIAN_POINT('Ctrl Pts',(98.7470605981185,831.263164940511,125.420244179844));
#75214=CARTESIAN_POINT('Ctrl Pts',(98.8967967463751,831.312302058446,125.44015905039));
#75215=CARTESIAN_POINT('Ctrl Pts',(99.1772272516042,831.46430886483,125.499720197219));
#75216=CARTESIAN_POINT('Ctrl Pts',(99.3034370287928,831.568759422086,125.539893404954));
#75217=CARTESIAN_POINT('Ctrl Pts',(99.5044062771853,831.817536546003,125.633794662295));
#75218=CARTESIAN_POINT('Ctrl Pts',(99.5774214571361,831.95924831943,125.686527395921));
#75219=CARTESIAN_POINT('Ctrl Pts',(99.6602090166774,832.260619193867,125.796732544454));
#75220=CARTESIAN_POINT('Ctrl Pts',(99.6696196598402,832.417222472356,125.853090860326));
#75221=CARTESIAN_POINT('Ctrl Pts',(99.6466515176081,832.571384524781,125.907576945857));
#75222=CARTESIAN_POINT('Ctrl Pts',(99.6382510228578,832.627768602301,125.927504986655));
#75223=CARTESIAN_POINT('Ctrl Pts',(99.6255599871384,832.683551389161,125.947087799584));
#75224=CARTESIAN_POINT('Ctrl Pts',(99.5629225224937,832.886672393037,126.01790531564));
#75225=CARTESIAN_POINT('Ctrl Pts',(99.4869779146069,833.025517301181,126.065312553998));
#75226=CARTESIAN_POINT('Ctrl Pts',(99.2836472483551,833.267980760135,126.146355878784));
#75227=CARTESIAN_POINT('Ctrl Pts',(99.1583912238311,833.369446712211,126.179291843365));
#75228=CARTESIAN_POINT('Ctrl Pts',(98.8728084678537,833.522624406972,126.227296997787));
#75229=CARTESIAN_POINT('Ctrl Pts',(98.7148885128273,833.572355949435,126.241736632413));
#75230=CARTESIAN_POINT('Ctrl Pts',(98.5009823002612,833.597998782357,126.247211076537));
#75231=CARTESIAN_POINT('Ctrl Pts',(98.4502350741954,833.601138611613,126.247515003057));
#75232=CARTESIAN_POINT('Ctrl Pts',(98.3995346119195,833.601376047086,126.246843208968));
#75233=CARTESIAN_POINT('Origin',(98.399534595272,835.339827038736,117.548878860097));
#75234=CARTESIAN_POINT('',(98.399534595272,833.676410407229,123.755774103585));
#75235=CARTESIAN_POINT('Origin',(98.399534595272,833.20498817662,123.589157536318));
#75236=CARTESIAN_POINT('',(98.399534595272,832.221318672676,127.872787210355));
#75237=CARTESIAN_POINT('',(98.399534595272,835.811249269344,117.715495427364));
#75238=CARTESIAN_POINT('Origin',(98.399534595272,831.749896442067,127.706170643088));
#75239=CARTESIAN_POINT('Origin',(61.7878068235231,819.371041962602,111.90496989684));
#75240=CARTESIAN_POINT('',(61.7878068235231,816.77947378506,122.415116739188));
#75241=CARTESIAN_POINT('Origin',(61.7878068235231,815.781111365933,122.062261679831));
#75242=CARTESIAN_POINT('',(61.7878068235231,817.445940054129,120.529427816752));
#75243=CARTESIAN_POINT('',(61.7878068235231,820.369404381729,112.257824956196));
#75244=CARTESIAN_POINT('Origin',(61.7878068235231,816.447577635001,120.176572757396));
#75245=CARTESIAN_POINT('Origin',(61.7878068235231,819.371041962602,111.90496989684));
#75246=CARTESIAN_POINT('',(61.7878068235231,817.707625331095,118.111865140328));
#75247=CARTESIAN_POINT('Origin',(61.7878068235231,817.236203100487,117.945248573061));
#75248=CARTESIAN_POINT('',(61.7878068235231,816.252533596542,122.228878247098));
#75249=CARTESIAN_POINT('',(61.7878068235231,819.84246419321,112.071586464107));
#75250=CARTESIAN_POINT('Origin',(61.7878068235231,815.781111365933,122.062261679831));
#75251=CARTESIAN_POINT('Origin',(65.540926091864,817.622837600195,111.287095323192));
#75252=CARTESIAN_POINT('',(65.540926091864,815.254676282909,121.876201709114));
#75253=CARTESIAN_POINT('Origin',(65.540926091864,814.032907003526,121.444387106183));
#75254=CARTESIAN_POINT('',(65.540926091864,815.921142551977,119.990512786679));
#75255=CARTESIAN_POINT('',(65.540926091864,818.844606879577,111.718909926123));
#75256=CARTESIAN_POINT('Origin',(65.540926091864,814.699373272594,119.558698183748));
#75257=CARTESIAN_POINT('Origin',(65.540926091864,817.622837600195,111.287095323192));
#75258=CARTESIAN_POINT('',(65.540926091864,815.959420968688,117.49399056668));
#75259=CARTESIAN_POINT('Origin',(65.540926091864,815.48799873808,117.327373999413));
#75260=CARTESIAN_POINT('',(65.540926091864,814.504329234135,121.61100367345));
#75261=CARTESIAN_POINT('',(65.540926091864,818.094259830803,111.453711890459));
#75262=CARTESIAN_POINT('Origin',(65.540926091864,814.032907003526,121.444387106183));
#75263=CARTESIAN_POINT('Origin',(70.0724253967104,816.278388763384,110.811921613699));
#75264=CARTESIAN_POINT('',(70.0724253967104,814.203174568716,121.504565424869));
#75265=CARTESIAN_POINT('Origin',(70.0724253967104,812.688458166716,120.969213396691));
#75266=CARTESIAN_POINT('',(70.0724253967104,814.869640837785,119.618876502433));
#75267=CARTESIAN_POINT('',(70.0724253967104,817.793105165385,111.347273641877));
#75268=CARTESIAN_POINT('Origin',(70.0724253967104,813.354924435784,119.083524474256));
#75269=CARTESIAN_POINT('Origin',(70.0724253967104,816.278388763384,110.811921613699));
#75270=CARTESIAN_POINT('',(70.0724253967104,814.614972131878,117.018816857188));
#75271=CARTESIAN_POINT('Origin',(70.0724253967104,814.143549901269,116.852200289921));
#75272=CARTESIAN_POINT('',(70.0724253967104,813.159880397325,121.135829963958));
#75273=CARTESIAN_POINT('',(70.0724253967104,816.749810993993,110.978538180967));
#75274=CARTESIAN_POINT('Origin',(70.0724253967104,812.688458166716,120.969213396691));
#75275=CARTESIAN_POINT('Origin',(74.7661792067218,815.91112846028,110.682119396019));
#75276=CARTESIAN_POINT('',(74.7661792067218,814.044810008058,121.448594030733));
#75277=CARTESIAN_POINT('Origin',(74.7661792067218,812.321197863611,120.839411179011));
#75278=CARTESIAN_POINT('',(74.7661792067218,814.711276277126,119.562905108298));
#75279=CARTESIAN_POINT('',(74.7661792067218,817.634740604727,111.291302247742));
#75280=CARTESIAN_POINT('Origin',(74.7661792067218,812.98766413268,118.953722256575));
#75281=CARTESIAN_POINT('Origin',(74.7661792067218,815.91112846028,110.682119396019));
#75282=CARTESIAN_POINT('',(74.7661792067218,814.247711828774,116.889014639508));
#75283=CARTESIAN_POINT('Origin',(74.7661792067218,813.776289598165,116.722398072241));
#75284=CARTESIAN_POINT('',(74.7661792067218,812.79262009422,121.006027746278));
#75285=CARTESIAN_POINT('',(74.7661792067218,816.382550690889,110.848735963286));
#75286=CARTESIAN_POINT('Origin',(74.7661792067218,812.321197863611,120.839411179011));
#75287=CARTESIAN_POINT('Origin',(79.8837159971768,816.101624938623,110.749447297075));
#75288=CARTESIAN_POINT('',(79.8837159971768,814.263893739516,121.526025634314));
#75289=CARTESIAN_POINT('Origin',(79.8837159971768,812.511694341955,120.906739080067));
#75290=CARTESIAN_POINT('',(79.8837159971768,814.930360008584,119.640336711878));
#75291=CARTESIAN_POINT('',(79.8837159971768,817.853824336185,111.368733851322));
#75292=CARTESIAN_POINT('Origin',(79.8837159971768,813.178160611023,119.021050157631));
#75293=CARTESIAN_POINT('Origin',(79.8837159971768,816.101624938623,110.749447297075));
#75294=CARTESIAN_POINT('',(79.8837159971768,814.438208307117,116.956342540564));
#75295=CARTESIAN_POINT('Origin',(79.8837159971768,813.966786076508,116.789725973297));
#75296=CARTESIAN_POINT('',(79.8837159971768,812.983116572563,121.073355647334));
#75297=CARTESIAN_POINT('',(79.8837159971768,816.573047169232,110.916063864342));
#75298=CARTESIAN_POINT('Origin',(79.8837159971768,812.511694341955,120.906739080067));
#75299=CARTESIAN_POINT('Origin',(84.4265709358799,817.441617637763,111.223046056738));
#75300=CARTESIAN_POINT('',(84.4265709358799,815.560929389475,121.984441919307));
#75301=CARTESIAN_POINT('Origin',(84.4265709358799,813.851687041094,121.380337839729));
#75302=CARTESIAN_POINT('',(84.4265709358799,816.227395658543,120.098752996872));
#75303=CARTESIAN_POINT('',(84.4265709358799,819.150859986143,111.827150136316));
#75304=CARTESIAN_POINT('Origin',(84.4265709358799,814.518153310162,119.494648917294));
#75305=CARTESIAN_POINT('Origin',(84.4265709358799,817.441617637763,111.223046056738));
#75306=CARTESIAN_POINT('',(84.4265709358799,815.778201006257,117.429941300226));
#75307=CARTESIAN_POINT('Origin',(84.4265709358799,815.306778775648,117.263324732959));
#75308=CARTESIAN_POINT('',(84.4265709358799,814.323109271703,121.546954406996));
#75309=CARTESIAN_POINT('',(84.4265709358799,817.913039868372,111.389662624005));
#75310=CARTESIAN_POINT('Origin',(84.4265709358799,813.851687041094,121.380337839729));
#75311=CARTESIAN_POINT('Origin',(89.9025716101847,819.484063277678,111.94491545376));
#75312=CARTESIAN_POINT('',(89.9025716101847,817.69634783105,122.739171050249));
#75313=CARTESIAN_POINT('Origin',(89.9025716101847,815.89413268101,122.102207236751));
#75314=CARTESIAN_POINT('',(89.9025716101847,818.362814100118,120.853482127814));
#75315=CARTESIAN_POINT('',(89.9025716101847,821.286278427719,112.581879267258));
#75316=CARTESIAN_POINT('Origin',(89.9025716101847,816.560598950078,120.216518314316));
#75317=CARTESIAN_POINT('Origin',(89.9025716101847,819.484063277678,111.94491545376));
#75318=CARTESIAN_POINT('',(89.9025716101847,817.820646646172,118.151810697248));
#75319=CARTESIAN_POINT('Origin',(89.9025716101847,817.349224415563,117.985194129981));
#75320=CARTESIAN_POINT('',(89.9025716101847,816.365554911618,122.268823804018));
#75321=CARTESIAN_POINT('',(89.9025716101847,819.955485508287,112.111532021027));
#75322=CARTESIAN_POINT('Origin',(89.9025716101847,815.89413268101,122.102207236751));
#75323=CARTESIAN_POINT('Origin',(94.2177634323048,822.354879367022,112.959558996225));
#75324=CARTESIAN_POINT('',(94.2177634323048,820.226047586151,123.633252538233));
#75325=CARTESIAN_POINT('Origin',(94.2177634323048,818.764948770354,123.116850779216));
#75326=CARTESIAN_POINT('',(94.2177634323048,820.892513855219,121.747563615798));
#75327=CARTESIAN_POINT('',(94.2177634323048,823.81597818282,113.475960755242));
#75328=CARTESIAN_POINT('Origin',(94.2177634323048,819.431415039422,121.231161856781));
#75329=CARTESIAN_POINT('Origin',(94.2177634323048,822.354879367022,112.959558996225));
#75330=CARTESIAN_POINT('',(94.2177634323048,820.691462735516,119.166454239713));
#75331=CARTESIAN_POINT('Origin',(94.2177634323048,820.220040504907,118.999837672446));
#75332=CARTESIAN_POINT('',(94.2177634323048,819.236371000962,123.283467346483));
#75333=CARTESIAN_POINT('',(94.2177634323048,822.826301597631,113.126175563492));
#75334=CARTESIAN_POINT('Origin',(94.2177634323048,818.764948770354,123.116850779216));
#75335=CARTESIAN_POINT('Origin',(98.7342701080466,826.284490021524,114.348416363226));
#75336=CARTESIAN_POINT('',(98.7342701080466,823.881941001817,124.925368971576));
#75337=CARTESIAN_POINT('Origin',(98.7342701080466,822.694559424855,124.505708146217));
#75338=CARTESIAN_POINT('',(98.7342701101916,824.547122491794,123.043315182399));
#75339=CARTESIAN_POINT('',(98.7342701080466,827.471871598486,114.768077188584));
#75340=CARTESIAN_POINT('',(97.9876492765575,824.317233404711,122.957975382871));
#75341=CARTESIAN_POINT('Ctrl Pts',(98.7342701123366,824.547122491794,123.043315182399));
#75342=CARTESIAN_POINT('Ctrl Pts',(98.7186233546984,824.547177168776,123.043160480388));
#75343=CARTESIAN_POINT('Ctrl Pts',(98.702965884564,824.546955160808,123.042913564466));
#75344=CARTESIAN_POINT('Ctrl Pts',(98.5349995581169,824.54159384245,123.039272550181));
#75345=CARTESIAN_POINT('Ctrl Pts',(98.384980613872,824.510527138023,123.027285369851));
#75346=CARTESIAN_POINT('Ctrl Pts',(98.1532939493101,824.418596946666,122.993934879506));
#75347=CARTESIAN_POINT('Ctrl Pts',(98.0670879888991,824.372372567245,122.977463428591));
#75348=CARTESIAN_POINT('Ctrl Pts',(97.9876492765573,824.317233404711,122.957975382871));
#75349=CARTESIAN_POINT('',(97.8536473849113,822.512207045121,122.320017992798));
#75350=CARTESIAN_POINT('Origin',(98.7342701080476,823.361025693924,122.620019223782));
#75351=CARTESIAN_POINT('Ctrl Pts',(97.8536473849113,822.512207045121,122.320017992798));
#75352=CARTESIAN_POINT('Ctrl Pts',(97.9608541687947,822.413334127242,122.285072958171));
#75353=CARTESIAN_POINT('Ctrl Pts',(98.0859734189423,822.333173563606,122.257057388288));
#75354=CARTESIAN_POINT('Ctrl Pts',(98.3621883418565,822.216982503381,122.21769116139));
#75355=CARTESIAN_POINT('Ctrl Pts',(98.5112981985599,822.182560285577,122.206915772957));
#75356=CARTESIAN_POINT('Ctrl Pts',(98.8204126527526,822.16485269463,122.204592783059));
#75357=CARTESIAN_POINT('Ctrl Pts',(98.9778887400996,822.183546018221,122.213747786592));
#75358=CARTESIAN_POINT('Ctrl Pts',(99.2861153936676,822.277218697885,122.252691679254));
#75359=CARTESIAN_POINT('Ctrl Pts',(99.4328257815214,822.354623700265,122.283306072786));
#75360=CARTESIAN_POINT('Ctrl Pts',(99.6846765146236,822.558527746896,122.361347666295));
#75361=CARTESIAN_POINT('Ctrl Pts',(99.787529153329,822.682811556581,122.407920767846));
#75362=CARTESIAN_POINT('Ctrl Pts',(99.9352202026085,822.96134270475,122.510053584314));
#75363=CARTESIAN_POINT('Ctrl Pts',(99.9790285654115,823.112672142274,122.564547946344));
#75364=CARTESIAN_POINT('Ctrl Pts',(99.9905574335051,823.267967791832,122.619434683458));
#75365=CARTESIAN_POINT('Ctrl Pts',(99.9947740651734,823.324766477407,122.639509260771));
#75366=CARTESIAN_POINT('Ctrl Pts',(99.9946521260043,823.381818990948,122.659540838072));
#75367=CARTESIAN_POINT('Ctrl Pts',(99.9781073773492,823.592786710345,122.733131648893));
#75368=CARTESIAN_POINT('Ctrl Pts',(99.9343244033688,823.743496256212,122.784732251672));
#75369=CARTESIAN_POINT('Ctrl Pts',(99.7885816504621,824.02055182496,122.878001598513));
#75370=CARTESIAN_POINT('Ctrl Pts',(99.6882348819836,824.144374324847,122.918839123543));
#75371=CARTESIAN_POINT('Ctrl Pts',(99.4422459149123,824.35022915398,122.985462159628));
#75372=CARTESIAN_POINT('Ctrl Pts',(99.2985261059392,824.429852275868,123.01046648983));
#75373=CARTESIAN_POINT('Ctrl Pts',(99.0112452426019,824.524339635425,123.038803592336));
#75374=CARTESIAN_POINT('Ctrl Pts',(98.873179893281,824.546637077005,123.044688605763));
#75375=CARTESIAN_POINT('Ctrl Pts',(98.7342701123366,824.547122491794,123.043315182399));
#75376=CARTESIAN_POINT('Origin',(98.7342701080466,826.284490021524,114.348416363226));
#75377=CARTESIAN_POINT('',(98.7342701080466,824.621073390018,120.555311606714));
#75378=CARTESIAN_POINT('Origin',(98.7342701080466,824.149651159408,120.388695039447));
#75379=CARTESIAN_POINT('',(98.7342701080466,823.165981655464,124.672324713484));
#75380=CARTESIAN_POINT('',(98.7342701080466,826.755912252132,114.515032930493));
#75381=CARTESIAN_POINT('Origin',(98.7342701080466,822.694559424855,124.505708146217));
#75382=CARTESIAN_POINT('Origin',(59.4012339544,817.84159912046,111.364413046435));
#75383=CARTESIAN_POINT('',(59.4012339544,815.250030942918,121.874559888782));
#75384=CARTESIAN_POINT('Origin',(59.4012339544,814.251668523791,121.521704829426));
#75385=CARTESIAN_POINT('',(59.4012339544,815.916497211987,119.988870966347));
#75386=CARTESIAN_POINT('',(59.4012339544,818.839961539587,111.717268105791));
#75387=CARTESIAN_POINT('Origin',(59.4012339544,814.91813479286,119.636015906991));
#75388=CARTESIAN_POINT('Origin',(59.4012339544,817.84159912046,111.364413046435));
#75389=CARTESIAN_POINT('',(59.4012339544,816.178182488954,117.571308289923));
#75390=CARTESIAN_POINT('Origin',(59.4012339544,815.706760258345,117.404691722656));
#75391=CARTESIAN_POINT('',(59.4012339544,814.7230907544,121.688321396693));
#75392=CARTESIAN_POINT('',(59.4012339544,818.313021351069,111.531029613702));
#75393=CARTESIAN_POINT('Origin',(59.4012339544,814.251668523791,121.521704829426));
#75394=CARTESIAN_POINT('Origin',(62.6868326383422,815.395879304728,110.500012910556));
#75395=CARTESIAN_POINT('',(62.6868326383422,813.027717987442,121.089119296479));
#75396=CARTESIAN_POINT('Origin',(62.6868326383422,811.80594870806,120.657304693548));
#75397=CARTESIAN_POINT('',(62.6868326383422,813.694184256511,119.203430374043));
#75398=CARTESIAN_POINT('',(62.6868326383422,816.617648584111,110.931827513487));
#75399=CARTESIAN_POINT('Origin',(62.6868326383422,812.472414977128,118.771615771112));
#75400=CARTESIAN_POINT('Origin',(62.6868326383422,815.395879304728,110.500012910556));
#75401=CARTESIAN_POINT('',(62.6868326383422,813.732462673222,116.706908154045));
#75402=CARTESIAN_POINT('Origin',(62.6868326383422,813.261040442613,116.540291586778));
#75403=CARTESIAN_POINT('',(62.6868326383422,812.277370938668,120.823921260815));
#75404=CARTESIAN_POINT('',(62.6868326383422,815.867301535337,110.666629477823));
#75405=CARTESIAN_POINT('Origin',(62.6868326383422,811.80594870806,120.657304693548));
#75406=CARTESIAN_POINT('Origin',(66.8228361846836,813.192507405306,109.721266728348));
#75407=CARTESIAN_POINT('',(66.8228361846836,811.117293210638,120.413910539517));
#75408=CARTESIAN_POINT('Origin',(66.8228361846836,809.602576808637,119.87855851134));
#75409=CARTESIAN_POINT('',(66.8228361846836,811.783759479706,118.528221617082));
#75410=CARTESIAN_POINT('',(66.8228361846836,814.707223807306,110.256618756526));
#75411=CARTESIAN_POINT('Origin',(66.8228361846836,810.269043077705,117.992869588904));
#75412=CARTESIAN_POINT('Origin',(66.8228361846836,813.192507405306,109.721266728348));
#75413=CARTESIAN_POINT('',(66.8228361846836,811.529090773799,115.928161971837));
#75414=CARTESIAN_POINT('Origin',(66.8228361846836,811.057668543191,115.76154540457));
#75415=CARTESIAN_POINT('',(66.8228361846836,810.073999039246,120.045175078607));
#75416=CARTESIAN_POINT('',(66.8228361846836,813.663929635914,109.887883295615));
#75417=CARTESIAN_POINT('Origin',(66.8228361846836,809.602576808637,119.87855851134));
#75418=CARTESIAN_POINT('Origin',(71.3330336724699,811.913163636806,109.269103352882));
#75419=CARTESIAN_POINT('',(71.3330336724699,810.046845184584,120.035577987596));
#75420=CARTESIAN_POINT('Origin',(71.3330336724699,808.323233040137,119.426395135873));
#75421=CARTESIAN_POINT('',(71.3330336724699,810.713311453652,118.14988906516));
#75422=CARTESIAN_POINT('',(71.3330336724699,813.636775781252,109.878286204604));
#75423=CARTESIAN_POINT('Origin',(71.3330336724699,808.989699309205,117.540706213438));
#75424=CARTESIAN_POINT('Origin',(71.3330336724699,811.913163636806,109.269103352882));
#75425=CARTESIAN_POINT('',(71.3330336724699,810.249747005299,115.47599859637));
#75426=CARTESIAN_POINT('Origin',(71.3330336724699,809.778324774691,115.309382029103));
#75427=CARTESIAN_POINT('',(71.3330336724699,808.794655270746,119.59301170314));
#75428=CARTESIAN_POINT('',(71.3330336724699,812.384585867414,109.435719920149));
#75429=CARTESIAN_POINT('Origin',(71.3330336724699,808.323233040137,119.426395135873));
#75430=CARTESIAN_POINT('Origin',(76.3807474062371,811.096314832155,108.980401346548));
#75431=CARTESIAN_POINT('',(76.3807474062371,809.258583633048,119.756979683786));
#75432=CARTESIAN_POINT('Origin',(76.3807474062371,807.506384235486,119.137693129539));
#75433=CARTESIAN_POINT('',(76.3807474062371,809.925049902116,117.871290761351));
#75434=CARTESIAN_POINT('',(76.3807474062371,812.848514229716,109.599687900795));
#75435=CARTESIAN_POINT('Origin',(76.3807474062371,808.172850504554,117.252004207104));
#75436=CARTESIAN_POINT('Origin',(76.3807474062371,811.096314832155,108.980401346548));
#75437=CARTESIAN_POINT('',(76.3807474062371,809.432898200648,115.187296590036));
#75438=CARTESIAN_POINT('Origin',(76.3807474062371,808.96147597004,115.020680022769));
#75439=CARTESIAN_POINT('',(76.3807474062371,807.977806466095,119.304309696806));
#75440=CARTESIAN_POINT('',(76.3807474062371,811.567737062763,109.147017913815));
#75441=CARTESIAN_POINT('Origin',(76.3807474062371,807.506384235486,119.137693129539));
#75442=CARTESIAN_POINT('Origin',(81.1198190446058,811.516496953853,109.128907925574));
#75443=CARTESIAN_POINT('',(81.1198190446058,809.635808705565,119.890303788143));
#75444=CARTESIAN_POINT('Origin',(81.1198190446058,807.926566357185,119.286199708565));
#75445=CARTESIAN_POINT('',(81.1198190446058,810.302274974634,118.004614865708));
#75446=CARTESIAN_POINT('',(81.1198190446058,813.225739302234,109.733012005152));
#75447=CARTESIAN_POINT('Origin',(81.1198190446058,808.593032626253,117.40051078613));
#75448=CARTESIAN_POINT('Origin',(81.1198190446058,811.516496953853,109.128907925574));
#75449=CARTESIAN_POINT('',(81.1198190446058,809.853080322347,115.335803169062));
#75450=CARTESIAN_POINT('Origin',(81.1198190446058,809.381658091738,115.169186601795));
#75451=CARTESIAN_POINT('',(81.1198190446058,808.397988587793,119.452816275832));
#75452=CARTESIAN_POINT('',(81.1198190446058,811.987919184462,109.295524492841));
#75453=CARTESIAN_POINT('Origin',(81.1198190446058,807.926566357185,119.286199708565));
#75454=CARTESIAN_POINT('Origin',(86.9265466122529,812.440858681645,109.455608636736));
#75455=CARTESIAN_POINT('',(86.9265466122529,810.653143235017,120.249864233226));
#75456=CARTESIAN_POINT('Origin',(86.9265466122529,808.850928084977,119.612900419728));
#75457=CARTESIAN_POINT('',(86.9265466122529,811.319609504086,118.364175310791));
#75458=CARTESIAN_POINT('',(86.9265466122529,814.243073831686,110.092572450235));
#75459=CARTESIAN_POINT('Origin',(86.9265466122529,809.517394354045,117.727211497293));
#75460=CARTESIAN_POINT('Origin',(86.9265466122529,812.440858681645,109.455608636736));
#75461=CARTESIAN_POINT('',(86.9265466122529,810.777442050139,115.662503880225));
#75462=CARTESIAN_POINT('Origin',(86.9265466122529,810.30601981953,115.495887312958));
#75463=CARTESIAN_POINT('',(86.9265466122529,809.322350315585,119.779516986995));
#75464=CARTESIAN_POINT('',(86.9265466122529,812.912280912254,109.622225204003));
#75465=CARTESIAN_POINT('Origin',(86.9265466122529,808.850928084977,119.612900419728));
#75466=CARTESIAN_POINT('Origin',(91.7805001985119,814.40304046294,110.149110070326));
#75467=CARTESIAN_POINT('',(91.7805001985119,812.274208682069,120.822803612335));
#75468=CARTESIAN_POINT('Origin',(91.7805001985119,810.813109866272,120.306401853318));
#75469=CARTESIAN_POINT('',(91.7805001985119,812.940674951138,118.9371146899));
#75470=CARTESIAN_POINT('',(91.7805001985119,815.864139278738,110.665511829344));
#75471=CARTESIAN_POINT('Origin',(91.7805001985119,811.47957613534,118.420712930883));
#75472=CARTESIAN_POINT('Origin',(91.7805001985119,814.40304046294,110.149110070326));
#75473=CARTESIAN_POINT('',(91.7805001985119,812.739623831434,116.356005313815));
#75474=CARTESIAN_POINT('Origin',(91.7805001985119,812.268201600825,116.189388746548));
#75475=CARTESIAN_POINT('',(91.7805001985119,811.28453209688,120.473018420585));
#75476=CARTESIAN_POINT('',(91.7805001985119,814.874462693549,110.315726637593));
#75477=CARTESIAN_POINT('Origin',(91.7805001985119,810.813109866272,120.306401853318));
#75478=CARTESIAN_POINT('Origin',(97.0648498961815,817.361416181959,111.194700148572));
#75479=CARTESIAN_POINT('',(97.0648498961815,814.958867162252,121.771652756922));
#75480=CARTESIAN_POINT('Origin',(97.0648498961815,813.77148558529,121.351991931564));
#75481=CARTESIAN_POINT('',(97.0648499049205,815.624798041961,119.887478656512));
#75482=CARTESIAN_POINT('',(97.0648498961815,818.548797758921,111.614360973931));
#75483=CARTESIAN_POINT('',(96.5454030138814,815.519623009101,119.848602194473));
#75484=CARTESIAN_POINT('Ctrl Pts',(97.0648499136594,815.624798041962,119.887478656512));
#75485=CARTESIAN_POINT('Ctrl Pts',(96.9852132592777,815.624972130868,119.886986095481));
#75486=CARTESIAN_POINT('Ctrl Pts',(96.905592296291,815.617976989133,119.884109694102));
#75487=CARTESIAN_POINT('Ctrl Pts',(96.7297894687742,815.586299535278,119.872302126068));
#75488=CARTESIAN_POINT('Ctrl Pts',(96.6352648323356,815.557985006066,119.862160622211));
#75489=CARTESIAN_POINT('Ctrl Pts',(96.5454030138814,815.519623009101,119.848602194473));
#75490=CARTESIAN_POINT('',(96.0162933379529,813.780308980762,119.233869765697));
#75491=CARTESIAN_POINT('Origin',(97.064849896183,814.437951854359,119.466303009129));
#75492=CARTESIAN_POINT('Ctrl Pts',(96.0162933379527,813.780308980762,119.233869765697));
#75493=CARTESIAN_POINT('Ctrl Pts',(96.0993543987815,813.662581100539,119.192260749403));
#75494=CARTESIAN_POINT('Ctrl Pts',(96.2040847426651,813.559643144079,119.156194878203));
#75495=CARTESIAN_POINT('Ctrl Pts',(96.4487595479483,813.391833502549,119.098584898114));
#75496=CARTESIAN_POINT('Ctrl Pts',(96.5871167127954,813.328924180813,119.077741203267));
#75497=CARTESIAN_POINT('Ctrl Pts',(96.8858441401799,813.250981315707,119.054129029369));
#75498=CARTESIAN_POINT('Ctrl Pts',(97.0441777059448,813.238378867134,119.0522230481));
#75499=CARTESIAN_POINT('Ctrl Pts',(97.3667295240589,813.269543326607,119.069074420728));
#75500=CARTESIAN_POINT('Ctrl Pts',(97.5275285746334,813.316475082749,119.088918537952));
#75501=CARTESIAN_POINT('Ctrl Pts',(97.8192537068948,813.466512421164,119.147921814152));
#75502=CARTESIAN_POINT('Ctrl Pts',(97.9474486505021,813.567900121045,119.186402655788));
#75503=CARTESIAN_POINT('Ctrl Pts',(98.153588381967,813.811367719415,119.276142827353));
#75504=CARTESIAN_POINT('Ctrl Pts',(98.2298798287403,813.950795632586,119.326430787979));
#75505=CARTESIAN_POINT('Ctrl Pts',(98.275401840303,814.1004377142,119.379319362887));
#75506=CARTESIAN_POINT('Ctrl Pts',(98.2920513113524,814.155168632718,119.398663121359));
#75507=CARTESIAN_POINT('Ctrl Pts',(98.304503798061,814.210999226654,119.418262830926));
#75508=CARTESIAN_POINT('Ctrl Pts',(98.3347748503032,814.420606711285,119.491372888756));
#75509=CARTESIAN_POINT('Ctrl Pts',(98.3250670362872,814.576617030885,119.544846964329));
#75510=CARTESIAN_POINT('Ctrl Pts',(98.24328185438,814.876219923119,119.646085298197));
#75511=CARTESIAN_POINT('Ctrl Pts',(98.1722299772469,815.017027505348,119.692925926032));
#75512=CARTESIAN_POINT('Ctrl Pts',(97.9765856973307,815.266646840541,119.775016819367));
#75513=CARTESIAN_POINT('Ctrl Pts',(97.8533472797075,815.372724707415,119.809371151566));
#75514=CARTESIAN_POINT('Ctrl Pts',(97.5793882296128,815.529173164405,119.859346437809));
#75515=CARTESIAN_POINT('Ctrl Pts',(97.4330741404546,815.581153925265,119.875541354133));
#75516=CARTESIAN_POINT('Ctrl Pts',(97.2091835566883,815.618596310145,119.886413968077));
#75517=CARTESIAN_POINT('Ctrl Pts',(97.1370102931382,815.62464029649,119.887924976));
#75518=CARTESIAN_POINT('Ctrl Pts',(97.0648499136594,815.624798041962,119.887478656512));
#75519=CARTESIAN_POINT('Origin',(97.0648498961815,817.361416181959,111.194700148572));
#75520=CARTESIAN_POINT('',(97.0648498961815,815.697999550452,117.401595392061));
#75521=CARTESIAN_POINT('Origin',(97.0648498961815,815.226577319843,117.234978824794));
#75522=CARTESIAN_POINT('',(97.0648498961815,814.242907815899,121.518608498831));
#75523=CARTESIAN_POINT('',(97.0648498961815,817.832838412567,111.361316715839));
#75524=CARTESIAN_POINT('Origin',(97.0648498961815,813.77148558529,121.351991931564));
#75525=CARTESIAN_POINT('Origin',(56.7295477813998,816.813414301827,111.001017742027));
#75526=CARTESIAN_POINT('',(56.7295477813998,814.221846124286,121.511164584375));
#75527=CARTESIAN_POINT('Origin',(56.7295477813998,813.223483705158,121.158309525018));
#75528=CARTESIAN_POINT('',(56.7295477813998,814.888312393354,119.625475661939));
#75529=CARTESIAN_POINT('',(56.7295477813998,817.811776720954,111.353872801383));
#75530=CARTESIAN_POINT('Origin',(56.7295477813998,813.889949974227,119.272620602583));
#75531=CARTESIAN_POINT('Origin',(56.7295477813998,816.813414301827,111.001017742027));
#75532=CARTESIAN_POINT('',(56.7295477813998,815.149997670321,117.207912985515));
#75533=CARTESIAN_POINT('Origin',(56.7295477813998,814.678575439712,117.041296418248));
#75534=CARTESIAN_POINT('',(56.7295477813998,813.694905935767,121.324926092285));
#75535=CARTESIAN_POINT('',(56.7295477813998,817.284836532436,111.167634309294));
#75536=CARTESIAN_POINT('Origin',(56.7295477813998,813.223483705158,121.158309525018));
#75537=CARTESIAN_POINT('Origin',(59.4040294524033,813.777068724584,109.927870477708));
#75538=CARTESIAN_POINT('',(59.4040294524033,811.408907407298,120.51697686363));
#75539=CARTESIAN_POINT('Origin',(59.4040294524033,810.187138127915,120.085162260699));
#75540=CARTESIAN_POINT('',(59.4040294524033,812.075373676366,118.631287941195));
#75541=CARTESIAN_POINT('',(59.4040294524033,814.998838003967,110.359685080639));
#75542=CARTESIAN_POINT('Origin',(59.4040294524033,810.853604396984,118.199473338264));
#75543=CARTESIAN_POINT('Origin',(59.4040294524033,813.777068724584,109.927870477708));
#75544=CARTESIAN_POINT('',(59.4040294524033,812.113652093078,116.134765721196));
#75545=CARTESIAN_POINT('Origin',(59.4040294524033,811.642229862469,115.968149153929));
#75546=CARTESIAN_POINT('',(59.4040294524033,810.658560358524,120.251778827966));
#75547=CARTESIAN_POINT('',(59.4040294524033,814.248490955193,110.094487044975));
#75548=CARTESIAN_POINT('Origin',(59.4040294524033,810.187138127915,120.085162260699));
#75549=CARTESIAN_POINT('Origin',(62.9637740385176,810.811071687506,108.879586767786));
#75550=CARTESIAN_POINT('',(62.9637740385176,808.735857492838,119.572230578955));
#75551=CARTESIAN_POINT('Origin',(62.9637740385176,807.221141090837,119.036878550777));
#75552=CARTESIAN_POINT('',(62.9637740385176,809.402323761906,117.68654165652));
#75553=CARTESIAN_POINT('',(62.9637740385176,812.325788089506,109.414938795964));
#75554=CARTESIAN_POINT('Origin',(62.9637740385176,807.887607359905,117.151189628342));
#75555=CARTESIAN_POINT('Origin',(62.9637740385176,810.811071687506,108.879586767786));
#75556=CARTESIAN_POINT('',(62.9637740385176,809.147655055999,115.086482011274));
#75557=CARTESIAN_POINT('Origin',(62.9637740385176,808.67623282539,114.919865444007));
#75558=CARTESIAN_POINT('',(62.9637740385176,807.692563321446,119.203495118044));
#75559=CARTESIAN_POINT('',(62.9637740385176,811.282493918114,109.046203335053));
#75560=CARTESIAN_POINT('Origin',(62.9637740385176,807.221141090837,119.036878550777));
#75561=CARTESIAN_POINT('Origin',(67.0932979315339,808.675557915266,108.124823943761));
#75562=CARTESIAN_POINT('',(67.0932979315339,806.809239463044,118.891298578475));
#75563=CARTESIAN_POINT('Origin',(67.0932979315339,805.085627318597,118.282115726753));
#75564=CARTESIAN_POINT('',(67.0932979315339,807.475705732112,117.00560965604));
#75565=CARTESIAN_POINT('',(67.0932979315339,810.399170059713,108.734006795484));
#75566=CARTESIAN_POINT('Origin',(67.0932979315339,805.752093587666,116.396426804318));
#75567=CARTESIAN_POINT('Origin',(67.0932979315339,808.675557915266,108.124823943761));
#75568=CARTESIAN_POINT('',(67.0932979315339,807.01214128376,114.33171918725));
#75569=CARTESIAN_POINT('Origin',(67.0932979315339,806.540719053151,114.165102619983));
#75570=CARTESIAN_POINT('',(67.0932979315339,805.557049549206,118.44873229402));
#75571=CARTESIAN_POINT('',(67.0932979315339,809.146980145875,108.291440511028));
#75572=CARTESIAN_POINT('Origin',(67.0932979315339,805.085627318597,118.282115726753));
#75573=CARTESIAN_POINT('Origin',(71.8505792968298,806.887064040059,107.49270969306));
#75574=CARTESIAN_POINT('',(71.8505792968298,805.049332840952,118.269288030299));
#75575=CARTESIAN_POINT('Origin',(71.8505792968298,803.29713344339,117.650001476052));
#75576=CARTESIAN_POINT('',(71.8505792968298,805.71579911002,116.383599107863));
#75577=CARTESIAN_POINT('',(71.8505792968298,808.63926343762,108.111996247307));
#75578=CARTESIAN_POINT('Origin',(71.8505792968298,803.963599712459,115.764312553616));
#75579=CARTESIAN_POINT('Origin',(71.8505792968298,806.887064040059,107.49270969306));
#75580=CARTESIAN_POINT('',(71.8505792968298,805.223647408553,113.699604936548));
#75581=CARTESIAN_POINT('Origin',(71.8505792968298,804.752225177944,113.532988369281));
#75582=CARTESIAN_POINT('',(71.8505792968298,803.768555673999,117.816618043319));
#75583=CARTESIAN_POINT('',(71.8505792968298,807.358486270668,107.659326260327));
#75584=CARTESIAN_POINT('Origin',(71.8505792968298,803.29713344339,117.650001476052));
#75585=CARTESIAN_POINT('Origin',(76.5787474636786,806.369071609341,107.309633641332));
#75586=CARTESIAN_POINT('',(76.5787474636786,804.488383361053,118.071029503902));
#75587=CARTESIAN_POINT('Origin',(76.5787474636786,802.779141012673,117.466925424324));
#75588=CARTESIAN_POINT('',(76.5787474636786,805.154849630121,116.185340581467));
#75589=CARTESIAN_POINT('',(76.5787474636786,808.078313957722,107.913737720911));
#75590=CARTESIAN_POINT('Origin',(76.5787474636786,803.445607281741,115.581236501889));
#75591=CARTESIAN_POINT('Origin',(76.5787474636786,806.369071609341,107.309633641332));
#75592=CARTESIAN_POINT('',(76.5787474636786,804.705654977835,113.516528884821));
#75593=CARTESIAN_POINT('Origin',(76.5787474636786,804.234232747226,113.349912317554));
#75594=CARTESIAN_POINT('',(76.5787474636786,803.250563243281,117.633541991591));
#75595=CARTESIAN_POINT('',(76.5787474636786,806.84049383995,107.4762502086));
#75596=CARTESIAN_POINT('Origin',(76.5787474636786,802.779141012673,117.466925424324));
#75597=CARTESIAN_POINT('Origin',(82.4624200661915,806.134950381925,107.226887277874));
#75598=CARTESIAN_POINT('',(82.4624200661915,804.347234935297,118.021142874364));
#75599=CARTESIAN_POINT('Origin',(82.4624200661915,802.545019785257,117.384179060865));
#75600=CARTESIAN_POINT('',(82.4624200661915,805.013701204366,116.135453951928));
#75601=CARTESIAN_POINT('',(82.4624200661915,807.937165531966,107.863851091372));
#75602=CARTESIAN_POINT('Origin',(82.4624200661915,803.211486054325,115.49849013843));
#75603=CARTESIAN_POINT('Origin',(82.4624200661915,806.134950381925,107.226887277874));
#75604=CARTESIAN_POINT('',(82.4624200661915,804.471533750419,113.433782521362));
#75605=CARTESIAN_POINT('Origin',(82.4624200661915,804.00011151981,113.267165954095));
#75606=CARTESIAN_POINT('',(82.4624200661915,803.016442015866,117.550795628132));
#75607=CARTESIAN_POINT('',(82.4624200661915,806.606372612534,107.393503845141));
#75608=CARTESIAN_POINT('Origin',(82.4624200661915,802.545019785257,117.384179060865));
#75609=CARTESIAN_POINT('Origin',(87.6429943530164,807.102741095736,107.568937262152));
#75610=CARTESIAN_POINT('',(87.6429943530164,804.973909314865,118.242630804161));
#75611=CARTESIAN_POINT('Origin',(87.6429943530164,803.512810499067,117.726229045143));
#75612=CARTESIAN_POINT('',(87.6429943530164,805.640375583933,116.356941881725));
#75613=CARTESIAN_POINT('',(87.6429943530164,808.563839911534,108.085339021169));
#75614=CARTESIAN_POINT('Origin',(87.6429943530164,804.179276768136,115.840540122708));
#75615=CARTESIAN_POINT('Origin',(87.6429943530164,807.102741095736,107.568937262152));
#75616=CARTESIAN_POINT('',(87.6429943530164,805.43932446423,113.77583250564));
#75617=CARTESIAN_POINT('Origin',(87.6429943530164,804.967902233621,113.609215938373));
#75618=CARTESIAN_POINT('',(87.6429943530164,803.984232729676,117.89284561241));
#75619=CARTESIAN_POINT('',(87.6429943530164,807.574163326345,107.735553829419));
#75620=CARTESIAN_POINT('Origin',(87.6429943530164,803.512810499067,117.726229045143));
#75621=CARTESIAN_POINT('Origin',(93.4642356337025,808.960586664488,108.225562747925));
#75622=CARTESIAN_POINT('',(93.4642356337025,806.558037644782,118.802515356275));
#75623=CARTESIAN_POINT('Origin',(93.4642356337025,805.37065606782,118.382854530917));
#75624=CARTESIAN_POINT('',(93.4642356337339,807.224380473639,116.917175693584));
#75625=CARTESIAN_POINT('',(93.4642356337025,810.14796824145,108.645223573284));
#75626=CARTESIAN_POINT('',(93.1946650219305,807.19698271569,116.907099511207));
#75627=CARTESIAN_POINT('Ctrl Pts',(93.4642356337653,807.224380473639,116.917175693584));
#75628=CARTESIAN_POINT('Ctrl Pts',(93.3734396015083,807.224468486999,116.916926670016));
#75629=CARTESIAN_POINT('Ctrl Pts',(93.2830615082368,807.215246128468,116.913554419244));
#75630=CARTESIAN_POINT('Ctrl Pts',(93.1946650260966,807.196982716551,116.907099511511));
#75631=CARTESIAN_POINT('',(92.2935721935075,805.599397387795,116.342458800678));
#75632=CARTESIAN_POINT('Origin',(93.464235633704,806.037122336889,116.497165608482));
#75633=CARTESIAN_POINT('Ctrl Pts',(92.2935721935074,805.599397387795,116.342458800678));
#75634=CARTESIAN_POINT('Ctrl Pts',(92.348857364355,805.46795981851,116.296004316392));
#75635=CARTESIAN_POINT('Ctrl Pts',(92.4286215833972,805.346739014297,116.25347666818));
#75636=CARTESIAN_POINT('Ctrl Pts',(92.6310628079813,805.134621539668,116.180206800681));
#75637=CARTESIAN_POINT('Ctrl Pts',(92.752620408957,805.045955458401,116.150259795513));
#75638=CARTESIAN_POINT('Ctrl Pts',(93.0279049875055,804.9111297565,116.106543302413));
#75639=CARTESIAN_POINT('Ctrl Pts',(93.1801760950964,804.867747333362,116.093758636667));
#75640=CARTESIAN_POINT('Ctrl Pts',(93.5029560155274,804.834961388344,116.088007772531));
#75641=CARTESIAN_POINT('Ctrl Pts',(93.6708160387134,804.849324033979,116.096340864099));
#75642=CARTESIAN_POINT('Ctrl Pts',(93.9896657820001,804.93885526688,116.133959235335));
#75643=CARTESIAN_POINT('Ctrl Pts',(94.1376002963257,805.01287938076,116.162768859809));
#75644=CARTESIAN_POINT('Ctrl Pts',(94.3931794145417,805.210592051185,116.236337691681));
#75645=CARTESIAN_POINT('Ctrl Pts',(94.4986196429727,805.33201091034,116.280260643265));
#75646=CARTESIAN_POINT('Ctrl Pts',(94.5761452676589,805.46945934698,116.328839571458));
#75647=CARTESIAN_POINT('Ctrl Pts',(94.6044999163115,805.519730494676,116.34660709602));
#75648=CARTESIAN_POINT('Ctrl Pts',(94.6289825954745,805.571900926472,116.364913180443));
#75649=CARTESIAN_POINT('Ctrl Pts',(94.7047464583719,805.771000674835,116.434309448738));
#75650=CARTESIAN_POINT('Ctrl Pts',(94.7295380823744,805.925516234931,116.487255225725));
#75651=CARTESIAN_POINT('Ctrl Pts',(94.7152848763623,806.234636238113,116.591857228622));
#75652=CARTESIAN_POINT('Ctrl Pts',(94.6766331985493,806.38631510761,116.642540137217));
#75653=CARTESIAN_POINT('Ctrl Pts',(94.5398841996231,806.66887360163,116.736272843806));
#75654=CARTESIAN_POINT('Ctrl Pts',(94.4425132835629,806.796813179746,116.778353844466));
#75655=CARTESIAN_POINT('Ctrl Pts',(94.2086716755231,807.003583131169,116.846114449512));
#75656=CARTESIAN_POINT('Ctrl Pts',(94.0768666383506,807.083124648092,116.872050269571));
#75657=CARTESIAN_POINT('Ctrl Pts',(93.7917530987918,807.191988806257,116.907335091828));
#75658=CARTESIAN_POINT('Ctrl Pts',(93.641165502188,807.221165990394,116.916640140119));
#75659=CARTESIAN_POINT('Ctrl Pts',(93.4805933409972,807.224289105858,116.91719520878));
#75660=CARTESIAN_POINT('Ctrl Pts',(93.4724127919216,807.224372547091,116.917198120831));
#75661=CARTESIAN_POINT('Ctrl Pts',(93.4642356337653,807.224380473639,116.917175693584));
#75662=CARTESIAN_POINT('Origin',(93.4642356337025,808.960586664488,108.225562747925));
#75663=CARTESIAN_POINT('',(93.4642356337025,807.297170032982,114.432457991414));
#75664=CARTESIAN_POINT('Origin',(93.4642356337025,806.825747802373,114.265841424147));
#75665=CARTESIAN_POINT('',(93.4642356337025,805.842078298429,118.549471098184));
#75666=CARTESIAN_POINT('',(93.4642356337025,809.432008895097,108.392179315193));
#75667=CARTESIAN_POINT('Origin',(93.4642356337025,805.37065606782,118.382854530917));
#75668=CARTESIAN_POINT('Origin',(53.889513810455,816.331424117056,110.830666102183));
#75669=CARTESIAN_POINT('',(53.889513810455,813.739855939514,121.340812944531));
#75670=CARTESIAN_POINT('Origin',(53.889513810455,812.741493520387,120.987957885174));
#75671=CARTESIAN_POINT('',(53.889513810455,814.406322208583,119.455124022096));
#75672=CARTESIAN_POINT('',(53.889513810455,817.329786536183,111.183521161539));
#75673=CARTESIAN_POINT('Origin',(53.889513810455,813.407959789456,119.102268962739));
#75674=CARTESIAN_POINT('Origin',(53.889513810455,816.331424117056,110.830666102183));
#75675=CARTESIAN_POINT('',(53.889513810455,814.668007485549,117.037561345671));
#75676=CARTESIAN_POINT('Origin',(53.889513810455,814.196585254941,116.870944778404));
#75677=CARTESIAN_POINT('',(53.889513810455,813.212915750996,121.154574452441));
#75678=CARTESIAN_POINT('',(53.889513810455,816.802846347665,110.99728266945));
#75679=CARTESIAN_POINT('Origin',(53.889513810455,812.741493520387,120.987957885174));
#75680=CARTESIAN_POINT('Origin',(55.83599078591,812.837155650029,109.595673394406));
#75681=CARTESIAN_POINT('',(55.83599078591,810.468994332743,120.184779780329));
#75682=CARTESIAN_POINT('Origin',(55.83599078591,809.247225053361,119.752965177398));
#75683=CARTESIAN_POINT('',(55.83599078591,811.135460601812,118.299090857894));
#75684=CARTESIAN_POINT('',(55.83599078591,814.058924929412,110.027487997337));
#75685=CARTESIAN_POINT('Origin',(55.83599078591,809.913691322429,117.867276254963));
#75686=CARTESIAN_POINT('Origin',(55.83599078591,812.837155650029,109.595673394406));
#75687=CARTESIAN_POINT('',(55.83599078591,811.173739018523,115.802568637895));
#75688=CARTESIAN_POINT('Origin',(55.83599078591,810.702316787914,115.635952070628));
#75689=CARTESIAN_POINT('',(55.83599078591,809.71864728397,119.919581744665));
#75690=CARTESIAN_POINT('',(55.83599078591,813.308577880638,109.762289961674));
#75691=CARTESIAN_POINT('Origin',(55.83599078591,809.247225053361,119.752965177398));
#75692=CARTESIAN_POINT('Origin',(58.6638984918342,809.238161778248,108.323667185117));
#75693=CARTESIAN_POINT('',(58.6638984918342,807.16294758358,119.016310996286));
#75694=CARTESIAN_POINT('Origin',(58.6638984918342,805.64823118158,118.480958968108));
#75695=CARTESIAN_POINT('',(58.6638984918342,807.829413852648,117.130622073851));
#75696=CARTESIAN_POINT('',(58.6638984918342,810.752878180249,108.859019213295));
#75697=CARTESIAN_POINT('Origin',(58.6638984918342,806.314697450648,116.595270045673));
#75698=CARTESIAN_POINT('Origin',(58.6638984918342,809.238161778248,108.323667185117));
#75699=CARTESIAN_POINT('',(58.6638984918342,807.574745146742,114.530562428605));
#75700=CARTESIAN_POINT('Origin',(58.6638984918342,807.103322916133,114.363945861338));
#75701=CARTESIAN_POINT('',(58.6638984918342,806.119653412188,118.647575535375));
#75702=CARTESIAN_POINT('',(58.6638984918342,809.709584008857,108.490283752384));
#75703=CARTESIAN_POINT('Origin',(58.6638984918342,805.64823118158,118.480958968108));
#75704=CARTESIAN_POINT('Origin',(62.2322687803016,806.339810201448,107.299291669698));
#75705=CARTESIAN_POINT('',(62.2322687803016,804.473491749226,118.065766304412));
#75706=CARTESIAN_POINT('Origin',(62.2322687803016,802.749879604779,117.45658345269));
#75707=CARTESIAN_POINT('',(62.2322687803016,805.139958018294,116.180077381977));
#75708=CARTESIAN_POINT('',(62.2322687803016,808.063422345894,107.908474521421));
#75709=CARTESIAN_POINT('Origin',(62.2322687803016,803.416345873847,115.570894530255));
#75710=CARTESIAN_POINT('Origin',(62.2322687803016,806.339810201448,107.299291669698));
#75711=CARTESIAN_POINT('',(62.2322687803016,804.676393569941,113.506186913187));
#75712=CARTESIAN_POINT('Origin',(62.2322687803016,804.204971339333,113.33957034592));
#75713=CARTESIAN_POINT('',(62.2322687803016,803.221301835388,117.623200019957));
#75714=CARTESIAN_POINT('',(62.2322687803016,806.811232432056,107.465908236965));
#75715=CARTESIAN_POINT('Origin',(62.2322687803016,802.749879604779,117.45658345269));
#75716=CARTESIAN_POINT('Origin',(66.491201753494,803.657837020177,106.351391600606));
#75717=CARTESIAN_POINT('',(66.491201753494,801.82010582107,117.127969937845));
#75718=CARTESIAN_POINT('Origin',(66.491201753494,800.067906423509,116.508683383598));
#75719=CARTESIAN_POINT('',(66.491201753494,802.486572090139,115.242281015409));
#75720=CARTESIAN_POINT('',(66.491201753494,805.410036417739,106.970678154853));
#75721=CARTESIAN_POINT('Origin',(66.491201753494,800.734372692577,114.622994461162));
#75722=CARTESIAN_POINT('Origin',(66.491201753494,803.657837020177,106.351391600606));
#75723=CARTESIAN_POINT('',(66.491201753494,801.994420388671,112.558286844094));
#75724=CARTESIAN_POINT('Origin',(66.491201753494,801.522998158062,112.391670276827));
#75725=CARTESIAN_POINT('',(66.491201753494,800.539328654118,116.675299950865));
#75726=CARTESIAN_POINT('',(66.491201753494,804.129259250786,106.518008167873));
#75727=CARTESIAN_POINT('Origin',(66.491201753494,800.067906423509,116.508683383598));
#75728=CARTESIAN_POINT('Origin',(76.705295723319,800.841936830322,105.356157195146));
#75729=CARTESIAN_POINT('',(76.705295723319,799.054221383694,116.150412791636));
#75730=CARTESIAN_POINT('Origin',(76.705295723319,797.252006233653,115.513448978138));
#75731=CARTESIAN_POINT('',(76.705295723319,799.720687652762,114.264723869201));
#75732=CARTESIAN_POINT('',(76.705295723319,802.644151980362,105.993121008645));
#75733=CARTESIAN_POINT('Origin',(76.705295723319,797.918472502722,113.627760055703));
#75734=CARTESIAN_POINT('Origin',(76.705295723319,800.841936830322,105.356157195146));
#75735=CARTESIAN_POINT('',(76.705295723319,799.178520198815,111.563052438635));
#75736=CARTESIAN_POINT('Origin',(76.705295723319,798.707097968207,111.396435871368));
#75737=CARTESIAN_POINT('',(76.705295723319,797.723428464262,115.680065545405));
#75738=CARTESIAN_POINT('',(76.705295723319,801.313359060931,105.522773762413));
#75739=CARTESIAN_POINT('Origin',(76.705295723319,797.252006233653,115.513448978138));
#75740=CARTESIAN_POINT('Origin',(81.986074755222,800.773039378479,105.331806504462));
#75741=CARTESIAN_POINT('',(81.986074755222,798.644207597608,116.00550004647));
#75742=CARTESIAN_POINT('Origin',(81.986074755222,797.183108781811,115.489098287453));
#75743=CARTESIAN_POINT('',(81.986074755222,799.310673866677,114.119811124035));
#75744=CARTESIAN_POINT('',(81.986074755222,802.234138194277,105.848208263479));
#75745=CARTESIAN_POINT('Origin',(81.986074755222,797.849575050879,113.603409365018));
#75746=CARTESIAN_POINT('Origin',(81.986074755222,800.773039378479,105.331806504462));
#75747=CARTESIAN_POINT('',(81.986074755222,799.109622746973,111.53870174795));
#75748=CARTESIAN_POINT('Origin',(81.986074755222,798.638200516364,111.372085180683));
#75749=CARTESIAN_POINT('',(81.986074755222,797.65453101242,115.65571485472));
#75750=CARTESIAN_POINT('',(81.986074755222,801.244461609088,105.498423071729));
#75751=CARTESIAN_POINT('Origin',(81.986074755222,797.183108781811,115.489098287453));
#75752=CARTESIAN_POINT('Origin',(88.0897914415438,801.449158030679,105.570769713196));
#75753=CARTESIAN_POINT('',(88.0897914415438,799.046609010973,116.147722321546));
#75754=CARTESIAN_POINT('Origin',(88.0897914415438,797.85922743401,115.728061496187));
#75755=CARTESIAN_POINT('',(88.0897914415438,799.713075280041,114.26203339911));
#75756=CARTESIAN_POINT('',(88.0897914415438,802.636539607641,105.990430538554));
#75757=CARTESIAN_POINT('',(88.0818786295781,799.713051841759,114.262025115228));
#75758=CARTESIAN_POINT('Ctrl Pts',(88.0897914415439,799.713075189938,114.262033654047));
#75759=CARTESIAN_POINT('Ctrl Pts',(88.0871539049629,799.71307525016,114.262033483656));
#75760=CARTESIAN_POINT('Ctrl Pts',(88.0845162887099,799.713067467756,114.262030637985));
#75761=CARTESIAN_POINT('Ctrl Pts',(88.0818786320383,799.713051841773,114.262025115233));
#75762=CARTESIAN_POINT('',(86.8481847291855,798.327017359201,113.772153631443));
#75763=CARTESIAN_POINT('Origin',(88.0897914415456,798.525693703079,113.842372573752));
#75764=CARTESIAN_POINT('Ctrl Pts',(86.8481847291853,798.327017359201,113.772153631443));
#75765=CARTESIAN_POINT('Ctrl Pts',(86.8732777827967,798.187614553342,113.722883963041));
#75766=CARTESIAN_POINT('Ctrl Pts',(86.9245897978729,798.053404494626,113.675765472785));
#75767=CARTESIAN_POINT('Ctrl Pts',(87.0759497888209,797.806226400021,113.590103995881));
#75768=CARTESIAN_POINT('Ctrl Pts',(87.175395175464,797.695659597608,113.552416534831));
#75769=CARTESIAN_POINT('Ctrl Pts',(87.4152056481323,797.509789549195,113.490659242545));
#75770=CARTESIAN_POINT('Ctrl Pts',(87.5547593194701,797.437488181679,113.467653643358));
#75771=CARTESIAN_POINT('Ctrl Pts',(87.8636603108241,797.342104587411,113.439778651934));
#75772=CARTESIAN_POINT('Ctrl Pts',(88.0312450181269,797.323225684679,113.436363055552));
#75773=CARTESIAN_POINT('Ctrl Pts',(88.3632841086485,797.348255821918,113.451184557132));
#75774=CARTESIAN_POINT('Ctrl Pts',(88.5244927455475,797.391644793613,113.469166685792));
#75775=CARTESIAN_POINT('Ctrl Pts',(88.8183412166434,797.53491086785,113.523492248324));
#75776=CARTESIAN_POINT('Ctrl Pts',(88.9483219827927,797.633000225401,113.559169764669));
#75777=CARTESIAN_POINT('Ctrl Pts',(89.0544629787952,797.752247860836,113.601315913876));
#75778=CARTESIAN_POINT('Ctrl Pts',(89.0932835708438,797.795862147326,113.616730678448));
#75779=CARTESIAN_POINT('Ctrl Pts',(89.1287264319009,797.842094141095,113.63293791794));
#75780=CARTESIAN_POINT('Ctrl Pts',(89.2466718610917,798.021997890187,113.695549670579));
#75781=CARTESIAN_POINT('Ctrl Pts',(89.304879410181,798.168288485704,113.745588466786));
#75782=CARTESIAN_POINT('Ctrl Pts',(89.3587811135626,798.47347944388,113.848801812235));
#75783=CARTESIAN_POINT('Ctrl Pts',(89.3542188988618,798.629440678153,113.900998253439));
#75784=CARTESIAN_POINT('Ctrl Pts',(89.2823417683743,798.932673384468,114.002037926182));
#75785=CARTESIAN_POINT('Ctrl Pts',(89.2150939301468,799.0769261784,114.049884569284));
#75786=CARTESIAN_POINT('Ctrl Pts',(89.0315897645301,799.325053821448,114.132262381922));
#75787=CARTESIAN_POINT('Ctrl Pts',(88.9200542919387,799.428709639743,114.166721012014));
#75788=CARTESIAN_POINT('Ctrl Pts',(88.6649562731285,799.591107113575,114.220926319372));
#75789=CARTESIAN_POINT('Ctrl Pts',(88.5240236153877,799.649173064636,114.240441635371));
#75790=CARTESIAN_POINT('Ctrl Pts',(88.2816857573755,799.702680388928,114.258502734602));
#75791=CARTESIAN_POINT('Ctrl Pts',(88.1857913741578,799.713072997999,114.262039855884));
#75792=CARTESIAN_POINT('Ctrl Pts',(88.0897914415439,799.713075189938,114.262033654047));
#75793=CARTESIAN_POINT('Origin',(88.0897914415438,801.449158030679,105.570769713196));
#75794=CARTESIAN_POINT('',(88.0897914415438,799.785741399173,111.777664956684));
#75795=CARTESIAN_POINT('Origin',(88.0897914415438,799.314319168564,111.611048389417));
#75796=CARTESIAN_POINT('',(88.0897914415438,798.330649664619,115.894678063454));
#75797=CARTESIAN_POINT('',(88.0897914415438,801.920580261288,105.737386280463));
#75798=CARTESIAN_POINT('Origin',(88.0897914415438,797.85922743401,115.728061496187));
#75799=CARTESIAN_POINT('Origin',(51.005255154091,816.416693850066,110.860803311002));
#75800=CARTESIAN_POINT('',(51.005255154091,813.825125672524,121.37095015335));
#75801=CARTESIAN_POINT('Origin',(51.005255154091,812.826763253397,121.018095093994));
#75802=CARTESIAN_POINT('',(51.005255154091,814.491591941593,119.485261230915));
#75803=CARTESIAN_POINT('',(51.005255154091,817.415056269193,111.213658370359));
#75804=CARTESIAN_POINT('Origin',(51.005255154091,813.493229522466,119.132406171558));
#75805=CARTESIAN_POINT('Origin',(51.005255154091,816.416693850066,110.860803311002));
#75806=CARTESIAN_POINT('',(51.005255154091,814.75327721856,117.067698554491));
#75807=CARTESIAN_POINT('Origin',(51.005255154091,814.281854987951,116.901081987224));
#75808=CARTESIAN_POINT('',(51.005255154091,813.298185484006,121.184711661261));
#75809=CARTESIAN_POINT('',(51.005255154091,816.888116080675,111.027419878269));
#75810=CARTESIAN_POINT('Origin',(51.005255154091,812.826763253397,121.018095093994));
#75811=CARTESIAN_POINT('Origin',(52.1386570499375,812.617218792626,109.51794026725));
#75812=CARTESIAN_POINT('',(52.1386570499375,810.24905747534,120.107046653173));
#75813=CARTESIAN_POINT('Origin',(52.1386570499375,809.027288195957,119.675232050242));
#75814=CARTESIAN_POINT('',(52.1386570499375,810.915523744408,118.221357730738));
#75815=CARTESIAN_POINT('',(52.1386570499375,813.838988072009,109.949754870181));
#75816=CARTESIAN_POINT('Origin',(52.1386570499375,809.693754465026,117.789543127807));
#75817=CARTESIAN_POINT('Origin',(52.1386570499375,812.617218792626,109.51794026725));
#75818=CARTESIAN_POINT('',(52.1386570499375,810.95380216112,115.724835510739));
#75819=CARTESIAN_POINT('Origin',(52.1386570499375,810.482379930511,115.558218943472));
#75820=CARTESIAN_POINT('',(52.1386570499375,809.498710426566,119.841848617509));
#75821=CARTESIAN_POINT('',(52.1386570499375,813.088641023235,109.684556834518));
#75822=CARTESIAN_POINT('Origin',(52.1386570499375,809.027288195957,119.675232050242));
#75823=CARTESIAN_POINT('Origin',(54.1111347391161,808.542521388227,108.077804333703));
#75824=CARTESIAN_POINT('',(54.1111347391161,806.467307193559,118.770448144872));
#75825=CARTESIAN_POINT('Origin',(54.1111347391161,804.952590791559,118.235096116694));
#75826=CARTESIAN_POINT('',(54.1111347391161,807.133773462628,116.884759222436));
#75827=CARTESIAN_POINT('',(54.1111347391161,810.057237790228,108.61315636188));
#75828=CARTESIAN_POINT('Origin',(54.1111347391161,805.619057060627,116.349407194259));
#75829=CARTESIAN_POINT('Origin',(54.1111347391161,808.542521388227,108.077804333703));
#75830=CARTESIAN_POINT('',(54.1111347391161,806.879104756721,114.284699577191));
#75831=CARTESIAN_POINT('Origin',(54.1111347391161,806.407682526112,114.118083009924));
#75832=CARTESIAN_POINT('',(54.1111347391161,805.424013022167,118.401712683961));
#75833=CARTESIAN_POINT('',(54.1111347391161,809.013943618836,108.24442090097));
#75834=CARTESIAN_POINT('Origin',(54.1111347391161,804.952590791559,118.235096116694));
#75835=CARTESIAN_POINT('Origin',(56.9623965184881,805.008003878606,106.828586252413));
#75836=CARTESIAN_POINT('',(56.9623965184881,803.141685426384,117.595060887126));
#75837=CARTESIAN_POINT('Origin',(56.9623965184881,801.418073281937,116.985878035404));
#75838=CARTESIAN_POINT('',(56.9623965184881,803.808151695452,115.709371964691));
#75839=CARTESIAN_POINT('',(56.9623965184881,806.731616023053,107.437769104135));
#75840=CARTESIAN_POINT('Origin',(56.9623965184881,802.084539551006,115.100189112969));
#75841=CARTESIAN_POINT('Origin',(56.9623965184881,805.008003878606,106.828586252413));
#75842=CARTESIAN_POINT('',(56.9623965184881,803.3445872471,113.035481495901));
#75843=CARTESIAN_POINT('Origin',(56.9623965184881,802.873165016491,112.868864928634));
#75844=CARTESIAN_POINT('',(56.9623965184881,801.889495512546,117.152494602671));
#75845=CARTESIAN_POINT('',(56.9623965184881,805.479426109215,106.99520281968));
#75846=CARTESIAN_POINT('Origin',(56.9623965184881,801.418073281937,116.985878035404));
#75847=CARTESIAN_POINT('Origin',(60.5368452920206,801.549766488829,105.606328146478));
#75848=CARTESIAN_POINT('',(60.5368452920206,799.712035289722,116.382906483716));
#75849=CARTESIAN_POINT('Origin',(60.5368452920206,797.959835892161,115.763619929469));
#75850=CARTESIAN_POINT('',(60.5368452920206,800.37850155879,114.497217561281));
#75851=CARTESIAN_POINT('',(60.5368452920206,803.301965886391,106.225614700725));
#75852=CARTESIAN_POINT('Origin',(60.5368452920206,798.626302161229,113.877931007034));
#75853=CARTESIAN_POINT('Origin',(60.5368452920206,801.549766488829,105.606328146478));
#75854=CARTESIAN_POINT('',(60.5368452920206,799.886349857323,111.813223389966));
#75855=CARTESIAN_POINT('Origin',(60.5368452920206,799.414927626714,111.646606822699));
#75856=CARTESIAN_POINT('',(60.5368452920206,798.431258122769,115.930236496736));
#75857=CARTESIAN_POINT('',(60.5368452920206,802.021188719438,105.772944713745));
#75858=CARTESIAN_POINT('Origin',(60.5368452920206,797.959835892161,115.763619929469));
#75859=CARTESIAN_POINT('Origin',(64.6327834569077,799.263354525339,104.798232795898));
#75860=CARTESIAN_POINT('',(64.6327834569077,797.382666277051,115.559628658467));
#75861=CARTESIAN_POINT('Origin',(64.6327834569077,795.67342392867,114.955524578889));
#75862=CARTESIAN_POINT('',(64.6327834569077,798.049132546119,113.673939736032));
#75863=CARTESIAN_POINT('',(64.6327834569077,800.972596873719,105.402336875476));
#75864=CARTESIAN_POINT('Origin',(64.6327834569077,796.339890197738,113.069835656454));
#75865=CARTESIAN_POINT('Origin',(64.6327834569077,799.263354525339,104.798232795898));
#75866=CARTESIAN_POINT('',(64.6327834569077,797.599937893832,111.005128039386));
#75867=CARTESIAN_POINT('Origin',(64.6327834569077,797.128515663224,110.838511472119));
#75868=CARTESIAN_POINT('',(64.6327834569077,796.144846159279,115.122141146156));
#75869=CARTESIAN_POINT('',(64.6327834569077,799.734776755947,104.964849363165));
#75870=CARTESIAN_POINT('Origin',(64.6327834569077,795.67342392867,114.955524578889));
#75871=CARTESIAN_POINT('Origin',(69.9067875431667,796.793148117736,103.925178269928));
#75872=CARTESIAN_POINT('',(69.9067875431667,795.005432671108,114.719433866418));
#75873=CARTESIAN_POINT('Origin',(69.9067875431667,793.203217521068,114.082470052919));
#75874=CARTESIAN_POINT('',(69.9067875431667,795.671898940177,112.833744943982));
#75875=CARTESIAN_POINT('',(69.9067875431667,798.595363267777,104.562142083426));
#75876=CARTESIAN_POINT('Origin',(69.9067875431667,793.869683790136,112.196781130484));
#75877=CARTESIAN_POINT('Origin',(69.9067875431667,796.793148117736,103.925178269928));
#75878=CARTESIAN_POINT('',(69.9067875431667,795.12973148623,110.132073513416));
#75879=CARTESIAN_POINT('Origin',(69.9067875431667,794.658309255621,109.965456946149));
#75880=CARTESIAN_POINT('',(69.9067875431667,793.674639751676,114.249086620186));
#75881=CARTESIAN_POINT('',(69.9067875431667,797.264570348345,104.091794837195));
#75882=CARTESIAN_POINT('Origin',(69.9067875431667,793.203217521068,114.082470052919));
#75883=CARTESIAN_POINT('Origin',(75.0569759364645,795.690573649493,103.535491146311));
#75884=CARTESIAN_POINT('',(75.0569759364645,793.561741868622,114.209184688319));
#75885=CARTESIAN_POINT('Origin',(75.0569759364645,792.100643052824,113.692782929302));
#75886=CARTESIAN_POINT('',(75.0569759364645,794.22820813769,112.323495765884));
#75887=CARTESIAN_POINT('',(75.0569759364645,797.151672465291,104.051892905328));
#75888=CARTESIAN_POINT('Origin',(75.0569759364645,792.767109321893,111.807094006867));
#75889=CARTESIAN_POINT('Origin',(75.0569759364645,795.690573649493,103.535491146311));
#75890=CARTESIAN_POINT('',(75.0569759364645,794.027157017987,109.742386389799));
#75891=CARTESIAN_POINT('Origin',(75.0569759364645,793.555734787378,109.575769822532));
#75892=CARTESIAN_POINT('',(75.0569759364645,792.572065283433,113.859399496569));
#75893=CARTESIAN_POINT('',(75.0569759364645,796.161995880102,103.702107713578));
#75894=CARTESIAN_POINT('Origin',(75.0569759364645,792.100643052824,113.692782929302));
#75895=CARTESIAN_POINT('Origin',(81.1764063203475,795.155415755662,103.346348239111));
#75896=CARTESIAN_POINT('',(81.1764063203475,792.752866735955,113.923300847461));
#75897=CARTESIAN_POINT('Origin',(81.1764063203475,791.565485158993,113.503640022102));
#75898=CARTESIAN_POINT('',(81.1764063203475,793.419333005024,112.037611925025));
#75899=CARTESIAN_POINT('',(81.1764063203475,796.342797332624,103.766009064469));
#75900=CARTESIAN_POINT('',(79.9181205070459,792.281006798982,111.63528892758));
#75901=CARTESIAN_POINT('Origin',(81.1764063203493,792.231951428062,111.617951099667));
#75902=CARTESIAN_POINT('',(81.4304971360407,793.394914078383,112.028981450115));
#75903=CARTESIAN_POINT('Ctrl Pts',(81.4304971360405,793.394914078382,112.028981450115));
#75904=CARTESIAN_POINT('Ctrl Pts',(81.5271123948389,793.37614905845,112.022349257141));
#75905=CARTESIAN_POINT('Ctrl Pts',(81.6212624745287,793.346663326874,112.012062193114));
#75906=CARTESIAN_POINT('Ctrl Pts',(81.8489627698746,793.245751417097,111.977255759942));
#75907=CARTESIAN_POINT('Ctrl Pts',(81.9740810553385,793.161320630065,111.948422218836));
#75908=CARTESIAN_POINT('Ctrl Pts',(82.1880145458838,792.952443566045,111.877789451628));
#75909=CARTESIAN_POINT('Ctrl Pts',(82.2744058185353,792.82917381175,111.8363985929));
#75910=CARTESIAN_POINT('Ctrl Pts',(82.3995525291408,792.550459809467,111.743210525993));
#75911=CARTESIAN_POINT('Ctrl Pts',(82.4337382363144,792.396155260957,111.691811252713));
#75912=CARTESIAN_POINT('Ctrl Pts',(82.4376021228561,792.085416851161,111.588118810398));
#75913=CARTESIAN_POINT('Ctrl Pts',(82.4078754837702,791.931949334495,111.536803733373));
#75914=CARTESIAN_POINT('Ctrl Pts',(82.2881746340815,791.643961859157,111.439670680854));
#75915=CARTESIAN_POINT('Ctrl Pts',(82.1990951091111,791.512266962877,111.394790498615));
#75916=CARTESIAN_POINT('Ctrl Pts',(82.0441228948492,791.35940851878,111.341737471862));
#75917=CARTESIAN_POINT('Ctrl Pts',(81.9992688749996,791.321133700687,111.328342567492));
#75918=CARTESIAN_POINT('Ctrl Pts',(81.9516789857087,791.286082429006,111.31595426209));
#75919=CARTESIAN_POINT('Ctrl Pts',(81.8215614892368,791.190247288659,111.282082880829));
#75920=CARTESIAN_POINT('Ctrl Pts',(81.6727209685682,791.119788269131,111.256170860838));
#75921=CARTESIAN_POINT('Ctrl Pts',(81.353445732818,791.037280881806,111.223319474081));
#75922=CARTESIAN_POINT('Ctrl Pts',(81.1860085643421,791.026459705763,111.216847906364));
#75923=CARTESIAN_POINT('Ctrl Pts',(80.8552918281437,791.067106646942,111.225238906537));
#75924=CARTESIAN_POINT('Ctrl Pts',(80.6953066925941,791.118446720726,111.240127379119));
#75925=CARTESIAN_POINT('Ctrl Pts',(80.4137850859091,791.27233939135,111.288681457831));
#75926=CARTESIAN_POINT('Ctrl Pts',(80.2930480159152,791.370434776423,111.320803535585));
#75927=CARTESIAN_POINT('Ctrl Pts',(80.0991925175211,791.599279798184,111.397749637547));
#75928=CARTESIAN_POINT('Ctrl Pts',(80.0262055857992,791.72693411675,111.441476404976));
#75929=CARTESIAN_POINT('Ctrl Pts',(79.9325419863974,791.998393300873,111.535719640487));
#75930=CARTESIAN_POINT('Ctrl Pts',(79.9119247565683,792.139731328094,111.585357395993));
#75931=CARTESIAN_POINT('Ctrl Pts',(79.9181205070457,792.281006798982,111.63528892758));
#75932=CARTESIAN_POINT('Origin',(81.1764063203493,792.231951428062,111.617951099667));
#75933=CARTESIAN_POINT('Origin',(81.1764063203475,795.155415755662,103.346348239111));
#75934=CARTESIAN_POINT('',(81.1764063203475,793.491999124156,109.553243482599));
#75935=CARTESIAN_POINT('Origin',(81.1764063203475,793.020576893547,109.386626915332));
#75936=CARTESIAN_POINT('',(81.1764063203475,792.036907389602,113.670256589369));
#75937=CARTESIAN_POINT('',(81.1764063203475,795.626837986271,103.512964806378));
#75938=CARTESIAN_POINT('Origin',(81.1764063203475,791.565485158993,113.503640022102));
#75939=CARTESIAN_POINT('Origin',(48.2028277557997,817.065496804356,111.090112227845));
#75940=CARTESIAN_POINT('',(48.2028277557997,814.473928626814,121.600259070193));
#75941=CARTESIAN_POINT('Origin',(48.2028277557997,813.475566207687,121.247404010836));
#75942=CARTESIAN_POINT('',(48.2028277557997,815.140394895883,119.714570147758));
#75943=CARTESIAN_POINT('',(48.2028277557997,818.063859223483,111.442967287202));
#75944=CARTESIAN_POINT('Origin',(48.2028277557997,814.142032476756,119.361715088401));
#75945=CARTESIAN_POINT('Origin',(48.2028277557997,817.065496804356,111.090112227845));
#75946=CARTESIAN_POINT('',(48.2028277557997,815.402080172849,117.297007471333));
#75947=CARTESIAN_POINT('Origin',(48.2028277557997,814.930657942241,117.130390904066));
#75948=CARTESIAN_POINT('',(48.2028277557997,813.946988438296,121.414020578103));
#75949=CARTESIAN_POINT('',(48.2028277557997,817.536919034965,111.256728795112));
#75950=CARTESIAN_POINT('Origin',(48.2028277557997,813.475566207687,121.247404010836));
#75951=CARTESIAN_POINT('Origin',(48.4736194705231,813.126870448416,109.698068406902));
#75952=CARTESIAN_POINT('',(48.4736194705231,810.75870913113,120.287174792824));
#75953=CARTESIAN_POINT('Origin',(48.4736194705231,809.536939851748,119.855360189893));
#75954=CARTESIAN_POINT('',(48.4736194705231,811.425175400199,118.401485870389));
#75955=CARTESIAN_POINT('',(48.4736194705231,814.348639727799,110.129883009833));
#75956=CARTESIAN_POINT('Origin',(48.4736194705231,810.203406120816,117.969671267458));
#75957=CARTESIAN_POINT('Origin',(48.4736194705231,813.126870448416,109.698068406902));
#75958=CARTESIAN_POINT('',(48.4736194705231,811.46345381691,115.90496365039));
#75959=CARTESIAN_POINT('Origin',(48.4736194705231,810.992031586301,115.738347083123));
#75960=CARTESIAN_POINT('',(48.4736194705231,810.008362082356,120.02197675716));
#75961=CARTESIAN_POINT('',(48.4736194705231,813.598292679025,109.864684974169));
#75962=CARTESIAN_POINT('Origin',(48.4736194705231,809.536939851748,119.855360189893));
#75963=CARTESIAN_POINT('Origin',(49.5044604029411,808.75455334054,108.15274359993));
#75964=CARTESIAN_POINT('',(49.5044604029411,806.679339145872,118.845387411099));
#75965=CARTESIAN_POINT('Origin',(49.5044604029411,805.164622743871,118.310035382922));
#75966=CARTESIAN_POINT('',(49.5044604029411,807.34580541494,116.959698488664));
#75967=CARTESIAN_POINT('',(49.5044604029411,810.269269742541,108.688095628108));
#75968=CARTESIAN_POINT('Origin',(49.5044604029411,805.83108901294,116.424346460486));
#75969=CARTESIAN_POINT('Origin',(49.5044604029411,808.75455334054,108.15274359993));
#75970=CARTESIAN_POINT('',(49.5044604029411,807.091136709034,114.359638843419));
#75971=CARTESIAN_POINT('Origin',(49.5044604029411,806.619714478425,114.193022276152));
#75972=CARTESIAN_POINT('',(49.5044604029411,805.63604497448,118.476651950189));
#75973=CARTESIAN_POINT('',(49.5044604029411,809.225975571149,108.319360167197));
#75974=CARTESIAN_POINT('Origin',(49.5044604029411,805.164622743871,118.310035382922));
#75975=CARTESIAN_POINT('Origin',(51.513999851587,804.738345273765,106.733279777335));
#75976=CARTESIAN_POINT('',(51.513999851587,802.872026821543,117.499754412049));
#75977=CARTESIAN_POINT('Origin',(51.513999851587,801.148414677097,116.890571560326));
#75978=CARTESIAN_POINT('',(51.513999851587,803.538493090612,115.614065489613));
#75979=CARTESIAN_POINT('',(51.513999851587,806.461957418212,107.342462629057));
#75980=CARTESIAN_POINT('Origin',(51.513999851587,801.814880946165,115.004882637891));
#75981=CARTESIAN_POINT('Origin',(51.513999851587,804.738345273765,106.733279777335));
#75982=CARTESIAN_POINT('',(51.513999851587,803.074928642259,112.940175020823));
#75983=CARTESIAN_POINT('Origin',(51.513999851587,802.60350641165,112.773558453556));
#75984=CARTESIAN_POINT('',(51.513999851587,801.619836907705,117.057188127593));
#75985=CARTESIAN_POINT('',(51.513999851587,805.209767504374,106.899896344602));
#75986=CARTESIAN_POINT('Origin',(51.513999851587,801.148414677097,116.890571560326));
#75987=CARTESIAN_POINT('Origin',(54.2477438619482,800.654985243879,105.290082178832));
#75988=CARTESIAN_POINT('',(54.2477438619482,798.817254044772,116.066660516071));
#75989=CARTESIAN_POINT('Origin',(54.2477438619482,797.06505464721,115.447373961824));
#75990=CARTESIAN_POINT('',(54.2477438619482,799.48372031384,114.180971593635));
#75991=CARTESIAN_POINT('',(54.2477438619482,802.40718464144,105.909368733079));
#75992=CARTESIAN_POINT('Origin',(54.2477438619482,797.731520916278,113.561685039388));
#75993=CARTESIAN_POINT('Origin',(54.2477438619482,800.654985243879,105.290082178832));
#75994=CARTESIAN_POINT('',(54.2477438619482,798.991568612372,111.496977422321));
#75995=CARTESIAN_POINT('Origin',(54.2477438619482,798.520146381764,111.330360855054));
#75996=CARTESIAN_POINT('',(54.2477438619482,797.536476877819,115.613990529091));
#75997=CARTESIAN_POINT('',(54.2477438619482,801.126407474487,105.456698746099));
#75998=CARTESIAN_POINT('Origin',(54.2477438619482,797.06505464721,115.447373961824));
#75999=CARTESIAN_POINT('Origin',(57.7499869812552,797.615616719433,104.215866502688));
#76000=CARTESIAN_POINT('',(57.7499869812552,795.734928471145,114.977262365258));
#76001=CARTESIAN_POINT('Origin',(57.7499869812552,794.025686122764,114.37315828568));
#76002=CARTESIAN_POINT('',(57.7499869812552,796.401394740213,113.091573442823));
#76003=CARTESIAN_POINT('',(57.7499869812552,799.324859067813,104.819970582266));
#76004=CARTESIAN_POINT('Origin',(57.7499869812552,794.692152391833,112.487469363244));
#76005=CARTESIAN_POINT('Origin',(57.7499869812552,797.615616719433,104.215866502688));
#76006=CARTESIAN_POINT('',(57.7499869812552,795.952200087927,110.422761746176));
#76007=CARTESIAN_POINT('Origin',(57.7499869812552,795.480777857318,110.256145178909));
#76008=CARTESIAN_POINT('',(57.7499869812552,794.497108353373,114.539774852947));
#76009=CARTESIAN_POINT('',(57.7499869812552,798.087038950042,104.382483069955));
#76010=CARTESIAN_POINT('Origin',(57.7499869812552,794.025686122764,114.37315828568));
#76011=CARTESIAN_POINT('Origin',(62.364022956069,794.165535739153,102.996491147849));
#76012=CARTESIAN_POINT('',(62.364022956069,792.377820292525,113.790746744339));
#76013=CARTESIAN_POINT('Origin',(62.364022956069,790.575605142485,113.15378293084));
#76014=CARTESIAN_POINT('',(62.364022956069,793.044286561593,111.905057821903));
#76015=CARTESIAN_POINT('',(62.364022956069,795.967750889194,103.633454961347));
#76016=CARTESIAN_POINT('Origin',(62.364022956069,791.242071411553,111.268094008405));
#76017=CARTESIAN_POINT('Origin',(62.364022956069,794.165535739153,102.996491147849));
#76018=CARTESIAN_POINT('',(62.364022956069,792.502119107647,109.203386391337));
#76019=CARTESIAN_POINT('Origin',(62.364022956069,792.030696877038,109.03676982407));
#76020=CARTESIAN_POINT('',(62.364022956069,791.047027373093,113.320399498107));
#76021=CARTESIAN_POINT('',(62.364022956069,794.636957969762,103.163107715116));
#76022=CARTESIAN_POINT('Origin',(62.364022956069,790.575605142485,113.15378293084));
#76023=CARTESIAN_POINT('Origin',(67.1585327646285,792.07747204951,102.258498788528));
#76024=CARTESIAN_POINT('',(67.1585327646285,789.94864026864,112.932192330537));
#76025=CARTESIAN_POINT('Origin',(67.1585327646285,788.487541452842,112.415790571519));
#76026=CARTESIAN_POINT('',(67.1585327646285,790.615106537832,111.04650340775));
#76027=CARTESIAN_POINT('',(67.1585327646285,793.538570865308,102.774900547545));
#76028=CARTESIAN_POINT('',(66.4584822850693,787.85048959706,110.069394238124));
#76029=CARTESIAN_POINT('Origin',(67.1585327646304,789.15400772191,110.530101649084));
#76030=CARTESIAN_POINT('',(67.5288831447128,787.735245668087,110.028663134249));
#76031=CARTESIAN_POINT('Ctrl Pts',(67.5288733605052,787.735245035326,110.02866291061));
#76032=CARTESIAN_POINT('Ctrl Pts',(67.4671620849654,787.720925260318,110.0236018176));
#76033=CARTESIAN_POINT('Ctrl Pts',(67.4045749097962,787.710195046386,110.019819666768));
#76034=CARTESIAN_POINT('Ctrl Pts',(67.2548610344048,787.693405932515,110.013913398071));
#76035=CARTESIAN_POINT('Ctrl Pts',(67.1675407850101,787.690603920603,110.012940933692));
#76036=CARTESIAN_POINT('Ctrl Pts',(67.0416065082334,787.696591904374,110.015068146693));
#76037=CARTESIAN_POINT('Ctrl Pts',(67.0028641856055,787.699815903729,110.016209079711));
#76038=CARTESIAN_POINT('Ctrl Pts',(66.8821639275677,787.714194190606,110.021288906651));
#76039=CARTESIAN_POINT('Ctrl Pts',(66.8009995388376,787.730169587177,110.026923647079));
#76040=CARTESIAN_POINT('Ctrl Pts',(66.6308922483411,787.777315396607,110.043554166242));
#76041=CARTESIAN_POINT('Ctrl Pts',(66.5428214394692,787.8102254516,110.055163526352));
#76042=CARTESIAN_POINT('Ctrl Pts',(66.4584818949366,787.850490113391,110.069394420613));
#76043=CARTESIAN_POINT('Origin',(67.1585327646304,789.15400772191,110.530101649084));
#76044=CARTESIAN_POINT('Origin',(67.1585327646285,792.07747204951,102.258498788528));
#76045=CARTESIAN_POINT('',(67.1585327646285,790.414055418004,108.465394032016));
#76046=CARTESIAN_POINT('Origin',(67.1585327646285,789.942633187395,108.298777464749));
#76047=CARTESIAN_POINT('',(67.1585327646285,788.958963683451,112.582407138786));
#76048=CARTESIAN_POINT('',(67.1585327646285,792.548894280119,102.425115355795));
#76049=CARTESIAN_POINT('Origin',(67.1585327646285,788.487541452842,112.415790571519));
#76050=CARTESIAN_POINT('Origin',(73.0262283740121,790.354426577582,101.649516218047));
#76051=CARTESIAN_POINT('',(73.0262283740121,787.951877557875,112.226468826397));
#76052=CARTESIAN_POINT('Origin',(73.0262283740121,786.764495980913,111.806808001039));
#76053=CARTESIAN_POINT('',(73.0262283740121,788.618343826943,110.340779903962));
#76054=CARTESIAN_POINT('',(73.0262283740121,791.541808154543,102.069177043406));
#76055=CARTESIAN_POINT('',(71.8612276196213,787.881917432482,110.080501898549));
#76056=CARTESIAN_POINT('Origin',(73.026228374014,787.430962249982,109.921119078603));
#76057=CARTESIAN_POINT('',(73.547638647088,788.511793322879,110.303121350599));
#76058=CARTESIAN_POINT('Ctrl Pts',(73.5476386478411,788.511793322897,110.303121350605));
#76059=CARTESIAN_POINT('Ctrl Pts',(73.6411231849667,788.471702806277,110.288952005535));
#76060=CARTESIAN_POINT('Ctrl Pts',(73.729056042615,788.420935975636,110.271151656072));
#76061=CARTESIAN_POINT('Ctrl Pts',(73.8817794828457,788.306353346367,110.231343155525));
#76062=CARTESIAN_POINT('Ctrl Pts',(73.9475471629768,788.244719253655,110.21006215985));
#76063=CARTESIAN_POINT('Ctrl Pts',(74.1079933820161,788.056975966865,110.145666872752));
#76064=CARTESIAN_POINT('Ctrl Pts',(74.1848486425081,787.919355348459,110.098916903248));
#76065=CARTESIAN_POINT('Ctrl Pts',(74.2760595756327,787.632863603953,110.002393768381));
#76066=CARTESIAN_POINT('Ctrl Pts',(74.293203957499,787.48758429983,109.953778221984));
#76067=CARTESIAN_POINT('Ctrl Pts',(74.2724489890072,787.207171966388,109.860239043525));
#76068=CARTESIAN_POINT('Ctrl Pts',(74.2380363542724,787.074013924212,109.815948173723));
#76069=CARTESIAN_POINT('Ctrl Pts',(74.1139149291181,786.803724199413,109.725899152577));
#76070=CARTESIAN_POINT('Ctrl Pts',(74.0171882043694,786.672308121852,109.682008166697));
#76071=CARTESIAN_POINT('Ctrl Pts',(73.8348841099355,786.50725247843,109.62630802448));
#76072=CARTESIAN_POINT('Ctrl Pts',(73.7677840018365,786.457770970221,109.609493877455));
#76073=CARTESIAN_POINT('Ctrl Pts',(73.6505262673303,786.388126103038,109.58558761328));
#76074=CARTESIAN_POINT('Ctrl Pts',(73.6033367136151,786.363944979445,109.577219223496));
#76075=CARTESIAN_POINT('Ctrl Pts',(73.5335192615212,786.333479727438,109.56656518841));
#76076=CARTESIAN_POINT('Ctrl Pts',(73.5121115414431,786.324815433283,109.563518615732));
#76077=CARTESIAN_POINT('Ctrl Pts',(73.4426717754365,786.298855829668,109.554334034923));
#76078=CARTESIAN_POINT('Ctrl Pts',(73.3937666214844,786.283794470383,109.54891317807));
#76079=CARTESIAN_POINT('Ctrl Pts',(73.2703323690151,786.253590252978,109.537774593641));
#76080=CARTESIAN_POINT('Ctrl Pts',(73.1950539083946,786.241959394905,109.533192361749));
#76081=CARTESIAN_POINT('Ctrl Pts',(72.9593318182645,786.226155947848,109.525592239343));
#76082=CARTESIAN_POINT('Ctrl Pts',(72.7987636659693,786.244536878615,109.529949011691));
#76083=CARTESIAN_POINT('Ctrl Pts',(72.5106810113424,786.332088715488,109.555992921144));
#76084=CARTESIAN_POINT('Ctrl Pts',(72.3835460494303,786.394616632969,109.575470922408));
#76085=CARTESIAN_POINT('Ctrl Pts',(72.1492360872349,786.562230779967,109.629231584724));
#76086=CARTESIAN_POINT('Ctrl Pts',(72.0457494325479,786.668422647191,109.663950958307));
#76087=CARTESIAN_POINT('Ctrl Pts',(71.8785559577171,786.91713604384,109.746731912045));
#76088=CARTESIAN_POINT('Ctrl Pts',(71.8190264473306,787.059150796,109.794708006097));
#76089=CARTESIAN_POINT('Ctrl Pts',(71.7675659500907,787.314715553241,109.882254532013));
#76090=CARTESIAN_POINT('Ctrl Pts',(71.761632694651,787.423919352526,109.920009091735));
#76091=CARTESIAN_POINT('Ctrl Pts',(71.7824174870735,787.652537898065,109.99966247971));
#76092=CARTESIAN_POINT('Ctrl Pts',(71.812679350666,787.770424668557,110.04109658337));
#76093=CARTESIAN_POINT('Ctrl Pts',(71.8612276196214,787.881917432482,110.080501898549));
#76094=CARTESIAN_POINT('Origin',(73.026228374014,787.430962249982,109.921119078603));
#76095=CARTESIAN_POINT('Origin',(73.0262283740121,790.354426577582,101.649516218047));
#76096=CARTESIAN_POINT('',(73.0262283740121,788.691009946075,107.856411461535));
#76097=CARTESIAN_POINT('Origin',(73.0262283740121,788.219587715466,107.689794894268));
#76098=CARTESIAN_POINT('',(73.0262283740121,787.235918211521,111.973424568306));
#76099=CARTESIAN_POINT('',(73.0262283740121,790.82584880819,101.816132785314));
#76100=CARTESIAN_POINT('Origin',(73.0262283740121,786.764495980913,111.806808001039));
#76101=CARTESIAN_POINT('Origin',(45.6047111404246,818.24947717752,111.508570952699));
#76102=CARTESIAN_POINT('',(45.6047111404246,815.657908999979,122.018717795047));
#76103=CARTESIAN_POINT('Origin',(45.6047111404246,814.659546580852,121.66586273569));
#76104=CARTESIAN_POINT('',(45.6047111404246,816.324375269047,120.133028872612));
#76105=CARTESIAN_POINT('',(45.6047111404246,819.247839596648,111.861426012055));
#76106=CARTESIAN_POINT('Origin',(45.6047111404246,815.32601284992,119.780173813255));
#76107=CARTESIAN_POINT('Origin',(45.6047111404246,818.24947717752,111.508570952699));
#76108=CARTESIAN_POINT('',(45.6047111404246,816.586060546014,117.715466196187));
#76109=CARTESIAN_POINT('Origin',(45.6047111404246,816.114638315406,117.54884962892));
#76110=CARTESIAN_POINT('',(45.6047111404246,815.130968811461,121.832479302957));
#76111=CARTESIAN_POINT('',(45.6047111404246,818.720899408129,111.675187519966));
#76112=CARTESIAN_POINT('Origin',(45.6047111404246,814.659546580852,121.66586273569));
#76113=CARTESIAN_POINT('Origin',(45.001057776689,814.343836394462,110.128185349306));
#76114=CARTESIAN_POINT('',(45.001057776689,811.975675077176,120.717291735229));
#76115=CARTESIAN_POINT('Origin',(45.001057776689,810.753905797794,120.285477132298));
#76116=CARTESIAN_POINT('',(45.001057776689,812.642141346244,118.831602812793));
#76117=CARTESIAN_POINT('',(45.001057776689,815.565605673845,110.559999952237));
#76118=CARTESIAN_POINT('Origin',(45.001057776689,811.420372066862,118.399788209863));
#76119=CARTESIAN_POINT('Origin',(45.001057776689,814.343836394462,110.128185349306));
#76120=CARTESIAN_POINT('',(45.001057776689,812.680419762956,116.335080592795));
#76121=CARTESIAN_POINT('Origin',(45.001057776689,812.208997532347,116.168464025528));
#76122=CARTESIAN_POINT('',(45.001057776689,811.225328028402,120.452093699565));
#76123=CARTESIAN_POINT('',(45.001057776689,814.815258625071,110.294801916574));
#76124=CARTESIAN_POINT('Origin',(45.001057776689,810.753905797794,120.285477132298));
#76125=CARTESIAN_POINT('Origin',(45.0452092570759,809.864990821428,108.545209778267));
#76126=CARTESIAN_POINT('',(45.0452092570759,807.78977662676,119.237853589437));
#76127=CARTESIAN_POINT('Origin',(45.0452092570759,806.275060224759,118.702501561259));
#76128=CARTESIAN_POINT('',(45.0452092570759,808.456242895828,117.352164667001));
#76129=CARTESIAN_POINT('',(45.0452092570759,811.379707223428,109.080561806445));
#76130=CARTESIAN_POINT('Origin',(45.0452092570759,806.941526493827,116.816812638824));
#76131=CARTESIAN_POINT('Origin',(45.0452092570759,809.864990821428,108.545209778267));
#76132=CARTESIAN_POINT('',(45.0452092570759,808.201574189921,114.752105021756));
#76133=CARTESIAN_POINT('Origin',(45.0452092570759,807.730151959312,114.585488454489));
#76134=CARTESIAN_POINT('',(45.0452092570759,806.746482455368,118.869118128526));
#76135=CARTESIAN_POINT('',(45.0452092570759,810.336413052037,108.711826345535));
#76136=CARTESIAN_POINT('Origin',(45.0452092570759,806.275060224759,118.702501561259));
#76137=CARTESIAN_POINT('Origin',(46.1251998582498,805.542619761922,107.017537594757));
#76138=CARTESIAN_POINT('',(46.1251998582498,803.6763013097,117.784012229471));
#76139=CARTESIAN_POINT('Origin',(46.1251998582498,801.952689165253,117.174829377748));
#76140=CARTESIAN_POINT('',(46.1251998582498,804.342767578769,115.898323307036));
#76141=CARTESIAN_POINT('',(46.1251998582498,807.266231906369,107.62672044648));
#76142=CARTESIAN_POINT('Origin',(46.1251998582498,802.619155434322,115.289140455313));
#76143=CARTESIAN_POINT('Origin',(46.1251998582498,805.542619761922,107.017537594757));
#76144=CARTESIAN_POINT('',(46.1251998582498,803.879203130416,113.224432838245));
#76145=CARTESIAN_POINT('Origin',(46.1251998582498,803.407780899807,113.057816270978));
#76146=CARTESIAN_POINT('',(46.1251998582498,802.424111395862,117.341445945016));
#76147=CARTESIAN_POINT('',(46.1251998582498,806.014041992531,107.184154162024));
#76148=CARTESIAN_POINT('Origin',(46.1251998582498,801.952689165253,117.174829377748));
#76149=CARTESIAN_POINT('Origin',(47.8987613742277,801.012599519368,105.416475163972));
#76150=CARTESIAN_POINT('',(47.8987613742277,799.174868320261,116.19305350121));
#76151=CARTESIAN_POINT('Origin',(47.8987613742277,797.422668922699,115.573766946963));
#76152=CARTESIAN_POINT('',(47.8987613742277,799.841334589329,114.307364578775));
#76153=CARTESIAN_POINT('',(47.8987613742277,802.764798916929,106.035761718219));
#76154=CARTESIAN_POINT('Origin',(47.8987613742277,798.089135191767,113.688078024528));
#76155=CARTESIAN_POINT('Origin',(47.8987613742277,801.012599519368,105.416475163972));
#76156=CARTESIAN_POINT('',(47.8987613742277,799.349182887861,111.62337040746));
#76157=CARTESIAN_POINT('Origin',(47.8987613742277,798.877760657253,111.456753840193));
#76158=CARTESIAN_POINT('',(47.8987613742277,797.894091153308,115.74038351423));
#76159=CARTESIAN_POINT('',(47.8987613742277,801.484021749976,105.583091731239));
#76160=CARTESIAN_POINT('Origin',(47.8987613742277,797.422668922699,115.573766946963));
#76161=CARTESIAN_POINT('Origin',(50.6542446180139,797.353109422993,104.12308754197));
#76162=CARTESIAN_POINT('',(50.6542446180139,795.472421174705,114.884483404539));
#76163=CARTESIAN_POINT('Origin',(50.6542446180139,793.763178826324,114.280379324961));
#76164=CARTESIAN_POINT('',(50.6542446180139,796.138887443773,112.998794482104));
#76165=CARTESIAN_POINT('',(50.6542446180139,799.062351771373,104.727191621548));
#76166=CARTESIAN_POINT('Origin',(50.6542446180139,794.429645095393,112.394690402526));
#76167=CARTESIAN_POINT('Origin',(50.6542446180139,797.353109422993,104.12308754197));
#76168=CARTESIAN_POINT('',(50.6542446180139,795.689692791486,110.329982785458));
#76169=CARTESIAN_POINT('Origin',(50.6542446180139,795.218270560878,110.163366218191));
#76170=CARTESIAN_POINT('',(50.6542446180139,794.234601056933,114.446995892228));
#76171=CARTESIAN_POINT('',(50.6542446180139,797.824531653602,104.289704109237));
#76172=CARTESIAN_POINT('Origin',(50.6542446180139,793.763178826324,114.280379324961));
#76173=CARTESIAN_POINT('Origin',(54.406656968682,793.073938964199,102.61068391248));
#76174=CARTESIAN_POINT('',(54.406656968682,791.286223517571,113.40493950897));
#76175=CARTESIAN_POINT('Origin',(54.406656968682,789.48400836753,112.767975695471));
#76176=CARTESIAN_POINT('',(54.406656968682,791.952689786913,111.519250585761));
#76177=CARTESIAN_POINT('',(54.406656968682,794.87615411424,103.247647725978));
#76178=CARTESIAN_POINT('',(53.0282509976584,788.901890948758,110.440995050868));
#76179=CARTESIAN_POINT('Origin',(54.4066569686837,790.150474636598,110.882286773036));
#76180=CARTESIAN_POINT('',(55.7276395803606,788.847878514773,110.421905229141));
#76181=CARTESIAN_POINT('Ctrl Pts',(55.7276395634569,788.847878682488,110.421905288417));
#76182=CARTESIAN_POINT('Ctrl Pts',(55.5456566202033,788.683820399216,110.363921539188));
#76183=CARTESIAN_POINT('Ctrl Pts',(55.3310737782485,788.555040568309,110.319135204066));
#76184=CARTESIAN_POINT('Ctrl Pts',(54.9643199501897,788.420973591252,110.272735437511));
#76185=CARTESIAN_POINT('Ctrl Pts',(54.8271319930196,788.386712853143,110.260948684297));
#76186=CARTESIAN_POINT('Ctrl Pts',(54.5812541501973,788.352204133832,110.249104533157));
#76187=CARTESIAN_POINT('Ctrl Pts',(54.4741664289805,788.34577865309,110.24691602536));
#76188=CARTESIAN_POINT('Ctrl Pts',(54.2597596859153,788.349965233717,110.248396777475));
#76189=CARTESIAN_POINT('Ctrl Pts',(54.1528214814057,788.360605741338,110.252075734691));
#76190=CARTESIAN_POINT('Ctrl Pts',(53.9076157883093,788.404957435148,110.267398592785));
#76191=CARTESIAN_POINT('Ctrl Pts',(53.7712598392015,788.4449186278,110.281197882194));
#76192=CARTESIAN_POINT('Ctrl Pts',(53.4105721629827,788.593926845041,110.33287678729));
#76193=CARTESIAN_POINT('Ctrl Pts',(53.2023852593083,788.730998225782,110.38059577992));
#76194=CARTESIAN_POINT('Ctrl Pts',(53.0282510499295,788.901890998491,110.440995068445));
#76195=CARTESIAN_POINT('Origin',(54.4066569686837,790.150474636598,110.882286773036));
#76196=CARTESIAN_POINT('Origin',(54.406656968682,793.073938964199,102.61068391248));
#76197=CARTESIAN_POINT('',(54.406656968682,791.410522332693,108.817579155968));
#76198=CARTESIAN_POINT('Origin',(54.406656968682,790.939100102084,108.650962588701));
#76199=CARTESIAN_POINT('',(54.406656968682,789.955430598139,112.934592262738));
#76200=CARTESIAN_POINT('',(54.406656968682,793.545361194808,102.777300479747));
#76201=CARTESIAN_POINT('Origin',(54.406656968682,789.48400836753,112.767975695471));
#76202=CARTESIAN_POINT('Origin',(43.3244554712047,819.916889345885,112.0978908313));
#76203=CARTESIAN_POINT('',(43.3244554712047,817.325321168344,122.608037673648));
#76204=CARTESIAN_POINT('Origin',(43.3244554712047,816.326958749216,122.255182614291));
#76205=CARTESIAN_POINT('',(43.3244554712047,817.991787437412,120.722348751213));
#76206=CARTESIAN_POINT('',(43.3244554712047,820.915251765012,112.450745890657));
#76207=CARTESIAN_POINT('Origin',(43.3244554712047,816.993425018285,120.369493691856));
#76208=CARTESIAN_POINT('Origin',(43.3244554712047,819.916889345885,112.0978908313));
#76209=CARTESIAN_POINT('',(43.3244554712047,818.253472714379,118.304786074788));
#76210=CARTESIAN_POINT('Origin',(43.3244554712047,817.78205048377,118.138169507521));
#76211=CARTESIAN_POINT('',(43.3244554712047,816.798380979825,122.421799181559));
#76212=CARTESIAN_POINT('',(43.3244554712047,820.388311576494,112.264507398567));
#76213=CARTESIAN_POINT('Origin',(43.3244554712047,816.326958749216,122.255182614291));
#76214=CARTESIAN_POINT('Origin',(41.8727395776554,816.214929379271,110.789492920152));
#76215=CARTESIAN_POINT('',(41.8727395776554,813.846768061985,121.378599306074));
#76216=CARTESIAN_POINT('Origin',(41.8727395776554,812.624998782603,120.946784703143));
#76217=CARTESIAN_POINT('',(41.8727395776554,814.513234331054,119.492910383639));
#76218=CARTESIAN_POINT('',(41.8727395776554,817.436698658654,111.221307523083));
#76219=CARTESIAN_POINT('Origin',(41.8727395776554,813.291465051671,119.061095780708));
#76220=CARTESIAN_POINT('Origin',(41.8727395776554,816.214929379271,110.789492920152));
#76221=CARTESIAN_POINT('',(41.8727395776554,814.551512747765,116.99638816364));
#76222=CARTESIAN_POINT('Origin',(41.8727395776554,814.080090517156,116.829771596373));
#76223=CARTESIAN_POINT('',(41.8727395776554,813.096421013212,121.11340127041));
#76224=CARTESIAN_POINT('',(41.8727395776554,816.68635160988,110.956109487419));
#76225=CARTESIAN_POINT('Origin',(41.8727395776554,812.624998782603,120.946784703143));
#76226=CARTESIAN_POINT('Origin',(40.9282719744559,811.825302384506,109.238050213459));
#76227=CARTESIAN_POINT('',(40.9282719744559,809.750088189838,119.930694024628));
#76228=CARTESIAN_POINT('Origin',(40.9282719744559,808.235371787837,119.395341996451));
#76229=CARTESIAN_POINT('',(40.9282719744559,810.416554458906,118.045005102193));
#76230=CARTESIAN_POINT('',(40.9282719744559,813.340018786506,109.773402241637));
#76231=CARTESIAN_POINT('Origin',(40.9282719744559,808.901838056905,117.509653074015));
#76232=CARTESIAN_POINT('Origin',(40.9282719744559,811.825302384506,109.238050213459));
#76233=CARTESIAN_POINT('',(40.9282719744559,810.161885753,115.444945456948));
#76234=CARTESIAN_POINT('Origin',(40.9282719744559,809.69046352239,115.27832888968));
#76235=CARTESIAN_POINT('',(40.9282719744559,808.706794018446,119.561958563718));
#76236=CARTESIAN_POINT('',(40.9282719744559,812.296724615114,109.404666780726));
#76237=CARTESIAN_POINT('Origin',(40.9282719744559,808.235371787837,119.395341996451));
#76238=CARTESIAN_POINT('Origin',(41.031512956517,807.385676688607,107.668936274038));
#76239=CARTESIAN_POINT('',(41.031512956517,805.519358236385,118.435410908752));
#76240=CARTESIAN_POINT('Origin',(41.031512956517,803.795746091938,117.826228057029));
#76241=CARTESIAN_POINT('',(41.031512956517,806.185824505454,116.549721986316));
#76242=CARTESIAN_POINT('',(41.031512956517,809.109288833054,108.27811912576));
#76243=CARTESIAN_POINT('Origin',(41.031512956517,804.462212361007,115.940539134594));
#76244=CARTESIAN_POINT('Origin',(41.031512956517,807.385676688607,107.668936274038));
#76245=CARTESIAN_POINT('',(41.031512956517,805.722260057101,113.875831517526));
#76246=CARTESIAN_POINT('Origin',(41.031512956517,805.250837826492,113.709214950259));
#76247=CARTESIAN_POINT('',(41.031512956517,804.267168322547,117.992844624296));
#76248=CARTESIAN_POINT('',(41.031512956517,807.857098919216,107.835552841305));
#76249=CARTESIAN_POINT('Origin',(41.031512956517,803.795746091938,117.826228057029));
#76250=CARTESIAN_POINT('Origin',(41.7673788293708,802.606979855433,105.979983121944));
#76251=CARTESIAN_POINT('',(41.7673788293708,800.769248656326,116.756561459183));
#76252=CARTESIAN_POINT('Origin',(41.7673788293708,799.017049258764,116.137274904936));
#76253=CARTESIAN_POINT('',(41.7673788293708,801.435714925394,114.870872536748));
#76254=CARTESIAN_POINT('',(41.7673788293708,804.359179252995,106.599269676191));
#76255=CARTESIAN_POINT('Origin',(41.7673788293708,799.683515527833,114.251585982501));
#76256=CARTESIAN_POINT('Origin',(41.7673788293708,802.606979855433,105.979983121944));
#76257=CARTESIAN_POINT('',(41.7673788293708,800.943563223927,112.186878365433));
#76258=CARTESIAN_POINT('Origin',(41.7673788293708,800.472140993318,112.020261798166));
#76259=CARTESIAN_POINT('',(41.7673788293708,799.488471489373,116.303891472203));
#76260=CARTESIAN_POINT('',(41.7673788293708,803.078402086042,106.146599689212));
#76261=CARTESIAN_POINT('Origin',(41.7673788293708,799.017049258764,116.137274904936));
#76262=CARTESIAN_POINT('Origin',(43.6556743576072,798.487305464523,104.523950799529));
#76263=CARTESIAN_POINT('',(43.6556743576072,796.606617216234,115.285346662099));
#76264=CARTESIAN_POINT('Origin',(43.6556743576072,794.897374867854,114.68124258252));
#76265=CARTESIAN_POINT('',(43.6556743576072,797.273083485303,113.399657739663));
#76266=CARTESIAN_POINT('',(43.6556743576072,800.196547812903,105.128054879107));
#76267=CARTESIAN_POINT('Origin',(43.6556743576072,795.563841136923,112.795553660085));
#76268=CARTESIAN_POINT('Origin',(43.6556743576072,798.487305464523,104.523950799529));
#76269=CARTESIAN_POINT('',(43.6556743576072,796.823888833016,110.730846043017));
#76270=CARTESIAN_POINT('Origin',(43.6556743576072,796.352466602408,110.56422947575));
#76271=CARTESIAN_POINT('',(43.6556743576072,795.368797098463,114.847859149787));
#76272=CARTESIAN_POINT('',(43.6556743576072,798.958727695131,104.690567366796));
#76273=CARTESIAN_POINT('Origin',(43.6556743576072,794.897374867854,114.68124258252));
#76274=CARTESIAN_POINT('Origin',(46.3824646583332,793.566065810002,102.784618191315));
#76275=CARTESIAN_POINT('',(46.3824646583332,791.778350363374,113.578873787805));
#76276=CARTESIAN_POINT('Origin',(46.3824646583332,789.976135213334,112.941909974306));
#76277=CARTESIAN_POINT('',(46.3824646583332,792.444816632443,111.693184865369));
#76278=CARTESIAN_POINT('',(46.3824646583332,795.368280960043,103.421582004813));
#76279=CARTESIAN_POINT('Origin',(46.3824646583332,790.642601482402,111.056221051871));
#76280=CARTESIAN_POINT('Origin',(46.3824646583332,793.566065810002,102.784618191315));
#76281=CARTESIAN_POINT('',(46.3824646583332,791.902649178496,108.991513434803));
#76282=CARTESIAN_POINT('Origin',(46.3824646583332,791.431226947887,108.824896867536));
#76283=CARTESIAN_POINT('',(46.3824646583332,790.447557443943,113.108526541573));
#76284=CARTESIAN_POINT('',(46.3824646583332,794.037488040611,102.951234758582));
#76285=CARTESIAN_POINT('Origin',(46.3824646583332,789.976135213334,112.941909974306));
#76286=CARTESIAN_POINT('Origin',(41.4617188627654,821.99485939656,112.832315757083));
#76287=CARTESIAN_POINT('',(41.4617188627654,819.403291219019,123.342462599431));
#76288=CARTESIAN_POINT('Origin',(41.4617188627654,818.404928799891,122.989607540074));
#76289=CARTESIAN_POINT('',(41.4617188627654,820.069757488087,121.456773676996));
#76290=CARTESIAN_POINT('',(41.4617188627654,822.993221815687,113.18517081644));
#76291=CARTESIAN_POINT('Origin',(41.4617188627654,819.07139506896,121.103918617639));
#76292=CARTESIAN_POINT('Origin',(41.4617188627654,821.99485939656,112.832315757083));
#76293=CARTESIAN_POINT('',(41.4617188627654,820.331442765054,119.039211000571));
#76294=CARTESIAN_POINT('Origin',(41.4617188627654,819.860020534445,118.872594433304));
#76295=CARTESIAN_POINT('',(41.4617188627654,818.8763510305,123.156224107341));
#76296=CARTESIAN_POINT('',(41.4617188627654,822.466281627169,112.99893232435));
#76297=CARTESIAN_POINT('Origin',(41.4617188627654,818.404928799891,122.989607540074));
#76298=CARTESIAN_POINT('Origin',(39.2253873900563,818.658373660907,111.653088805286));
#76299=CARTESIAN_POINT('',(39.2253873900563,816.290212343621,122.242195191208));
#76300=CARTESIAN_POINT('Origin',(39.2253873900563,815.068443064238,121.810380588277));
#76301=CARTESIAN_POINT('',(39.2253873900563,816.956678612689,120.356506268773));
#76302=CARTESIAN_POINT('',(39.2253873900563,819.880142940289,112.084903408217));
#76303=CARTESIAN_POINT('Origin',(39.2253873900563,815.734909333306,119.924691665842));
#76304=CARTESIAN_POINT('Origin',(39.2253873900563,818.658373660907,111.653088805286));
#76305=CARTESIAN_POINT('',(39.2253873900563,816.9949570294,117.859984048774));
#76306=CARTESIAN_POINT('Origin',(39.2253873900563,816.523534798792,117.693367481507));
#76307=CARTESIAN_POINT('',(39.2253873900563,815.539865294847,121.976997155544));
#76308=CARTESIAN_POINT('',(39.2253873900563,819.129795891515,111.819705372553));
#76309=CARTESIAN_POINT('Origin',(39.2253873900563,815.068443064238,121.810380588277));
#76310=CARTESIAN_POINT('Origin',(37.333578469589,814.549813007849,110.20098445387));
#76311=CARTESIAN_POINT('',(37.333578469589,812.474598813181,120.893628265039));
#76312=CARTESIAN_POINT('Origin',(37.333578469589,810.95988241118,120.358276236862));
#76313=CARTESIAN_POINT('',(37.333578469589,813.141065082249,119.007939342604));
#76314=CARTESIAN_POINT('',(37.333578469589,816.064529409849,110.736336482048));
#76315=CARTESIAN_POINT('Origin',(37.333578469589,811.626348680248,118.472587314426));
#76316=CARTESIAN_POINT('Origin',(37.333578469589,814.549813007849,110.20098445387));
#76317=CARTESIAN_POINT('',(37.333578469589,812.886396376342,116.407879697359));
#76318=CARTESIAN_POINT('Origin',(37.333578469589,812.414974145734,116.241263130091));
#76319=CARTESIAN_POINT('',(37.333578469589,811.431304641789,120.524892804129));
#76320=CARTESIAN_POINT('',(37.333578469589,815.021235238458,110.367601021137));
#76321=CARTESIAN_POINT('Origin',(37.333578469589,810.95988241118,120.358276236862));
#76322=CARTESIAN_POINT('Origin',(36.4555577062156,810.186965622156,108.659006567134));
#76323=CARTESIAN_POINT('',(36.4555577062156,808.320647169934,119.425481201848));
#76324=CARTESIAN_POINT('Origin',(36.4555577062156,806.597035025487,118.816298350126));
#76325=CARTESIAN_POINT('',(36.4555577062156,808.987113439002,117.539792279413));
#76326=CARTESIAN_POINT('',(36.4555577062156,811.910577766602,109.268189418857));
#76327=CARTESIAN_POINT('Origin',(36.4555577062156,807.263501294555,116.930609427691));
#76328=CARTESIAN_POINT('Origin',(36.4555577062156,810.186965622156,108.659006567134));
#76329=CARTESIAN_POINT('',(36.4555577062156,808.523548990649,114.865901810623));
#76330=CARTESIAN_POINT('Origin',(36.4555577062156,808.05212676004,114.699285243356));
#76331=CARTESIAN_POINT('',(36.4555577062156,807.068457256096,118.982914917393));
#76332=CARTESIAN_POINT('',(36.4555577062156,810.658387852764,108.825623134402));
#76333=CARTESIAN_POINT('Origin',(36.4555577062156,806.597035025487,118.816298350126));
#76334=CARTESIAN_POINT('Origin',(36.1215670662255,805.368444180703,106.955978050976));
#76335=CARTESIAN_POINT('',(36.1215670662255,803.530712981596,117.732556388215));
#76336=CARTESIAN_POINT('Origin',(36.1215670662255,801.778513584035,117.113269833968));
#76337=CARTESIAN_POINT('',(36.1215670662255,804.197179250664,115.846867465779));
#76338=CARTESIAN_POINT('',(36.1215670662255,807.120643578265,107.575264605223));
#76339=CARTESIAN_POINT('Origin',(36.1215670662255,802.444979853103,115.227580911532));
#76340=CARTESIAN_POINT('Origin',(36.1215670662255,805.368444180703,106.955978050976));
#76341=CARTESIAN_POINT('',(36.1215670662255,803.705027549197,113.162873294465));
#76342=CARTESIAN_POINT('Origin',(36.1215670662255,803.233605318588,112.996256727198));
#76343=CARTESIAN_POINT('',(36.1215670662255,802.249935814643,117.279886401235));
#76344=CARTESIAN_POINT('',(36.1215670662255,805.839866411312,107.122594618243));
#76345=CARTESIAN_POINT('Origin',(36.1215670662255,801.778513584035,117.113269833968));
#76346=CARTESIAN_POINT('Origin',(38.6421417333314,795.620407971914,103.510692221739));
#76347=CARTESIAN_POINT('',(38.6421417333314,793.832692525286,114.304947818229));
#76348=CARTESIAN_POINT('Origin',(38.6421417333314,792.030477375246,113.667984004731));
#76349=CARTESIAN_POINT('',(38.6421417333314,794.499158794355,112.419258895794));
#76350=CARTESIAN_POINT('',(38.6421417333314,797.422623121955,104.147656035238));
#76351=CARTESIAN_POINT('Origin',(38.6421417333314,792.696943644314,111.782295082296));
#76352=CARTESIAN_POINT('Origin',(38.6421417333314,795.620407971914,103.510692221739));
#76353=CARTESIAN_POINT('',(38.6421417333314,793.956991340408,109.717587465228));
#76354=CARTESIAN_POINT('Origin',(38.6421417333314,793.485569109799,109.550970897961));
#76355=CARTESIAN_POINT('',(38.6421417333314,792.501899605855,113.834600571998));
#76356=CARTESIAN_POINT('',(38.6421417333314,796.091830202523,103.677308789006));
#76357=CARTESIAN_POINT('Origin',(38.6421417333314,792.030477375246,113.667984004731));
#76358=CARTESIAN_POINT('Origin',(41.2192472761507,791.274059237588,101.974545516642));
#76359=CARTESIAN_POINT('',(41.2192472761507,789.145227456717,112.648239058651));
#76360=CARTESIAN_POINT('Origin',(41.2192472761507,787.684128640919,112.131837299634));
#76361=CARTESIAN_POINT('',(41.2192472761507,789.811693725789,110.762550136206));
#76362=CARTESIAN_POINT('',(41.2192472761507,792.735158053385,102.49094727566));
#76363=CARTESIAN_POINT('',(39.7442317533746,787.902560458671,110.087797842478));
#76364=CARTESIAN_POINT('Origin',(41.2192472761522,788.350594909987,110.246148377198));
#76365=CARTESIAN_POINT('',(42.7661923053508,788.263967910344,110.215531464427));
#76366=CARTESIAN_POINT('Ctrl Pts',(42.7661922957563,788.263967909607,110.215531464166));
#76367=CARTESIAN_POINT('Ctrl Pts',(42.7576496927167,788.128357840798,110.167602277356));
#76368=CARTESIAN_POINT('Ctrl Pts',(42.729089354505,787.994387123929,110.120716649006));
#76369=CARTESIAN_POINT('Ctrl Pts',(42.627691869533,787.721691289648,110.026032551387));
#76370=CARTESIAN_POINT('Ctrl Pts',(42.5504466448361,787.586099090374,109.97941496988));
#76371=CARTESIAN_POINT('Ctrl Pts',(42.3277194563926,787.30916137911,109.884730050415));
#76372=CARTESIAN_POINT('Ctrl Pts',(42.1716038272599,787.179045937569,109.840642865158));
#76373=CARTESIAN_POINT('Ctrl Pts',(41.889457604766,787.025002344919,109.78838353968));
#76374=CARTESIAN_POINT('Ctrl Pts',(41.7791159733533,786.979941045624,109.773079760154));
#76375=CARTESIAN_POINT('Ctrl Pts',(41.5826242356446,786.924183406791,109.754005617275));
#76376=CARTESIAN_POINT('Ctrl Pts',(41.4989623551683,786.90742981042,109.748218661099));
#76377=CARTESIAN_POINT('Ctrl Pts',(41.3756211561855,786.892678768829,109.743001632323));
#76378=CARTESIAN_POINT('Ctrl Pts',(41.3368035967877,786.889441333856,109.741828028186));
#76379=CARTESIAN_POINT('Ctrl Pts',(41.2095058860293,786.88340089315,109.739505704016));
#76380=CARTESIAN_POINT('Ctrl Pts',(41.1208920861614,786.886399441584,109.740290711422));
#76381=CARTESIAN_POINT('Ctrl Pts',(40.9019145860912,786.911704903613,109.74823340755));
#76382=CARTESIAN_POINT('Ctrl Pts',(40.7733674323024,786.94268665391,109.758303443042));
#76383=CARTESIAN_POINT('Ctrl Pts',(40.458350410294,787.060702263822,109.797357332023));
#76384=CARTESIAN_POINT('Ctrl Pts',(40.2832716228728,787.168316322986,109.833418795446));
#76385=CARTESIAN_POINT('Ctrl Pts',(40.0416454203311,787.392022078613,109.909768279067));
#76386=CARTESIAN_POINT('Ctrl Pts',(39.9597641668178,787.489881377695,109.943441271257));
#76387=CARTESIAN_POINT('Ctrl Pts',(39.830368156229,787.69271580738,110.013947340926));
#76388=CARTESIAN_POINT('Ctrl Pts',(39.7808072878434,787.795518055038,110.049965435164));
#76389=CARTESIAN_POINT('Ctrl Pts',(39.7442317638745,787.902560455324,110.087797841296));
#76390=CARTESIAN_POINT('Origin',(41.2192472761522,788.350594909987,110.246148377198));
#76391=CARTESIAN_POINT('Origin',(41.2192472761507,791.274059237588,101.974545516642));
#76392=CARTESIAN_POINT('',(41.2192472761507,789.610642606081,108.181440760131));
#76393=CARTESIAN_POINT('Origin',(41.2192472761507,789.139220375473,108.014824192864));
#76394=CARTESIAN_POINT('',(41.2192472761507,788.155550871528,112.298453866901));
#76395=CARTESIAN_POINT('',(41.2192472761507,791.745481468196,102.141162083909));
#76396=CARTESIAN_POINT('Origin',(41.2192472761507,787.684128640919,112.131837299634));
#76397=CARTESIAN_POINT('Origin',(40.0979118432977,824.392570067125,113.679747836629));
#76398=CARTESIAN_POINT('',(40.0979118432977,821.801001889583,124.189894678977));
#76399=CARTESIAN_POINT('Origin',(40.0979118432977,820.802639470456,123.837039619621));
#76400=CARTESIAN_POINT('',(40.0979118432977,822.467468158652,122.304205756542));
#76401=CARTESIAN_POINT('',(40.0979118432977,825.390932486252,114.032602895986));
#76402=CARTESIAN_POINT('Origin',(40.0979118432977,821.469105739524,121.951350697185));
#76403=CARTESIAN_POINT('Origin',(40.0979118432977,824.392570067125,113.679747836629));
#76404=CARTESIAN_POINT('',(40.0979118432977,822.729153435618,119.886643080118));
#76405=CARTESIAN_POINT('Origin',(40.0979118432977,822.257731205009,119.720026512851));
#76406=CARTESIAN_POINT('',(40.0979118432977,821.274061701065,124.003656186888));
#76407=CARTESIAN_POINT('',(40.0979118432977,824.863992297733,113.846364403896));
#76408=CARTESIAN_POINT('Origin',(40.0979118432977,820.802639470456,123.837039619621));
#76409=CARTESIAN_POINT('Origin',(37.1747032078952,821.567378999314,112.681229720536));
#76410=CARTESIAN_POINT('',(37.1747032078952,819.199217682029,123.270336106458));
#76411=CARTESIAN_POINT('Origin',(37.1747032078952,817.977448402646,122.838521503527));
#76412=CARTESIAN_POINT('',(37.1747032078952,819.865683951097,121.384647184023));
#76413=CARTESIAN_POINT('',(37.1747032078952,822.789148278697,113.113044323467));
#76414=CARTESIAN_POINT('Origin',(37.1747032078952,818.643914671714,120.952832581092));
#76415=CARTESIAN_POINT('Origin',(37.1747032078952,821.567378999314,112.681229720536));
#76416=CARTESIAN_POINT('',(37.1747032078952,819.903962367808,118.888124964024));
#76417=CARTESIAN_POINT('Origin',(37.1747032078952,819.432540137199,118.721508396757));
#76418=CARTESIAN_POINT('',(37.1747032078952,818.448870633255,123.005138070794));
#76419=CARTESIAN_POINT('',(37.1747032078952,822.038801229923,112.847846287803));
#76420=CARTESIAN_POINT('Origin',(37.1747032078952,817.977448402646,122.838521503527));
#76421=CARTESIAN_POINT('Origin',(34.4182340978906,817.919448503564,111.391927652523));
#76422=CARTESIAN_POINT('',(34.4182340978906,815.844234308896,122.084571463692));
#76423=CARTESIAN_POINT('Origin',(34.4182340978906,814.329517906896,121.549219435515));
#76424=CARTESIAN_POINT('',(34.4182340978906,816.510700577964,120.198882541257));
#76425=CARTESIAN_POINT('',(34.4182340978906,819.434164905565,111.927279680701));
#76426=CARTESIAN_POINT('Origin',(34.4182340978906,814.995984175964,119.66353051308));
#76427=CARTESIAN_POINT('Origin',(34.4182340978906,817.919448503564,111.391927652523));
#76428=CARTESIAN_POINT('',(34.4182340978906,816.256031872058,117.598822896012));
#76429=CARTESIAN_POINT('Origin',(34.4182340978906,815.784609641449,117.432206328745));
#76430=CARTESIAN_POINT('',(34.4182340978906,814.800940137504,121.715836002782));
#76431=CARTESIAN_POINT('',(34.4182340978906,818.390870734173,111.558544219791));
#76432=CARTESIAN_POINT('Origin',(34.4182340978906,814.329517906896,121.549219435515));
#76433=CARTESIAN_POINT('Origin',(32.5973253096532,813.824056794096,109.944477651355));
#76434=CARTESIAN_POINT('',(32.5973253096532,811.957738341874,120.710952286068));
#76435=CARTESIAN_POINT('Origin',(32.5973253096532,810.234126197427,120.101769434346));
#76436=CARTESIAN_POINT('',(32.5973253096532,812.624204610942,118.825263363633));
#76437=CARTESIAN_POINT('',(32.5973253096532,815.547668938542,110.553660503077));
#76438=CARTESIAN_POINT('Origin',(32.5973253096532,810.900592466495,118.216080511911));
#76439=CARTESIAN_POINT('Origin',(32.5973253096532,813.824056794096,109.944477651355));
#76440=CARTESIAN_POINT('',(32.5973253096532,812.160640162589,116.151372894843));
#76441=CARTESIAN_POINT('Origin',(32.5973253096532,811.68921793198,115.984756327576));
#76442=CARTESIAN_POINT('',(32.5973253096532,810.705548428036,120.268386001613));
#76443=CARTESIAN_POINT('',(32.5973253096532,814.295479024704,110.111094218622));
#76444=CARTESIAN_POINT('Origin',(32.5973253096532,810.234126197427,120.101769434346));
#76445=CARTESIAN_POINT('Origin',(31.2080751504518,809.176303253188,108.301804289325));
#76446=CARTESIAN_POINT('',(31.2080751504518,807.338572054081,119.078382626563));
#76447=CARTESIAN_POINT('Origin',(31.2080751504518,805.586372656519,118.459096072316));
#76448=CARTESIAN_POINT('',(31.2080751504518,808.005038323149,117.192693704128));
#76449=CARTESIAN_POINT('',(31.2080751504518,810.928502650749,108.921090843572));
#76450=CARTESIAN_POINT('Origin',(31.2080751504518,806.252838925588,116.573407149881));
#76451=CARTESIAN_POINT('Origin',(31.2080751504518,809.176303253188,108.301804289325));
#76452=CARTESIAN_POINT('',(31.2080751504518,807.512886621681,114.508699532813));
#76453=CARTESIAN_POINT('Origin',(31.2080751504518,807.041464391073,114.342082965546));
#76454=CARTESIAN_POINT('',(31.2080751504518,806.057794887128,118.625712639584));
#76455=CARTESIAN_POINT('',(31.2080751504518,809.647725483797,108.468420856592));
#76456=CARTESIAN_POINT('Origin',(31.2080751504518,805.586372656519,118.459096072316));
#76457=CARTESIAN_POINT('Origin',(31.1559196361592,804.688652124068,106.715716536822));
#76458=CARTESIAN_POINT('',(31.1559196361592,802.80796387578,117.477112399392));
#76459=CARTESIAN_POINT('Origin',(31.1559196361592,801.0987215274,116.873008319814));
#76460=CARTESIAN_POINT('',(31.1559196361592,803.474430144848,115.591423476957));
#76461=CARTESIAN_POINT('',(31.1559196361592,806.397894472449,107.319820616401));
#76462=CARTESIAN_POINT('Origin',(31.1559196361592,801.765187796468,114.987319397378));
#76463=CARTESIAN_POINT('Origin',(31.1559196361592,804.688652124068,106.715716536822));
#76464=CARTESIAN_POINT('',(31.1559196361592,803.025235492562,112.922611780311));
#76465=CARTESIAN_POINT('Origin',(31.1559196361592,802.553813261953,112.755995213043));
#76466=CARTESIAN_POINT('',(31.1559196361592,801.570143758008,117.039624887081));
#76467=CARTESIAN_POINT('',(31.1559196361592,805.160074354677,106.882333104089));
#76468=CARTESIAN_POINT('Origin',(31.1559196361592,801.0987215274,116.873008319814));
#76469=CARTESIAN_POINT('Origin',(31.5239774476895,799.147180839632,104.757173084534));
#76470=CARTESIAN_POINT('',(31.5239774476895,797.359465393004,115.551428681024));
#76471=CARTESIAN_POINT('Origin',(31.5239774476895,795.557250242964,114.914464867526));
#76472=CARTESIAN_POINT('',(31.5239774476895,798.025931662073,113.665739758589));
#76473=CARTESIAN_POINT('',(31.5239774476895,800.949395989673,105.394136898033));
#76474=CARTESIAN_POINT('Origin',(31.5239774476895,796.223716512032,113.02877594509));
#76475=CARTESIAN_POINT('Origin',(31.5239774476895,799.147180839632,104.757173084534));
#76476=CARTESIAN_POINT('',(31.5239774476895,797.483764208126,110.964068328022));
#76477=CARTESIAN_POINT('Origin',(31.5239774476895,797.012341977518,110.797451760755));
#76478=CARTESIAN_POINT('',(31.5239774476895,796.028672473573,115.081081434793));
#76479=CARTESIAN_POINT('',(31.5239774476895,799.618603070241,104.923789651801));
#76480=CARTESIAN_POINT('Origin',(31.5239774476895,795.557250242964,114.914464867526));
#76481=CARTESIAN_POINT('Origin',(33.0863303722204,794.390624412805,103.076045101183));
#76482=CARTESIAN_POINT('',(33.0863303722204,792.261792631934,113.749738643192));
#76483=CARTESIAN_POINT('Origin',(33.0863303722204,790.800693816136,113.233336884174));
#76484=CARTESIAN_POINT('',(33.0863303722204,792.928258901002,111.864049720756));
#76485=CARTESIAN_POINT('',(33.0863303722204,795.851723228602,103.5924468602));
#76486=CARTESIAN_POINT('Origin',(33.0863303722204,791.467160085205,111.347647961739));
#76487=CARTESIAN_POINT('Origin',(33.0863303722204,794.390624412805,103.076045101183));
#76488=CARTESIAN_POINT('',(33.0863303722204,792.727207781298,109.282940344671));
#76489=CARTESIAN_POINT('Origin',(33.0863303722204,792.25578555069,109.116323777404));
#76490=CARTESIAN_POINT('',(33.0863303722204,791.272116046745,113.399953451442));
#76491=CARTESIAN_POINT('',(33.0863303722204,794.862046643414,103.24266166845));
#76492=CARTESIAN_POINT('Origin',(33.0863303722204,790.800693816136,113.233336884174));
#76493=CARTESIAN_POINT('Origin',(39.2926393238238,827.005229895783,114.603150221633));
#76494=CARTESIAN_POINT('',(39.2926393238238,824.413661718241,125.11329706398));
#76495=CARTESIAN_POINT('Origin',(39.2926393238238,823.415299299114,124.760442004624));
#76496=CARTESIAN_POINT('',(39.2926393238238,825.08012798731,123.227608141545));
#76497=CARTESIAN_POINT('',(39.2926393238238,828.00359231491,114.956005280989));
#76498=CARTESIAN_POINT('Origin',(39.2926393238238,824.081765568183,122.874753082189));
#76499=CARTESIAN_POINT('Origin',(39.2926393238238,827.005229895783,114.603150221633));
#76500=CARTESIAN_POINT('',(39.2926393238238,825.341813264276,120.810045465121));
#76501=CARTESIAN_POINT('Origin',(39.2926393238238,824.870391033668,120.643428897854));
#76502=CARTESIAN_POINT('',(39.2926393238238,823.886721529723,124.927058571891));
#76503=CARTESIAN_POINT('',(39.2926393238238,827.476652126392,114.7697667889));
#76504=CARTESIAN_POINT('Origin',(39.2926393238238,823.415299299114,124.760442004624));
#76505=CARTESIAN_POINT('Origin',(35.8103117702064,824.81480790225,113.828980974337));
#76506=CARTESIAN_POINT('',(35.8103117702064,822.446646584964,124.418087360259));
#76507=CARTESIAN_POINT('Origin',(35.8103117702064,821.224877305582,123.986272757328));
#76508=CARTESIAN_POINT('',(35.8103117702064,823.113112854032,122.532398437824));
#76509=CARTESIAN_POINT('',(35.8103117702064,826.036577181633,114.260795577268));
#76510=CARTESIAN_POINT('Origin',(35.8103117702064,821.89134357465,122.100583834893));
#76511=CARTESIAN_POINT('Origin',(35.8103117702064,824.81480790225,113.828980974337));
#76512=CARTESIAN_POINT('',(35.8103117702064,823.151391270744,120.035876217825));
#76513=CARTESIAN_POINT('Origin',(35.8103117702064,822.679969040135,119.869259650558));
#76514=CARTESIAN_POINT('',(35.8103117702064,821.69629953619,124.152889324596));
#76515=CARTESIAN_POINT('',(35.8103117702064,825.286230132859,113.995597541604));
#76516=CARTESIAN_POINT('Origin',(35.8103117702064,821.224877305582,123.986272757328));
#76517=CARTESIAN_POINT('Origin',(32.3096533977779,821.786939631185,112.758829876858));
#76518=CARTESIAN_POINT('',(32.3096533977779,819.711725436516,123.451473688027));
#76519=CARTESIAN_POINT('Origin',(32.3096533977779,818.197009034516,122.91612165985));
#76520=CARTESIAN_POINT('',(32.3096533977779,820.378191705585,121.565784765592));
#76521=CARTESIAN_POINT('',(32.3096533977779,823.301656033185,113.294181905036));
#76522=CARTESIAN_POINT('Origin',(32.3096533977779,818.863475303584,121.030432737414));
#76523=CARTESIAN_POINT('Origin',(32.3096533977779,821.786939631185,112.758829876858));
#76524=CARTESIAN_POINT('',(32.3096533977779,820.123522999678,118.965725120347));
#76525=CARTESIAN_POINT('Origin',(32.3096533977779,819.652100769069,118.79910855308));
#76526=CARTESIAN_POINT('',(32.3096533977779,818.668431265125,123.082738227117));
#76527=CARTESIAN_POINT('',(32.3096533977779,822.258361861793,112.925446444125));
#76528=CARTESIAN_POINT('Origin',(32.3096533977779,818.197009034516,122.91612165985));
#76529=CARTESIAN_POINT('Origin',(29.6254390364126,818.137991867514,111.469168271943));
#76530=CARTESIAN_POINT('',(29.6254390364126,816.271673415292,122.235642906657));
#76531=CARTESIAN_POINT('Origin',(29.6254390364126,814.548061270846,121.626460054934));
#76532=CARTESIAN_POINT('',(29.6254390364126,816.93813968436,120.349953984221));
#76533=CARTESIAN_POINT('',(29.6254390364126,819.861604011961,112.078351123665));
#76534=CARTESIAN_POINT('Origin',(29.6254390364126,815.214527539914,119.740771132499));
#76535=CARTESIAN_POINT('Origin',(29.6254390364126,818.137991867514,111.469168271943));
#76536=CARTESIAN_POINT('',(29.6254390364126,816.474575236008,117.676063515431));
#76537=CARTESIAN_POINT('Origin',(29.6254390364126,816.003153005399,117.509446948164));
#76538=CARTESIAN_POINT('',(29.6254390364126,815.019483501454,121.793076622201));
#76539=CARTESIAN_POINT('',(29.6254390364126,818.609414098123,111.63578483921));
#76540=CARTESIAN_POINT('Origin',(29.6254390364126,814.548061270846,121.626460054934));
#76541=CARTESIAN_POINT('Origin',(27.2416462563186,813.864135359284,109.958642772384));
#76542=CARTESIAN_POINT('',(27.2416462563186,812.026404160177,120.735221109623));
#76543=CARTESIAN_POINT('Origin',(27.2416462563186,810.274204762616,120.115934555376));
#76544=CARTESIAN_POINT('',(27.2416462563186,812.692870429245,118.849532187187));
#76545=CARTESIAN_POINT('',(27.2416462563186,815.616334756846,110.577929326631));
#76546=CARTESIAN_POINT('Origin',(27.2416462563186,810.940671031684,118.23024563294));
#76547=CARTESIAN_POINT('Origin',(27.2416462563186,813.864135359284,109.958642772384));
#76548=CARTESIAN_POINT('',(27.2416462563186,812.200718727778,116.165538015873));
#76549=CARTESIAN_POINT('Origin',(27.2416462563186,811.729296497169,115.998921448606));
#76550=CARTESIAN_POINT('',(27.2416462563186,810.745626993224,120.282551122643));
#76551=CARTESIAN_POINT('',(27.2416462563186,814.335557589893,110.125259339651));
#76552=CARTESIAN_POINT('Origin',(27.2416462563186,810.274204762616,120.115934555376));
#76553=CARTESIAN_POINT('Origin',(26.2010344369226,809.484774135699,108.410828336578));
#76554=CARTESIAN_POINT('',(26.2010344369226,807.604085887411,119.172224199147));
#76555=CARTESIAN_POINT('Origin',(26.2010344369226,805.89484353903,118.568120119569));
#76556=CARTESIAN_POINT('',(26.2010344369226,808.270552156479,117.286535276712));
#76557=CARTESIAN_POINT('',(26.2010344369226,811.194016484079,109.014932416156));
#76558=CARTESIAN_POINT('Origin',(26.2010344369226,806.561309808099,116.682431197134));
#76559=CARTESIAN_POINT('Origin',(26.2010344369226,809.484774135699,108.410828336578));
#76560=CARTESIAN_POINT('',(26.2010344369226,807.821357504193,114.617723580066));
#76561=CARTESIAN_POINT('Origin',(26.2010344369226,807.349935273584,114.451107012799));
#76562=CARTESIAN_POINT('',(26.2010344369226,806.366265769639,118.734736686836));
#76563=CARTESIAN_POINT('',(26.2010344369226,809.956196366308,108.577444903845));
#76564=CARTESIAN_POINT('Origin',(26.2010344369226,805.89484353903,118.568120119569));
#76565=CARTESIAN_POINT('Origin',(25.3390697374316,803.992247515504,106.469583584716));
#76566=CARTESIAN_POINT('',(25.3390697374316,802.204532068876,117.263839181206));
#76567=CARTESIAN_POINT('Origin',(25.3390697374316,800.402316918835,116.626875367708));
#76568=CARTESIAN_POINT('',(25.3390697374316,802.870998337944,115.378150258771));
#76569=CARTESIAN_POINT('',(25.3390697374316,805.794462665544,107.106547398215));
#76570=CARTESIAN_POINT('Origin',(25.3390697374316,801.068783187903,114.741186445273));
#76571=CARTESIAN_POINT('Origin',(25.3390697374316,803.992247515504,106.469583584716));
#76572=CARTESIAN_POINT('',(25.3390697374316,802.328830883997,112.676478828205));
#76573=CARTESIAN_POINT('Origin',(25.3390697374316,801.857408653389,112.509862260938));
#76574=CARTESIAN_POINT('',(25.3390697374316,800.873739149444,116.793491934975));
#76575=CARTESIAN_POINT('',(25.3390697374316,804.463669746112,106.636200151984));
#76576=CARTESIAN_POINT('Origin',(25.3390697374316,800.402316918835,116.626875367708));
#76577=CARTESIAN_POINT('Origin',(25.818387723871,799.033367736517,104.716947682931));
#76578=CARTESIAN_POINT('',(25.818387723871,796.904535955646,115.390641224939));
#76579=CARTESIAN_POINT('Origin',(25.818387723871,795.443437139849,114.874239465922));
#76580=CARTESIAN_POINT('',(25.818387723871,797.571002224714,113.504952302504));
#76581=CARTESIAN_POINT('',(25.818387723871,800.494466552315,105.233349441948));
#76582=CARTESIAN_POINT('Origin',(25.818387723871,796.109903408917,112.988550543487));
#76583=CARTESIAN_POINT('Origin',(25.818387723871,799.033367736517,104.716947682931));
#76584=CARTESIAN_POINT('',(25.818387723871,797.369951105011,110.923842926419));
#76585=CARTESIAN_POINT('Origin',(25.818387723871,796.898528874402,110.757226359152));
#76586=CARTESIAN_POINT('',(25.818387723871,795.914859370457,115.040856033189));
#76587=CARTESIAN_POINT('',(25.818387723871,799.504789967126,104.883564250198));
#76588=CARTESIAN_POINT('Origin',(25.818387723871,795.443437139849,114.874239465922));
#76589=CARTESIAN_POINT('Origin',(27.1695766575127,793.380711610087,102.719107745449));
#76590=CARTESIAN_POINT('',(27.1695766575127,790.97816259038,113.296060353798));
#76591=CARTESIAN_POINT('Origin',(27.1695766575127,789.790781013418,112.87639952844));
#76592=CARTESIAN_POINT('',(27.1695766575127,791.644628859449,111.410371431363));
#76593=CARTESIAN_POINT('',(27.1695766575127,794.568093187049,103.138768570807));
#76594=CARTESIAN_POINT('',(26.8302275943695,791.600709061904,111.394848688847));
#76595=CARTESIAN_POINT('Origin',(27.1695766575141,790.457247282485,110.990710606004));
#76596=CARTESIAN_POINT('',(25.9127399611503,790.376124123725,110.981073928445));
#76597=CARTESIAN_POINT('Ctrl Pts',(25.9127399611504,790.376124123725,110.981073928445));
#76598=CARTESIAN_POINT('Ctrl Pts',(25.9055874800323,790.483136414161,111.016781431184));
#76599=CARTESIAN_POINT('Ctrl Pts',(25.9136369112483,790.590820092905,111.052683799123));
#76600=CARTESIAN_POINT('Ctrl Pts',(25.9690778860656,790.842405034397,111.136728108892));
#76601=CARTESIAN_POINT('Ctrl Pts',(26.0299102940817,790.981536107245,111.183353587182));
#76602=CARTESIAN_POINT('Ctrl Pts',(26.1995966396547,791.226937399855,111.266151235457));
#76603=CARTESIAN_POINT('Ctrl Pts',(26.3053678987038,791.332133910036,111.301940653525));
#76604=CARTESIAN_POINT('Ctrl Pts',(26.5497091625053,791.500376393043,111.359703614437));
#76605=CARTESIAN_POINT('Ctrl Pts',(26.6858070399473,791.562608259858,111.381382576231));
#76606=CARTESIAN_POINT('Ctrl Pts',(26.8302275943693,791.600709061904,111.394848688848));
#76607=CARTESIAN_POINT('',(28.4218514091029,790.583031932634,111.035167157397));
#76608=CARTESIAN_POINT('Ctrl Pts',(28.4218514095886,790.583031931885,111.035167157132));
#76609=CARTESIAN_POINT('Ctrl Pts',(28.4337689638032,790.477559435438,110.997889608137));
#76610=CARTESIAN_POINT('Ctrl Pts',(28.430643339413,790.371000767451,110.960403070916));
#76611=CARTESIAN_POINT('Ctrl Pts',(28.3962813721003,790.171821902233,110.890856204986));
#76612=CARTESIAN_POINT('Ctrl Pts',(28.3680120124044,790.079599353015,110.858882283526));
#76613=CARTESIAN_POINT('Ctrl Pts',(28.2650618942256,789.850809070196,110.780282222341));
#76614=CARTESIAN_POINT('Ctrl Pts',(28.1737123951907,789.722733212863,110.737038440023));
#76615=CARTESIAN_POINT('Ctrl Pts',(27.9518861123843,789.512401256264,110.667606548889));
#76616=CARTESIAN_POINT('Ctrl Pts',(27.8259459980945,789.429555555268,110.641103162105));
#76617=CARTESIAN_POINT('Ctrl Pts',(27.5578613172935,789.313752584681,110.605707845539));
#76618=CARTESIAN_POINT('Ctrl Pts',(27.4191425282237,789.278839242261,110.596067471477));
#76619=CARTESIAN_POINT('Ctrl Pts',(27.1259918700454,789.253550609447,110.59206710079));
#76620=CARTESIAN_POINT('Ctrl Pts',(26.9735308851987,789.266538812695,110.598802966545));
#76621=CARTESIAN_POINT('Ctrl Pts',(26.75335717898,789.324487291314,110.62142302944));
#76622=CARTESIAN_POINT('Ctrl Pts',(26.6814475117158,789.350361655281,110.631098020792));
#76623=CARTESIAN_POINT('Ctrl Pts',(26.563258185529,789.405151119292,110.651011114534));
#76624=CARTESIAN_POINT('Ctrl Pts',(26.5156521743354,789.431027062694,110.660277588935));
#76625=CARTESIAN_POINT('Ctrl Pts',(26.44898174078,789.473016771392,110.675134208564));
#76626=CARTESIAN_POINT('Ctrl Pts',(26.4283985204782,789.486849842576,110.68000507493));
#76627=CARTESIAN_POINT('Ctrl Pts',(26.3605541410553,789.535436747924,110.697037838876));
#76628=CARTESIAN_POINT('Ctrl Pts',(26.3154825093639,789.57281589133,110.710020416739));
#76629=CARTESIAN_POINT('Ctrl Pts',(26.2055383718527,789.67809999404,110.746308960983));
#76630=CARTESIAN_POINT('Ctrl Pts',(26.1458120891379,789.750329498672,110.77094586298));
#76631=CARTESIAN_POINT('Ctrl Pts',(26.0364130077358,789.919666471888,110.828284944853));
#76632=CARTESIAN_POINT('Ctrl Pts',(25.9906709130046,790.018147111709,110.861386421255));
#76633=CARTESIAN_POINT('Ctrl Pts',(25.9341567116865,790.204254288454,110.92370472727));
#76634=CARTESIAN_POINT('Ctrl Pts',(25.9185125677585,790.289756911455,110.952255206282));
#76635=CARTESIAN_POINT('Ctrl Pts',(25.9127399611503,790.376124123725,110.981073928445));
#76636=CARTESIAN_POINT('Origin',(27.1695766575141,790.457247282485,110.990710606004));
#76637=CARTESIAN_POINT('Origin',(27.1695766575127,793.380711610087,102.719107745449));
#76638=CARTESIAN_POINT('',(27.1695766575127,791.717294978581,108.926002988937));
#76639=CARTESIAN_POINT('Origin',(27.1695766575127,791.245872747972,108.75938642167));
#76640=CARTESIAN_POINT('',(27.1695766575127,790.262203244027,113.043016095707));
#76641=CARTESIAN_POINT('',(27.1695766575127,793.852133840696,102.885724312716));
#76642=CARTESIAN_POINT('Origin',(27.1695766575127,789.790781013418,112.87639952844));
#76643=CARTESIAN_POINT('Origin',(39.0810955775722,829.718653111089,115.562165796892));
#76644=CARTESIAN_POINT('',(39.0810955775722,827.127084933548,126.072312639239));
#76645=CARTESIAN_POINT('Origin',(39.0810955775722,826.128722514421,125.719457579883));
#76646=CARTESIAN_POINT('',(39.0810955775722,827.793551202616,124.186623716804));
#76647=CARTESIAN_POINT('',(39.0810955775722,830.717015530217,115.915020856248));
#76648=CARTESIAN_POINT('Origin',(39.0810955775722,826.795188783489,123.833768657448));
#76649=CARTESIAN_POINT('Origin',(39.0810955775722,829.718653111089,115.562165796892));
#76650=CARTESIAN_POINT('',(39.0810955775722,828.055236479583,121.76906104038));
#76651=CARTESIAN_POINT('Origin',(39.0810955775722,827.583814248974,121.602444473113));
#76652=CARTESIAN_POINT('',(39.0810955775722,826.60014474503,125.88607414715));
#76653=CARTESIAN_POINT('',(39.0810955775722,830.190075341698,115.728782364159));
#76654=CARTESIAN_POINT('Origin',(39.0810955775722,826.128722514421,125.719457579883));
#76655=CARTESIAN_POINT('Origin',(35.1918435298943,828.258732143763,115.046180329378));
#76656=CARTESIAN_POINT('',(35.1918435298943,825.890570826477,125.6352867153));
#76657=CARTESIAN_POINT('Origin',(35.1918435298943,824.668801547094,125.203472112369));
#76658=CARTESIAN_POINT('',(35.1918435298943,826.557037095545,123.749597792865));
#76659=CARTESIAN_POINT('',(35.1918435298943,829.480501423146,115.477994932309));
#76660=CARTESIAN_POINT('Origin',(35.1918435298943,825.335267816163,123.317783189934));
#76661=CARTESIAN_POINT('Origin',(35.1918435298943,828.258732143763,115.046180329378));
#76662=CARTESIAN_POINT('',(35.1918435298943,826.595315512257,121.253075572866));
#76663=CARTESIAN_POINT('Origin',(35.1918435298943,826.123893281648,121.086459005599));
#76664=CARTESIAN_POINT('',(35.1918435298943,825.140223777703,125.370088679636));
#76665=CARTESIAN_POINT('',(35.1918435298943,828.730154374372,115.212796896645));
#76666=CARTESIAN_POINT('Origin',(35.1918435298943,824.668801547094,125.203472112369));
#76667=CARTESIAN_POINT('Origin',(31.0999914639398,825.983258470151,114.241950940547));
#76668=CARTESIAN_POINT('',(31.0999914639398,823.908044275483,124.934594751716));
#76669=CARTESIAN_POINT('Origin',(31.0999914639398,822.393327873482,124.399242723538));
#76670=CARTESIAN_POINT('',(31.0999914639398,824.574510544551,123.048905829281));
#76671=CARTESIAN_POINT('',(31.0999914639398,827.497974872151,114.777302968724));
#76672=CARTESIAN_POINT('Origin',(31.0999914639398,823.05979414255,122.513553801103));
#76673=CARTESIAN_POINT('Origin',(31.0999914639398,825.983258470151,114.241950940547));
#76674=CARTESIAN_POINT('',(31.0999914639398,824.319841838645,120.448846184035));
#76675=CARTESIAN_POINT('Origin',(31.0999914639398,823.848419608036,120.282229616768));
#76676=CARTESIAN_POINT('',(31.0999914639398,822.864750104091,124.565859290805));
#76677=CARTESIAN_POINT('',(31.0999914639398,826.45468070076,114.408567507814));
#76678=CARTESIAN_POINT('Origin',(31.0999914639398,822.393327873482,124.399242723538));
#76679=CARTESIAN_POINT('Origin',(27.6697845773275,822.940231179145,113.166442132503));
#76680=CARTESIAN_POINT('',(27.6697845773275,821.073912726923,123.932916767216));
#76681=CARTESIAN_POINT('Origin',(27.6697845773275,819.350300582477,123.323733915494));
#76682=CARTESIAN_POINT('',(27.6697845773275,821.740378995992,122.047227844781));
#76683=CARTESIAN_POINT('',(27.6697845773275,824.663843323592,113.775624984225));
#76684=CARTESIAN_POINT('Origin',(27.6697845773275,820.016766851545,121.438044993059));
#76685=CARTESIAN_POINT('Origin',(27.6697845773275,822.940231179145,113.166442132503));
#76686=CARTESIAN_POINT('',(27.6697845773275,821.276814547639,119.373337375991));
#76687=CARTESIAN_POINT('Origin',(27.6697845773275,820.80539231703,119.206720808724));
#76688=CARTESIAN_POINT('',(27.6697845773275,819.821722813085,123.490350482761));
#76689=CARTESIAN_POINT('',(27.6697845773275,823.411653409754,113.33305869977));
#76690=CARTESIAN_POINT('Origin',(27.6697845773275,819.350300582477,123.323733915494));
#76691=CARTESIAN_POINT('Origin',(24.3956323595381,819.227059741242,111.854081708051));
#76692=CARTESIAN_POINT('',(24.3956323595381,817.389328542135,122.630660045289));
#76693=CARTESIAN_POINT('Origin',(24.3956323595381,815.637129144574,122.011373491042));
#76694=CARTESIAN_POINT('',(24.3956323595381,818.055794811203,120.744971122854));
#76695=CARTESIAN_POINT('',(24.3956323595381,820.979259138803,112.473368262298));
#76696=CARTESIAN_POINT('Origin',(24.3956323595381,816.303595413642,120.125684568607));
#76697=CARTESIAN_POINT('Origin',(24.3956323595381,819.227059741242,111.854081708051));
#76698=CARTESIAN_POINT('',(24.3956323595381,817.563643109736,118.060976951539));
#76699=CARTESIAN_POINT('Origin',(24.3956323595381,817.092220879127,117.894360384272));
#76700=CARTESIAN_POINT('',(24.3956323595381,816.108551375182,122.177990058309));
#76701=CARTESIAN_POINT('',(24.3956323595381,819.698481971851,112.020698275318));
#76702=CARTESIAN_POINT('Origin',(24.3956323595381,815.637129144574,122.011373491042));
#76703=CARTESIAN_POINT('Origin',(22.4120439649557,815.147387523168,110.412187507023));
#76704=CARTESIAN_POINT('',(22.4120439649557,813.26669927488,121.173583369593));
#76705=CARTESIAN_POINT('Origin',(22.4120439649557,811.5574569265,120.569479290015));
#76706=CARTESIAN_POINT('',(22.4120439649557,813.933165543949,119.287894447158));
#76707=CARTESIAN_POINT('',(22.4120439649557,816.856629871549,111.016291586602));
#76708=CARTESIAN_POINT('Origin',(22.4120439649557,812.223923195568,118.68379036758));
#76709=CARTESIAN_POINT('Origin',(22.4120439649557,815.147387523168,110.412187507023));
#76710=CARTESIAN_POINT('',(22.4120439649557,813.483970891662,116.619082750512));
#76711=CARTESIAN_POINT('Origin',(22.4120439649557,813.012548661053,116.452466183245));
#76712=CARTESIAN_POINT('',(22.4120439649557,812.028879157109,120.736095857282));
#76713=CARTESIAN_POINT('',(22.4120439649557,815.618809753777,110.578804074291));
#76714=CARTESIAN_POINT('Origin',(22.4120439649557,811.5574569265,120.569479290015));
#76715=CARTESIAN_POINT('Origin',(20.3577287479766,809.943855336583,108.573083166371));
#76716=CARTESIAN_POINT('',(20.3577287479766,808.156139889955,119.367338762861));
#76717=CARTESIAN_POINT('Origin',(20.3577287479766,806.353924739914,118.730374949362));
#76718=CARTESIAN_POINT('',(20.3577287479766,808.822606159023,117.481649840425));
#76719=CARTESIAN_POINT('',(20.3577287479766,811.746070486623,109.210046979869));
#76720=CARTESIAN_POINT('Origin',(20.3577287479766,807.020391008982,116.844686026927));
#76721=CARTESIAN_POINT('Origin',(20.3577287479766,809.943855336583,108.573083166371));
#76722=CARTESIAN_POINT('',(20.3577287479766,808.280438705076,114.779978409859));
#76723=CARTESIAN_POINT('Origin',(20.3577287479766,807.809016474468,114.613361842592));
#76724=CARTESIAN_POINT('',(20.3577287479766,806.825346970523,118.896991516629));
#76725=CARTESIAN_POINT('',(20.3577287479766,810.415277567191,108.739699733638));
#76726=CARTESIAN_POINT('Origin',(20.3577287479766,806.353924739914,118.730374949362));
#76727=CARTESIAN_POINT('Origin',(19.7330633002943,804.999379047125,106.825537945139));
#76728=CARTESIAN_POINT('',(19.7330633002943,802.870547266253,117.499231487147));
#76729=CARTESIAN_POINT('Origin',(19.7330633002943,801.409448450456,116.98282972813));
#76730=CARTESIAN_POINT('',(19.7330633002943,803.537013535322,115.613542564712));
#76731=CARTESIAN_POINT('',(19.7330633002943,806.460477862922,107.341939704156));
#76732=CARTESIAN_POINT('Origin',(19.7330633002943,802.075914719524,115.097140805695));
#76733=CARTESIAN_POINT('Origin',(19.7330633002943,804.999379047125,106.825537945139));
#76734=CARTESIAN_POINT('',(19.7330633002943,803.335962415618,113.032433188627));
#76735=CARTESIAN_POINT('Origin',(19.7330633002943,802.864540185009,112.86581662136));
#76736=CARTESIAN_POINT('',(19.7330633002943,801.880870681065,117.149446295397));
#76737=CARTESIAN_POINT('',(19.7330633002943,805.470801277733,106.992154512406));
#76738=CARTESIAN_POINT('Origin',(19.7330633002943,801.409448450456,116.98282972813));
#76739=CARTESIAN_POINT('Origin',(19.8082279830515,799.205375633292,104.777741093684));
#76740=CARTESIAN_POINT('',(19.8082279830515,796.802826613586,115.354693702033));
#76741=CARTESIAN_POINT('Origin',(19.8082279830515,795.615445036624,114.935032876675));
#76742=CARTESIAN_POINT('',(19.8082279830515,797.469292882654,113.469004779598));
#76743=CARTESIAN_POINT('',(19.8082279830515,800.392757210254,105.197401919042));
#76744=CARTESIAN_POINT('',(19.7284454031586,797.466907750936,113.468161793346));
#76745=CARTESIAN_POINT('Origin',(19.8082279830522,796.281911305691,113.049343954239));
#76746=CARTESIAN_POINT('',(21.061492498137,796.165218265362,113.008100685379));
#76747=CARTESIAN_POINT('Ctrl Pts',(21.0614924981326,796.165218265362,113.008100685379));
#76748=CARTESIAN_POINT('Ctrl Pts',(21.051798009416,796.072662642909,112.975388396707));
#76749=CARTESIAN_POINT('Ctrl Pts',(21.030581995983,795.981260194669,112.943217870007));
#76750=CARTESIAN_POINT('Ctrl Pts',(20.9482250146403,795.756960391498,112.864801980375));
#76751=CARTESIAN_POINT('Ctrl Pts',(20.8725787658467,795.630530765864,112.821124628641));
#76752=CARTESIAN_POINT('Ctrl Pts',(20.67567293284,795.407198225804,112.745382807087));
#76753=CARTESIAN_POINT('Ctrl Pts',(20.5553985159303,795.312693260727,112.71415839815));
#76754=CARTESIAN_POINT('Ctrl Pts',(20.2762522758205,795.164715767788,112.667177037225));
#76755=CARTESIAN_POINT('Ctrl Pts',(20.118103337146,795.11564868478,112.652972245053));
#76756=CARTESIAN_POINT('Ctrl Pts',(19.792769730301,795.077819089887,112.645735012025));
#76757=CARTESIAN_POINT('Ctrl Pts',(19.6287529031382,795.088828338619,112.652551589102));
#76758=CARTESIAN_POINT('Ctrl Pts',(19.3140101801986,795.16965780951,112.685770924614));
#76759=CARTESIAN_POINT('Ctrl Pts',(19.1663375993738,795.238951474633,112.711926900593));
#76760=CARTESIAN_POINT('Ctrl Pts',(18.9892241897138,795.368014120911,112.758514326216));
#76761=CARTESIAN_POINT('Ctrl Pts',(18.9442069834037,795.406034668372,112.772084785551));
#76762=CARTESIAN_POINT('Ctrl Pts',(18.9022600487226,795.446994874529,112.78656150833));
#76763=CARTESIAN_POINT('Ctrl Pts',(18.7875711892465,795.558985878489,112.82614291844));
#76764=CARTESIAN_POINT('Ctrl Pts',(18.6973577013089,795.69146959996,112.871957729857));
#76765=CARTESIAN_POINT('Ctrl Pts',(18.5757316682768,795.983261361675,112.9713963271));
#76766=CARTESIAN_POINT('Ctrl Pts',(18.5459381968071,796.139877355637,113.024102720641));
#76767=CARTESIAN_POINT('Ctrl Pts',(18.5522635281122,796.455913449457,113.129825565382));
#76768=CARTESIAN_POINT('Ctrl Pts',(18.5886152141294,796.612211023319,113.181809569817));
#76769=CARTESIAN_POINT('Ctrl Pts',(18.7195813826428,796.893916373066,113.275536973982));
#76770=CARTESIAN_POINT('Ctrl Pts',(18.8095884522755,797.018099714331,113.316879418162));
#76771=CARTESIAN_POINT('Ctrl Pts',(19.0294088382157,797.224902079374,113.386034899408));
#76772=CARTESIAN_POINT('Ctrl Pts',(19.1559698441546,797.307075171622,113.413687062561));
#76773=CARTESIAN_POINT('Ctrl Pts',(19.4319539624635,797.423754998297,113.45322603606));
#76774=CARTESIAN_POINT('Ctrl Pts',(19.5787789720714,797.457950071032,113.464995846177));
#76775=CARTESIAN_POINT('Ctrl Pts',(19.7284454031586,797.466907750936,113.468161793346));
#76776=CARTESIAN_POINT('Origin',(19.8082279830522,796.281911305691,113.049343954239));
#76777=CARTESIAN_POINT('Origin',(19.8082279830515,799.205375633292,104.777741093684));
#76778=CARTESIAN_POINT('',(19.8082279830515,797.541959001786,110.984636337172));
#76779=CARTESIAN_POINT('Origin',(19.8082279830515,797.070536771177,110.818019769905));
#76780=CARTESIAN_POINT('',(19.8082279830515,796.086867267232,115.101649443942));
#76781=CARTESIAN_POINT('',(19.8082279830515,799.676797863901,104.944357660951));
#76782=CARTESIAN_POINT('Origin',(19.8082279830515,795.615445036624,114.935032876675));
#76783=CARTESIAN_POINT('Origin',(39.4725260813523,832.414250098087,116.514880979901));
#76784=CARTESIAN_POINT('',(39.4725260813523,829.822681920545,127.025027822248));
#76785=CARTESIAN_POINT('Origin',(39.4725260813523,828.824319501418,126.672172762892));
#76786=CARTESIAN_POINT('',(39.4725260813523,830.489148189613,125.139338899813));
#76787=CARTESIAN_POINT('',(39.4725260813523,833.412612517214,116.867736039257));
#76788=CARTESIAN_POINT('Origin',(39.4725260813523,829.490785770486,124.786483840457));
#76789=CARTESIAN_POINT('Origin',(39.4725260813523,832.414250098087,116.514880979901));
#76790=CARTESIAN_POINT('',(39.4725260813523,830.75083346658,122.721776223389));
#76791=CARTESIAN_POINT('Origin',(39.4725260813523,830.279411235971,122.555159656122));
#76792=CARTESIAN_POINT('',(39.4725260813523,829.295741732027,126.838789330159));
#76793=CARTESIAN_POINT('',(39.4725260813523,832.885672328695,116.681497547168));
#76794=CARTESIAN_POINT('Origin',(39.4725260813523,828.824319501418,126.672172762892));
#76795=CARTESIAN_POINT('Origin',(35.3463285167995,831.748635708716,116.279630333071));
#76796=CARTESIAN_POINT('',(35.3463285167995,829.38047439143,126.868736718993));
#76797=CARTESIAN_POINT('Origin',(35.3463285167995,828.158705112047,126.436922116062));
#76798=CARTESIAN_POINT('',(35.3463285167995,830.046940660498,124.983047796558));
#76799=CARTESIAN_POINT('',(35.3463285167995,832.970404988099,116.711444936002));
#76800=CARTESIAN_POINT('Origin',(35.3463285167995,828.825171381116,124.551233193627));
#76801=CARTESIAN_POINT('Origin',(35.3463285167995,831.748635708716,116.279630333071));
#76802=CARTESIAN_POINT('',(35.3463285167995,830.08521907721,122.48652557656));
#76803=CARTESIAN_POINT('Origin',(35.3463285167995,829.613796846601,122.319909009292));
#76804=CARTESIAN_POINT('',(35.3463285167995,828.630127342656,126.60353868333));
#76805=CARTESIAN_POINT('',(35.3463285167995,832.220057939325,116.446246900338));
#76806=CARTESIAN_POINT('Origin',(35.3463285167995,828.158705112047,126.436922116062));
#76807=CARTESIAN_POINT('Origin',(30.8421163274859,830.325005751029,115.776471336301));
#76808=CARTESIAN_POINT('',(30.8421163274859,828.249791556361,126.46911514747));
#76809=CARTESIAN_POINT('Origin',(30.8421163274859,826.73507515436,125.933763119292));
#76810=CARTESIAN_POINT('',(30.8421163274859,828.916257825429,124.583426225035));
#76811=CARTESIAN_POINT('',(30.8421163274859,831.839722153029,116.311823364479));
#76812=CARTESIAN_POINT('Origin',(30.8421163274859,827.401541423429,124.048074196857));
#76813=CARTESIAN_POINT('Origin',(30.8421163274859,830.325005751029,115.776471336301));
#76814=CARTESIAN_POINT('',(30.8421163274859,828.661589119523,121.983366579789));
#76815=CARTESIAN_POINT('Origin',(30.8421163274859,828.190166888914,121.816750012522));
#76816=CARTESIAN_POINT('',(30.8421163274859,827.206497384969,126.100379686559));
#76817=CARTESIAN_POINT('',(30.8421163274859,830.796427981638,115.943087903568));
#76818=CARTESIAN_POINT('Origin',(30.8421163274859,826.73507515436,125.933763119292));
#76819=CARTESIAN_POINT('Origin',(26.8158334165305,828.02089382737,114.962120220904));
#76820=CARTESIAN_POINT('',(26.8158334165305,826.154575375148,125.728594855617));
#76821=CARTESIAN_POINT('Origin',(26.8158334165305,824.430963230701,125.119412003895));
#76822=CARTESIAN_POINT('',(26.8158334165305,826.821041644216,123.842905933182));
#76823=CARTESIAN_POINT('',(26.8158334165305,829.744505971817,115.571303072626));
#76824=CARTESIAN_POINT('Origin',(26.8158334165305,825.09742949977,123.23372308146));
#76825=CARTESIAN_POINT('Origin',(26.8158334165305,828.02089382737,114.962120220904));
#76826=CARTESIAN_POINT('',(26.8158334165305,826.357477195864,121.169015464392));
#76827=CARTESIAN_POINT('Origin',(26.8158334165305,825.886054965255,121.002398897125));
#76828=CARTESIAN_POINT('',(26.8158334165305,824.90238546131,125.286028571162));
#76829=CARTESIAN_POINT('',(26.8158334165305,828.492316057979,115.128736788171));
#76830=CARTESIAN_POINT('Origin',(26.8158334165305,824.430963230701,125.119412003895));
#76831=CARTESIAN_POINT('Origin',(22.7944179240885,825.030690869403,113.905281319512));
#76832=CARTESIAN_POINT('',(22.7944179240885,823.192959670296,124.68185965675));
#76833=CARTESIAN_POINT('Origin',(22.7944179240885,821.440760272734,124.062573102503));
#76834=CARTESIAN_POINT('',(22.7944179240885,823.859425939364,122.796170734315));
#76835=CARTESIAN_POINT('',(22.7944179240885,826.782890266964,114.524567873759));
#76836=CARTESIAN_POINT('Origin',(22.7944179240885,822.107226541802,122.176884180068));
#76837=CARTESIAN_POINT('Origin',(22.7944179240885,825.030690869403,113.905281319512));
#76838=CARTESIAN_POINT('',(22.7944179240885,823.367274237896,120.112176563));
#76839=CARTESIAN_POINT('Origin',(22.7944179240885,822.895852007288,119.945559995733));
#76840=CARTESIAN_POINT('',(22.7944179240885,821.912182503343,124.22918966977));
#76841=CARTESIAN_POINT('',(22.7944179240885,825.502113100012,114.071897886779));
#76842=CARTESIAN_POINT('Origin',(22.7944179240885,821.440760272734,124.062573102503));
#76843=CARTESIAN_POINT('Origin',(19.9545452854761,821.42900890921,112.632325048824));
#76844=CARTESIAN_POINT('',(19.9545452854761,819.548320660922,123.393720911393));
#76845=CARTESIAN_POINT('Origin',(19.9545452854761,817.839078312542,122.789616831815));
#76846=CARTESIAN_POINT('',(19.9545452854761,820.21478692999,121.508031988958));
#76847=CARTESIAN_POINT('',(19.9545452854761,823.138251257591,113.236429128402));
#76848=CARTESIAN_POINT('Origin',(19.9545452854761,818.50554458161,120.90392790938));
#76849=CARTESIAN_POINT('Origin',(19.9545452854761,821.42900890921,112.632325048824));
#76850=CARTESIAN_POINT('',(19.9545452854761,819.765592277704,118.839220292312));
#76851=CARTESIAN_POINT('Origin',(19.9545452854761,819.294170047095,118.672603725045));
#76852=CARTESIAN_POINT('',(19.9545452854761,818.31050054315,122.956233399082));
#76853=CARTESIAN_POINT('',(19.9545452854761,821.900431139819,112.798941616091));
#76854=CARTESIAN_POINT('Origin',(19.9545452854761,817.839078312542,122.789616831815));
#76855=CARTESIAN_POINT('Origin',(16.7976629836891,816.741890482106,110.975738804068));
#76856=CARTESIAN_POINT('',(16.7976629836891,814.954175035478,121.769994400558));
#76857=CARTESIAN_POINT('Origin',(16.7976629836891,813.151959885437,121.13303058706));
#76858=CARTESIAN_POINT('',(16.7976629836891,815.620641304546,119.884305478123));
#76859=CARTESIAN_POINT('',(16.7976629836891,818.544105632146,111.612702617567));
#76860=CARTESIAN_POINT('Origin',(16.7976629836891,813.818426154505,119.247341664624));
#76861=CARTESIAN_POINT('Origin',(16.7976629836891,816.741890482106,110.975738804068));
#76862=CARTESIAN_POINT('',(16.7976629836891,815.078473850599,117.182634047557));
#76863=CARTESIAN_POINT('Origin',(16.7976629836891,814.60705161999,117.016017480289));
#76864=CARTESIAN_POINT('',(16.7976629836891,813.623382116046,121.299647154327));
#76865=CARTESIAN_POINT('',(16.7976629836891,817.213312712714,111.142355371335));
#76866=CARTESIAN_POINT('Origin',(16.7976629836891,813.151959885437,121.13303058706));
#76867=CARTESIAN_POINT('Origin',(15.0963149794262,812.027915022255,109.30966037521));
#76868=CARTESIAN_POINT('',(15.0963149794262,809.899083241384,119.983353917218));
#76869=CARTESIAN_POINT('Origin',(15.0963149794262,808.437984425586,119.466952158201));
#76870=CARTESIAN_POINT('',(15.0963149794262,810.565549510452,118.097664994783));
#76871=CARTESIAN_POINT('',(15.0963149794262,813.489013838052,109.826062134227));
#76872=CARTESIAN_POINT('Origin',(15.0963149794262,809.104450694654,117.581263235766));
#76873=CARTESIAN_POINT('Origin',(15.0963149794262,812.027915022255,109.30966037521));
#76874=CARTESIAN_POINT('',(15.0963149794262,810.364498390749,115.516555618698));
#76875=CARTESIAN_POINT('Origin',(15.0963149794262,809.893076160139,115.349939051431));
#76876=CARTESIAN_POINT('',(15.0963149794262,808.909406656195,119.633568725468));
#76877=CARTESIAN_POINT('',(15.0963149794262,812.499337252864,109.476276942477));
#76878=CARTESIAN_POINT('Origin',(15.0963149794262,808.437984425586,119.466952158201));
#76879=CARTESIAN_POINT('Origin',(13.8921703539818,806.345790072918,107.30140515861));
#76880=CARTESIAN_POINT('',(13.8921703539818,803.943241053211,117.87835776696));
#76881=CARTESIAN_POINT('Origin',(13.8921703539818,802.755859476249,117.458696941601));
#76882=CARTESIAN_POINT('',(13.8921703526055,804.609653252271,115.992821829335));
#76883=CARTESIAN_POINT('',(13.8921703539818,807.53317164988,107.721065983968));
#76884=CARTESIAN_POINT('',(15.0923154240742,803.062507307636,115.445836008528));
#76885=CARTESIAN_POINT('Ctrl Pts',(13.892170353543,804.609653252273,115.992821829331));
#76886=CARTESIAN_POINT('Ctrl Pts',(13.8039600128603,804.609598801071,115.992975892591));
#76887=CARTESIAN_POINT('Ctrl Pts',(13.7158062647662,804.600761138376,115.990168610606));
#76888=CARTESIAN_POINT('Ctrl Pts',(13.4803696455484,804.552934593457,115.97461895202));
#76889=CARTESIAN_POINT('Ctrl Pts',(13.3385502159868,804.497357182754,115.956366602613));
#76890=CARTESIAN_POINT('Ctrl Pts',(13.078202995359,804.338137961123,115.904028614265));
#76891=CARTESIAN_POINT('Ctrl Pts',(12.9629550049546,804.234294769472,115.869875067184));
#76892=CARTESIAN_POINT('Ctrl Pts',(12.7731347945951,803.984378370213,115.787382953728));
#76893=CARTESIAN_POINT('Ctrl Pts',(12.7033371078485,803.838599875019,115.739116747616));
#76894=CARTESIAN_POINT('Ctrl Pts',(12.6278731521198,803.530668849765,115.636258508348));
#76895=CARTESIAN_POINT('Ctrl Pts',(12.6226627237605,803.371616751307,115.58269111305));
#76896=CARTESIAN_POINT('Ctrl Pts',(12.677542057288,803.0623338468,115.477070554118));
#76897=CARTESIAN_POINT('Ctrl Pts',(12.7366394034306,802.915053877657,115.426026248129));
#76898=CARTESIAN_POINT('Ctrl Pts',(12.8241262990056,802.783027873801,115.379363791155));
#76899=CARTESIAN_POINT('Ctrl Pts',(12.8561242376968,802.734739956517,115.362297207324));
#76900=CARTESIAN_POINT('Ctrl Pts',(12.8917644004736,802.688726510102,115.345901787053));
#76901=CARTESIAN_POINT('Ctrl Pts',(13.0364797953235,802.527771612137,115.288042560581));
#76902=CARTESIAN_POINT('Ctrl Pts',(13.1655296844413,802.431055595334,115.25219459766));
#76903=CARTESIAN_POINT('Ctrl Pts',(13.4552481156411,802.290325870049,115.19780448547));
#76904=CARTESIAN_POINT('Ctrl Pts',(13.613050383001,802.247425331864,115.179716447631));
#76905=CARTESIAN_POINT('Ctrl Pts',(13.9391917620889,802.220695745209,115.164136281486));
#76906=CARTESIAN_POINT('Ctrl Pts',(14.104487459637,802.237710452545,115.167012679576));
#76907=CARTESIAN_POINT('Ctrl Pts',(14.4097964864331,802.327770213418,115.193523954294));
#76908=CARTESIAN_POINT('Ctrl Pts',(14.5481315972824,802.396647764069,115.215690767848));
#76909=CARTESIAN_POINT('Ctrl Pts',(14.7897617083049,802.576522731334,115.276073212751));
#76910=CARTESIAN_POINT('Ctrl Pts',(14.8915648013111,802.685367669113,115.313535540805));
#76911=CARTESIAN_POINT('Ctrl Pts',(15.02152410657,802.888627576681,115.384515219428));
#76912=CARTESIAN_POINT('Ctrl Pts',(15.0624228462959,802.973874642577,115.414510225735));
#76913=CARTESIAN_POINT('Ctrl Pts',(15.0923154240733,803.062507307637,115.445836008528));
#76914=CARTESIAN_POINT('',(14.0754411389211,804.597066825487,115.988201265256));
#76915=CARTESIAN_POINT('Origin',(13.8921703539826,803.422325745316,115.573008019166));
#76916=CARTESIAN_POINT('Ctrl Pts',(14.0754411389211,804.597066825487,115.988201265256));
#76917=CARTESIAN_POINT('Ctrl Pts',(14.0146511156019,804.605497522896,115.99118095898));
#76918=CARTESIAN_POINT('Ctrl Pts',(13.9533971024774,804.609691046822,115.992714894107));
#76919=CARTESIAN_POINT('Ctrl Pts',(13.892170353543,804.609653252273,115.992821829331));
#76920=CARTESIAN_POINT('Origin',(13.8921703539818,806.345790072918,107.30140515861));
#76921=CARTESIAN_POINT('',(13.8921703539818,804.682373441412,113.508300402098));
#76922=CARTESIAN_POINT('Origin',(13.8921703539818,804.210951210803,113.341683834831));
#76923=CARTESIAN_POINT('',(13.8921703539818,803.227281706858,117.625313508868));
#76924=CARTESIAN_POINT('',(13.8921703539818,806.817212303527,107.468021725877));
#76925=CARTESIAN_POINT('Origin',(13.8921703539818,802.755859476249,117.458696941601));
#76926=CARTESIAN_POINT('Origin',(40.4498234438578,834.974210333533,117.419657545528));
#76927=CARTESIAN_POINT('',(40.4498234438578,832.382642155992,127.929804387875));
#76928=CARTESIAN_POINT('Origin',(40.4498234438578,831.384279736864,127.576949328519));
#76929=CARTESIAN_POINT('',(40.4498234438578,833.04910842506,126.04411546544));
#76930=CARTESIAN_POINT('',(40.4498234438578,835.97257275266,117.772512604884));
#76931=CARTESIAN_POINT('Origin',(40.4498234438578,832.050746005933,125.691260406084));
#76932=CARTESIAN_POINT('Origin',(40.4498234438578,834.974210333533,117.419657545528));
#76933=CARTESIAN_POINT('',(40.4498234438578,833.310793702027,123.626552789016));
#76934=CARTESIAN_POINT('Origin',(40.4498234438578,832.839371471418,123.459936221749));
#76935=CARTESIAN_POINT('',(40.4498234438578,831.855701967473,127.743565895786));
#76936=CARTESIAN_POINT('',(40.4498234438578,835.445632564142,117.586274112795));
#76937=CARTESIAN_POINT('Origin',(40.4498234438578,831.384279736864,127.576949328519));
#76938=CARTESIAN_POINT('Origin',(36.2670149956938,835.131993064906,117.475423301507));
#76939=CARTESIAN_POINT('',(36.2670149956938,832.76383174762,128.064529687429));
#76940=CARTESIAN_POINT('Origin',(36.2670149956938,831.542062468237,127.632715084498));
#76941=CARTESIAN_POINT('',(36.2670149956938,833.430298016688,126.178840764994));
#76942=CARTESIAN_POINT('',(36.2670149956938,836.353762344289,117.907237904438));
#76943=CARTESIAN_POINT('Origin',(36.2670149956938,832.208528737306,125.747026162063));
#76944=CARTESIAN_POINT('Origin',(36.2670149956938,835.131993064906,117.475423301507));
#76945=CARTESIAN_POINT('',(36.2670149956938,833.4685764334,123.682318544995));
#76946=CARTESIAN_POINT('Origin',(36.2670149956938,832.997154202791,123.515701977728));
#76947=CARTESIAN_POINT('',(36.2670149956938,832.013484698846,127.799331651765));
#76948=CARTESIAN_POINT('',(36.2670149956938,835.603415295515,117.642039868774));
#76949=CARTESIAN_POINT('Origin',(36.2670149956938,831.542062468237,127.632715084498));
#76950=CARTESIAN_POINT('Origin',(31.547298369302,834.622426283629,117.295325159381));
#76951=CARTESIAN_POINT('',(31.547298369302,832.547212088961,127.98796897055));
#76952=CARTESIAN_POINT('Origin',(31.547298369302,831.032495686961,127.452616942372));
#76953=CARTESIAN_POINT('',(31.547298369302,833.21367835803,126.102280048115));
#76954=CARTESIAN_POINT('',(31.547298369302,836.13714268563,117.830677187558));
#76955=CARTESIAN_POINT('Origin',(31.547298369302,831.698961956029,125.566928019937));
#76956=CARTESIAN_POINT('Origin',(31.547298369302,834.622426283629,117.295325159381));
#76957=CARTESIAN_POINT('',(31.547298369302,832.959009652123,123.502220402869));
#76958=CARTESIAN_POINT('Origin',(31.547298369302,832.487587421514,123.335603835602));
#76959=CARTESIAN_POINT('',(31.547298369302,831.503917917569,127.619233509639));
#76960=CARTESIAN_POINT('',(31.547298369302,835.093848514238,117.461941726648));
#76961=CARTESIAN_POINT('Origin',(31.547298369302,831.032495686961,127.452616942372));
#76962=CARTESIAN_POINT('Origin',(27.1009073174613,833.157930474737,116.777722788063));
#76963=CARTESIAN_POINT('',(27.1009073174613,831.291612022515,127.544197422777));
#76964=CARTESIAN_POINT('Origin',(27.1009073174613,829.567999878068,126.935014571055));
#76965=CARTESIAN_POINT('',(27.1009073174613,831.958078291583,125.658508500342));
#76966=CARTESIAN_POINT('',(27.1009073174613,834.881542619183,117.386905639786));
#76967=CARTESIAN_POINT('Origin',(27.1009073174613,830.234466147136,125.04932564862));
#76968=CARTESIAN_POINT('Origin',(27.1009073174613,833.157930474737,116.777722788063));
#76969=CARTESIAN_POINT('',(27.1009073174613,831.49451384323,122.984618031552));
#76970=CARTESIAN_POINT('Origin',(27.1009073174613,831.023091612622,122.818001464285));
#76971=CARTESIAN_POINT('',(27.1009073174613,830.039422108677,127.101631138322));
#76972=CARTESIAN_POINT('',(27.1009073174613,833.629352705345,116.944339355331));
#76973=CARTESIAN_POINT('Origin',(27.1009073174613,829.567999878068,126.935014571055));
#76974=CARTESIAN_POINT('Origin',(22.5079837042789,831.021382214555,116.022594340998));
#76975=CARTESIAN_POINT('',(22.5079837042789,829.183651015447,126.799172678236));
#76976=CARTESIAN_POINT('Origin',(22.5079837042789,827.431451617886,126.179886123989));
#76977=CARTESIAN_POINT('',(22.5079837042789,829.850117284516,124.913483755801));
#76978=CARTESIAN_POINT('',(22.5079837042789,832.773581612116,116.641880895245));
#76979=CARTESIAN_POINT('Origin',(22.5079837042789,828.097917886954,124.294197201554));
#76980=CARTESIAN_POINT('Origin',(22.5079837042789,831.021382214555,116.022594340998));
#76981=CARTESIAN_POINT('',(22.5079837042789,829.357965583048,122.229489584486));
#76982=CARTESIAN_POINT('Origin',(22.5079837042789,828.88654335244,122.062873017219));
#76983=CARTESIAN_POINT('',(22.5079837042789,827.902873848495,126.346502691256));
#76984=CARTESIAN_POINT('',(22.5079837042789,831.492804445163,116.189210908265));
#76985=CARTESIAN_POINT('Origin',(22.5079837042789,827.431451617886,126.179886123989));
#76986=CARTESIAN_POINT('Origin',(14.8144644015597,824.089246195621,113.57254291722));
#76987=CARTESIAN_POINT('',(14.8144644015597,822.301530748994,124.36679851371));
#76988=CARTESIAN_POINT('Origin',(14.8144644015597,820.499315598953,123.729834700212));
#76989=CARTESIAN_POINT('',(14.8144644015597,822.967997018062,122.481109591275));
#76990=CARTESIAN_POINT('',(14.8144644015597,825.891461345662,114.209506730719));
#76991=CARTESIAN_POINT('Origin',(14.8144644015597,821.165781868021,121.844145777777));
#76992=CARTESIAN_POINT('Origin',(14.8144644015597,824.089246195621,113.57254291722));
#76993=CARTESIAN_POINT('',(14.8144644015597,822.425829564115,119.779438160709));
#76994=CARTESIAN_POINT('Origin',(14.8144644015597,821.954407333506,119.612821593442));
#76995=CARTESIAN_POINT('',(14.8144644015597,820.970737829562,123.896451267479));
#76996=CARTESIAN_POINT('',(14.8144644015597,824.56066842623,113.739159484487));
#76997=CARTESIAN_POINT('Origin',(14.8144644015597,820.499315598953,123.729834700212));
#76998=CARTESIAN_POINT('Origin',(12.110790912476,819.811794913137,112.060746902808));
#76999=CARTESIAN_POINT('',(12.110790912476,817.682963132266,122.734440444817));
#77000=CARTESIAN_POINT('Origin',(12.110790912476,816.221864316469,122.218038685799));
#77001=CARTESIAN_POINT('',(12.110790912476,818.349429401335,120.848751522381));
#77002=CARTESIAN_POINT('',(12.110790912476,821.272893728935,112.577148661825));
#77003=CARTESIAN_POINT('Origin',(12.110790912476,816.888330585537,120.332349763364));
#77004=CARTESIAN_POINT('Origin',(12.110790912476,819.811794913137,112.060746902808));
#77005=CARTESIAN_POINT('',(12.110790912476,818.148378281631,118.267642146296));
#77006=CARTESIAN_POINT('Origin',(12.110790912476,817.676956051022,118.101025579029));
#77007=CARTESIAN_POINT('',(12.110790912476,816.693286547077,122.384655253066));
#77008=CARTESIAN_POINT('',(12.110790912476,820.283217143746,112.227363470075));
#77009=CARTESIAN_POINT('Origin',(12.110790912476,816.221864316469,122.218038685799));
#77010=CARTESIAN_POINT('Origin',(9.67996387708925,814.489884554442,110.179803710707));
#77011=CARTESIAN_POINT('',(9.67996387708925,812.087335534736,120.756756319056));
#77012=CARTESIAN_POINT('Origin',(9.67996387708925,810.899953957774,120.337095493698));
#77013=CARTESIAN_POINT('',(9.67996387708875,812.75343949573,118.872092505248));
#77014=CARTESIAN_POINT('',(9.67996387708925,815.677266131404,110.599464536065));
#77015=CARTESIAN_POINT('',(10.7745374036936,810.979202184137,118.243863845951));
#77016=CARTESIAN_POINT('Ctrl Pts',(9.67996387708853,812.75343949573,118.872092505248));
#77017=CARTESIAN_POINT('Ctrl Pts',(9.67956979645961,812.753438801654,118.872094469055));
#77018=CARTESIAN_POINT('Ctrl Pts',(9.67917570725331,812.753437932054,118.872096374398));
#77019=CARTESIAN_POINT('Ctrl Pts',(9.52661826611054,812.753033349318,118.872811309619));
#77020=CARTESIAN_POINT('Ctrl Pts',(9.37573860252287,812.726461524862,118.86481051582));
#77021=CARTESIAN_POINT('Ctrl Pts',(9.08624297003607,812.621730050792,118.831730341099));
#77022=CARTESIAN_POINT('Ctrl Pts',(8.95079094906213,812.542730464648,118.80635736481));
#77023=CARTESIAN_POINT('Ctrl Pts',(8.71041275090674,812.335445413876,118.738932612376));
#77024=CARTESIAN_POINT('Ctrl Pts',(8.61021955726934,812.206512495788,118.696620203197));
#77025=CARTESIAN_POINT('Ctrl Pts',(8.46891511410034,811.920062556869,118.601354106671));
#77026=CARTESIAN_POINT('Ctrl Pts',(8.4289285066343,811.765489346632,118.549369702018));
#77027=CARTESIAN_POINT('Ctrl Pts',(8.41466265044363,811.452181770553,118.442326687973));
#77028=CARTESIAN_POINT('Ctrl Pts',(8.44006101718495,811.296528534306,118.388322986074));
#77029=CARTESIAN_POINT('Ctrl Pts',(8.49652235171455,811.150237700456,118.336618855517));
#77030=CARTESIAN_POINT('Ctrl Pts',(8.51717283095315,811.096732485738,118.317708302242));
#77031=CARTESIAN_POINT('Ctrl Pts',(8.54187830406437,811.044738971098,118.299199323518));
#77032=CARTESIAN_POINT('Ctrl Pts',(8.64787092692629,810.858939674224,118.232559245842));
#77033=CARTESIAN_POINT('Ctrl Pts',(8.75265802493252,810.739051126119,118.188521326296));
#77034=CARTESIAN_POINT('Ctrl Pts',(9.004690078727,810.54463558224,118.11515682931));
#77035=CARTESIAN_POINT('Ctrl Pts',(9.14938106998037,810.47175888592,118.086474202917));
#77036=CARTESIAN_POINT('Ctrl Pts',(9.46207627804917,810.381722544442,118.04851928758));
#77037=CARTESIAN_POINT('Ctrl Pts',(9.62729451931023,810.365984329808,118.039819694823));
#77038=CARTESIAN_POINT('Ctrl Pts',(9.94542286328407,810.394263351174,118.044495565795));
#77039=CARTESIAN_POINT('Ctrl Pts',(10.0957727599236,810.434533099207,118.056551413935));
#77040=CARTESIAN_POINT('Ctrl Pts',(10.3715667536406,810.56313291787,118.098811486384));
#77041=CARTESIAN_POINT('Ctrl Pts',(10.4950774071888,810.649649951457,118.128382377614));
#77042=CARTESIAN_POINT('Ctrl Pts',(10.6669591911075,810.822998328889,118.188790309404));
#77043=CARTESIAN_POINT('Ctrl Pts',(10.725753185945,810.898366149242,118.215293656064));
#77044=CARTESIAN_POINT('Ctrl Pts',(10.7745374036927,810.979202184137,118.243863845952));
#77045=CARTESIAN_POINT('',(10.1182782141275,812.679564119701,118.844829287164));
#77046=CARTESIAN_POINT('Origin',(9.67996387708958,811.566420226841,118.451406571262));
#77047=CARTESIAN_POINT('Ctrl Pts',(10.1182782141275,812.679564119701,118.844829287164));
#77048=CARTESIAN_POINT('Ctrl Pts',(9.97805606177369,812.728647120432,118.862176880387));
#77049=CARTESIAN_POINT('Ctrl Pts',(9.82962852093729,812.753703093081,118.871346687152));
#77050=CARTESIAN_POINT('Ctrl Pts',(9.67996387708853,812.75343949573,118.872092505248));
#77051=CARTESIAN_POINT('Origin',(9.67996387708925,814.489884554442,110.179803710707));
#77052=CARTESIAN_POINT('',(9.67996387708925,812.826467922936,116.386698954195));
#77053=CARTESIAN_POINT('Origin',(9.67996387708925,812.355045692327,116.220082386928));
#77054=CARTESIAN_POINT('',(9.67996387708925,811.371376188383,120.503712060965));
#77055=CARTESIAN_POINT('',(9.67996387708925,814.961306785051,110.346420277974));
#77056=CARTESIAN_POINT('Origin',(9.67996387708925,810.899953957774,120.337095493698));
#77057=CARTESIAN_POINT('Origin',(41.970275080754,837.286651271087,118.236952416254));
#77058=CARTESIAN_POINT('',(41.970275080754,834.695083093546,128.747099258602));
#77059=CARTESIAN_POINT('Origin',(41.970275080754,833.696720674418,128.394244199246));
#77060=CARTESIAN_POINT('',(41.970275080754,835.361549362614,126.861410336167));
#77061=CARTESIAN_POINT('',(41.970275080754,838.285013690214,118.589807475611));
#77062=CARTESIAN_POINT('Origin',(41.970275080754,834.363186943487,126.50855527681));
#77063=CARTESIAN_POINT('Origin',(41.970275080754,837.286651271087,118.236952416254));
#77064=CARTESIAN_POINT('',(41.970275080754,835.623234639581,124.443847659743));
#77065=CARTESIAN_POINT('Origin',(41.970275080754,835.151812408972,124.277231092476));
#77066=CARTESIAN_POINT('',(41.970275080754,834.168142905027,128.560860766513));
#77067=CARTESIAN_POINT('',(41.970275080754,837.758073501696,118.403568983521));
#77068=CARTESIAN_POINT('Origin',(41.970275080754,833.696720674418,128.394244199246));
#77069=CARTESIAN_POINT('Origin',(37.9136645495052,838.260935260717,118.581297343913));
#77070=CARTESIAN_POINT('',(37.9136645495052,835.892773943431,129.170403729835));
#77071=CARTESIAN_POINT('Origin',(37.9136645495052,834.671004664049,128.738589126904));
#77072=CARTESIAN_POINT('',(37.9136645495052,836.5592402125,127.2847148074));
#77073=CARTESIAN_POINT('',(37.9136645495052,839.4827045401,119.013111946843));
#77074=CARTESIAN_POINT('Origin',(37.9136645495052,835.337470933117,126.852900204469));
#77075=CARTESIAN_POINT('Origin',(37.9136645495052,838.260935260717,118.581297343913));
#77076=CARTESIAN_POINT('',(37.9136645495052,836.597518629211,124.788192587401));
#77077=CARTESIAN_POINT('Origin',(37.9136645495052,836.126096398602,124.621576020134));
#77078=CARTESIAN_POINT('',(37.9136645495052,835.142426894657,128.905205694171));
#77079=CARTESIAN_POINT('',(37.9136645495052,838.732357491326,118.74791391118));
#77080=CARTESIAN_POINT('Origin',(37.9136645495052,834.671004664049,128.738589126904));
#77081=CARTESIAN_POINT('Origin',(33.1847177503218,838.687702169366,118.732131209448));
#77082=CARTESIAN_POINT('',(33.1847177503218,836.612487974698,129.424775020617));
#77083=CARTESIAN_POINT('Origin',(33.1847177503218,835.097771572697,128.889422992439));
#77084=CARTESIAN_POINT('',(33.1847177503218,837.278954243766,127.539086098182));
#77085=CARTESIAN_POINT('',(33.1847177503218,840.202418571366,119.267483237626));
#77086=CARTESIAN_POINT('Origin',(33.1847177503218,835.764237841765,127.003734070004));
#77087=CARTESIAN_POINT('Origin',(33.1847177503218,838.687702169366,118.732131209448));
#77088=CARTESIAN_POINT('',(33.1847177503218,837.024285537859,124.939026452937));
#77089=CARTESIAN_POINT('Origin',(33.1847177503218,836.552863307251,124.772409885669));
#77090=CARTESIAN_POINT('',(33.1847177503218,835.569193803306,129.056039559707));
#77091=CARTESIAN_POINT('',(33.1847177503218,839.159124399974,118.898747776715));
#77092=CARTESIAN_POINT('Origin',(33.1847177503218,835.097771572697,128.889422992439));
#77093=CARTESIAN_POINT('Origin',(28.5125471827126,838.126827969518,118.533899289569));
#77094=CARTESIAN_POINT('',(28.5125471827126,836.260509517296,129.300373924283));
#77095=CARTESIAN_POINT('Origin',(28.5125471827126,834.536897372849,128.69119107256));
#77096=CARTESIAN_POINT('',(28.5125471827126,836.926975786364,127.414685001848));
#77097=CARTESIAN_POINT('',(28.5125471827126,839.850440113965,119.143082141291));
#77098=CARTESIAN_POINT('Origin',(28.5125471827126,835.203363641918,126.805502150125));
#77099=CARTESIAN_POINT('Origin',(28.5125471827126,838.126827969518,118.533899289569));
#77100=CARTESIAN_POINT('',(28.5125471827126,836.463411338012,124.740794533057));
#77101=CARTESIAN_POINT('Origin',(28.5125471827126,835.991989107403,124.57417796579));
#77102=CARTESIAN_POINT('',(28.5125471827126,835.008319603458,128.857807639828));
#77103=CARTESIAN_POINT('',(28.5125471827126,838.598250200127,118.700515856836));
#77104=CARTESIAN_POINT('Origin',(28.5125471827126,834.536897372849,128.69119107256));
#77105=CARTESIAN_POINT('Origin',(23.5488482499785,836.937311818387,118.113484033474));
#77106=CARTESIAN_POINT('',(23.5488482499785,835.09958061928,128.890062370713));
#77107=CARTESIAN_POINT('Origin',(23.5488482499785,833.347381221719,128.270775816466));
#77108=CARTESIAN_POINT('',(23.5488482499785,835.766046888348,127.004373448277));
#77109=CARTESIAN_POINT('',(23.5488482499785,838.689511215949,118.732770587721));
#77110=CARTESIAN_POINT('Origin',(23.5488482499785,834.013847490787,126.385086894031));
#77111=CARTESIAN_POINT('Origin',(23.5488482499785,836.937311818387,118.113484033474));
#77112=CARTESIAN_POINT('',(23.5488482499785,835.273895186881,124.320379276963));
#77113=CARTESIAN_POINT('Origin',(23.5488482499785,834.802472956272,124.153762709696));
#77114=CARTESIAN_POINT('',(23.5488482499785,833.818803452328,128.437392383733));
#77115=CARTESIAN_POINT('',(23.5488482499785,837.408734048996,118.280100600741));
#77116=CARTESIAN_POINT('Origin',(23.5488482499785,833.347381221719,128.270775816466));
#77117=CARTESIAN_POINT('Origin',(19.4007545707989,834.736072652758,117.335491631552));
#77118=CARTESIAN_POINT('',(19.4007545707989,832.85538440447,128.096887494121));
#77119=CARTESIAN_POINT('Origin',(19.4007545707989,831.14614205609,127.492783414543));
#77120=CARTESIAN_POINT('',(19.4007545707989,833.521850673538,126.211198571686));
#77121=CARTESIAN_POINT('',(19.4007545707989,836.445315001138,117.93959571113));
#77122=CARTESIAN_POINT('Origin',(19.4007545707989,831.812608325158,125.607094492108));
#77123=CARTESIAN_POINT('Origin',(19.4007545707989,834.736072652758,117.335491631552));
#77124=CARTESIAN_POINT('',(19.4007545707989,833.072656021252,123.54238687504));
#77125=CARTESIAN_POINT('Origin',(19.4007545707989,832.601233790643,123.375770307773));
#77126=CARTESIAN_POINT('',(19.4007545707989,831.617564286698,127.65939998181));
#77127=CARTESIAN_POINT('',(19.4007545707989,835.207494883367,117.502108198819));
#77128=CARTESIAN_POINT('Origin',(19.4007545707989,831.14614205609,127.492783414543));
#77129=CARTESIAN_POINT('Origin',(14.4948082960701,831.664807775925,116.250002705234));
#77130=CARTESIAN_POINT('',(14.4948082960701,829.877092329297,127.044258301724));
#77131=CARTESIAN_POINT('Origin',(14.4948082960701,828.074877179256,126.407294488225));
#77132=CARTESIAN_POINT('',(14.4948082960701,830.543558598365,125.158569379288));
#77133=CARTESIAN_POINT('',(14.4948082960701,833.467022925965,116.886966518732));
#77134=CARTESIAN_POINT('Origin',(14.4948082960701,828.741343448324,124.52160556579));
#77135=CARTESIAN_POINT('Origin',(14.4948082960701,831.664807775925,116.250002705234));
#77136=CARTESIAN_POINT('',(14.4948082960701,830.001391144418,122.456897948722));
#77137=CARTESIAN_POINT('Origin',(14.4948082960701,829.52996891381,122.290281381455));
#77138=CARTESIAN_POINT('',(14.4948082960701,828.546299409865,126.573911055492));
#77139=CARTESIAN_POINT('',(14.4948082960701,832.136230006534,116.416619272501));
#77140=CARTESIAN_POINT('Origin',(14.4948082960701,828.074877179256,126.407294488225));
#77141=CARTESIAN_POINT('Origin',(10.9069728273033,828.01082581734,114.9585618455));
#77142=CARTESIAN_POINT('',(10.9069728273033,825.881994036469,125.632255387508));
#77143=CARTESIAN_POINT('Origin',(10.9069728273033,824.420895220671,125.115853628491));
#77144=CARTESIAN_POINT('',(10.9069728273033,826.548460305538,123.746566465073));
#77145=CARTESIAN_POINT('',(10.9069728273033,829.471924633138,115.474963604517));
#77146=CARTESIAN_POINT('Origin',(10.9069728273033,825.08736148974,123.230164706056));
#77147=CARTESIAN_POINT('Origin',(10.9069728273033,828.01082581734,114.9585618455));
#77148=CARTESIAN_POINT('',(10.9069728273033,826.347409185834,121.165457088988));
#77149=CARTESIAN_POINT('Origin',(10.9069728273033,825.875986955225,120.998840521721));
#77150=CARTESIAN_POINT('',(10.9069728273033,824.892317451281,125.282470195758));
#77151=CARTESIAN_POINT('',(10.9069728273033,828.482248047949,115.125178412767));
#77152=CARTESIAN_POINT('Origin',(10.9069728273033,824.420895220671,125.115853628491));
#77153=CARTESIAN_POINT('Origin',(7.35570218782278,823.281723069322,113.287136921158));
#77154=CARTESIAN_POINT('',(7.35570218782278,820.879174049615,123.864089529508));
#77155=CARTESIAN_POINT('Origin',(7.35570218782278,819.691792472653,123.444428704149));
#77156=CARTESIAN_POINT('',(7.35570217511657,821.544643257089,121.981221677081));
#77157=CARTESIAN_POINT('',(7.35570218782278,824.469104646284,113.706797746516));
#77158=CARTESIAN_POINT('',(8.29686605548008,819.569305340243,121.279896954726));
#77159=CARTESIAN_POINT('Ctrl Pts',(7.35570217511549,821.544643257128,121.981221676971));
#77160=CARTESIAN_POINT('Ctrl Pts',(7.29157612797449,821.544446918859,121.981777191364));
#77161=CARTESIAN_POINT('Ctrl Pts',(7.22741742029148,821.539601725858,121.98078819253));
#77162=CARTESIAN_POINT('Ctrl Pts',(7.00817618497621,821.506843259943,121.972029984534));
#77163=CARTESIAN_POINT('Ctrl Pts',(6.85844003671936,821.456104950426,121.956645499649));
#77164=CARTESIAN_POINT('Ctrl Pts',(6.57800953149111,821.300430451649,121.907461662577));
#77165=CARTESIAN_POINT('Ctrl Pts',(6.45179975430232,821.193933376551,121.873078839447));
#77166=CARTESIAN_POINT('Ctrl Pts',(6.25083050590953,820.941401715186,121.789800609862));
#77167=CARTESIAN_POINT('Ctrl Pts',(6.17781532595884,820.798026636983,121.741774003968));
#77168=CARTESIAN_POINT('Ctrl Pts',(6.09502776641756,820.494336758009,121.638130209503));
#77169=CARTESIAN_POINT('Ctrl Pts',(6.08561712325453,820.337099187181,121.583566550156));
#77170=CARTESIAN_POINT('Ctrl Pts',(6.10858526548658,820.182937134755,121.529080464625));
#77171=CARTESIAN_POINT('Ctrl Pts',(6.11698576023683,820.126553057236,121.509152423826));
#77172=CARTESIAN_POINT('Ctrl Pts',(6.12967679595621,820.070853662776,121.489333661784));
#77173=CARTESIAN_POINT('Ctrl Pts',(6.19231426060091,819.868343639213,121.416787447873));
#77174=CARTESIAN_POINT('Ctrl Pts',(6.26825886848808,819.730545130996,121.366419542425));
#77175=CARTESIAN_POINT('Ctrl Pts',(6.47158953473939,819.491004532206,121.277106324189));
#77176=CARTESIAN_POINT('Ctrl Pts',(6.59684555926346,819.39137691102,121.238969015809));
#77177=CARTESIAN_POINT('Ctrl Pts',(6.88242831524046,819.242053050402,121.180059885164));
#77178=CARTESIAN_POINT('Ctrl Pts',(7.04034827026691,819.194292827357,121.160042631143));
#77179=CARTESIAN_POINT('Ctrl Pts',(7.35739219623943,819.15962821654,121.142472092751));
#77180=CARTESIAN_POINT('Ctrl Pts',(7.51318586672746,819.169560072011,121.143805503151));
#77181=CARTESIAN_POINT('Ctrl Pts',(7.81109022220729,819.241308136301,121.165972241978));
#77182=CARTESIAN_POINT('Ctrl Pts',(7.950910428069,819.301729885915,121.186320176895));
#77183=CARTESIAN_POINT('Ctrl Pts',(8.15720263191499,819.437602376076,121.233482862095));
#77184=CARTESIAN_POINT('Ctrl Pts',(8.23132230216756,819.499798858129,121.255331012136));
#77185=CARTESIAN_POINT('Ctrl Pts',(8.29686605547942,819.569305340243,121.279896954726));
#77186=CARTESIAN_POINT('',(8.02990363716613,821.361155717694,121.91319750689));
#77187=CARTESIAN_POINT('Origin',(7.355702187823,820.35825874172,121.558739781714));
#77188=CARTESIAN_POINT('Ctrl Pts',(8.02990363716613,821.361155717694,121.91319750689));
#77189=CARTESIAN_POINT('Ctrl Pts',(7.90323658112111,821.43685245227,121.939951294153));
#77190=CARTESIAN_POINT('Ctrl Pts',(7.76319673633093,821.490538065063,121.959241491818));
#77191=CARTESIAN_POINT('Ctrl Pts',(7.53050212542476,821.536536404112,121.976836420245));
#77192=CARTESIAN_POINT('Ctrl Pts',(7.44313250309093,821.544910947404,121.980464281065));
#77193=CARTESIAN_POINT('Ctrl Pts',(7.35570217511549,821.544643257128,121.981221676971));
#77194=CARTESIAN_POINT('Origin',(7.35570218782278,823.281723069322,113.287136921158));
#77195=CARTESIAN_POINT('',(7.35570218782278,821.618306437815,119.494032164646));
#77196=CARTESIAN_POINT('Origin',(7.35570218782278,821.146884207207,119.327415597379));
#77197=CARTESIAN_POINT('',(7.35570218782278,820.163214703262,123.611045271416));
#77198=CARTESIAN_POINT('',(7.35570218782278,823.75314529993,113.453753488425));
#77199=CARTESIAN_POINT('Origin',(7.35570218782278,819.691792472653,123.444428704149));
#77200=CARTESIAN_POINT('Origin',(43.9674299595719,839.250508145456,118.931045884415));
#77201=CARTESIAN_POINT('',(43.9674299595719,836.658939967914,129.441192726762));
#77202=CARTESIAN_POINT('Origin',(43.9674299595719,835.660577548787,129.088337667406));
#77203=CARTESIAN_POINT('',(43.9674299595719,837.325406236982,127.555503804327));
#77204=CARTESIAN_POINT('',(43.9674299595719,840.248870564583,119.283900943771));
#77205=CARTESIAN_POINT('Origin',(43.9674299595719,836.327043817855,127.202648744971));
#77206=CARTESIAN_POINT('Origin',(43.9674299595719,839.250508145456,118.931045884415));
#77207=CARTESIAN_POINT('',(43.9674299595719,837.587091513949,125.137941127903));
#77208=CARTESIAN_POINT('Origin',(43.9674299595719,837.11566928334,124.971324560636));
#77209=CARTESIAN_POINT('',(43.9674299595719,836.131999779396,129.254954234673));
#77210=CARTESIAN_POINT('',(43.9674299595719,839.721930376064,119.097662451682));
#77211=CARTESIAN_POINT('Origin',(43.9674299595719,835.660577548787,129.088337667406));
#77212=CARTESIAN_POINT('Origin',(40.214310691231,840.998712507863,119.548920458063));
#77213=CARTESIAN_POINT('',(40.214310691231,838.630551190577,130.138026843985));
#77214=CARTESIAN_POINT('Origin',(40.214310691231,837.408781911194,129.706212241054));
#77215=CARTESIAN_POINT('',(40.214310691231,839.297017459645,128.25233792155));
#77216=CARTESIAN_POINT('',(40.214310691231,842.220481787245,119.980735060994));
#77217=CARTESIAN_POINT('Origin',(40.214310691231,838.075248180263,127.820523318619));
#77218=CARTESIAN_POINT('Origin',(40.214310691231,840.998712507863,119.548920458063));
#77219=CARTESIAN_POINT('',(40.214310691231,839.335295876356,125.755815701551));
#77220=CARTESIAN_POINT('Origin',(40.214310691231,838.863873645748,125.589199134284));
#77221=CARTESIAN_POINT('',(40.214310691231,837.880204141803,129.872828808321));
#77222=CARTESIAN_POINT('',(40.214310691231,841.470134738472,119.71553702533));
#77223=CARTESIAN_POINT('Origin',(40.214310691231,837.408781911194,129.706212241054));
#77224=CARTESIAN_POINT('Origin',(35.6828113863847,842.343161344673,120.024094167555));
#77225=CARTESIAN_POINT('',(35.6828113863847,840.267947150005,130.716737978724));
#77226=CARTESIAN_POINT('Origin',(35.6828113863847,838.753230748005,130.181385950546));
#77227=CARTESIAN_POINT('',(35.6828113863847,840.934413419073,128.831049056289));
#77228=CARTESIAN_POINT('',(35.6828113863847,843.857877746674,120.559446195733));
#77229=CARTESIAN_POINT('Origin',(35.6828113863847,839.419697017073,128.295697028111));
#77230=CARTESIAN_POINT('Origin',(35.6828113863847,842.343161344673,120.024094167555));
#77231=CARTESIAN_POINT('',(35.6828113863847,840.679744713167,126.230989411044));
#77232=CARTESIAN_POINT('Origin',(35.6828113863847,840.208322482558,126.064372843776));
#77233=CARTESIAN_POINT('',(35.6828113863847,839.224652978613,130.348002517814));
#77234=CARTESIAN_POINT('',(35.6828113863847,842.814583575282,120.190710734822));
#77235=CARTESIAN_POINT('Origin',(35.6828113863847,838.753230748005,130.181385950546));
#77236=CARTESIAN_POINT('Origin',(30.9890575763733,842.710421647777,120.153896385235));
#77237=CARTESIAN_POINT('',(30.9890575763733,840.844103195556,130.920371019949));
#77238=CARTESIAN_POINT('Origin',(30.9890575763733,839.120491051109,130.311188168227));
#77239=CARTESIAN_POINT('',(30.9890575763733,841.510569464624,129.034682097514));
#77240=CARTESIAN_POINT('',(30.9890575763733,844.434033792224,120.763079236958));
#77241=CARTESIAN_POINT('Origin',(30.9890575763733,839.786957320177,128.425499245791));
#77242=CARTESIAN_POINT('Origin',(30.9890575763733,842.710421647777,120.153896385235));
#77243=CARTESIAN_POINT('',(30.9890575763733,841.047005016271,126.360791628724));
#77244=CARTESIAN_POINT('Origin',(30.9890575763733,840.575582785662,126.194175061457));
#77245=CARTESIAN_POINT('',(30.9890575763733,839.591913281718,130.477804735494));
#77246=CARTESIAN_POINT('',(30.9890575763733,843.181843878386,120.320512952502));
#77247=CARTESIAN_POINT('Origin',(30.9890575763733,839.120491051109,130.311188168227));
#77248=CARTESIAN_POINT('Origin',(25.8715207859182,842.519925169434,120.086568484179));
#77249=CARTESIAN_POINT('',(25.8715207859182,840.682193970327,130.863146821418));
#77250=CARTESIAN_POINT('Origin',(25.8715207859182,838.929994572766,130.243860267171));
#77251=CARTESIAN_POINT('',(25.8715207859182,841.348660239395,128.977457898982));
#77252=CARTESIAN_POINT('',(25.8715207859182,844.272124566995,120.705855038426));
#77253=CARTESIAN_POINT('Origin',(25.8715207859182,839.596460841834,128.358171344736));
#77254=CARTESIAN_POINT('Origin',(25.8715207859182,842.519925169434,120.086568484179));
#77255=CARTESIAN_POINT('',(25.8715207859182,840.856508537928,126.293463727668));
#77256=CARTESIAN_POINT('Origin',(25.8715207859182,840.385086307319,126.126847160401));
#77257=CARTESIAN_POINT('',(25.8715207859182,839.401416803374,130.410476834438));
#77258=CARTESIAN_POINT('',(25.8715207859182,842.991347400043,120.253185051446));
#77259=CARTESIAN_POINT('Origin',(25.8715207859182,838.929994572766,130.243860267171));
#77260=CARTESIAN_POINT('Origin',(21.3286658472151,841.179932470295,119.612969724517));
#77261=CARTESIAN_POINT('',(21.3286658472151,839.299244222006,130.374365587087));
#77262=CARTESIAN_POINT('Origin',(21.3286658472151,837.590001873626,129.770261507508));
#77263=CARTESIAN_POINT('',(21.3286658472151,839.965710491075,128.488676664651));
#77264=CARTESIAN_POINT('',(21.3286658472151,842.889174818675,120.217073804095));
#77265=CARTESIAN_POINT('Origin',(21.3286658472151,838.256468142695,127.884572585073));
#77266=CARTESIAN_POINT('Origin',(21.3286658472151,841.179932470295,119.612969724517));
#77267=CARTESIAN_POINT('',(21.3286658472151,839.516515838788,125.819864968005));
#77268=CARTESIAN_POINT('Origin',(21.3286658472151,839.04509360818,125.653248400738));
#77269=CARTESIAN_POINT('',(21.3286658472151,838.061424104235,129.936878074775));
#77270=CARTESIAN_POINT('',(21.3286658472151,841.651354700903,119.779586291784));
#77271=CARTESIAN_POINT('Origin',(21.3286658472151,837.590001873626,129.770261507508));
#77272=CARTESIAN_POINT('Origin',(15.8526651729103,839.137486830379,118.891100327495));
#77273=CARTESIAN_POINT('',(15.8526651729103,837.349771383751,129.685355923985));
#77274=CARTESIAN_POINT('Origin',(15.8526651729103,835.547556233711,129.048392110486));
#77275=CARTESIAN_POINT('',(15.8526651729103,838.016237652819,127.799667001549));
#77276=CARTESIAN_POINT('',(15.8526651729103,840.93970198042,119.528064140993));
#77277=CARTESIAN_POINT('Origin',(15.8526651729103,836.214022502779,127.162703188051));
#77278=CARTESIAN_POINT('Origin',(15.8526651729103,839.137486830379,118.891100327495));
#77279=CARTESIAN_POINT('',(15.8526651729103,837.474070198873,125.097995570983));
#77280=CARTESIAN_POINT('Origin',(15.8526651729103,837.002647968264,124.931379003716));
#77281=CARTESIAN_POINT('',(15.8526651729103,836.018978464319,129.215008677753));
#77282=CARTESIAN_POINT('',(15.8526651729103,839.608909060988,119.057716894762));
#77283=CARTESIAN_POINT('Origin',(15.8526651729103,835.547556233711,129.048392110486));
#77284=CARTESIAN_POINT('Origin',(11.5374733507902,836.266670741035,117.87645678503));
#77285=CARTESIAN_POINT('',(11.5374733507902,834.137838960164,128.550150327038));
#77286=CARTESIAN_POINT('Origin',(11.5374733507902,832.676740144367,128.033748568021));
#77287=CARTESIAN_POINT('',(11.5374733507902,834.804305229233,126.664461404603));
#77288=CARTESIAN_POINT('',(11.5374733507902,837.727769556833,118.392858544047));
#77289=CARTESIAN_POINT('Origin',(11.5374733507902,833.343206413435,126.148059645586));
#77290=CARTESIAN_POINT('Origin',(11.5374733507902,836.266670741035,117.87645678503));
#77291=CARTESIAN_POINT('',(11.5374733507902,834.603254109529,124.083352028518));
#77292=CARTESIAN_POINT('Origin',(11.5374733507902,834.13183187892,123.916735461251));
#77293=CARTESIAN_POINT('',(11.5374733507902,833.148162374975,128.200365135288));
#77294=CARTESIAN_POINT('',(11.5374733507902,836.738092971644,118.043073352297));
#77295=CARTESIAN_POINT('Origin',(11.5374733507902,832.676740144367,128.033748568021));
#77296=CARTESIAN_POINT('Origin',(7.02096667504837,832.337060086534,116.487599418029));
#77297=CARTESIAN_POINT('',(7.02096667504837,829.934511066827,127.064552026378));
#77298=CARTESIAN_POINT('Origin',(7.02096667504837,828.747129489865,126.64489120102));
#77299=CARTESIAN_POINT('',(7.02096666994515,830.599004089277,125.184446176129));
#77300=CARTESIAN_POINT('',(7.02096667504837,833.524441663496,116.907260243387));
#77301=CARTESIAN_POINT('',(7.76758750653674,828.457388048144,124.421246119495));
#77302=CARTESIAN_POINT('Ctrl Pts',(7.02096666484195,830.599004089278,125.184446176129));
#77303=CARTESIAN_POINT('Ctrl Pts',(6.88754184176866,830.598428459883,125.186074849416));
#77304=CARTESIAN_POINT('Ctrl Pts',(6.75480841283368,830.577742800318,125.180967780531));
#77305=CARTESIAN_POINT('Ctrl Pts',(6.46912138942601,830.487520618593,125.154490180543));
#77306=CARTESIAN_POINT('Ctrl Pts',(6.32241100157311,830.408069098372,125.129666171615));
#77307=CARTESIAN_POINT('Ctrl Pts',(6.0705602684719,830.200410514294,125.062247605861));
#77308=CARTESIAN_POINT('Ctrl Pts',(5.9677076297661,830.074463399832,125.020380632044));
#77309=CARTESIAN_POINT('Ctrl Pts',(5.82001658048626,829.793613247126,124.924809169643));
#77310=CARTESIAN_POINT('Ctrl Pts',(5.77620821768348,829.641649517263,124.872109464138));
#77311=CARTESIAN_POINT('Ctrl Pts',(5.76467934958987,829.486353867704,124.817222727024));
#77312=CARTESIAN_POINT('Ctrl Pts',(5.76046271792157,829.42955518213,124.79714814971));
#77313=CARTESIAN_POINT('Ctrl Pts',(5.7605846570906,829.372586060989,124.776880623296));
#77314=CARTESIAN_POINT('Ctrl Pts',(5.77712940574573,829.162229321906,124.70156111462));
#77315=CARTESIAN_POINT('Ctrl Pts',(5.82091237972588,829.012566175966,124.646999844751));
#77316=CARTESIAN_POINT('Ctrl Pts',(5.96665513263313,828.738433467381,124.545460604461));
#77317=CARTESIAN_POINT('Ctrl Pts',(6.0670019011125,828.616449298384,124.499421735631));
#77318=CARTESIAN_POINT('Ctrl Pts',(6.31299086818166,828.414448303395,124.421894723324));
#77319=CARTESIAN_POINT('Ctrl Pts',(6.456710677155,828.336796500924,124.391312773727));
#77320=CARTESIAN_POINT('Ctrl Pts',(6.75881384421649,828.240776304019,124.352057095193));
#77321=CARTESIAN_POINT('Ctrl Pts',(6.91324235757128,828.219966088468,124.34252521751));
#77322=CARTESIAN_POINT('Ctrl Pts',(7.22023722497622,828.23177048709,124.343505836645));
#77323=CARTESIAN_POINT('Ctrl Pts',(7.37025616922219,828.263470062076,124.35370238321));
#77324=CARTESIAN_POINT('Ctrl Pts',(7.60194283378443,828.355940183934,124.385525202896));
#77325=CARTESIAN_POINT('Ctrl Pts',(7.68814879419479,828.402248885612,124.401758073776));
#77326=CARTESIAN_POINT('Ctrl Pts',(7.76758750653594,828.457388048145,124.421246119495));
#77327=CARTESIAN_POINT('',(7.90158939818299,830.262414407737,125.059203509569));
#77328=CARTESIAN_POINT('Origin',(7.02096667504848,829.413595758933,124.759202278584));
#77329=CARTESIAN_POINT('Ctrl Pts',(7.90158939818298,830.262414407737,125.059203509569));
#77330=CARTESIAN_POINT('Ctrl Pts',(7.79438261430018,830.361287325615,125.094148544196));
#77331=CARTESIAN_POINT('Ctrl Pts',(7.66926336415262,830.44124939494,125.122725730685));
#77332=CARTESIAN_POINT('Ctrl Pts',(7.39304844123785,830.556372454823,125.165113740543));
#77333=CARTESIAN_POINT('Ctrl Pts',(7.24393858453375,830.589920863212,125.17836147125));
#77334=CARTESIAN_POINT('Ctrl Pts',(7.06833649789207,830.598575376114,125.18365593624));
#77335=CARTESIAN_POINT('Ctrl Pts',(7.04464069952261,830.599106225221,125.184157194911));
#77336=CARTESIAN_POINT('Ctrl Pts',(7.02096666484194,830.599004089278,125.184446176129));
#77337=CARTESIAN_POINT('Origin',(7.02096667504837,832.337060086534,116.487599418029));
#77338=CARTESIAN_POINT('',(7.02096667504837,830.673643455028,122.694494661517));
#77339=CARTESIAN_POINT('Origin',(7.02096667504837,830.202221224419,122.52787809425));
#77340=CARTESIAN_POINT('',(7.02096667504837,829.218551720474,126.811507768287));
#77341=CARTESIAN_POINT('',(7.02096667504837,832.808482317143,116.654215985296));
#77342=CARTESIAN_POINT('Origin',(7.02096667504837,828.747129489865,126.64489120102));
#77343=CARTESIAN_POINT('Ctrl Pts',(17.2487640684582,778.138083759694,108.757942040107));
#77344=CARTESIAN_POINT('Ctrl Pts',(-19.6797178494731,802.718757630444,117.445583893923));
#77345=CARTESIAN_POINT('Ctrl Pts',(-6.00421854062202,843.341877796349,131.803169078188));
#77346=CARTESIAN_POINT('Ctrl Pts',(7.67128076822907,883.964997962254,146.160754262452));
#77347=CARTESIAN_POINT('Ctrl Pts',(52.875234385587,883.966642709865,146.161335571909));
#77348=CARTESIAN_POINT('Ctrl Pts',(98.0791880029448,883.968287457475,146.161916881366));
#77349=CARTESIAN_POINT('Ctrl Pts',(111.75801268726,843.346162579713,131.804683465608));
#77350=CARTESIAN_POINT('Ctrl Pts',(125.436837371576,802.72403770195,117.447450049849));
#77351=CARTESIAN_POINT('Ctrl Pts',(88.5103677421852,778.140676615915,108.758858443227));
#77352=CARTESIAN_POINT('Ctrl Pts',(21.9700649362988,785.109903755238,109.100778471584));
#77353=CARTESIAN_POINT('Ctrl Pts',(-10.0648980335876,806.433308789172,116.637191306022));
#77354=CARTESIAN_POINT('Ctrl Pts',(1.79841427173159,841.673320905785,129.092203963653));
#77355=CARTESIAN_POINT('Ctrl Pts',(13.6617265770508,876.913333022398,141.547216621283));
#77356=CARTESIAN_POINT('Ctrl Pts',(52.8755502983386,876.914759818899,141.547720899443));
#77357=CARTESIAN_POINT('Ctrl Pts',(92.0893740196265,876.9161866154,141.548225177604));
#77358=CARTESIAN_POINT('Ctrl Pts',(103.955571043578,841.677037897907,129.093517674436));
#77359=CARTESIAN_POINT('Ctrl Pts',(115.82176806753,806.437889180414,116.638810171269));
#77360=CARTESIAN_POINT('Ctrl Pts',(83.7885507309743,785.112153023248,109.101573439004));
#77361=CARTESIAN_POINT('Ctrl Pts',(26.83022759437,791.600709061904,111.394848688847));
#77362=CARTESIAN_POINT('Ctrl Pts',(-0.167289399587949,809.571043234409,
117.746172826868));
#77363=CARTESIAN_POINT('Ctrl Pts',(9.83053628444845,839.269620594397,128.242654942375));
#77364=CARTESIAN_POINT('Ctrl Pts',(19.8283619684848,868.968197954386,138.739137057882));
#77365=CARTESIAN_POINT('Ctrl Pts',(52.8758755026418,868.969400389451,138.739562039119));
#77366=CARTESIAN_POINT('Ctrl Pts',(85.9233890367988,868.970602824516,138.739987020357));
#77367=CARTESIAN_POINT('Ctrl Pts',(95.9236458221411,839.272753095536,128.243762074268));
#77368=CARTESIAN_POINT('Ctrl Pts',(105.923902607483,809.574903366556,117.74753712818));
#77369=CARTESIAN_POINT('Ctrl Pts',(78.9278567488456,791.602604636167,111.39551864893));
#77370=CARTESIAN_POINT('',(17.244803233355,778.140660313945,108.758852681557));
#77371=CARTESIAN_POINT('',(88.5104020101015,778.140638997398,108.758845147568));
#77372=CARTESIAN_POINT('Origin',(52.8776183915471,825.72084445736,125.575299673619));
#77373=CARTESIAN_POINT('Origin',(26.8353066323039,768.271008451119,177.392764388526));
#77374=CARTESIAN_POINT('Origin',(52.8776183915471,826.387310726428,123.689610751183));
#77375=CARTESIAN_POINT('Origin',(52.8776183915471,826.387310726428,123.689610751183));
#77376=CARTESIAN_POINT('Origin',(52.8776183915471,826.387310726428,123.689610751183));
#77377=CARTESIAN_POINT('Origin',(52.8776183915471,826.387310726428,123.689610751183));
#77378=CARTESIAN_POINT('Origin',(52.8776183915471,826.387310726428,123.689610751183));
#77379=CARTESIAN_POINT('Origin',(52.8776183915471,826.387310726428,123.689610751183));
#77380=CARTESIAN_POINT('Origin',(52.8776183915471,826.387310726428,123.689610751183));
#77381=CARTESIAN_POINT('Origin',(52.8776183915471,826.387310726428,123.689610751183));
#77382=CARTESIAN_POINT('Origin',(52.8776183915471,826.387310726428,123.689610751183));
#77383=CARTESIAN_POINT('Origin',(52.8776183915471,826.387310726428,123.689610751183));
#77384=CARTESIAN_POINT('Origin',(52.8776183915471,826.387310726428,123.689610751183));
#77385=CARTESIAN_POINT('Origin',(52.8776183915471,826.387310726428,123.689610751183));
#77386=CARTESIAN_POINT('Origin',(52.8776183915471,826.387310726428,123.689610751183));
#77387=CARTESIAN_POINT('Origin',(52.8776183915471,826.387310726428,123.689610751183));
#77388=CARTESIAN_POINT('Origin',(52.8776183915471,826.387310726428,123.689610751183));
#77389=CARTESIAN_POINT('Origin',(52.8776183915471,826.387310726428,123.689610751183));
#77390=CARTESIAN_POINT('Origin',(52.8776183915471,826.387310726428,123.689610751183));
#77391=CARTESIAN_POINT('Origin',(52.8776183915471,826.387310726428,123.689610751183));
#77392=CARTESIAN_POINT('Origin',(52.8776183915471,826.387310726428,123.689610751183));
#77393=CARTESIAN_POINT('Origin',(52.8776183915471,826.387310726428,123.689610751183));
#77394=CARTESIAN_POINT('Origin',(52.8776183915471,826.387310726428,123.689610751183));
#77395=CARTESIAN_POINT('Origin',(52.8776183915471,826.387310726428,123.689610751183));
#77396=CARTESIAN_POINT('Origin',(52.8776183915471,826.387310726428,123.689610751183));
#77397=CARTESIAN_POINT('Origin',(52.8776183915471,826.387310726428,123.689610751183));
#77398=CARTESIAN_POINT('',(78.9278568228492,791.602604685434,111.395518666343));
#77399=CARTESIAN_POINT('Origin',(52.8776183915471,826.387310726428,123.689610751183));
#77400=CARTESIAN_POINT('Origin',(78.9278568223621,768.27628526772,177.394630951443));
#77401=CARTESIAN_POINT('',(3.61051440984461,833.840239926159,126.494338492581));
#77402=CARTESIAN_POINT('',(3.61051441020205,835.757685720563,127.199440688052));
#77403=CARTESIAN_POINT('Ctrl Pts',(3.61051440984449,833.840239926159,126.494338492581));
#77404=CARTESIAN_POINT('Ctrl Pts',(3.55313771416574,833.838958115137,126.497965228091));
#77405=CARTESIAN_POINT('Ctrl Pts',(3.49573635195613,833.842193256988,126.503319790014));
#77406=CARTESIAN_POINT('Ctrl Pts',(3.30520855208768,833.868273506038,126.526964401137));
#77407=CARTESIAN_POINT('Ctrl Pts',(3.17736063026302,833.911378108521,126.552640578553));
#77408=CARTESIAN_POINT('Ctrl Pts',(2.94960675592224,834.041491045101,126.618638538412));
#77409=CARTESIAN_POINT('Ctrl Pts',(2.85158409278753,834.126777814448,126.658162113752));
#77410=CARTESIAN_POINT('Ctrl Pts',(2.6974110396019,834.328833530119,126.745719811672));
#77411=CARTESIAN_POINT('Ctrl Pts',(2.64270068035171,834.443611592352,126.792888318793));
#77412=CARTESIAN_POINT('Ctrl Pts',(2.59881997156012,834.627261138451,126.864661375413));
#77413=CARTESIAN_POINT('Ctrl Pts',(2.59071064179276,834.690196650513,126.888671386677));
#77414=CARTESIAN_POINT('Ctrl Pts',(2.58791622229759,834.817756032106,126.936151111776));
#77415=CARTESIAN_POINT('Ctrl Pts',(2.59339322055599,834.882059819712,126.959488083182));
#77416=CARTESIAN_POINT('Ctrl Pts',(2.60567260254573,834.945556746391,126.981930045542));
#77417=CARTESIAN_POINT('Ctrl Pts',(2.62956184569571,835.069088494322,127.025590345062));
#77418=CARTESIAN_POINT('Ctrl Pts',(2.67883925702017,835.187724180532,127.065203300552));
#77419=CARTESIAN_POINT('Ctrl Pts',(2.82255402142357,835.401816423126,127.132019117587));
#77420=CARTESIAN_POINT('Ctrl Pts',(2.91559073162443,835.495181789821,127.158575017672));
#77421=CARTESIAN_POINT('Ctrl Pts',(3.13391416585918,835.644350256091,127.195443722542));
#77422=CARTESIAN_POINT('Ctrl Pts',(3.25724404832662,835.698551579164,127.20533847109));
#77423=CARTESIAN_POINT('Ctrl Pts',(3.46087175387042,835.746353580736,127.206816337373));
#77424=CARTESIAN_POINT('Ctrl Pts',(3.53566947643406,835.755896971539,127.204501745718));
#77425=CARTESIAN_POINT('Ctrl Pts',(3.61051441020204,835.757685720563,127.199440688052));
#77426=CARTESIAN_POINT('Ctrl Pts',(3.61051441020204,835.757685720563,127.199440688052));
#77427=CARTESIAN_POINT('Ctrl Pts',(3.66908123832854,835.759085432626,127.195480365296));
#77428=CARTESIAN_POINT('Ctrl Pts',(3.72767695938084,835.755737011247,127.18983816472));
#77429=CARTESIAN_POINT('Ctrl Pts',(3.9178418146544,835.729076184011,127.165953427404));
#77430=CARTESIAN_POINT('Ctrl Pts',(4.04425758411047,835.686040761199,127.141154082189));
#77431=CARTESIAN_POINT('Ctrl Pts',(4.26994430756122,835.556469380439,127.078149835135));
#77432=CARTESIAN_POINT('Ctrl Pts',(4.36731125541824,835.471583502163,127.040668047308));
#77433=CARTESIAN_POINT('Ctrl Pts',(4.52209435269776,835.269301288954,126.956770266859));
#77434=CARTESIAN_POINT('Ctrl Pts',(4.57745399047076,835.153507816833,126.911067195361));
#77435=CARTESIAN_POINT('Ctrl Pts',(4.6366816470894,834.907180994579,126.817516065391));
#77436=CARTESIAN_POINT('Ctrl Pts',(4.63987650281397,834.779083509209,126.770590605619));
#77437=CARTESIAN_POINT('Ctrl Pts',(4.59320506619355,834.529395965551,126.682246407946));
#77438=CARTESIAN_POINT('Ctrl Pts',(4.54432105488512,834.410196679952,126.6416420912));
#77439=CARTESIAN_POINT('Ctrl Pts',(4.40087906004098,834.195441023357,126.571921209333));
#77440=CARTESIAN_POINT('Ctrl Pts',(4.30775633773022,834.101960639812,126.543482977807));
#77441=CARTESIAN_POINT('Ctrl Pts',(4.08966906260932,833.953395096546,126.503050947673));
#77442=CARTESIAN_POINT('Ctrl Pts',(3.96691783599692,833.899611590578,126.491400668772));
#77443=CARTESIAN_POINT('Ctrl Pts',(3.76264653461912,833.851582931137,126.487758649126));
#77444=CARTESIAN_POINT('Ctrl Pts',(3.68660214370276,833.841939746873,126.489529047161));
#77445=CARTESIAN_POINT('Ctrl Pts',(3.61051440984449,833.840239926159,126.494338492581));
#77446=CARTESIAN_POINT('Origin',(52.8776183915471,825.82081439772,125.292446335253));
#77447=CARTESIAN_POINT('',(89.6658953216452,777.849661941175,108.656004010442));
#77448=CARTESIAN_POINT('',(16.0893414616814,777.849661941191,108.656004010448));
#77449=CARTESIAN_POINT('Origin',(52.8776183915471,825.72084445736,125.575299673619));
#77450=CARTESIAN_POINT('',(89.8419123794813,777.72172974858,108.288790430857));
#77451=CARTESIAN_POINT('Origin',(89.6658475858845,777.949599270907,108.373139155083));
#77452=CARTESIAN_POINT('',(90.0889201803354,777.892818101182,108.344695672232));
#77453=CARTESIAN_POINT('Ctrl Pts',(89.8419355198187,777.722828038471,108.285587078659));
#77454=CARTESIAN_POINT('Ctrl Pts',(89.9244204729452,777.77927806364,108.305192971918));
#77455=CARTESIAN_POINT('Ctrl Pts',(90.0067649765183,777.835914159845,108.324880126932));
#77456=CARTESIAN_POINT('Ctrl Pts',(90.0889691576735,777.892731478081,108.344662072744));
#77457=CARTESIAN_POINT('',(93.6680441109739,780.557861377815,109.278881970676));
#77458=CARTESIAN_POINT('Ctrl Pts',(90.0889201803354,777.892818101182,108.344695672232));
#77459=CARTESIAN_POINT('Ctrl Pts',(91.3154631687481,778.7366822112,108.651320889096));
#77460=CARTESIAN_POINT('Ctrl Pts',(92.5094987365803,779.625048288525,108.965299465377));
#77461=CARTESIAN_POINT('Ctrl Pts',(93.667901465805,780.558016866062,109.278945885626));
#77462=CARTESIAN_POINT('',(52.8776183915471,885.221162372646,146.286427926904));
#77463=CARTESIAN_POINT('Ctrl Pts',(93.6680441109739,780.557861377815,109.278881970676));
#77464=CARTESIAN_POINT('Ctrl Pts',(94.197024709261,780.980338314738,109.431683914032));
#77465=CARTESIAN_POINT('Ctrl Pts',(94.7185981290245,781.41128110683,109.586717706928));
#77466=CARTESIAN_POINT('Ctrl Pts',(95.2324518299379,781.850431742364,109.744058725421));
#77467=CARTESIAN_POINT('Ctrl Pts',(95.8193315364788,782.351992002905,109.923760166893));
#77468=CARTESIAN_POINT('Ctrl Pts',(96.3961413415951,782.864258158874,110.106471169126));
#77469=CARTESIAN_POINT('Ctrl Pts',(96.9624586130382,783.386794371866,110.292284981594));
#77470=CARTESIAN_POINT('Ctrl Pts',(97.6184571070962,783.992078699396,110.507524013319));
#77471=CARTESIAN_POINT('Ctrl Pts',(98.2603768782123,784.611142413407,110.726926031512));
#77472=CARTESIAN_POINT('Ctrl Pts',(98.8876154581229,785.243257192534,110.950615259769));
#77473=CARTESIAN_POINT('Ctrl Pts',(99.4301896715193,785.790049418086,111.144111021914));
#77474=CARTESIAN_POINT('Ctrl Pts',(99.9617797418856,786.346606065637,111.340814223757));
#77475=CARTESIAN_POINT('Ctrl Pts',(100.482019891401,786.912438172296,111.540798435659));
#77476=CARTESIAN_POINT('Ctrl Pts',(101.131349594451,787.618672772097,111.790405639273));
#77477=CARTESIAN_POINT('Ctrl Pts',(101.762996785547,788.339359682015,112.04512077829));
#77478=CARTESIAN_POINT('Ctrl Pts',(102.376257962256,789.073696230874,112.304660161555));
#77479=CARTESIAN_POINT('Ctrl Pts',(102.989518339807,789.808031822797,112.564199206606));
#77480=CARTESIAN_POINT('Ctrl Pts',(103.584392649411,790.556016896556,112.82856244038));
#77481=CARTESIAN_POINT('Ctrl Pts',(104.160218346474,791.316818379583,113.097455426844));
#77482=CARTESIAN_POINT('Ctrl Pts',(104.736043308847,792.077618891913,113.36634807023));
#77483=CARTESIAN_POINT('Ctrl Pts',(105.292819612004,792.851235654898,113.639770410246));
#77484=CARTESIAN_POINT('Ctrl Pts',(105.829927144797,793.63680705073,113.917417922006));
#77485=CARTESIAN_POINT('Ctrl Pts',(106.367034006896,794.422377465605,114.195065087063));
#77486=CARTESIAN_POINT('Ctrl Pts',(106.884472058878,795.219902353467,114.476937367362));
#77487=CARTESIAN_POINT('Ctrl Pts',(107.381665004123,796.028493470983,114.762720827657));
#77488=CARTESIAN_POINT('Ctrl Pts',(107.878857342036,796.837083600788,115.048503938861));
#77489=CARTESIAN_POINT('Ctrl Pts',(108.355804540403,797.656739799398,115.338198173211));
#77490=CARTESIAN_POINT('Ctrl Pts',(108.811975400586,798.486549176966,115.631480884545));
#77491=CARTESIAN_POINT('Ctrl Pts',(109.268145715963,799.31635756349,115.924763245612));
#77492=CARTESIAN_POINT('Ctrl Pts',(109.703539667303,800.156318967395,116.221634026556));
#77493=CARTESIAN_POINT('Ctrl Pts',(110.117672336942,801.0054978862,116.521762589149));
#77494=CARTESIAN_POINT('Ctrl Pts',(110.531804523245,801.854675813923,116.82189080146));
#77495=CARTESIAN_POINT('Ctrl Pts',(110.924675408953,802.713071094501,117.125276738147));
#77496=CARTESIAN_POINT('Ctrl Pts',(111.295847437258,803.579727697054,117.431582505548));
#77497=CARTESIAN_POINT('Ctrl Pts',(111.667019042458,804.446383311692,117.737887923787));
#77498=CARTESIAN_POINT('Ctrl Pts',(112.016491778313,805.321300086051,118.047113115394));
#77499=CARTESIAN_POINT('Ctrl Pts',(112.343876423242,806.203503590788,118.35891368407));
#77500=CARTESIAN_POINT('Ctrl Pts',(112.671260703895,807.08570611391,118.67071390581));
#77501=CARTESIAN_POINT('Ctrl Pts',(112.97655688861,807.975195205204,118.985089447289));
#77502=CARTESIAN_POINT('Ctrl Pts',(113.259424957734,808.870980207768,119.301690176839));
#77503=CARTESIAN_POINT('Ctrl Pts',(113.54229271982,809.766764238006,119.618290562735));
#77504=CARTESIAN_POINT('Ctrl Pts',(113.802732368204,810.668844017608,119.937116079479));
#77505=CARTESIAN_POINT('Ctrl Pts',(114.040453842246,811.576214869137,120.25781164007));
#77506=CARTESIAN_POINT('Ctrl Pts',(114.27817506469,812.483584760335,120.578506861247));
#77507=CARTESIAN_POINT('Ctrl Pts',(114.493178121551,813.396245562106,120.901072069243));
#77508=CARTESIAN_POINT('Ctrl Pts',(114.685223556998,814.313180814713,121.225148012794));
#77509=CARTESIAN_POINT('Ctrl Pts',(114.87726879443,815.230115121885,121.549223622197));
#77510=CARTESIAN_POINT('Ctrl Pts',(115.046356426019,816.151323719344,121.874809910411));
#77511=CARTESIAN_POINT('Ctrl Pts',(115.19229813381,817.075780629512,122.201544262246));
#77512=CARTESIAN_POINT('Ctrl Pts',(115.3382396951,818.000236611673,122.528278286091));
#77513=CARTESIAN_POINT('Ctrl Pts',(115.46103535492,818.927940747042,122.856160317185));
#77514=CARTESIAN_POINT('Ctrl Pts',(115.560548352345,819.857859825842,123.184825184231));
#77515=CARTESIAN_POINT('Ctrl Pts',(115.660061252576,820.78777799639,123.513489730271));
#77516=CARTESIAN_POINT('Ctrl Pts',(115.736291519433,821.71991095216,123.842937056347));
#77517=CARTESIAN_POINT('Ctrl Pts',(115.789154253324,822.6532205529,124.172800248569));
#77518=CARTESIAN_POINT('Ctrl Pts',(115.842016937023,823.586529267472,124.502663127588));
#77519=CARTESIAN_POINT('Ctrl Pts',(115.87151212339,824.521014470338,124.832941817379));
#77520=CARTESIAN_POINT('Ctrl Pts',(115.877606962946,825.455635403465,125.163268478836));
#77521=CARTESIAN_POINT('Ctrl Pts',(115.883969825378,826.431356645674,125.508121380186));
#77522=CARTESIAN_POINT('Ctrl Pts',(115.864828583856,827.407225640495,125.853026502308));
#77523=CARTESIAN_POINT('Ctrl Pts',(115.820206471894,828.382057884472,126.197565201603));
#77524=CARTESIAN_POINT('Ctrl Pts',(115.776978800931,829.326426620824,126.531337066545));
#77525=CARTESIAN_POINT('Ctrl Pts',(115.709838235661,830.269822231259,126.864764995862));
#77526=CARTESIAN_POINT('Ctrl Pts',(115.61886125874,831.211170053946,127.197469167699));
#77527=CARTESIAN_POINT('Ctrl Pts',(115.528902022302,832.141987214704,127.526451447297));
#77528=CARTESIAN_POINT('Ctrl Pts',(115.415636810722,833.070801999554,127.854726019497));
#77529=CARTESIAN_POINT('Ctrl Pts',(115.279191779543,833.996579888444,128.181927249908));
#77530=CARTESIAN_POINT('Ctrl Pts',(115.142747206403,834.922354669536,128.509127381919));
#77531=CARTESIAN_POINT('Ctrl Pts',(114.983122991902,835.845092421845,128.835254125198));
#77532=CARTESIAN_POINT('Ctrl Pts',(114.800496925351,836.763765400855,129.159944240057));
#77533=CARTESIAN_POINT('Ctrl Pts',(114.617871451988,837.682435395922,129.48463330029));
#77534=CARTESIAN_POINT('Ctrl Pts',(114.412244306252,838.597040492061,129.807885687703));
#77535=CARTESIAN_POINT('Ctrl Pts',(114.183844513994,839.506562009519,130.129341366402));
#77536=CARTESIAN_POINT('Ctrl Pts',(113.955445438748,840.416080671732,130.450796035962));
#77537=CARTESIAN_POINT('Ctrl Pts',(113.704273897785,841.320515636666,130.770453954891));
#77538=CARTESIAN_POINT('Ctrl Pts',(113.430609642179,842.218859558297,131.087959093022));
#77539=CARTESIAN_POINT('Ctrl Pts',(113.1569462159,843.117200757535,131.405463268968));
#77540=CARTESIAN_POINT('Ctrl Pts',(112.86079025662,844.009450801726,131.720814624619));
#77541=CARTESIAN_POINT('Ctrl Pts',(112.54247161638,844.894615922248,132.033661928523));
#77542=CARTESIAN_POINT('Ctrl Pts',(112.224153906152,845.779778456638,132.346508318399));
#77543=CARTESIAN_POINT('Ctrl Pts',(111.883673697169,846.657855962279,132.656850619388));
#77544=CARTESIAN_POINT('Ctrl Pts',(111.52141020664,847.527870461329,132.964343181029));
#77545=CARTESIAN_POINT('Ctrl Pts',(111.159147735086,848.397882513203,133.271834877755));
#77546=CARTESIAN_POINT('Ctrl Pts',(110.775102164503,849.259831459875,133.57647680028));
#77547=CARTESIAN_POINT('Ctrl Pts',(110.369701231559,850.112757292431,133.877929648973));
#77548=CARTESIAN_POINT('Ctrl Pts',(109.96430139481,850.965680818696,134.179381682544));
#77549=CARTESIAN_POINT('Ctrl Pts',(109.5375463783,851.809581138503,134.477644609644));
#77550=CARTESIAN_POINT('Ctrl Pts',(109.08991148443,852.643518349956,134.772386237143));
#77551=CARTESIAN_POINT('Ctrl Pts',(108.642277752234,853.477453397227,135.067127099746));
#77552=CARTESIAN_POINT('Ctrl Pts',(108.173764325148,854.30142524986,135.358346632251));
#77553=CARTESIAN_POINT('Ctrl Pts',(107.684893011688,855.114516206239,135.645720487856));
#77554=CARTESIAN_POINT('Ctrl Pts',(107.196022913727,855.927605140998,135.933093628952));
#77555=CARTESIAN_POINT('Ctrl Pts',(106.686795111545,856.729813099066,136.216621064718));
#77556=CARTESIAN_POINT('Ctrl Pts',(106.157776756618,857.520246622884,136.495987017022));
#77557=CARTESIAN_POINT('Ctrl Pts',(105.628759659444,858.310678267429,136.775352305128));
#77558=CARTESIAN_POINT('Ctrl Pts',(105.079952191192,859.089335402919,137.050556083333));
#77559=CARTESIAN_POINT('Ctrl Pts',(104.511965582211,859.855350805601,137.321291845419));
#77560=CARTESIAN_POINT('Ctrl Pts',(103.943980261838,860.621364470401,137.59202699328));
#77561=CARTESIAN_POINT('Ctrl Pts',(103.356815981767,861.374736333003,137.858294100498));
#77562=CARTESIAN_POINT('Ctrl Pts',(102.751126689003,862.114627334749,138.119796615353));
#77563=CARTESIAN_POINT('Ctrl Pts',(102.145438704458,862.854516738416,138.381298565393));
#77564=CARTESIAN_POINT('Ctrl Pts',(101.521225887489,863.580925217035,138.638035900382));
#77565=CARTESIAN_POINT('Ctrl Pts',(100.87918344445,864.293043745578,138.889722683502));
#77566=CARTESIAN_POINT('Ctrl Pts',(100.237142318287,865.005160813513,139.141408950394));
#77567=CARTESIAN_POINT('Ctrl Pts',(99.5772717454529,865.702987872164,139.388044644489));
#77568=CARTESIAN_POINT('Ctrl Pts',(98.9003066425044,866.385747731757,139.629355080627));
#77569=CARTESIAN_POINT('Ctrl Pts',(98.2233428544031,867.068506265249,139.870665048076));
#77570=CARTESIAN_POINT('Ctrl Pts',(97.5292847146265,867.736197545241,140.106649738324));
#77571=CARTESIAN_POINT('Ctrl Pts',(96.8189052123928,868.388077947923,140.337046329557));
#77572=CARTESIAN_POINT('Ctrl Pts',(96.0929140815661,869.054284375921,140.57250622287));
#77573=CARTESIAN_POINT('Ctrl Pts',(95.3498763203634,869.703977103575,140.802129615725));
#77574=CARTESIAN_POINT('Ctrl Pts',(94.5906562273834,870.336400410859,141.025649411097));
#77575=CARTESIAN_POINT('Ctrl Pts',(93.8477364929531,870.955245670409,141.244370264975));
#77576=CARTESIAN_POINT('Ctrl Pts',(93.089322087264,871.557555123933,141.4572468055));
#77577=CARTESIAN_POINT('Ctrl Pts',(92.3162577333526,872.142657918312,141.664041930481));
#77578=CARTESIAN_POINT('Ctrl Pts',(91.5431983690533,872.727756936244,141.870835720739));
#77579=CARTESIAN_POINT('Ctrl Pts',(90.7554893736169,873.295649420353,142.071548139746));
#77580=CARTESIAN_POINT('Ctrl Pts',(89.9540080871138,873.845702859351,142.265955636611));
#77581=CARTESIAN_POINT('Ctrl Pts',(89.1525316247205,874.395752987581,142.460361963339));
#77582=CARTESIAN_POINT('Ctrl Pts',(88.3372831697205,874.927964194455,142.648463411664));
#77583=CARTESIAN_POINT('Ctrl Pts',(87.5091707243506,875.441743717161,142.830050479154));
#77584=CARTESIAN_POINT('Ctrl Pts',(86.681062902896,875.955520371087,143.011636532719));
#77585=CARTESIAN_POINT('Ctrl Pts',(85.8400913717978,876.450865461692,143.186708248159));
#77586=CARTESIAN_POINT('Ctrl Pts',(84.9871927725203,876.927227292831,143.355070637389));
#77587=CARTESIAN_POINT('Ctrl Pts',(84.1342985643052,877.403586671469,143.523432159822));
#77588=CARTESIAN_POINT('Ctrl Pts',(83.269477551886,877.860962907313,143.685084397281));
#77589=CARTESIAN_POINT('Ctrl Pts',(82.3936929294395,878.2988465977,143.839847309629));
#77590=CARTESIAN_POINT('Ctrl Pts',(81.5179124346959,878.736728224277,143.994609492556));
#77591=CARTESIAN_POINT('Ctrl Pts',(80.6311685782169,879.15511741671,144.142482389715));
#77592=CARTESIAN_POINT('Ctrl Pts',(79.7344489614346,879.553548198539,144.283301309255));
#77593=CARTESIAN_POINT('Ctrl Pts',(78.8377331806933,879.951977275936,144.424119626392));
#77594=CARTESIAN_POINT('Ctrl Pts',(77.9310418734027,880.330448047585,144.557884002972));
#77595=CARTESIAN_POINT('Ctrl Pts',(77.0153848486169,880.688538999341,144.684445461633));
#77596=CARTESIAN_POINT('Ctrl Pts',(76.0620139019287,881.061378938789,144.816219711588));
#77597=CARTESIAN_POINT('Ctrl Pts',(75.0989234943549,881.412125271284,144.940185333291));
#77598=CARTESIAN_POINT('Ctrl Pts',(74.1272763932478,881.740354530471,145.056192659402));
#77599=CARTESIAN_POINT('Ctrl Pts',(73.1940407178224,882.055608138538,145.167613951365));
#77600=CARTESIAN_POINT('Ctrl Pts',(72.2529117951107,882.350090054414,145.271693824481));
#77601=CARTESIAN_POINT('Ctrl Pts',(71.3049378455667,882.623472286938,145.368316355574));
#77602=CARTESIAN_POINT('Ctrl Pts',(70.3569750989512,882.896851288697,145.464937744805));
#77603=CARTESIAN_POINT('Ctrl Pts',(69.4021676441985,883.149131060654,145.554101952314));
#77604=CARTESIAN_POINT('Ctrl Pts',(68.441578911655,883.380030622634,145.6357096702));
#77605=CARTESIAN_POINT('Ctrl Pts',(67.4809998585701,883.610927857934,145.717316565758));
#77606=CARTESIAN_POINT('Ctrl Pts',(66.514639803188,883.820445276004,145.791367110503));
#77607=CARTESIAN_POINT('Ctrl Pts',(65.5435750210444,884.00834952855,145.857778831252));
#77608=CARTESIAN_POINT('Ctrl Pts',(64.5799300420301,884.194818024608,145.923683107079));
#77609=CARTESIAN_POINT('Ctrl Pts',(63.6116521277509,884.360002410964,145.98206485837));
#77610=CARTESIAN_POINT('Ctrl Pts',(62.6398032780485,884.503721514643,146.032860052468));
#77611=CARTESIAN_POINT('Ctrl Pts',(61.6632079549134,884.648142537049,146.083903328394));
#77612=CARTESIAN_POINT('Ctrl Pts',(60.6830046352858,884.770888340889,146.127285848679));
#77613=CARTESIAN_POINT('Ctrl Pts',(59.7002803969362,884.871822593871,146.162959428879));
#77614=CARTESIAN_POINT('Ctrl Pts',(58.7171808562614,884.972795393638,146.198646632816));
#77615=CARTESIAN_POINT('Ctrl Pts',(57.7315589965718,885.051939905625,146.226618981274));
#77616=CARTESIAN_POINT('Ctrl Pts',(56.7445099147395,885.109168319521,146.246845439117));
#77617=CARTESIAN_POINT('Ctrl Pts',(55.7574501536532,885.166397352592,146.267072115797));
#77618=CARTESIAN_POINT('Ctrl Pts',(54.768963305234,885.201709803786,146.279552730875));
#77619=CARTESIAN_POINT('Ctrl Pts',(53.7801476712614,885.215066915775,146.284273586201));
#77620=CARTESIAN_POINT('Ctrl Pts',(53.4793246798471,885.219130490669,146.285709791063));
#77621=CARTESIAN_POINT('Ctrl Pts',(53.1784712709463,885.221162372646,146.286427926904));
#77622=CARTESIAN_POINT('Ctrl Pts',(52.8776183915471,885.221162372646,146.286427926904));
#77623=CARTESIAN_POINT('',(12.0877107975547,780.556697717533,109.280534704239));
#77624=CARTESIAN_POINT('Ctrl Pts',(52.8776183915471,885.221162372646,146.286427926904));
#77625=CARTESIAN_POINT('Ctrl Pts',(51.8886967717354,885.221162372646,146.286427926904));
#77626=CARTESIAN_POINT('Ctrl Pts',(50.8997695057188,885.199204645394,146.278667323135));
#77627=CARTESIAN_POINT('Ctrl Pts',(49.9119353918395,885.155313002713,146.263154531501));
#77628=CARTESIAN_POINT('Ctrl Pts',(48.9241072223979,885.111421624157,146.247641833217));
#77629=CARTESIAN_POINT('Ctrl Pts',(47.9373723577675,885.045596601369,146.224377042919));
#77630=CARTESIAN_POINT('Ctrl Pts',(46.9528271634588,884.957910840272,146.193385928025));
#77631=CARTESIAN_POINT('Ctrl Pts',(45.96861372072,884.8702546257,146.162405255874));
#77632=CARTESIAN_POINT('Ctrl Pts',(44.9865886376979,884.760752420113,146.123703471319));
#77633=CARTESIAN_POINT('Ctrl Pts',(44.0078422813454,884.629525928522,146.077323589032));
#77634=CARTESIAN_POINT('Ctrl Pts',(43.0258069589663,884.497858465203,146.030787852415));
#77635=CARTESIAN_POINT('Ctrl Pts',(42.0470723074263,884.344320502467,145.976522341297));
#77636=CARTESIAN_POINT('Ctrl Pts',(41.0727270204261,884.169082909413,145.914587446599));
#77637=CARTESIAN_POINT('Ctrl Pts',(40.0989774107091,883.993952449893,145.852690416518));
#77638=CARTESIAN_POINT('Ctrl Pts',(39.129612715469,883.797149013145,145.78313342296));
#77639=CARTESIAN_POINT('Ctrl Pts',(38.1657125620015,883.578891788462,145.705993934839));
#77640=CARTESIAN_POINT('Ctrl Pts',(37.2018135599169,883.360634824488,145.628854538862));
#77641=CARTESIAN_POINT('Ctrl Pts',(36.243379246057,883.120924159959,145.544132679205));
#77642=CARTESIAN_POINT('Ctrl Pts',(35.2914770714854,882.860026771341,145.451922714383));
#77643=CARTESIAN_POINT('Ctrl Pts',(34.3395760080784,882.59912968727,145.359712857199));
#77644=CARTESIAN_POINT('Ctrl Pts',(33.39420722623,882.317045971755,145.260014927594));
#77645=CARTESIAN_POINT('Ctrl Pts',(32.4564236228807,882.014089793283,145.152939963344));
#77646=CARTESIAN_POINT('Ctrl Pts',(31.518641088697,881.711133960212,145.04586512117));
#77647=CARTESIAN_POINT('Ctrl Pts',(30.5884438708996,881.38730576192,144.931413278892));
#77648=CARTESIAN_POINT('Ctrl Pts',(29.6668679668588,881.042965858658,144.809711906048));
#77649=CARTESIAN_POINT('Ctrl Pts',(28.7452930884338,880.69862633861,144.688010668644));
#77650=CARTESIAN_POINT('Ctrl Pts',(27.832339657076,880.333775216237,144.559059936951));
#77651=CARTESIAN_POINT('Ctrl Pts',(26.9290244628079,879.948818839737,144.423003328171));
#77652=CARTESIAN_POINT('Ctrl Pts',(26.0257102492375,879.56386288117,144.286946867103));
#77653=CARTESIAN_POINT('Ctrl Pts',(25.1320344013059,879.158801775842,144.143784566895));
#77654=CARTESIAN_POINT('Ctrl Pts',(24.2489922367168,878.734086654315,143.993675872352));
#77655=CARTESIAN_POINT('Ctrl Pts',(23.3659510068373,878.309371982354,143.843567336701));
#77656=CARTESIAN_POINT('Ctrl Pts',(22.49354358391,877.865003406093,143.686512446264));
#77657=CARTESIAN_POINT('Ctrl Pts',(21.6327415962015,877.401475833138,143.522686118134));
#77658=CARTESIAN_POINT('Ctrl Pts',(20.7719404962203,876.937948738209,143.358859958955));
#77659=CARTESIAN_POINT('Ctrl Pts',(19.9227449499613,876.455262762814,143.188262403162));
#77660=CARTESIAN_POINT('Ctrl Pts',(19.086100731926,875.953955488774,143.01108345036));
#77661=CARTESIAN_POINT('Ctrl Pts',(18.2494573539578,875.452648718092,142.833904675462));
#77662=CARTESIAN_POINT('Ctrl Pts',(17.4253654174497,874.932720769122,142.650144546094));
#77663=CARTESIAN_POINT('Ctrl Pts',(16.6147427364191,874.394750700022,142.460007721002));
#77664=CARTESIAN_POINT('Ctrl Pts',(15.8041208472464,873.85678115644,142.269871081646));
#77665=CARTESIAN_POINT('Ctrl Pts',(15.0069683213714,873.300769617006,142.073357790489));
#77666=CARTESIAN_POINT('Ctrl Pts',(14.2241729679096,872.727335325964,141.8706867094));
#77667=CARTESIAN_POINT('Ctrl Pts',(13.4413783578525,872.1539015795,141.668015820784));
#77668=CARTESIAN_POINT('Ctrl Pts',(12.6729410224688,871.563045209417,141.459187187472));
#77669=CARTESIAN_POINT('Ctrl Pts',(11.9197167884083,870.955424266287,141.244433386801));
#77670=CARTESIAN_POINT('Ctrl Pts',(11.1332002832681,870.320946671129,141.020187536586));
#77671=CARTESIAN_POINT('Ctrl Pts',(10.3632718518326,869.66818958464,140.789481095633));
#77672=CARTESIAN_POINT('Ctrl Pts',(9.61086642972582,868.997945659523,140.552594214226));
#77673=CARTESIAN_POINT('Ctrl Pts',(8.88197367705985,868.348646857067,140.323110047864));
#77674=CARTESIAN_POINT('Ctrl Pts',(8.16952578585541,867.682937388807,140.087825796938));
#77675=CARTESIAN_POINT('Ctrl Pts',(7.47433468430374,867.001575918348,139.847009598836));
#77676=CARTESIAN_POINT('Ctrl Pts',(6.78706819199614,866.327981410663,139.60893850818));
#77677=CARTESIAN_POINT('Ctrl Pts',(6.11666734831014,865.639089886227,139.365460934217));
#77678=CARTESIAN_POINT('Ctrl Pts',(5.46387885017508,864.935668637012,139.116848063891));
#77679=CARTESIAN_POINT('Ctrl Pts',(4.81109254389226,864.232249749657,138.868236028327));
#77680=CARTESIAN_POINT('Ctrl Pts',(4.17591857290188,863.514301351529,138.614488772037));
#77681=CARTESIAN_POINT('Ctrl Pts',(3.55906439345839,862.782623092972,138.355888918511));
#77682=CARTESIAN_POINT('Ctrl Pts',(2.94221221808227,862.050947211529,138.097289905136));
#77683=CARTESIAN_POINT('Ctrl Pts',(2.34367981728249,861.305541679978,137.833838368859));
#77684=CARTESIAN_POINT('Ctrl Pts',(1.76413383163206,860.547236725002,137.565827739881));
#77685=CARTESIAN_POINT('Ctrl Pts',(1.18458966576892,859.78893415112,137.297817952462));
#77686=CARTESIAN_POINT('Ctrl Pts',(0.624031891709943,859.017732360335,137.025249145334));
#77687=CARTESIAN_POINT('Ctrl Pts',(0.083084850274769,858.234490305603,136.748424901534));
#77688=CARTESIAN_POINT('Ctrl Pts',(-0.457860551453115,857.451250625018,
136.471601496838));
#77689=CARTESIAN_POINT('Ctrl Pts',(-0.979195249943123,856.655970883114,
136.190522727086));
#77690=CARTESIAN_POINT('Ctrl Pts',(-1.48033859396631,855.849536845141,135.905501651689));
#77691=CARTESIAN_POINT('Ctrl Pts',(-1.98148047346789,855.043105163859,135.620481409226));
#77692=CARTESIAN_POINT('Ctrl Pts',(-2.46243103360221,854.225519385171,135.331518931331));
#77693=CARTESIAN_POINT('Ctrl Pts',(-2.92265460524362,853.397690112986,135.038936056237));
#77694=CARTESIAN_POINT('Ctrl Pts',(-3.38287688203091,852.569863169926,134.746354004335));
#77695=CARTESIAN_POINT('Ctrl Pts',(-3.82237221081663,851.731792928016,134.450151624029));
#77696=CARTESIAN_POINT('Ctrl Pts',(-4.24065109689235,850.884412800929,134.150658815293));
#77697=CARTESIAN_POINT('Ctrl Pts',(-4.65892885164612,850.037034965757,133.851166816597));
#77698=CARTESIAN_POINT('Ctrl Pts',(-5.05599020925946,849.18034743601,133.548384456837));
#77699=CARTESIAN_POINT('Ctrl Pts',(-5.43139293890597,848.31530435549,133.242648962717));
#77700=CARTESIAN_POINT('Ctrl Pts',(-5.80679469402922,847.450263520572,132.936914262269));
#77701=CARTESIAN_POINT('Ctrl Pts',(-6.16053787153141,846.576867321423,132.62822649339));
#77702=CARTESIAN_POINT('Ctrl Pts',(-6.49222848866201,845.696088506238,132.316929458208));
#77703=CARTESIAN_POINT('Ctrl Pts',(-6.82391828088239,844.815311881538,132.005633197217));
#77704=CARTESIAN_POINT('Ctrl Pts',(-7.13355556755057,843.927152823285,131.691727734417));
#77705=CARTESIAN_POINT('Ctrl Pts',(-7.42079549072711,843.032600516941,131.375562681421));
#77706=CARTESIAN_POINT('Ctrl Pts',(-7.70803473077437,842.138050338069,131.059398380346));
#77707=CARTESIAN_POINT('Ctrl Pts',(-7.97287666634953,841.237107089555,130.740974552144));
#77708=CARTESIAN_POINT('Ctrl Pts',(-8.21502633165284,840.330774190458,130.420645839062));
#77709=CARTESIAN_POINT('Ctrl Pts',(-8.4571754474035,839.42444334826,130.100317852959));
#77710=CARTESIAN_POINT('Ctrl Pts',(-8.67663235582913,838.512723029929,129.778085043633));
#77711=CARTESIAN_POINT('Ctrl Pts',(-8.87315263948633,837.5966286528,129.454306293927));
#77712=CARTESIAN_POINT('Ctrl Pts',(-9.06967249854039,836.68053625499,129.13052824378));
#77713=CARTESIAN_POINT('Ctrl Pts',(-9.2432557994382,835.760069968883,128.805204313514));
#77714=CARTESIAN_POINT('Ctrl Pts',(-9.39370921673994,834.836254948099,128.478696827106));
#77715=CARTESIAN_POINT('Ctrl Pts',(-9.54416232533976,833.912441822809,128.15219001063));
#77716=CARTESIAN_POINT('Ctrl Pts',(-9.67148562038048,832.985280129458,127.8244996969));
#77717=CARTESIAN_POINT('Ctrl Pts',(-9.77553729829627,832.055802474329,127.495990843915));
#77718=CARTESIAN_POINT('Ctrl Pts',(-9.87958877403793,831.12632662519,127.167482629228));
#77719=CARTESIAN_POINT('Ctrl Pts',(-9.96036870588743,830.194534977082,126.838155932827));
#77720=CARTESIAN_POINT('Ctrl Pts',(-10.0177871272924,829.261465288766,126.508377533774));
#77721=CARTESIAN_POINT('Ctrl Pts',(-10.0764915750459,828.307497216711,126.171212938794));
#77722=CARTESIAN_POINT('Ctrl Pts',(-10.1107761009928,827.352193369348,125.833576235622));
#77723=CARTESIAN_POINT('Ctrl Pts',(-10.1206007926555,826.396665867741,125.495860485472));
#77724=CARTESIAN_POINT('Ctrl Pts',(-10.130210591096,825.4620383995,125.165531514285));
#77725=CARTESIAN_POINT('Ctrl Pts',(-10.1164190566398,824.527197115671,124.835126973434));
#77726=CARTESIAN_POINT('Ctrl Pts',(-10.0792415503186,823.593183243885,124.505014867996));
#77727=CARTESIAN_POINT('Ctrl Pts',(-10.0420642840558,822.659175403107,124.174904894119));
#77728=CARTESIAN_POINT('Ctrl Pts',(-9.98150135414635,821.72599511826,123.84508740651));
#77729=CARTESIAN_POINT('Ctrl Pts',(-9.89762021480198,820.794681753534,123.515929751641));
#77730=CARTESIAN_POINT('Ctrl Pts',(-9.81373958056812,819.863373996936,123.186774078873));
#77731=CARTESIAN_POINT('Ctrl Pts',(-9.70654103166478,818.933933292096,122.85827828537));
#77732=CARTESIAN_POINT('Ctrl Pts',(-9.57614396301838,818.007394825643,122.530808241113));
#77733=CARTESIAN_POINT('Ctrl Pts',(-9.44574762282193,817.080861535203,122.203340026234));
#77734=CARTESIAN_POINT('Ctrl Pts',(-9.29215304370139,816.157230604051,121.876897603331));
#77735=CARTESIAN_POINT('Ctrl Pts',(-9.11553129335159,815.237530736552,121.551844551334));
#77736=CARTESIAN_POINT('Ctrl Pts',(-8.93891045280868,814.317835606575,121.226793173737));
#77737=CARTESIAN_POINT('Ctrl Pts',(-8.73926270754151,813.402071651942,120.903131206522));
#77738=CARTESIAN_POINT('Ctrl Pts',(-8.51681041518808,812.491258804582,120.581219128141));
#77739=CARTESIAN_POINT('Ctrl Pts',(-8.29435917190049,811.580450252537,120.259308567871));
#77740=CARTESIAN_POINT('Ctrl Pts',(-8.04910363346647,810.674592911782,119.939147933199));
#77741=CARTESIAN_POINT('Ctrl Pts',(-7.78131695061947,809.774695671244,119.621093799608));
#77742=CARTESIAN_POINT('Ctrl Pts',(-7.51353141406179,808.874802282812,119.303041027482));
#77743=CARTESIAN_POINT('Ctrl Pts',(-7.22321497033357,807.980869092476,118.987094791032));
#77744=CARTESIAN_POINT('Ctrl Pts',(-6.91069095350244,807.093891700248,118.673606968988));
#77745=CARTESIAN_POINT('Ctrl Pts',(-6.58504807005736,806.169681527588,118.346959822537));
#77746=CARTESIAN_POINT('Ctrl Pts',(-6.23529373717443,805.253023668774,118.022981919338));
#77747=CARTESIAN_POINT('Ctrl Pts',(-5.86185086381152,804.345026509845,117.702065000521));
#77748=CARTESIAN_POINT('Ctrl Pts',(-5.5034427310267,803.473585147543,117.394068137128));
#77749=CARTESIAN_POINT('Ctrl Pts',(-5.12321546462664,802.610121193389,117.088890759696));
#77750=CARTESIAN_POINT('Ctrl Pts',(-4.72159255818815,801.755596365468,116.786872771939));
#77751=CARTESIAN_POINT('Ctrl Pts',(-4.3199744018931,800.901081644331,116.48485835626));
#77752=CARTESIAN_POINT('Ctrl Pts',(-3.89696117822355,800.055505979351,116.186003305489));
#77753=CARTESIAN_POINT('Ctrl Pts',(-3.45302402421467,799.219811142534,115.890640473716));
#77754=CARTESIAN_POINT('Ctrl Pts',(-3.00909134785035,798.384124734713,115.595280621036));
#77755=CARTESIAN_POINT('Ctrl Pts',(-2.54423523677349,797.558319093993,115.303412965772));
#77756=CARTESIAN_POINT('Ctrl Pts',(-2.05897342069375,796.743313954683,115.015362573152));
#77757=CARTESIAN_POINT('Ctrl Pts',(-1.57371565419147,795.928315616704,114.727314584352));
#77758=CARTESIAN_POINT('Ctrl Pts',(-1.06805260362502,795.124117734704,114.443083842138));
#77759=CARTESIAN_POINT('Ctrl Pts',(-0.54254743770422,794.331615962585,114.162986900903));
#77760=CARTESIAN_POINT('Ctrl Pts',(-0.0170308548852931,793.539096972915,
113.882883874403));
#77761=CARTESIAN_POINT('Ctrl Pts',(0.528328618654131,792.758274732585,113.606914874889));
#77762=CARTESIAN_POINT('Ctrl Pts',(1.09292357699108,791.990018899273,113.335387268811));
#77763=CARTESIAN_POINT('Ctrl Pts',(1.65750755153488,791.221778011831,113.063864945109));
#77764=CARTESIAN_POINT('Ctrl Pts',(2.24132616889006,790.466103169512,112.796783886936));
#77765=CARTESIAN_POINT('Ctrl Pts',(2.8437292137206,789.723835988798,112.534441550034));
#77766=CARTESIAN_POINT('Ctrl Pts',(3.4461352662169,788.981565102108,112.272097903314));
#77767=CARTESIAN_POINT('Ctrl Pts',(4.06712583211287,788.252702133763,112.014493068606));
#77768=CARTESIAN_POINT('Ctrl Pts',(4.70600928971643,787.538058847205,111.761913950576));
#77769=CARTESIAN_POINT('Ctrl Pts',(4.89369464802301,787.328117456952,111.687713559716));
#77770=CARTESIAN_POINT('Ctrl Pts',(5.08292392017445,787.119403041301,111.613946823196));
#77771=CARTESIAN_POINT('Ctrl Pts',(5.27367891242885,786.911935667425,111.540620833434));
#77772=CARTESIAN_POINT('Ctrl Pts',(5.8889578504258,786.242751055482,111.304108349146));
#77773=CARTESIAN_POINT('Ctrl Pts',(6.52011267108288,785.586541088171,111.072184698428));
#77774=CARTESIAN_POINT('Ctrl Pts',(7.16653231814136,784.944093264104,110.844773330027));
#77775=CARTESIAN_POINT('Ctrl Pts',(7.76297552640692,784.351314806528,110.634943745203));
#77776=CARTESIAN_POINT('Ctrl Pts',(8.37241468131322,783.770253293932,110.428955962841));
#77777=CARTESIAN_POINT('Ctrl Pts',(8.99433775587323,783.201503264864,110.22674055518));
#77778=CARTESIAN_POINT('Ctrl Pts',(9.53777057157126,782.704532751359,110.050045891711));
#77779=CARTESIAN_POINT('Ctrl Pts',(10.0907350345358,782.216962646337,109.876231644642));
#77780=CARTESIAN_POINT('Ctrl Pts',(10.6528630950096,781.7391645579,109.70524141257));
#77781=CARTESIAN_POINT('Ctrl Pts',(11.1247663754188,781.338055805001,109.561696094151));
#77782=CARTESIAN_POINT('Ctrl Pts',(11.6031274536375,780.94383391265,109.42014094233));
#77783=CARTESIAN_POINT('Ctrl Pts',(12.0877107975547,780.556697717533,109.280534704239));
#77784=CARTESIAN_POINT('',(15.6662215388589,777.892883824876,108.344718533713));
#77785=CARTESIAN_POINT('Ctrl Pts',(12.0879058517676,780.556909685729,109.280623951409));
#77786=CARTESIAN_POINT('Ctrl Pts',(13.2461021182051,779.624779114207,108.965204337006));
#77787=CARTESIAN_POINT('Ctrl Pts',(14.4399142821894,778.736588450391,108.651287750854));
#77788=CARTESIAN_POINT('Ctrl Pts',(15.6662215388589,777.892883824876,108.344718533713));
#77789=CARTESIAN_POINT('',(15.9133244032209,777.721729749158,108.288790421306));
#77790=CARTESIAN_POINT('Ctrl Pts',(15.6661725562014,777.892797194896,108.344684931383));
#77791=CARTESIAN_POINT('Ctrl Pts',(15.7484074658122,777.83595842687,108.324895482652));
#77792=CARTESIAN_POINT('Ctrl Pts',(15.8307836517621,777.779300419268,108.305200714399));
#77793=CARTESIAN_POINT('Ctrl Pts',(15.9133012616994,777.722828034493,108.285587077081));
#77794=CARTESIAN_POINT('Origin',(16.0893891985929,777.949599269962,108.373139154749));
#77795=CARTESIAN_POINT('Origin',(52.8776183915471,826.553927293695,123.218188520575));
#77796=CARTESIAN_POINT('',(52.8776183915471,817.923891256083,120.210169373246));
#77797=CARTESIAN_POINT('',(52.8776183915471,835.157491445947,126.301106793786));
#77798=CARTESIAN_POINT('Origin',(52.8776183915471,826.540691351014,123.255638083516));
#77799=CARTESIAN_POINT('',(52.8776183915471,836.515175234928,127.233000992115));
#77800=CARTESIAN_POINT('',(52.8776183915471,835.030963717011,126.214260020273));
#77801=CARTESIAN_POINT('Origin',(52.8776183915471,826.39866537014,123.657484105229));
#77802=CARTESIAN_POINT('Origin',(52.8776183915471,826.540691351014,123.255638083516));
#77803=CARTESIAN_POINT('Origin',(52.8776183915471,826.720543860959,122.746766289965));
#77804=CARTESIAN_POINT('',(52.8776183915471,836.747846694345,127.351374719744));
#77805=CARTESIAN_POINT('Origin',(52.8776183915471,837.081079828879,126.408530258526));
#77806=CARTESIAN_POINT('Origin',(52.8776183915471,826.387310726425,123.689610751182));
#77807=CARTESIAN_POINT('Origin',(52.8776183915471,826.605067049179,123.073494520463));
#77808=CARTESIAN_POINT('',(52.8776183915471,818.128030625863,120.077423020765));
#77809=CARTESIAN_POINT('Origin',(52.8776183915471,817.93946173362,120.010776393858));
#77810=CARTESIAN_POINT('',(52.8776183915471,835.082103472494,126.069566020161));
#77811=CARTESIAN_POINT('Origin',(52.8776183915471,826.605067049179,123.073494520463));
#77812=CARTESIAN_POINT('Origin',(52.8776183915471,826.605067049179,123.073494520463));
#77813=CARTESIAN_POINT('Origin',(52.8776183915471,826.387310726428,123.689610751183));
#77814=CARTESIAN_POINT('',(11.859543044092,780.20945181141,109.457020834635));
#77815=CARTESIAN_POINT('',(93.8960334963338,780.209723961161,109.457117026756));
#77816=CARTESIAN_POINT('Origin',(52.8776183915471,825.731304036591,125.545705508684));
#77817=CARTESIAN_POINT('',(94.9631204076456,779.681651525798,107.182848479366));
#77818=CARTESIAN_POINT('Ctrl Pts',(94.9630822777178,779.681610364452,107.182867696666));
#77819=CARTESIAN_POINT('Ctrl Pts',(94.9631775102079,779.603493726972,107.402215219776));
#77820=CARTESIAN_POINT('Ctrl Pts',(94.9366427780809,779.555592945074,107.631525596045));
#77821=CARTESIAN_POINT('Ctrl Pts',(94.8338455012492,779.524285459544,108.083418924359));
#77822=CARTESIAN_POINT('Ctrl Pts',(94.7576080457245,779.540886396965,108.305891585224));
#77823=CARTESIAN_POINT('Ctrl Pts',(94.564542439954,779.636618923506,108.71737180854));
#77824=CARTESIAN_POINT('Ctrl Pts',(94.4477614101949,779.715727147703,108.90627894322));
#77825=CARTESIAN_POINT('Ctrl Pts',(94.1876223298964,779.926998404112,109.227910928672));
#77826=CARTESIAN_POINT('Ctrl Pts',(94.0443277701068,780.059109872482,109.360557280451));
#77827=CARTESIAN_POINT('Ctrl Pts',(93.8961044974596,780.209688803323,109.456966042443));
#77828=CARTESIAN_POINT('',(10.7920801946104,779.681690583154,107.182830244375));
#77829=CARTESIAN_POINT('Origin',(52.8776183915471,826.387310726428,123.689610751183));
#77830=CARTESIAN_POINT('Ctrl Pts',(10.7921545066383,779.681610363091,107.182867697302));
#77831=CARTESIAN_POINT('Ctrl Pts',(10.7929881005113,779.604523358188,107.401313219156));
#77832=CARTESIAN_POINT('Ctrl Pts',(10.8194412281584,779.556508528823,107.630605497856));
#77833=CARTESIAN_POINT('Ctrl Pts',(10.9221008132029,779.524954693993,108.082505965785));
#77834=CARTESIAN_POINT('Ctrl Pts',(10.9982822164968,779.541423389251,108.305003868565));
#77835=CARTESIAN_POINT('Ctrl Pts',(11.1912682486577,779.636889115481,108.716575677992));
#77836=CARTESIAN_POINT('Ctrl Pts',(11.3080257792239,779.715862848014,108.905549140411));
#77837=CARTESIAN_POINT('Ctrl Pts',(11.5681536396292,779.926879240623,109.227347596125));
#77838=CARTESIAN_POINT('Ctrl Pts',(11.7114604851836,780.058870402084,109.360094054407));
#77839=CARTESIAN_POINT('Ctrl Pts',(11.8594721313973,780.209416745796,109.456869892554));
#77840=CARTESIAN_POINT('Origin',(52.8776183915471,640.625373764374,98.8443190641064));
#77841=CARTESIAN_POINT('',(68.1332263705066,640.627119090081,81.6674251557765));
#77842=CARTESIAN_POINT('',(37.6220104125875,640.627119090085,81.6674251557765));
#77843=CARTESIAN_POINT('Origin',(52.8776183915471,640.627119090081,98.8443190641064));
#77844=CARTESIAN_POINT('',(67.8012014212036,640.125373764374,82.0412652109852));
#77845=CARTESIAN_POINT('Origin',(67.8012014212036,640.625373764374,82.0412652109852));
#77846=CARTESIAN_POINT('',(37.9540353618905,640.125373764374,82.0412652109853));
#77847=CARTESIAN_POINT('Origin',(52.8776183915471,640.125373764374,98.8443190641064));
#77848=CARTESIAN_POINT('Origin',(37.9540353618905,640.625373764374,82.0412652109853));
#77849=CARTESIAN_POINT('Origin',(68.3051174347811,640.625373764374,82.3731046594733));
#77850=CARTESIAN_POINT('',(68.3051174347811,640.125373764374,83.1627853766115));
#77851=CARTESIAN_POINT('',(68.8051174347811,640.625373764374,83.1627853766115));
#77852=CARTESIAN_POINT('Origin',(68.3051174347811,640.625373764374,83.1627853766115));
#77853=CARTESIAN_POINT('',(68.80511438861,640.627119090084,83.1627853766115));
#77854=CARTESIAN_POINT('Origin',(68.3051174347811,640.625373764374,83.1627853766115));
#77855=CARTESIAN_POINT('',(68.80511438861,640.627119090078,98.0546383469682));
#77856=CARTESIAN_POINT('',(68.80511438861,640.627119090081,82.287785267134));
#77857=CARTESIAN_POINT('',(68.3051174347811,640.125373764374,98.0546383469682));
#77858=CARTESIAN_POINT('Origin',(68.3051174347811,640.625373764374,98.0546383469682));
#77859=CARTESIAN_POINT('',(68.3051174347811,640.125373764374,82.3731046594733));
#77860=CARTESIAN_POINT('Origin',(52.8776183915471,825.829705040065,125.267291295063));
#77861=CARTESIAN_POINT('Ctrl Pts',(93.6680386448423,780.55786728502,109.278884568687));
#77862=CARTESIAN_POINT('Ctrl Pts',(93.6684006063571,780.552263632436,109.293364314974));
#77863=CARTESIAN_POINT('Ctrl Pts',(93.6695470714606,780.54579059155,109.307535012193));
#77864=CARTESIAN_POINT('Ctrl Pts',(93.6714688592443,780.53853308618,109.321188415692));
#77865=CARTESIAN_POINT('Ctrl Pts',(93.6735703333615,780.530597007171,109.336118406563));
#77866=CARTESIAN_POINT('Ctrl Pts',(93.6765985254415,780.521723742468,109.350428795394));
#77867=CARTESIAN_POINT('Ctrl Pts',(93.6805040104157,780.512054570306,109.363893905088));
#77868=CARTESIAN_POINT('Ctrl Pts',(93.6845685330264,780.501991653885,109.377907335729));
#77869=CARTESIAN_POINT('Ctrl Pts',(93.6895823854221,780.491067718938,109.391005393111));
#77870=CARTESIAN_POINT('Ctrl Pts',(93.695461822842,780.479457398172,109.402989163316));
#77871=CARTESIAN_POINT('Ctrl Pts',(93.702041769321,780.46646375885,109.416400746931));
#77872=CARTESIAN_POINT('Ctrl Pts',(93.7097054443003,780.452610794498,109.428417101803));
#77873=CARTESIAN_POINT('Ctrl Pts',(93.718312273728,780.438149357518,109.438824117562));
#77874=CARTESIAN_POINT('Ctrl Pts',(93.7241837646935,780.428283913187,109.445923677222));
#77875=CARTESIAN_POINT('Ctrl Pts',(93.7304938312127,780.418135258818,109.4522756276));
#77876=CARTESIAN_POINT('Ctrl Pts',(93.7371927454339,780.407785047693,109.457824301935));
#77877=CARTESIAN_POINT('Ctrl Pts',(93.7480264169828,780.391046396609,109.466797773349));
#77878=CARTESIAN_POINT('Ctrl Pts',(93.7598269340027,780.37385921059,109.473625169796));
#77879=CARTESIAN_POINT('Ctrl Pts',(93.7723431068519,780.356589301551,109.478180574098));
#77880=CARTESIAN_POINT('Ctrl Pts',(93.782596465795,780.342441640088,109.48191240139));
#77881=CARTESIAN_POINT('Ctrl Pts',(93.7933303813018,780.328237953836,109.484119948096));
#77882=CARTESIAN_POINT('Ctrl Pts',(93.804388447967,780.31419121037,109.484765154944));
#77883=CARTESIAN_POINT('Ctrl Pts',(93.8147461868357,780.301034073125,109.485369499649));
#77884=CARTESIAN_POINT('Ctrl Pts',(93.8253884059732,780.288014795392,109.4846023526));
#77885=CARTESIAN_POINT('Ctrl Pts',(93.836166085422,780.275321659614,109.482467289298));
#77886=CARTESIAN_POINT('Ctrl Pts',(93.8462299626048,780.263469186162,109.480473630556));
#77887=CARTESIAN_POINT('Ctrl Pts',(93.8564115840146,780.251901722966,109.47728674108));
#77888=CARTESIAN_POINT('Ctrl Pts',(93.8665734130811,780.240778459561,109.472950114439));
#77889=CARTESIAN_POINT('Ctrl Pts',(93.8764579813262,780.22995868927,109.468731810656));
#77890=CARTESIAN_POINT('Ctrl Pts',(93.8863232420543,780.219560060177,109.463425299444));
#77891=CARTESIAN_POINT('Ctrl Pts',(93.8960335411076,780.209723997027,109.457117039439));
#77892=CARTESIAN_POINT('Origin',(11.8936587105147,780.345763542483,109.19196327747));
#77893=CARTESIAN_POINT('Origin',(52.8776183915471,826.720543860962,122.746766289966));
#77894=CARTESIAN_POINT('',(52.8776183915471,818.163626601955,119.976708339595));
#77895=CARTESIAN_POINT('',(52.8776183915471,835.117699448586,125.968851338991));
#77896=CARTESIAN_POINT('Origin',(52.8776183915471,826.64066302527,122.972779839293));
#77897=CARTESIAN_POINT('',(52.8776183915471,835.197580284278,125.742837789664));
#77898=CARTESIAN_POINT('Origin',(52.8776183915471,826.64066302527,122.972779839293));
#77899=CARTESIAN_POINT('Origin',(52.8776183915471,826.64066302527,122.972779839293));
#77900=CARTESIAN_POINT('',(52.8776183915471,818.246409367408,120.213087978549));
#77901=CARTESIAN_POINT('Origin',(52.8776183915471,818.352195494198,120.043354966502));
#77902=CARTESIAN_POINT('Origin',(52.8776183915471,826.575588168114,123.156901591529));
#77903=CARTESIAN_POINT('Origin',(3.61051441020205,837.780336961955,118.41143764368));
#77904=CARTESIAN_POINT('',(3.61051441020205,836.116920330448,124.618332887168));
#77905=CARTESIAN_POINT('Origin',(3.61051441020205,835.645498099839,124.451716319901));
#77906=CARTESIAN_POINT('',(3.61051441020237,834.62882423843,128.828727991124));
#77907=CARTESIAN_POINT('',(3.61051441020205,838.251759192563,118.578054210947));
#77908=CARTESIAN_POINT('Ctrl Pts',(3.61023855880141,833.690302175803,128.48326536002));
#77909=CARTESIAN_POINT('Ctrl Pts',(3.54970624529949,833.688968919781,128.487137870804));
#77910=CARTESIAN_POINT('Ctrl Pts',(3.48969016814101,833.697918586839,128.494902083681));
#77911=CARTESIAN_POINT('Ctrl Pts',(3.37188423689048,833.737039310482,128.518373667602));
#77912=CARTESIAN_POINT('Ctrl Pts',(3.31579912354491,833.768524751875,128.534458727518));
#77913=CARTESIAN_POINT('Ctrl Pts',(3.22048458350583,833.850144207547,128.572392016225));
#77914=CARTESIAN_POINT('Ctrl Pts',(3.1821019261915,833.899442320513,128.593857577818));
#77915=CARTESIAN_POINT('Ctrl Pts',(3.12820529820177,834.009523847839,128.639201274647));
#77916=CARTESIAN_POINT('Ctrl Pts',(3.1131494283263,834.069215464973,128.66263211001));
#77917=CARTESIAN_POINT('Ctrl Pts',(3.10851033861788,834.191402337082,128.708319672525));
#77918=CARTESIAN_POINT('Ctrl Pts',(3.1189842716532,834.25269542384,128.730124180922));
#77919=CARTESIAN_POINT('Ctrl Pts',(3.16441820688302,834.368927344028,128.769238568114));
#77920=CARTESIAN_POINT('Ctrl Pts',(3.1990099353471,834.42268871086,128.786145498392));
#77921=CARTESIAN_POINT('Ctrl Pts',(3.28805051477577,834.515358321064,128.812847356105));
#77922=CARTESIAN_POINT('Ctrl Pts',(3.34169967361902,834.553298184813,128.822356138207));
#77923=CARTESIAN_POINT('Ctrl Pts',(3.46101423119602,834.607921907473,128.832756247285));
#77924=CARTESIAN_POINT('Ctrl Pts',(3.52555294689342,834.624039698791,128.833535305143));
#77925=CARTESIAN_POINT('Ctrl Pts',(3.65798399987879,834.63204521721,128.826236604458));
#77926=CARTESIAN_POINT('Ctrl Pts',(3.72460865089341,834.623439329546,128.818083126898));
#77927=CARTESIAN_POINT('Ctrl Pts',(3.84924104636131,834.582078715853,128.793884832996));
#77928=CARTESIAN_POINT('Ctrl Pts',(3.90608099408457,834.549896254268,128.778130750541));
#77929=CARTESIAN_POINT('Ctrl Pts',(4.00244766333427,834.466234776723,128.740977444715));
#77930=CARTESIAN_POINT('Ctrl Pts',(4.04105590966,834.415630846942,128.719955933113));
#77931=CARTESIAN_POINT('Ctrl Pts',(4.09472970727648,834.302600429106,128.6751956904));
#77932=CARTESIAN_POINT('Ctrl Pts',(4.1092069337592,834.241289170898,128.651897825474));
#77933=CARTESIAN_POINT('Ctrl Pts',(4.1116547785933,834.116320260818,128.606071945226));
#77934=CARTESIAN_POINT('Ctrl Pts',(4.09955730020252,834.053924847908,128.584007358413));
#77935=CARTESIAN_POINT('Ctrl Pts',(4.05018166696433,833.936857875505,128.544242066616));
#77936=CARTESIAN_POINT('Ctrl Pts',(4.01344192677525,833.883355043824,128.526937604381));
#77937=CARTESIAN_POINT('Ctrl Pts',(3.9202568917958,833.792623252911,128.499637264666));
#77938=CARTESIAN_POINT('Ctrl Pts',(3.86478659222662,833.756269032296,128.489904210129));
#77939=CARTESIAN_POINT('Ctrl Pts',(3.74236795433918,833.705563571832,128.479531579772));
#77940=CARTESIAN_POINT('Ctrl Pts',(3.67661606883661,833.69176417535,128.479018907034));
#77941=CARTESIAN_POINT('Ctrl Pts',(3.61023855880141,833.690302175803,128.48326536002));
#77942=CARTESIAN_POINT('Origin',(3.61051441020205,837.780336961955,118.41143764368));
#77943=CARTESIAN_POINT('',(3.610514410202,833.200671336708,128.303923553727));
#77944=CARTESIAN_POINT('',(3.61051441019541,835.117863715507,129.009742759232));
#77945=CARTESIAN_POINT('Ctrl Pts',(3.61051441020201,833.200671336708,128.303923553727));
#77946=CARTESIAN_POINT('Ctrl Pts',(3.607420505753,833.200603853511,128.304114489599));
#77947=CARTESIAN_POINT('Ctrl Pts',(3.60432596997758,833.200549435127,128.304310645018));
#77948=CARTESIAN_POINT('Ctrl Pts',(3.4673576701867,833.198720168197,128.313222308701));
#77949=CARTESIAN_POINT('Ctrl Pts',(3.33506769578121,833.221432861026,128.331556653784));
#77950=CARTESIAN_POINT('Ctrl Pts',(3.08885719489787,833.31315177346,128.385241364804));
#77951=CARTESIAN_POINT('Ctrl Pts',(2.97723197304173,833.381238660411,128.420056263876));
#77952=CARTESIAN_POINT('Ctrl Pts',(2.78989253690627,833.554051605796,128.501007325928));
#77953=CARTESIAN_POINT('Ctrl Pts',(2.71578278492597,833.657007447089,128.546322414568));
#77954=CARTESIAN_POINT('Ctrl Pts',(2.61493637022606,833.884781048766,128.640900564318));
#77955=CARTESIAN_POINT('Ctrl Pts',(2.58903224367024,834.007350332351,128.689230558964));
#77956=CARTESIAN_POINT('Ctrl Pts',(2.58918047884613,834.256867321233,128.782327108995));
#77957=CARTESIAN_POINT('Ctrl Pts',(2.61533535784576,834.381343663168,128.826155651171));
#77958=CARTESIAN_POINT('Ctrl Pts',(2.71714194869618,834.616112757335,128.90357578295));
#77959=CARTESIAN_POINT('Ctrl Pts',(2.7920532267335,834.723959726474,128.936334868865));
#77960=CARTESIAN_POINT('Ctrl Pts',(2.98137159503634,834.907968170851,128.986643990243));
#77961=CARTESIAN_POINT('Ctrl Pts',(3.09410414598422,834.982164030165,129.003640167242));
#77962=CARTESIAN_POINT('Ctrl Pts',(3.34231950686057,835.085908810425,129.020009783769));
#77963=CARTESIAN_POINT('Ctrl Pts',(3.47545047883008,835.11442517967,129.019227036856));
#77964=CARTESIAN_POINT('Ctrl Pts',(3.60989644190229,835.117848159014,129.009786213532));
#77965=CARTESIAN_POINT('Ctrl Pts',(3.61010243425556,835.117853403556,129.009771748707));
#77966=CARTESIAN_POINT('Ctrl Pts',(3.61030842369358,835.117858589052,129.009757263938));
#77967=CARTESIAN_POINT('Ctrl Pts',(3.6105144101888,835.117863715506,129.009742759232));
#77968=CARTESIAN_POINT('',(3.61051441020205,838.743366102197,118.751804726747));
#77969=CARTESIAN_POINT('Ctrl Pts',(3.6105144101888,835.117863715507,129.009742759232));
#77970=CARTESIAN_POINT('Ctrl Pts',(3.74358702873083,835.121175537834,129.000372342509));
#77971=CARTESIAN_POINT('Ctrl Pts',(3.87543331537735,835.099838142981,128.982703984738));
#77972=CARTESIAN_POINT('Ctrl Pts',(4.12318024047454,835.009653073117,128.932477177548));
#77973=CARTESIAN_POINT('Ctrl Pts',(4.23646391221276,834.941155999679,128.900240030458));
#77974=CARTESIAN_POINT('Ctrl Pts',(4.42691427816867,834.766191500003,128.82512706458));
#77975=CARTESIAN_POINT('Ctrl Pts',(4.50235825038151,834.661612991776,128.783019910645));
#77976=CARTESIAN_POINT('Ctrl Pts',(4.60556281030655,834.429622981205,128.693411449959));
#77977=CARTESIAN_POINT('Ctrl Pts',(4.63210431266964,834.304430572222,128.646760959523));
#77978=CARTESIAN_POINT('Ctrl Pts',(4.63173866563419,834.050426145918,128.554659044094));
#77979=CARTESIAN_POINT('Ctrl Pts',(4.60467802583654,833.924134376609,128.510120334094));
#77980=CARTESIAN_POINT('Ctrl Pts',(4.50013123319633,833.688443712997,128.429552133629));
#77981=CARTESIAN_POINT('Ctrl Pts',(4.42384712657423,833.581316578468,128.394299832691));
#77982=CARTESIAN_POINT('Ctrl Pts',(4.23230042940205,833.400593907936,128.33847956846));
#77983=CARTESIAN_POINT('Ctrl Pts',(4.11906927618906,833.328650323819,128.318425858318));
#77984=CARTESIAN_POINT('Ctrl Pts',(3.87260447181931,833.230048980955,128.297143385851));
#77985=CARTESIAN_POINT('Ctrl Pts',(3.74213002483795,833.203542091986,128.295801085002));
#77986=CARTESIAN_POINT('Ctrl Pts',(3.610514410202,833.200671336708,128.303923553727));
#77987=CARTESIAN_POINT('Ctrl Pts',(4.82708931360096,834.938756820481,128.868207249531));
#77988=CARTESIAN_POINT('Ctrl Pts',(4.6896478039067,834.31354365703,128.647235762952));
#77989=CARTESIAN_POINT('Ctrl Pts',(4.56596057298178,833.685782312016,128.425363662788));
#77990=CARTESIAN_POINT('Ctrl Pts',(4.45608061274202,833.055741740253,128.202686006771));
#77991=CARTESIAN_POINT('Ctrl Pts',(3.82123976285279,835.120615159236,128.979286076428));
#77992=CARTESIAN_POINT('Ctrl Pts',(3.68092116765224,834.482314306813,128.753688957733));
#77993=CARTESIAN_POINT('Ctrl Pts',(3.55464477177853,833.841411931325,128.527172372761));
#77994=CARTESIAN_POINT('Ctrl Pts',(3.4424646764359,833.198182617664,128.299833369106));
#77995=CARTESIAN_POINT('Ctrl Pts',(2.79286361328544,835.287202884736,129.147582594022));
#77996=CARTESIAN_POINT('Ctrl Pts',(2.6496034985378,834.635521236761,128.917256249428));
#77997=CARTESIAN_POINT('Ctrl Pts',(2.52067995182663,833.981183529609,128.685991163651));
#77998=CARTESIAN_POINT('Ctrl Pts',(2.40614820848774,833.324470104333,128.453886418704));
#77999=CARTESIAN_POINT('Origin',(52.8776183915471,827.175936191914,121.458286566849));
#78000=CARTESIAN_POINT('Origin',(52.8776183915471,839.88934933413,85.4871602829437));
#78001=CARTESIAN_POINT('Origin',(44.574479425553,750.796902408053,107.247996346823));
#78002=CARTESIAN_POINT('',(44.574479425553,751.028294523684,104.84489734479));
#78003=CARTESIAN_POINT('',(44.574479425553,751.190391228939,103.16145621705));
#78004=CARTESIAN_POINT('',(44.574479425553,750.796902408053,107.247996346823));
#78005=CARTESIAN_POINT('',(44.5744737598758,740.123648048838,102.671482055163));
#78006=CARTESIAN_POINT('Ctrl Pts',(44.574479425553,751.190390984301,103.161456255756));
#78007=CARTESIAN_POINT('Ctrl Pts',(44.574479425553,749.674634276855,102.996991076383));
#78008=CARTESIAN_POINT('Ctrl Pts',(44.5744794185563,748.157236956516,102.868136570664));
#78009=CARTESIAN_POINT('Ctrl Pts',(44.5744794208369,746.637666420114,102.785395558612));
#78010=CARTESIAN_POINT('Ctrl Pts',(44.5744794212215,746.381436650187,102.771443780808));
#78011=CARTESIAN_POINT('Ctrl Pts',(44.5744794220274,746.125145008676,102.75880305028));
#78012=CARTESIAN_POINT('Ctrl Pts',(44.5744794229963,745.868788828836,102.747523631887));
#78013=CARTESIAN_POINT('Ctrl Pts',(44.5744794232527,745.800952768154,102.744538912302));
#78014=CARTESIAN_POINT('Ctrl Pts',(44.5744794235174,745.733112429613,102.741646736372));
#78015=CARTESIAN_POINT('Ctrl Pts',(44.5744794237779,745.66526790518,102.738845268841));
#78016=CARTESIAN_POINT('Ctrl Pts',(44.5744794271895,744.776818912522,102.702159021465));
#78017=CARTESIAN_POINT('Ctrl Pts',(44.5744794246643,743.887633214054,102.68114827826));
#78018=CARTESIAN_POINT('Ctrl Pts',(44.57447942518,742.997909741617,102.671614854512));
#78019=CARTESIAN_POINT('Ctrl Pts',(44.5744794251997,742.963938779512,102.67125085425));
#78020=CARTESIAN_POINT('Ctrl Pts',(44.5744794252212,742.929967047581,102.670903547168));
#78021=CARTESIAN_POINT('Ctrl Pts',(44.5744794252439,742.895994571136,102.670572357382));
#78022=CARTESIAN_POINT('Ctrl Pts',(44.5744794257199,742.184192104095,102.663633160374));
#78023=CARTESIAN_POINT('Ctrl Pts',(44.5744805176467,741.472051967534,102.663812317252));
#78024=CARTESIAN_POINT('Ctrl Pts',(44.5744783292307,740.759831783239,102.666908058489));
#78025=CARTESIAN_POINT('Ctrl Pts',(44.5744776776485,740.547774267963,102.667829789169));
#78026=CARTESIAN_POINT('Ctrl Pts',(44.5744765953231,740.335709718464,102.669010137175));
#78027=CARTESIAN_POINT('Ctrl Pts',(44.5744741956371,740.123643706643,102.670338613259));
#78028=CARTESIAN_POINT('',(44.574479425553,737.487748923763,102.682654164686));
#78029=CARTESIAN_POINT('',(44.574479425553,740.123646440349,102.672625562047));
#78030=CARTESIAN_POINT('',(44.5744794255551,737.051924408278,102.796187237243));
#78031=CARTESIAN_POINT('Ctrl Pts',(44.574479425553,737.487748923764,102.682654164686));
#78032=CARTESIAN_POINT('Ctrl Pts',(44.574479425553,737.483496025753,102.683718797301));
#78033=CARTESIAN_POINT('Ctrl Pts',(44.574479425553,737.479243465217,102.684784786436));
#78034=CARTESIAN_POINT('Ctrl Pts',(44.574479425553,737.406445987069,102.703057328914));
#78035=CARTESIAN_POINT('Ctrl Pts',(44.5744794246898,737.337998433286,102.72060842095));
#78036=CARTESIAN_POINT('Ctrl Pts',(44.5744794246898,737.196963765955,102.757400510756));
#78037=CARTESIAN_POINT('Ctrl Pts',(44.574479425553,737.124447291944,102.776662229155));
#78038=CARTESIAN_POINT('Ctrl Pts',(44.574479425553,737.051933705082,102.796186515614));
#78039=CARTESIAN_POINT('',(44.574479425553,736.984851146654,103.492667548598));
#78040=CARTESIAN_POINT('',(44.574479425553,736.753459031024,105.895766550631));
#78041=CARTESIAN_POINT('',(44.574479425553,751.028294523684,104.84489734479));
#78042=CARTESIAN_POINT('Origin',(52.8776183915471,736.753459031024,105.895766550631));
#78043=CARTESIAN_POINT('',(61.1807573575412,736.984851146654,103.492667548599));
#78044=CARTESIAN_POINT('',(60.8450373933169,734.658443669204,103.268659986875));
#78045=CARTESIAN_POINT('Origin',(52.8776183915471,736.984851146654,103.492667548598));
#78046=CARTESIAN_POINT('',(61.1807573575412,737.051933882625,102.795986698316));
#78047=CARTESIAN_POINT('Ctrl Pts',(60.8450364033132,734.658440391634,103.268658813673));
#78048=CARTESIAN_POINT('Ctrl Pts',(60.9043602784127,734.86592469736,103.223858487515));
#78049=CARTESIAN_POINT('Ctrl Pts',(60.9560530979001,735.075773134149,103.1806805371));
#78050=CARTESIAN_POINT('Ctrl Pts',(60.9999054241525,735.287413267627,103.138859881021));
#78051=CARTESIAN_POINT('Ctrl Pts',(61.0381189952664,735.471839636361,103.102416737598));
#78052=CARTESIAN_POINT('Ctrl Pts',(61.07037943333,735.657626095902,103.067004230362));
#78053=CARTESIAN_POINT('Ctrl Pts',(61.096578180922,735.84438204548,103.032445812295));
#78054=CARTESIAN_POINT('Ctrl Pts',(61.1218367646853,736.024436102613,102.999127551779));
#78055=CARTESIAN_POINT('Ctrl Pts',(61.1414225510105,736.205129994327,102.966676983641));
#78056=CARTESIAN_POINT('Ctrl Pts',(61.1553113009867,736.38614342945,102.933437414957));
#78057=CARTESIAN_POINT('Ctrl Pts',(61.1568911442891,736.406733681532,102.929656418824));
#78058=CARTESIAN_POINT('Ctrl Pts',(61.1583973289327,736.427328066591,102.925865213634));
#78059=CARTESIAN_POINT('Ctrl Pts',(61.1598298619551,736.447926112677,102.922061360995));
#78060=CARTESIAN_POINT('Ctrl Pts',(61.1657763651597,736.53342944499,102.90627141301));
#78061=CARTESIAN_POINT('Ctrl Pts',(61.1704619101878,736.619114102371,102.890867626113));
#78062=CARTESIAN_POINT('Ctrl Pts',(61.1738683606914,736.704671003371,102.874266030665));
#78063=CARTESIAN_POINT('Ctrl Pts',(61.1772935325301,736.790698112117,102.857573195367));
#78064=CARTESIAN_POINT('Ctrl Pts',(61.1794255194344,736.876595794494,102.839669324177));
#78065=CARTESIAN_POINT('Ctrl Pts',(61.180298716096,736.962049331845,102.818944138484));
#78066=CARTESIAN_POINT('Ctrl Pts',(61.1806054804515,736.99207017419,102.811663134659));
#78067=CARTESIAN_POINT('Ctrl Pts',(61.1807573575412,737.022036214132,102.804033925453));
#78068=CARTESIAN_POINT('Ctrl Pts',(61.1807573575412,737.051933882625,102.795986698316));
#78069=CARTESIAN_POINT('',(61.1807573575412,736.753459031024,105.895766550631));
#78070=CARTESIAN_POINT('Origin',(52.8776183915471,736.984851146654,103.492667548598));
#78071=CARTESIAN_POINT('',(59.2182833240547,732.044715789226,103.727362864435));
#78072=CARTESIAN_POINT('Ctrl Pts',(60.8450391521548,734.658446660987,103.268691491693));
#78073=CARTESIAN_POINT('Ctrl Pts',(60.808566415916,734.530888123547,103.296230653766));
#78074=CARTESIAN_POINT('Ctrl Pts',(60.7665091025834,734.403593561596,103.322321835396));
#78075=CARTESIAN_POINT('Ctrl Pts',(60.6844080075902,734.183682229405,103.366659532388));
#78076=CARTESIAN_POINT('Ctrl Pts',(60.6462367344819,734.089804826984,103.385276064217));
#78077=CARTESIAN_POINT('Ctrl Pts',(60.5779754381771,733.934622540943,103.4157764696));
#78078=CARTESIAN_POINT('Ctrl Pts',(60.5492824792608,733.872619393186,103.427884070048));
#78079=CARTESIAN_POINT('Ctrl Pts',(60.5057507842612,733.783010299744,103.44528574064));
#78080=CARTESIAN_POINT('Ctrl Pts',(60.4918352280297,733.754981403043,103.450714514658));
#78081=CARTESIAN_POINT('Ctrl Pts',(60.4457279638996,733.664072444659,103.468275193877));
#78082=CARTESIAN_POINT('Ctrl Pts',(60.4125546154033,733.601679353953,103.480254800349));
#78083=CARTESIAN_POINT('Ctrl Pts',(60.323194734268,733.441055008029,103.510868758104));
#78084=CARTESIAN_POINT('Ctrl Pts',(60.2652170234325,733.343914031774,103.529162067083));
#78085=CARTESIAN_POINT('Ctrl Pts',(60.0834842500503,733.05878163104,103.581795960366));
#78086=CARTESIAN_POINT('Ctrl Pts',(59.9521350216947,732.876983742758,103.613928489012));
#78087=CARTESIAN_POINT('Ctrl Pts',(59.6261861561843,732.470798745779,103.678791567783));
#78088=CARTESIAN_POINT('Ctrl Pts',(59.4281892680164,732.254744633062,103.707859181998));
#78089=CARTESIAN_POINT('Ctrl Pts',(59.2182845115635,732.044714413234,103.72736082686));
#78090=CARTESIAN_POINT('',(60.8878641387277,736.917077965099,104.196518950431));
#78091=CARTESIAN_POINT('Origin',(60.1807573575412,736.984851146654,103.492667548598));
#78092=CARTESIAN_POINT('Origin',(52.8776183915471,736.917077965099,104.196518950431));
#78093=CARTESIAN_POINT('Origin',(52.8776183915471,750.796902408053,107.247996346823));
#78094=CARTESIAN_POINT('',(61.1807573575412,751.190390849763,103.161460105204));
#78095=CARTESIAN_POINT('',(61.1807573575412,751.59614455564,98.947549280963));
#78096=CARTESIAN_POINT('',(61.1807573575412,750.796902408053,107.247996346823));
#78097=CARTESIAN_POINT('',(44.574479425553,751.59614455564,98.947549280963));
#78098=CARTESIAN_POINT('Origin',(52.8776183915471,751.59614455564,98.947549280963));
#78099=CARTESIAN_POINT('',(44.574479425553,750.796902408053,107.247996346823));
#78100=CARTESIAN_POINT('',(61.1807573575412,751.028294523684,104.84489734479));
#78101=CARTESIAN_POINT('Origin',(52.8776183915471,751.028294523684,104.84489734479));
#78102=CARTESIAN_POINT('',(61.1807573575412,750.796902408053,107.247996346823));
#78103=CARTESIAN_POINT('Origin',(52.8776183915471,736.753459031024,105.895766550631));
#78104=CARTESIAN_POINT('',(44.9102331003523,734.658332041414,103.268620312408));
#78105=CARTESIAN_POINT('Ctrl Pts',(44.5744794255595,737.051924855535,102.796188898326));
#78106=CARTESIAN_POINT('Ctrl Pts',(44.5744791286989,736.807354199727,102.86204099027));
#78107=CARTESIAN_POINT('Ctrl Pts',(44.5834464915899,736.379766761261,102.933369831913));
#78108=CARTESIAN_POINT('Ctrl Pts',(44.7152766932813,735.441353648989,103.107028422208));
#78109=CARTESIAN_POINT('Ctrl Pts',(44.7992091262746,735.046632082973,103.184616559007));
#78110=CARTESIAN_POINT('Ctrl Pts',(44.9102335588522,734.658333245328,103.268591502399));
#78111=CARTESIAN_POINT('Origin',(52.8776183915471,736.984851146654,103.492667548598));
#78112=CARTESIAN_POINT('Origin',(61.1807573575412,750.796902408053,107.247996346823));
#78113=CARTESIAN_POINT('',(61.1807573575412,737.487748923763,102.682654164686));
#78114=CARTESIAN_POINT('',(61.1807605165803,740.123621968703,102.670910437332));
#78115=CARTESIAN_POINT('',(61.1807573575412,737.487748923763,102.682654164686));
#78116=CARTESIAN_POINT('Ctrl Pts',(61.1807586638608,740.12361543648,102.669195273733));
#78117=CARTESIAN_POINT('Ctrl Pts',(61.1807560496647,741.047936554133,102.664564349666));
#78118=CARTESIAN_POINT('Ctrl Pts',(61.1807573574534,741.972239121777,102.661547405019));
#78119=CARTESIAN_POINT('Ctrl Pts',(61.180757357629,742.89597670391,102.67056249796));
#78120=CARTESIAN_POINT('Ctrl Pts',(61.1807573576322,742.912710422517,102.67072580844));
#78121=CARTESIAN_POINT('Ctrl Pts',(61.1807573576353,742.929443959488,102.670893055289));
#78122=CARTESIAN_POINT('Ctrl Pts',(61.1807573576383,742.946177311763,102.671064307693));
#78123=CARTESIAN_POINT('Ctrl Pts',(61.1807573578003,743.853161319358,102.680346559628));
#78124=CARTESIAN_POINT('Ctrl Pts',(61.1807573561954,744.759591967292,102.701437959504));
#78125=CARTESIAN_POINT('Ctrl Pts',(61.1807573589444,745.665256166094,102.738838654994));
#78126=CARTESIAN_POINT('Ctrl Pts',(61.1807573591155,745.721625214061,102.74116649527));
#78127=CARTESIAN_POINT('Ctrl Pts',(61.1807573592889,745.777991366072,102.743557133276));
#78128=CARTESIAN_POINT('Ctrl Pts',(61.1807573594589,745.834354568082,102.746011643787));
#78129=CARTESIAN_POINT('Ctrl Pts',(61.1807573641388,747.38638228969,102.813599506415));
#78130=CARTESIAN_POINT('Ctrl Pts',(61.1807573577533,748.936047138209,102.931108441007));
#78131=CARTESIAN_POINT('Ctrl Pts',(61.1807573575642,750.483918388405,103.087438878833));
#78132=CARTESIAN_POINT('Ctrl Pts',(61.1807573575354,750.719450082243,103.111226886276));
#78133=CARTESIAN_POINT('Ctrl Pts',(61.1807573575412,750.95494017589,103.135913703081));
#78134=CARTESIAN_POINT('Ctrl Pts',(61.1807573575412,751.190390600116,103.161460144679));
#78135=CARTESIAN_POINT('',(61.1807573575412,736.984851146654,103.492667548599));
#78136=CARTESIAN_POINT('Ctrl Pts',(61.180829512521,737.051935013493,102.795969534154));
#78137=CARTESIAN_POINT('Ctrl Pts',(61.180808006567,737.148389738621,102.770016804829));
#78138=CARTESIAN_POINT('Ctrl Pts',(61.1807835398961,737.244967673439,102.744516726847));
#78139=CARTESIAN_POINT('Ctrl Pts',(61.1807690759748,737.341710445985,102.719649607981));
#78140=CARTESIAN_POINT('Ctrl Pts',(61.1807626840078,737.384463486494,102.708660208853));
#78141=CARTESIAN_POINT('Ctrl Pts',(61.1807584586882,737.427248534081,102.697795029881));
#78142=CARTESIAN_POINT('Ctrl Pts',(61.1807575470676,737.470068261744,102.687072865374));
#78143=CARTESIAN_POINT('Ctrl Pts',(61.1807574216098,737.475961142441,102.685597273639));
#78144=CARTESIAN_POINT('Ctrl Pts',(61.1807573575412,737.481855369893,102.684127065464));
#78145=CARTESIAN_POINT('Ctrl Pts',(61.1807573575412,737.487748923763,102.682654164686));
#78146=CARTESIAN_POINT('Origin',(52.8776183915471,750.796902408053,107.247996346823));
#78147=CARTESIAN_POINT('',(46.9886929879261,750.796902408053,107.247996346823));
#78148=CARTESIAN_POINT('',(46.9886929879261,736.753459031024,105.895766550631));
#78149=CARTESIAN_POINT('',(46.9886929879261,750.796902408053,107.247996346823));
#78150=CARTESIAN_POINT('',(58.7665437951681,736.753459031024,105.895766550631));
#78151=CARTESIAN_POINT('Origin',(52.8776183915471,736.753459031024,105.895766550631));
#78152=CARTESIAN_POINT('',(58.7665437951681,750.796902408053,107.247996346823));
#78153=CARTESIAN_POINT('',(58.7665437951681,750.796902408053,107.247996346823));
#78154=CARTESIAN_POINT('Origin',(52.8776183915471,750.796902408053,107.247996346823));
#78155=CARTESIAN_POINT('Origin',(59.1807573575412,750.796902408053,107.247996346823));
#78156=CARTESIAN_POINT('',(59.4736505763546,750.824974979019,106.956451550289));
#78157=CARTESIAN_POINT('',(60.8878641387277,750.960521342129,105.548748746623));
#78158=CARTESIAN_POINT('',(59.1807573575412,750.796902408053,107.247996346823));
#78159=CARTESIAN_POINT('',(59.4736505763546,736.781531601989,105.604221754097));
#78160=CARTESIAN_POINT('',(59.4736505763546,750.824974979019,106.956451550289));
#78161=CARTESIAN_POINT('',(61.1807573575412,736.945150536064,103.904974153897));
#78162=CARTESIAN_POINT('',(60.8878641387277,750.960521342129,105.548748746623));
#78163=CARTESIAN_POINT('Origin',(52.8776183915471,750.796902408053,107.247996346823));
#78164=CARTESIAN_POINT('',(46.2815862067395,750.824974979019,106.956451550289));
#78165=CARTESIAN_POINT('',(44.8673726443664,750.960521342129,105.548748746623));
#78166=CARTESIAN_POINT('',(46.574479425553,750.796902408053,107.247996346823));
#78167=CARTESIAN_POINT('Origin',(52.8776183915471,750.824974979019,106.956451550289));
#78168=CARTESIAN_POINT('Origin',(52.8776183915471,750.960521342129,105.548748746623));
#78169=CARTESIAN_POINT('Origin',(52.8776183915471,736.753459031024,105.895766550631));
#78170=CARTESIAN_POINT('',(58.3219300063767,731.218651083621,103.766631312401));
#78171=CARTESIAN_POINT('Ctrl Pts',(59.2182826984074,732.044716514228,103.727363937984));
#78172=CARTESIAN_POINT('Ctrl Pts',(59.1410053172168,731.967395409693,103.734545295664));
#78173=CARTESIAN_POINT('Ctrl Pts',(59.0625975079218,731.891133513513,103.741163687107));
#78174=CARTESIAN_POINT('Ctrl Pts',(58.9833028731213,731.815787977957,103.746880332788));
#78175=CARTESIAN_POINT('Ctrl Pts',(58.9043155133724,731.740734414278,103.752574825866));
#78176=CARTESIAN_POINT('Ctrl Pts',(58.8244484793124,731.666589906708,103.757374527535));
#78177=CARTESIAN_POINT('Ctrl Pts',(58.7439078609761,731.59317536338,103.76094093225));
#78178=CARTESIAN_POINT('Ctrl Pts',(58.6638424024685,731.520193938676,103.764486296498));
#78179=CARTESIAN_POINT('Ctrl Pts',(58.5831115382727,731.447933633485,103.766812848102));
#78180=CARTESIAN_POINT('Ctrl Pts',(58.5018793316936,731.376184532491,103.76758476604));
#78181=CARTESIAN_POINT('Ctrl Pts',(58.4421511530334,731.323429063898,103.768152339598));
#78182=CARTESIAN_POINT('Ctrl Pts',(58.3821511559648,731.270949246123,103.767879358289));
#78183=CARTESIAN_POINT('Ctrl Pts',(58.3219300063767,731.218651083621,103.766631312401));
#78184=CARTESIAN_POINT('',(46.2815862067395,736.781531601989,105.604221754097));
#78185=CARTESIAN_POINT('Origin',(52.8776183915471,736.781531601989,105.604221754097));
#78186=CARTESIAN_POINT('',(44.8673726443664,736.917077965099,104.196518950431));
#78187=CARTESIAN_POINT('',(44.574479425553,736.945150536064,103.904974153897));
#78188=CARTESIAN_POINT('',(46.5369840943911,732.044637214649,103.727329693178));
#78189=CARTESIAN_POINT('Origin',(52.8776183915471,736.917077965099,104.196518950431));
#78190=CARTESIAN_POINT('',(47.4333208409147,731.218654873935,103.766631507277));
#78191=CARTESIAN_POINT('Ctrl Pts',(47.4333199694293,731.218655630363,103.766645149501));
#78192=CARTESIAN_POINT('Ctrl Pts',(47.2825110232573,731.349638140042,103.769783701346));
#78193=CARTESIAN_POINT('Ctrl Pts',(47.1293091961631,731.484318580969,103.766191622297));
#78194=CARTESIAN_POINT('Ctrl Pts',(46.8277456416006,731.760758895609,103.751646950206));
#78195=CARTESIAN_POINT('Ctrl Pts',(46.6809723070849,731.900553502369,103.7406976256));
#78196=CARTESIAN_POINT('Ctrl Pts',(46.5369645910256,732.044621808575,103.727301634748));
#78197=CARTESIAN_POINT('Ctrl Pts',(58.3219249040931,731.21864665262,103.766631206657));
#78198=CARTESIAN_POINT('Ctrl Pts',(58.2440956171014,731.151056992137,103.765018172219));
#78199=CARTESIAN_POINT('Ctrl Pts',(58.1647207776151,731.084673275731,103.763443633293));
#78200=CARTESIAN_POINT('Ctrl Pts',(58.084094661515,731.019772305155,103.761912350037));
#78201=CARTESIAN_POINT('Ctrl Pts',(58.0034573035392,730.954862285294,103.760380853271));
#78202=CARTESIAN_POINT('Ctrl Pts',(57.92156855916,730.891435630024,103.758892624238));
#78203=CARTESIAN_POINT('Ctrl Pts',(57.8387558587535,730.82972881865,103.75745242509));
#78204=CARTESIAN_POINT('Ctrl Pts',(57.8050394303558,730.804605458621,103.756866061269));
#78205=CARTESIAN_POINT('Ctrl Pts',(57.7711702037205,730.779766703224,103.756287659056));
#78206=CARTESIAN_POINT('Ctrl Pts',(57.7371716948611,730.755226485564,103.755717539843));
#78207=CARTESIAN_POINT('Ctrl Pts',(57.6043222460252,730.659335386223,103.753489794402));
#78208=CARTESIAN_POINT('Ctrl Pts',(57.4691061887164,730.567711554512,103.75138016625));
#78209=CARTESIAN_POINT('Ctrl Pts',(57.3315633396149,730.480289249374,103.7493829085));
#78210=CARTESIAN_POINT('Ctrl Pts',(57.261007256714,730.435443767046,103.748358364626));
#78211=CARTESIAN_POINT('Ctrl Pts',(57.1898382886597,730.391704490583,103.74736339031));
#78212=CARTESIAN_POINT('Ctrl Pts',(57.1180583559394,730.349066580572,103.7463972098));
#78213=CARTESIAN_POINT('Ctrl Pts',(56.9774193116041,730.26552575392,103.744504163952));
#78214=CARTESIAN_POINT('Ctrl Pts',(56.8344421594333,730.1862135713,103.742720926515));
#78215=CARTESIAN_POINT('Ctrl Pts',(56.6891216129092,730.111126398369,103.741044697022));
#78216=CARTESIAN_POINT('Ctrl Pts',(56.5430260983871,730.035638799226,103.739359528502));
#78217=CARTESIAN_POINT('Ctrl Pts',(56.3945615921378,729.964421061701,103.737782512277));
#78218=CARTESIAN_POINT('Ctrl Pts',(56.2437010615264,729.897518087519,103.736310802839));
#78219=CARTESIAN_POINT('Ctrl Pts',(56.092840530915,729.830615113337,103.7348390934));
#78220=CARTESIAN_POINT('Ctrl Pts',(55.9395833889696,729.768026641657,103.733472690748));
#78221=CARTESIAN_POINT('Ctrl Pts',(55.7838894679809,729.709850421025,103.732208749374));
#78222=CARTESIAN_POINT('Ctrl Pts',(55.6765488700272,729.669741788205,103.731337345904));
#78223=CARTESIAN_POINT('Ctrl Pts',(55.5682311649451,729.631805000722,103.730517048397));
#78224=CARTESIAN_POINT('Ctrl Pts',(55.4593025183271,729.596169629469,103.729748945441));
#78225=CARTESIAN_POINT('Ctrl Pts',(55.3502206571051,729.560484134952,103.728979762102));
#78226=CARTESIAN_POINT('Ctrl Pts',(55.2405264652308,729.527106629751,103.728262920248));
#78227=CARTESIAN_POINT('Ctrl Pts',(55.1306025848533,729.496117118348,103.727599513066));
#78228=CARTESIAN_POINT('Ctrl Pts',(55.1118928282375,729.490842502733,103.727486596866));
#78229=CARTESIAN_POINT('Ctrl Pts',(55.0931764455505,729.485636948906,103.727375228681));
#78230=CARTESIAN_POINT('Ctrl Pts',(55.074455355652,729.480500704696,103.727265413902));
#78231=CARTESIAN_POINT('Ctrl Pts',(54.9159162785624,729.437004550303,103.726335450221));
#78232=CARTESIAN_POINT('Ctrl Pts',(54.7565538689342,729.398340894392,103.725512891532));
#78233=CARTESIAN_POINT('Ctrl Pts',(54.5963803385134,729.364450698395,103.724794379583));
#78234=CARTESIAN_POINT('Ctrl Pts',(54.5155470402871,729.34734764577,103.724431774786));
#78235=CARTESIAN_POINT('Ctrl Pts',(54.4345068451812,729.331461078676,103.724095668872));
#78236=CARTESIAN_POINT('Ctrl Pts',(54.3532597720157,729.316788196599,103.723785630211));
#78237=CARTESIAN_POINT('Ctrl Pts',(54.1931230587091,729.287868175004,103.72317454885));
#78238=CARTESIAN_POINT('Ctrl Pts',(54.0321913209344,729.263661319254,103.722663775038));
#78239=CARTESIAN_POINT('Ctrl Pts',(53.8704525191743,729.244181911624,103.72225375967));
#78240=CARTESIAN_POINT('Ctrl Pts',(53.706657913141,729.224454908186,103.721838532742));
#78241=CARTESIAN_POINT('Ctrl Pts',(53.5420349654433,729.20957610299,103.721526641947));
#78242=CARTESIAN_POINT('Ctrl Pts',(53.3765697975624,729.199614985232,103.721318555591));
#78243=CARTESIAN_POINT('Ctrl Pts',(53.2111046296815,729.189653867473,103.721110469236));
#78244=CARTESIAN_POINT('Ctrl Pts',(53.0447965770304,729.184610396008,103.721006187319));
#78245=CARTESIAN_POINT('Ctrl Pts',(52.8776401587059,729.184609957798,103.721006178149));
#78246=CARTESIAN_POINT('Ctrl Pts',(52.7137023104169,729.184609528025,103.721006169156));
#78247=CARTESIAN_POINT('Ctrl Pts',(52.5505758965974,729.189460030891,103.721106467457));
#78248=CARTESIAN_POINT('Ctrl Pts',(52.3882588644791,729.199043117555,103.721306625593));
#78249=CARTESIAN_POINT('Ctrl Pts',(52.2222003373688,729.208847099526,103.721511397481));
#78250=CARTESIAN_POINT('Ctrl Pts',(52.0569883213915,729.223604188265,103.721820685908));
#78251=CARTESIAN_POINT('Ctrl Pts',(51.8926120674172,729.243242920974,103.722234011753));
#78252=CARTESIAN_POINT('Ctrl Pts',(51.7282358134428,729.262881653682,103.722647337599));
#78253=CARTESIAN_POINT('Ctrl Pts',(51.564694672195,729.287402108584,103.723164700862));
#78254=CARTESIAN_POINT('Ctrl Pts',(51.4019790523234,729.316787827959,103.723785622422));
#78255=CARTESIAN_POINT('Ctrl Pts',(51.2409737783516,729.34586466645,103.724400017315));
#78256=CARTESIAN_POINT('Ctrl Pts',(51.0807815335725,729.379704317724,103.725116773544));
#78257=CARTESIAN_POINT('Ctrl Pts',(50.9214059654977,729.418340665856,103.725939243923));
#78258=CARTESIAN_POINT('Ctrl Pts',(50.8409931639961,729.437834601035,103.726354220623));
#78259=CARTESIAN_POINT('Ctrl Pts',(50.7607884800892,729.458550422199,103.726796108954));
#78260=CARTESIAN_POINT('Ctrl Pts',(50.680794100972,729.480497227648,103.727265339561));
#78261=CARTESIAN_POINT('Ctrl Pts',(50.5704196242906,729.51077894485,103.727912773585));
#78262=CARTESIAN_POINT('Ctrl Pts',(50.4602121832636,729.543473259537,103.72861418246));
#78263=CARTESIAN_POINT('Ctrl Pts',(50.3505563395933,729.578509132596,103.729368495549));
#78264=CARTESIAN_POINT('Ctrl Pts',(50.2410631623908,729.613493032486,103.73012168967));
#78265=CARTESIAN_POINT('Ctrl Pts',(50.1321202807258,729.650811465402,103.730927631162));
#78266=CARTESIAN_POINT('Ctrl Pts',(50.0240965575535,729.690343596891,103.731785254144));
#78267=CARTESIAN_POINT('Ctrl Pts',(50.0064974381545,729.696784133116,103.731924977242));
#78268=CARTESIAN_POINT('Ctrl Pts',(49.9889226791992,729.703283320467,103.732066072102));
#78269=CARTESIAN_POINT('Ctrl Pts',(49.9713738312623,729.709840513116,103.732208534114));
#78270=CARTESIAN_POINT('Ctrl Pts',(49.8177009328862,729.767260966198,103.733456054769));
#78271=CARTESIAN_POINT('Ctrl Pts',(49.6664031093005,729.828979546795,103.734803384278));
#78272=CARTESIAN_POINT('Ctrl Pts',(49.5174415848815,729.894901729426,103.736253254073));
#78273=CARTESIAN_POINT('Ctrl Pts',(49.365930849862,729.961952052545,103.737727935801));
#78274=CARTESIAN_POINT('Ctrl Pts',(49.2168364407443,730.033351192812,103.739308697432));
#78275=CARTESIAN_POINT('Ctrl Pts',(49.0701306934366,730.109052960563,103.740998413044));
#78276=CARTESIAN_POINT('Ctrl Pts',(48.9234249461288,730.184754728315,103.742688128655));
#78277=CARTESIAN_POINT('Ctrl Pts',(48.7791072888848,730.264759419022,103.744486798248));
#78278=CARTESIAN_POINT('Ctrl Pts',(48.6371720308017,730.349070380066,103.746397295897));
#78279=CARTESIAN_POINT('Ctrl Pts',(48.4972332733578,730.432195399787,103.748280919957));
#78280=CARTESIAN_POINT('Ctrl Pts',(48.3596156778622,730.519503358546,103.750273968768));
#78281=CARTESIAN_POINT('Ctrl Pts',(48.2243412484543,730.611039789433,103.752382185054));
#78282=CARTESIAN_POINT('Ctrl Pts',(48.154963352582,730.657985875241,103.753463421254));
#78283=CARTESIAN_POINT('Ctrl Pts',(48.0862022998346,730.706044851327,103.754574950341));
#78284=CARTESIAN_POINT('Ctrl Pts',(48.0180646604849,730.755226794314,103.755717547016));
#78285=CARTESIAN_POINT('Ctrl Pts',(47.9345157570287,730.815532631816,103.757118574411));
#78286=CARTESIAN_POINT('Ctrl Pts',(47.8517492715001,730.877644568796,103.758569627446));
#78287=CARTESIAN_POINT('Ctrl Pts',(47.77010514203,730.941343414278,103.760065946964));
#78288=CARTESIAN_POINT('Ctrl Pts',(47.6884928602638,731.005017412145,103.761561682797));
#78289=CARTESIAN_POINT('Ctrl Pts',(47.6080023160632,731.070276898363,103.763102649804));
#78290=CARTESIAN_POINT('Ctrl Pts',(47.5289415695104,731.136861352564,103.764684094393));
#78291=CARTESIAN_POINT('Ctrl Pts',(47.4968230726771,731.163911344812,103.765326557628));
#78292=CARTESIAN_POINT('Ctrl Pts',(47.4649401663363,731.191179547578,103.765975701273));
#78293=CARTESIAN_POINT('Ctrl Pts',(47.4333118811382,731.218646650764,103.766631206613));
#78294=CARTESIAN_POINT('Origin',(46.574479425553,750.796902408053,107.247996346823));
#78295=CARTESIAN_POINT('',(46.2815862067395,750.824974979019,106.956451550289));
#78296=CARTESIAN_POINT('',(44.8673726443664,736.917077965099,104.196518950431));
#78297=CARTESIAN_POINT('Origin',(52.8776183915471,750.892748160574,106.252600148456));
#78298=CARTESIAN_POINT('Origin',(58.7665437951681,750.892748160574,106.252600148456));
#78299=CARTESIAN_POINT('Origin',(46.9886929879261,750.892748160574,106.252600148456));
#78300=CARTESIAN_POINT('Origin',(46.9886929879261,750.892748160574,106.252600148456));
#78301=CARTESIAN_POINT('Origin',(46.9886929879261,736.849304783544,104.900370352264));
#78302=CARTESIAN_POINT('Origin',(58.7665437951681,750.892748160574,106.252600148456));
#78303=CARTESIAN_POINT('Origin',(58.7665437951681,736.849304783544,104.900370352264));
#78304=CARTESIAN_POINT('Origin',(52.8776183915471,736.849304783544,104.900370352264));
#78305=CARTESIAN_POINT('Origin',(52.8776183915471,736.984851146654,103.492667548598));
#78306=CARTESIAN_POINT('Ctrl Pts',(46.5369645921949,732.044621809289,103.727301632047));
#78307=CARTESIAN_POINT('Ctrl Pts',(46.3225264216533,732.259153081262,103.707349715149));
#78308=CARTESIAN_POINT('Ctrl Pts',(46.1205233504414,732.480034869399,103.677463263573));
#78309=CARTESIAN_POINT('Ctrl Pts',(45.7933717648021,732.89018316908,103.611665037245));
#78310=CARTESIAN_POINT('Ctrl Pts',(45.664030910038,733.070178870018,103.579805976886));
#78311=CARTESIAN_POINT('Ctrl Pts',(45.4855803385425,733.351362146652,103.527862348267));
#78312=CARTESIAN_POINT('Ctrl Pts',(45.4289758251606,733.446475095519,103.509933886774));
#78313=CARTESIAN_POINT('Ctrl Pts',(45.3415828623108,733.603808834803,103.479938974266));
#78314=CARTESIAN_POINT('Ctrl Pts',(45.3090974516336,733.6649463005,103.468193759419));
#78315=CARTESIAN_POINT('Ctrl Pts',(45.2638137275495,733.754201624595,103.450940497582));
#78316=CARTESIAN_POINT('Ctrl Pts',(45.2500770414093,733.781852806832,103.445580763039));
#78317=CARTESIAN_POINT('Ctrl Pts',(45.2066141899079,733.871237044652,103.42820896964));
#78318=CARTESIAN_POINT('Ctrl Pts',(45.1778247696134,733.933397521809,103.416059205064));
#78319=CARTESIAN_POINT('Ctrl Pts',(45.1085970074955,734.090669669677,103.385121922763));
#78320=CARTESIAN_POINT('Ctrl Pts',(45.0696884673827,734.186463068881,103.36611067962));
#78321=CARTESIAN_POINT('Ctrl Pts',(44.9876931506015,734.406729887678,103.321673608498));
#78322=CARTESIAN_POINT('Ctrl Pts',(44.946241754629,734.532389344382,103.295830687479));
#78323=CARTESIAN_POINT('Ctrl Pts',(44.9102342133583,734.658330962292,103.268591994624));
#78324=CARTESIAN_POINT('Origin',(45.574479425553,736.984851146654,103.492667548598));
#78325=CARTESIAN_POINT('Origin',(45.574479425553,751.028294523684,104.84489734479));
#78326=CARTESIAN_POINT('Origin',(45.574479425553,751.028294523684,104.84489734479));
#78327=CARTESIAN_POINT('Origin',(60.1807573575412,751.028294523684,104.84489734479));
#78328=CARTESIAN_POINT('Origin',(60.1807573575412,751.028294523684,104.84489734479));
#78329=CARTESIAN_POINT('Origin',(52.8776183915471,751.028294523684,104.84489734479));
#78330=CARTESIAN_POINT('Ctrl Pts',(44.574479425553,739.297010529679,102.671020968754));
#78331=CARTESIAN_POINT('Ctrl Pts',(44.5744794255741,739.29810258077,103.433937572034));
#78332=CARTESIAN_POINT('Ctrl Pts',(43.8749449432361,739.298063899118,103.129485841296));
#78333=CARTESIAN_POINT('Ctrl Pts',(44.574479425553,740.530857021924,102.667286233968));
#78334=CARTESIAN_POINT('Ctrl Pts',(44.5744794255372,740.537828296885,103.430114647369));
#78335=CARTESIAN_POINT('Ctrl Pts',(43.874983425004,740.533976463203,103.125741677408));
#78336=CARTESIAN_POINT('Ctrl Pts',(44.574479425553,741.764892155927,102.658402212418));
#78337=CARTESIAN_POINT('Ctrl Pts',(44.5744794255229,741.762501809108,103.421959943614));
#78338=CARTESIAN_POINT('Ctrl Pts',(43.8746011421895,741.765219958194,103.116745243982));
#78339=CARTESIAN_POINT('Ctrl Pts',(44.574479425553,743.955576229434,102.681842604063));
#78340=CARTESIAN_POINT('Ctrl Pts',(44.5744794255763,743.938984899097,103.440683584674));
#78341=CARTESIAN_POINT('Ctrl Pts',(43.8771264840893,743.946601258126,103.141178205667));
#78342=CARTESIAN_POINT('Ctrl Pts',(44.574479425553,744.912616217256,102.705438138897));
#78343=CARTESIAN_POINT('Ctrl Pts',(44.574479425553,744.883170807362,103.459905019968));
#78344=CARTESIAN_POINT('Ctrl Pts',(43.8793242348887,744.898138964526,103.165604660246));
#78345=CARTESIAN_POINT('Ctrl Pts',(44.574479425553,748.056063398855,102.843629112592));
#78346=CARTESIAN_POINT('Ctrl Pts',(44.574479425553,747.973884049545,103.575040888373));
#78347=CARTESIAN_POINT('Ctrl Pts',(43.8912182783842,748.022533230734,103.307895376711));
#78348=CARTESIAN_POINT('Ctrl Pts',(44.5744794255529,750.238556260715,103.039162325259));
#78349=CARTESIAN_POINT('Ctrl Pts',(44.5744794256417,750.101103921648,103.736030596296));
#78350=CARTESIAN_POINT('Ctrl Pts',(43.9071717466752,750.190640286152,103.508440148698));
#78351=CARTESIAN_POINT('Ctrl Pts',(44.574479425553,752.418162461714,103.302274539183));
#78352=CARTESIAN_POINT('Ctrl Pts',(44.5744794255157,752.338363272777,103.97656838147));
#78353=CARTESIAN_POINT('Ctrl Pts',(43.9260235934534,752.361394691197,103.776329042103));
#78354=CARTESIAN_POINT('',(43.8763887996152,740.125375114458,103.127134598756));
#78355=CARTESIAN_POINT('Origin',(44.074479425553,740.123635038617,102.66805173472));
#78356=CARTESIAN_POINT('',(44.574479425553,751.59614455564,103.206327301003));
#78357=CARTESIAN_POINT('Ctrl Pts',(44.574479425553,751.59614455564,103.206327301003));
#78358=CARTESIAN_POINT('Ctrl Pts',(44.574479425553,751.460907273987,103.19109258465));
#78359=CARTESIAN_POINT('Ctrl Pts',(44.574479425553,751.325656135411,103.176133022638));
#78360=CARTESIAN_POINT('Ctrl Pts',(44.574479425553,751.190391221941,103.161456281541));
#78361=CARTESIAN_POINT('',(43.9196965836671,751.54292215966,103.678777984592));
#78362=CARTESIAN_POINT('Origin',(44.074479425553,751.59614455564,103.206327301003));
#78363=CARTESIAN_POINT('Ctrl Pts',(43.8763918793368,740.125375235339,103.127136791686));
#78364=CARTESIAN_POINT('Ctrl Pts',(43.8761609839388,740.382537008607,103.12606196984));
#78365=CARTESIAN_POINT('Ctrl Pts',(43.8760246822405,740.639656652116,103.12503062257));
#78366=CARTESIAN_POINT('Ctrl Pts',(43.8759483580193,740.896786009906,103.124321807132));
#78367=CARTESIAN_POINT('Ctrl Pts',(43.8758735861635,741.14868559011,103.123627408357));
#78368=CARTESIAN_POINT('Ctrl Pts',(43.8758561270906,741.400594538677,103.12324269677));
#78369=CARTESIAN_POINT('Ctrl Pts',(43.8758880528351,741.652523518746,103.123411688851));
#78370=CARTESIAN_POINT('Ctrl Pts',(43.8759192074444,741.898367399276,103.123576599093));
#78371=CARTESIAN_POINT('Ctrl Pts',(43.8759972035132,742.144230284881,103.12426888698));
#78372=CARTESIAN_POINT('Ctrl Pts',(43.8761415145388,742.390085708688,103.12569590925));
#78373=CARTESIAN_POINT('Ctrl Pts',(43.8762581050598,742.588715105541,103.126848816794));
#78374=CARTESIAN_POINT('Ctrl Pts',(43.876418424685,742.787338947153,103.128480971918));
#78375=CARTESIAN_POINT('Ctrl Pts',(43.8766472931601,742.985925842393,103.130691443671));
#78376=CARTESIAN_POINT('Ctrl Pts',(43.8769322533183,743.233182932084,103.13344366361));
#78377=CARTESIAN_POINT('Ctrl Pts',(43.8773287442974,743.480413177981,103.137095886245));
#78378=CARTESIAN_POINT('Ctrl Pts',(43.8777960574979,743.727640306692,103.141770103925));
#78379=CARTESIAN_POINT('Ctrl Pts',(43.8782647951713,743.975621037748,103.146458569643));
#78380=CARTESIAN_POINT('Ctrl Pts',(43.8788046918661,744.223598486502,103.152175306106));
#78381=CARTESIAN_POINT('Ctrl Pts',(43.8794071456804,744.471561541077,103.159021276459));
#78382=CARTESIAN_POINT('Ctrl Pts',(43.8800141469592,744.721396279667,103.165918921822));
#78383=CARTESIAN_POINT('Ctrl Pts',(43.880684554495,744.97121626136,103.173962947854));
#78384=CARTESIAN_POINT('Ctrl Pts',(43.881444002068,745.220976746973,103.183233610531));
#78385=CARTESIAN_POINT('Ctrl Pts',(43.8820768967054,745.429117608275,103.190959427165));
#78386=CARTESIAN_POINT('Ctrl Pts',(43.8827722350252,745.637216499217,103.199536718816));
#78387=CARTESIAN_POINT('Ctrl Pts',(43.8835635166994,745.84523122278,103.208999702177));
#78388=CARTESIAN_POINT('Ctrl Pts',(43.8846113185723,746.1206808181,103.221530425449));
#78389=CARTESIAN_POINT('Ctrl Pts',(43.8858848744824,746.395912657287,103.23563536325));
#78390=CARTESIAN_POINT('Ctrl Pts',(43.88729096164,746.671006938799,103.251288589859));
#78391=CARTESIAN_POINT('Ctrl Pts',(43.8887485706763,746.956181231446,103.267515382366));
#78392=CARTESIAN_POINT('Ctrl Pts',(43.8903487160162,747.241207475621,103.285405858764));
#78393=CARTESIAN_POINT('Ctrl Pts',(43.8920261956294,747.52613890873,103.304907908265));
#78394=CARTESIAN_POINT('Ctrl Pts',(43.8937725314076,747.822766034346,103.325210466056));
#78395=CARTESIAN_POINT('Ctrl Pts',(43.8956028269719,748.119290175308,103.34725943002));
#78396=CARTESIAN_POINT('Ctrl Pts',(43.8974826562651,748.415736514845,103.370973860377));
#78397=CARTESIAN_POINT('Ctrl Pts',(43.8994982690507,748.733595713221,103.396401227217));
#78398=CARTESIAN_POINT('Ctrl Pts',(43.9015708694549,749.05136534484,103.4237431833));
#78399=CARTESIAN_POINT('Ctrl Pts',(43.9037009210375,749.369039730519,103.452877636005));
#78400=CARTESIAN_POINT('Ctrl Pts',(43.9059365213006,749.702455571738,103.483455764097));
#78401=CARTESIAN_POINT('Ctrl Pts',(43.9082357098795,750.035766184794,103.516008089841));
#78402=CARTESIAN_POINT('Ctrl Pts',(43.9106417524483,750.368929551215,103.55037389145));
#78403=CARTESIAN_POINT('Ctrl Pts',(43.9132468091299,750.729650290319,103.58758223608));
#78404=CARTESIAN_POINT('Ctrl Pts',(43.9159773869033,751.090198191152,103.626916043815));
#78405=CARTESIAN_POINT('Ctrl Pts',(43.9189330996857,751.450483445277,103.668154957693));
#78406=CARTESIAN_POINT('Ctrl Pts',(43.9191858990892,751.481298312631,103.671682084176));
#78407=CARTESIAN_POINT('Ctrl Pts',(43.9194403687895,751.512111239579,103.675223140215));
#78408=CARTESIAN_POINT('Ctrl Pts',(43.9196965836671,751.54292215966,103.678777984592));
#78409=CARTESIAN_POINT('Ctrl Pts',(44.5744794255529,751.59614455564,103.206327301003));
#78410=CARTESIAN_POINT('Ctrl Pts',(44.5744794255529,751.519059169342,103.890607720566));
#78411=CARTESIAN_POINT('Ctrl Pts',(43.9196965836671,751.54292215966,103.678777984592));
#78412=CARTESIAN_POINT('Ctrl Pts',(44.5744794255529,752.148115347472,103.272252174199));
#78413=CARTESIAN_POINT('Ctrl Pts',(44.5694175928971,752.047430714789,103.941138173534));
#78414=CARTESIAN_POINT('Ctrl Pts',(43.9245398403207,752.125343909066,103.745975546382));
#78415=CARTESIAN_POINT('Ctrl Pts',(44.6288816340649,752.687363884647,103.360500944369));
#78416=CARTESIAN_POINT('Ctrl Pts',(44.6138450657875,752.573635763871,104.010544030293));
#78417=CARTESIAN_POINT('Ctrl Pts',(43.9880971321887,752.695085898244,103.83582173207));
#78418=CARTESIAN_POINT('Ctrl Pts',(44.786533250981,753.480032342672,103.51306294943));
#78419=CARTESIAN_POINT('Ctrl Pts',(44.759884698206,753.364651507361,104.137065762323));
#78420=CARTESIAN_POINT('Ctrl Pts',(44.1649153929541,753.533629601795,103.990943559498));
#78421=CARTESIAN_POINT('Ctrl Pts',(44.8518746516715,753.741539999995,103.567315461367));
#78422=CARTESIAN_POINT('Ctrl Pts',(44.8206625872923,753.624759284194,104.182208679739));
#78423=CARTESIAN_POINT('Ctrl Pts',(44.2375623083812,753.810449016713,104.046078043825));
#78424=CARTESIAN_POINT('Ctrl Pts',(45.0085265998517,754.259352877323,103.680782752095));
#78425=CARTESIAN_POINT('Ctrl Pts',(44.9690396895463,754.142216340654,104.278001051109));
#78426=CARTESIAN_POINT('Ctrl Pts',(44.4106063671844,754.358904400579,104.161327568411));
#78427=CARTESIAN_POINT('Ctrl Pts',(45.1002504493515,754.516305080123,103.74017707805));
#78428=CARTESIAN_POINT('Ctrl Pts',(45.0566143202729,754.400226022768,104.328716018458));
#78429=CARTESIAN_POINT('Ctrl Pts',(44.5114523561693,754.631227769305,104.221624502903));
#78430=CARTESIAN_POINT('Ctrl Pts',(45.4089475002517,755.263809131338,103.919511248394));
#78431=CARTESIAN_POINT('Ctrl Pts',(45.3524248984368,755.147282537831,104.482366235933));
#78432=CARTESIAN_POINT('Ctrl Pts',(44.8495485943442,755.423863452299,104.403592609289));
#78433=CARTESIAN_POINT('Ctrl Pts',(45.6603645608836,755.736496797567,104.041550175918));
#78434=CARTESIAN_POINT('Ctrl Pts',(45.5975986674501,755.628487215605,104.590077208969));
#78435=CARTESIAN_POINT('Ctrl Pts',(45.1233896323209,755.925647089536,104.527303365006));
#78436=CARTESIAN_POINT('Ctrl Pts',(46.1061076400661,756.40873710487,104.220441809427));
#78437=CARTESIAN_POINT('Ctrl Pts',(46.0413560410478,756.317625207438,104.751047110497));
#78438=CARTESIAN_POINT('Ctrl Pts',(45.6068395559476,756.639778449399,104.708487339111));
#78439=CARTESIAN_POINT('Ctrl Pts',(46.2668483778836,756.627399620023,104.279627720028));
#78440=CARTESIAN_POINT('Ctrl Pts',(46.2008832979289,756.540949210339,104.804363833508));
#78441=CARTESIAN_POINT('Ctrl Pts',(45.7808868346458,756.872158644901,104.768404935654));
#78442=CARTESIAN_POINT('Ctrl Pts',(46.6095956365525,757.048455848963,104.394751624816));
#78443=CARTESIAN_POINT('Ctrl Pts',(46.5423197953537,756.971159154162,104.908585762778));
#78444=CARTESIAN_POINT('Ctrl Pts',(46.151447281953,757.319765230662,104.884904813448));
#78445=CARTESIAN_POINT('Ctrl Pts',(46.7901385762444,757.249215258982,104.45023537906));
#78446=CARTESIAN_POINT('Ctrl Pts',(46.7227447552921,757.176852686386,104.959173188352));
#78447=CARTESIAN_POINT('Ctrl Pts',(46.3463802154442,757.533253384794,104.941027707592));
#78448=CARTESIAN_POINT('Ctrl Pts',(47.3587160332289,757.823009112407,104.609666709733));
#78449=CARTESIAN_POINT('Ctrl Pts',(47.2893552731759,757.761581290454,105.104277070691));
#78450=CARTESIAN_POINT('Ctrl Pts',(46.9595638789727,758.143567934702,105.102237696256));
#78451=CARTESIAN_POINT('Ctrl Pts',(47.7734412621022,758.167848086674,104.706595789808));
#78452=CARTESIAN_POINT('Ctrl Pts',(47.706990188793,758.117175996062,105.194224195243));
#78453=CARTESIAN_POINT('Ctrl Pts',(47.4059222897145,758.510547383819,105.200167705424));
#78454=CARTESIAN_POINT('Ctrl Pts',(48.4514501703775,758.626478847941,104.835483439563));
#78455=CARTESIAN_POINT('Ctrl Pts',(48.3932481566116,758.589939004014,105.314345113022));
#78456=CARTESIAN_POINT('Ctrl Pts',(48.134519768385,758.998737734966,105.330317611021));
#78457=CARTESIAN_POINT('Ctrl Pts',(48.6874818606445,758.76966617092,104.875741471088));
#78458=CARTESIAN_POINT('Ctrl Pts',(48.6316846628547,758.737249348849,105.351893075696));
#78459=CARTESIAN_POINT('Ctrl Pts',(48.38798759889,759.151176514627,105.370956824011));
#78460=CARTESIAN_POINT('Ctrl Pts',(49.1677758503293,759.029429484382,104.948719148144));
#78461=CARTESIAN_POINT('Ctrl Pts',(49.1170905060348,759.004243100467,105.420023263218));
#78462=CARTESIAN_POINT('Ctrl Pts',(48.9034665725843,759.427748450228,105.444608450082));
#78463=CARTESIAN_POINT('Ctrl Pts',(49.4132813461956,759.146937273221,104.981702524249));
#78464=CARTESIAN_POINT('Ctrl Pts',(49.3655541140878,759.125201002094,105.45093035461));
#78465=CARTESIAN_POINT('Ctrl Pts',(49.1668145853464,759.552873463948,105.477887235526));
#78466=CARTESIAN_POINT('Ctrl Pts',(49.9148905872182,759.35748115349,105.040728766851));
#78467=CARTESIAN_POINT('Ctrl Pts',(49.8732615932761,759.341703719427,105.506261540841));
#78468=CARTESIAN_POINT('Ctrl Pts',(49.7046495990986,759.77707896997,105.537431528601));
#78469=CARTESIAN_POINT('Ctrl Pts',(50.1709940815575,759.450517538234,105.066772942566));
#78470=CARTESIAN_POINT('Ctrl Pts',(50.132764946986,759.437496221055,105.530750099739));
#78471=CARTESIAN_POINT('Ctrl Pts',(49.9791362390332,759.876159864622,105.563698346379));
#78472=CARTESIAN_POINT('Ctrl Pts',(50.6939870257785,759.611675989273,105.11183475266));
#78473=CARTESIAN_POINT('Ctrl Pts',(50.6626659053261,759.60326155973,105.573119554025));
#78474=CARTESIAN_POINT('Ctrl Pts',(50.5394972721225,760.047795397873,105.60913954858));
#78475=CARTESIAN_POINT('Ctrl Pts',(50.9619905198647,759.680016906257,105.130914271761));
#78476=CARTESIAN_POINT('Ctrl Pts',(50.9344582158919,759.673639259957,105.591104788454));
#78477=CARTESIAN_POINT('Ctrl Pts',(50.8265645638574,760.120583193639,105.628376318847));
#78478=CARTESIAN_POINT('Ctrl Pts',(51.7753420479021,759.84436412666,105.176763005322));
#78479=CARTESIAN_POINT('Ctrl Pts',(51.7582264576729,759.842529266706,105.634258674167));
#78480=CARTESIAN_POINT('Ctrl Pts',(51.6975998109845,760.295628418505,105.674599430838));
#78481=CARTESIAN_POINT('Ctrl Pts',(52.3204317814714,759.89866305656,105.191873856739));
#78482=CARTESIAN_POINT('Ctrl Pts',(52.3123691280982,759.898645098071,105.648594749949));
#78483=CARTESIAN_POINT('Ctrl Pts',(52.2811255874571,760.35346752339,105.689829315887));
#78484=CARTESIAN_POINT('Ctrl Pts',(53.1422255185264,759.899585901188,105.192131310029));
#78485=CARTESIAN_POINT('Ctrl Pts',(53.1460494438434,759.899594647449,105.64883774948));
#78486=CARTESIAN_POINT('Ctrl Pts',(53.1608917437895,760.354450523046,105.690088828146));
#78487=CARTESIAN_POINT('Ctrl Pts',(53.4168551254893,759.886373409819,105.188450617713));
#78488=CARTESIAN_POINT('Ctrl Pts',(53.4247959624678,759.885985202566,105.645359420836));
#78489=CARTESIAN_POINT('Ctrl Pts',(53.4548903834744,760.340376857288,105.686378827854));
#78490=CARTESIAN_POINT('Ctrl Pts',(53.9675536213112,759.832084811908,105.17332453908));
#78491=CARTESIAN_POINT('Ctrl Pts',(53.9833766930975,759.830129923587,105.631089132305));
#78492=CARTESIAN_POINT('Ctrl Pts',(54.0444787668349,760.28255157886,105.671131426169));
#78493=CARTESIAN_POINT('Ctrl Pts',(54.2419099682168,759.791027458344,105.161883921301));
#78494=CARTESIAN_POINT('Ctrl Pts',(54.2617662228772,759.787844040971,105.620286614436));
#78495=CARTESIAN_POINT('Ctrl Pts',(54.3382358524801,760.238819943468,105.659598813989));
#78496=CARTESIAN_POINT('Ctrl Pts',(55.0489471047564,759.629112297025,105.116715339214));
#78497=CARTESIAN_POINT('Ctrl Pts',(55.0809094134985,759.621093926842,105.577680193947));
#78498=CARTESIAN_POINT('Ctrl Pts',(55.2025043190926,760.066364963711,105.61406153305));
#78499=CARTESIAN_POINT('Ctrl Pts',(55.5710463976871,759.469419747382,105.072109809235));
#78500=CARTESIAN_POINT('Ctrl Pts',(55.6111133398768,759.456081709598,105.535495281444));
#78501=CARTESIAN_POINT('Ctrl Pts',(55.7618470107023,759.896281612356,105.569087544629));
#78502=CARTESIAN_POINT('Ctrl Pts',(56.3303163159383,759.152348544857,104.983223153246));
#78503=CARTESIAN_POINT('Ctrl Pts',(56.3779146260612,759.130763073273,105.452353711034));
#78504=CARTESIAN_POINT('Ctrl Pts',(56.5759381906951,759.558635651997,105.479421434344));
#78505=CARTESIAN_POINT('Ctrl Pts',(56.5802727164515,759.033027300629,104.94973178096));
#78506=CARTESIAN_POINT('Ctrl Pts',(56.6308781790121,759.007942241034,105.42097037371));
#78507=CARTESIAN_POINT('Ctrl Pts',(56.8440578657723,759.431579412207,105.445630264923));
#78508=CARTESIAN_POINT('Ctrl Pts',(57.0615059695379,758.773327759877,104.876773293326));
#78509=CARTESIAN_POINT('Ctrl Pts',(57.1172413600607,758.741012612513,105.352855148836));
#78510=CARTESIAN_POINT('Ctrl Pts',(57.3605396045951,759.155074860993,105.371998350356));
#78511=CARTESIAN_POINT('Ctrl Pts',(57.294018868685,758.632543759301,104.83719138845));
#78512=CARTESIAN_POINT('Ctrl Pts',(57.3521149071898,758.596181765672,105.315938102217));
#78513=CARTESIAN_POINT('Ctrl Pts',(57.6102260026136,759.005194380144,105.332041857984));
#78514=CARTESIAN_POINT('Ctrl Pts',(57.7432907980298,758.329697775192,104.75208224537));
#78515=CARTESIAN_POINT('Ctrl Pts',(57.8052249848145,758.285129533451,105.236897381044));
#78516=CARTESIAN_POINT('Ctrl Pts',(58.0930084527051,758.682827936322,105.246100041666));
#78517=CARTESIAN_POINT('Ctrl Pts',(57.9600487684303,758.167634829186,104.706552727405));
#78518=CARTESIAN_POINT('Ctrl Pts',(58.0236467810424,758.118539254183,105.194680055239));
#78519=CARTESIAN_POINT('Ctrl Pts',(58.3261033342161,758.510340844161,105.20011241727));
#78520=CARTESIAN_POINT('Ctrl Pts',(58.3778094652649,757.822177088784,104.609756284298));
#78521=CARTESIAN_POINT('Ctrl Pts',(58.4437597202967,757.76411531061,105.105383013978));
#78522=CARTESIAN_POINT('Ctrl Pts',(58.7757333828905,758.142735072835,105.102306949991));
#78523=CARTESIAN_POINT('Ctrl Pts',(58.5797093488485,757.637852690173,104.558228376542));
#78524=CARTESIAN_POINT('Ctrl Pts',(58.6465023262139,757.574888333299,105.057958577838));
#78525=CARTESIAN_POINT('Ctrl Pts',(58.9932364046669,757.94662755088,105.050225183338));
#78526=CARTESIAN_POINT('Ctrl Pts',(59.1544072875436,757.058734139539,104.397303612921));
#78527=CARTESIAN_POINT('Ctrl Pts',(59.2251233187521,756.97865409733,104.909978577497));
#78528=CARTESIAN_POINT('Ctrl Pts',(59.6130103989281,757.330647109462,104.887506015757));
#78529=CARTESIAN_POINT('Ctrl Pts',(59.4935762137873,756.641866404394,104.282546238651));
#78530=CARTESIAN_POINT('Ctrl Pts',(59.562918319445,756.550559643376,104.805531171682));
#78531=CARTESIAN_POINT('Ctrl Pts',(59.9797033840178,756.887441018598,104.771385918518));
#78532=CARTESIAN_POINT('Ctrl Pts',(59.9394997893029,755.971526865868,104.104068709291));
#78533=CARTESIAN_POINT('Ctrl Pts',(60.0010294218336,755.87243549109,104.647027891106));
#78534=CARTESIAN_POINT('Ctrl Pts',(60.4633225313643,756.175320476182,104.590623776178));
#78535=CARTESIAN_POINT('Ctrl Pts',(60.0775910818274,755.74051238977,104.043534590738));
#78536=CARTESIAN_POINT('Ctrl Pts',(60.1369009815706,755.637390179665,104.593249818085));
#78537=CARTESIAN_POINT('Ctrl Pts',(60.6133744486101,755.929997358585,104.529288381377));
#78538=CARTESIAN_POINT('Ctrl Pts',(60.3322391296729,755.262753497981,103.921522025463));
#78539=CARTESIAN_POINT('Ctrl Pts',(60.3862493070344,755.153147854279,104.485863090903));
#78540=CARTESIAN_POINT('Ctrl Pts',(60.8906892901628,755.422887310523,104.405602436978));
#78541=CARTESIAN_POINT('Ctrl Pts',(60.447901738291,755.017429606684,103.860427381585));
#78542=CARTESIAN_POINT('Ctrl Pts',(60.4986089402268,754.905013930175,104.432563256064));
#78543=CARTESIAN_POINT('Ctrl Pts',(61.0169814111351,755.162609709595,104.343640628005));
#78544=CARTESIAN_POINT('Ctrl Pts',(60.7560740078579,754.27217004841,103.681568565603));
#78545=CARTESIAN_POINT('Ctrl Pts',(60.7986572104131,754.148276419581,104.276856895969));
#78546=CARTESIAN_POINT('Ctrl Pts',(61.3544921187512,754.372350029824,104.162155689742));
#78547=CARTESIAN_POINT('Ctrl Pts',(60.9123307712354,753.759154140586,103.567040624627));
#78548=CARTESIAN_POINT('Ctrl Pts',(60.9446633007839,753.63474809668,104.180498188071));
#78549=CARTESIAN_POINT('Ctrl Pts',(61.5271361446121,753.828916680788,104.045825043828));
#78550=CARTESIAN_POINT('Ctrl Pts',(61.1251758119162,752.697511926956,103.362211444783));
#78551=CARTESIAN_POINT('Ctrl Pts',(61.1403990245377,752.583507919546,104.011897615359));
#78552=CARTESIAN_POINT('Ctrl Pts',(61.7657767399434,752.705810036518,103.837562632188));
#78553=CARTESIAN_POINT('Ctrl Pts',(61.1807573575412,752.146129805475,103.272018526422));
#78554=CARTESIAN_POINT('Ctrl Pts',(61.1858008747042,752.04551697713,103.940958574835));
#78555=CARTESIAN_POINT('Ctrl Pts',(61.8307144309821,752.123237070503,103.745735973319));
#78556=CARTESIAN_POINT('Ctrl Pts',(61.1807573575412,751.59614455564,103.206330589227));
#78557=CARTESIAN_POINT('Ctrl Pts',(61.1807573575412,751.519058933453,103.89061093067));
#78558=CARTESIAN_POINT('Ctrl Pts',(61.8355401657986,751.54292199161,103.678781264903));
#78559=CARTESIAN_POINT('',(61.1807573575412,751.59614455564,103.206330589227));
#78560=CARTESIAN_POINT('',(61.8355401657986,751.54292199161,103.678781264903));
#78561=CARTESIAN_POINT('Origin',(61.6807573575412,751.59614455564,103.206330589227));
#78562=CARTESIAN_POINT('Ctrl Pts',(43.9196965836672,751.54292215966,103.678777984592));
#78563=CARTESIAN_POINT('Ctrl Pts',(43.9222882420743,751.854579858462,103.714735840723));
#78564=CARTESIAN_POINT('Ctrl Pts',(43.9416843025476,752.162082511931,103.757115234728));
#78565=CARTESIAN_POINT('Ctrl Pts',(43.9770626340715,752.465825441172,103.804485148761));
#78566=CARTESIAN_POINT('Ctrl Pts',(44.0079926061767,752.731376695964,103.845898919748));
#78567=CARTESIAN_POINT('Ctrl Pts',(44.0511391087946,752.994054039292,103.891127868557));
#78568=CARTESIAN_POINT('Ctrl Pts',(44.1059768732623,753.254114812661,103.939236516006));
#78569=CARTESIAN_POINT('Ctrl Pts',(44.1070628642689,753.259264979954,103.940189245552));
#78570=CARTESIAN_POINT('Ctrl Pts',(44.1081534842892,753.264414115119,103.941143116971));
#78571=CARTESIAN_POINT('Ctrl Pts',(44.1092487338049,753.26956221924,103.942098124302));
#78572=CARTESIAN_POINT('Ctrl Pts',(44.1676695835732,753.54416322397,103.993038425126));
#78573=CARTESIAN_POINT('Ctrl Pts',(44.239273149121,753.815847378745,104.047214475678));
#78574=CARTESIAN_POINT('Ctrl Pts',(44.3240881220502,754.084675390243,104.103703645877));
#78575=CARTESIAN_POINT('Ctrl Pts',(44.3261337935242,754.091159313724,104.105066120923));
#78576=CARTESIAN_POINT('Ctrl Pts',(44.328187400331,754.097641960348,104.106430043822));
#78577=CARTESIAN_POINT('Ctrl Pts',(44.3302489077782,754.104123247547,104.107795383506));
#78578=CARTESIAN_POINT('Ctrl Pts',(44.4077281650296,754.347714566551,104.159110019675));
#78579=CARTESIAN_POINT('Ctrl Pts',(44.4964062601969,754.589472508106,104.212446643126));
#78580=CARTESIAN_POINT('Ctrl Pts',(44.5944959003185,754.825061900319,104.266177546448));
#78581=CARTESIAN_POINT('Ctrl Pts',(44.6042892519893,754.848583342186,104.271542084754));
#78582=CARTESIAN_POINT('Ctrl Pts',(44.6141764317493,754.872043333742,104.27691056703));
#78583=CARTESIAN_POINT('Ctrl Pts',(44.6241556689194,754.8954375867,104.282281382562));
#78584=CARTESIAN_POINT('Ctrl Pts',(44.6271462429718,754.902448367652,104.283890906546));
#78585=CARTESIAN_POINT('Ctrl Pts',(44.6301452662658,754.909454266755,104.285500809474));
#78586=CARTESIAN_POINT('Ctrl Pts',(44.6331527373413,754.916455286669,104.287111078783));
#78587=CARTESIAN_POINT('Ctrl Pts',(44.8234368635388,755.359413148416,104.388993584289));
#78588=CARTESIAN_POINT('Ctrl Pts',(45.0475806350685,755.783008851131,104.492369940441));
#78589=CARTESIAN_POINT('Ctrl Pts',(45.3053136151034,756.187928903774,104.594105064536));
#78590=CARTESIAN_POINT('Ctrl Pts',(45.3510494184664,756.2597836734,104.612158391006));
#78591=CARTESIAN_POINT('Ctrl Pts',(45.3978429047043,756.331050318697,104.630160157722));
#78592=CARTESIAN_POINT('Ctrl Pts',(45.4456925075793,756.401732640839,104.64809300649));
#78593=CARTESIAN_POINT('Ctrl Pts',(45.45003966964,756.408154167679,104.649722215409));
#78594=CARTESIAN_POINT('Ctrl Pts',(45.4543961181741,756.414571424984,104.651351039854));
#78595=CARTESIAN_POINT('Ctrl Pts',(45.4587618192155,756.420984356023,104.652979456487));
#78596=CARTESIAN_POINT('Ctrl Pts',(45.6163109922364,756.652413849778,104.711745664119));
#78597=CARTESIAN_POINT('Ctrl Pts',(45.7859551656581,756.878279376204,104.769998200999));
#78598=CARTESIAN_POINT('Ctrl Pts',(45.9661679585971,757.095961187712,104.826654941289));
#78599=CARTESIAN_POINT('Ctrl Pts',(46.1514947957323,757.319820332065,104.884919475725));
#78600=CARTESIAN_POINT('Ctrl Pts',(46.3464184182909,757.533287259426,104.941037304803));
#78601=CARTESIAN_POINT('Ctrl Pts',(46.5507789485454,757.736687387445,104.994764523293));
#78602=CARTESIAN_POINT('Ctrl Pts',(46.5553762786402,757.741263112164,104.995973180162));
#78603=CARTESIAN_POINT('Ctrl Pts',(46.5599783502191,757.745833779824,104.997180627251));
#78604=CARTESIAN_POINT('Ctrl Pts',(46.5645851663029,757.750399388697,104.998386862409));
#78605=CARTESIAN_POINT('Ctrl Pts',(46.9137288383299,758.096420028114,105.089805613366));
#78606=CARTESIAN_POINT('Ctrl Pts',(47.2901206721729,758.413385452472,105.174261793583));
#78607=CARTESIAN_POINT('Ctrl Pts',(47.6947821660368,758.700291748076,105.250752122856));
#78608=CARTESIAN_POINT('Ctrl Pts',(47.7596785582558,758.746303498074,105.263019033557));
#78609=CARTESIAN_POINT('Ctrl Pts',(47.8253019526046,758.791542230477,105.275081093836));
#78610=CARTESIAN_POINT('Ctrl Pts',(47.8916564802653,758.836003896006,105.286934195027));
#78611=CARTESIAN_POINT('Ctrl Pts',(47.8956664048994,758.838690795215,105.287650499462));
#78612=CARTESIAN_POINT('Ctrl Pts',(47.8996792064592,758.841374880698,105.288366053528));
#78613=CARTESIAN_POINT('Ctrl Pts',(47.9036948563414,758.844056135095,105.289080852419));
#78614=CARTESIAN_POINT('Ctrl Pts',(48.1428788724764,759.003759598727,105.331656394186));
#78615=CARTESIAN_POINT('Ctrl Pts',(48.3922085638967,759.153441202998,105.371559916014));
#78616=CARTESIAN_POINT('Ctrl Pts',(48.6457272938702,759.28946210282,105.407782617332));
#78617=CARTESIAN_POINT('Ctrl Pts',(48.6491409775775,759.291293653214,105.408270363722));
#78618=CARTESIAN_POINT('Ctrl Pts',(48.6525556554173,759.293122900299,105.408757489342));
#78619=CARTESIAN_POINT('Ctrl Pts',(48.6559713274725,759.294949844451,105.4092439943));
#78620=CARTESIAN_POINT('Ctrl Pts',(48.9104046830959,759.431038884519,105.445483740654));
#78621=CARTESIAN_POINT('Ctrl Pts',(49.1703412219104,759.554343580572,105.478277671731));
#78622=CARTESIAN_POINT('Ctrl Pts',(49.4357322277162,759.664975899792,105.507659360736));
#78623=CARTESIAN_POINT('Ctrl Pts',(49.4384950114107,759.666127608633,105.507965231129));
#78624=CARTESIAN_POINT('Ctrl Pts',(49.4412583861498,759.667277944231,105.508270731881));
#78625=CARTESIAN_POINT('Ctrl Pts',(49.444022352054,759.668426906305,105.508575862942));
#78626=CARTESIAN_POINT('Ctrl Pts',(49.7102673651492,759.779103171087,105.537968274488));
#78627=CARTESIAN_POINT('Ctrl Pts',(49.9820143411467,759.877040020028,105.563931608773));
#78628=CARTESIAN_POINT('Ctrl Pts',(50.2593169608851,759.961976978418,105.586418896536));
#78629=CARTESIAN_POINT('Ctrl Pts',(50.261424521963,759.962622518038,105.586589804883));
#78630=CARTESIAN_POINT('Ctrl Pts',(50.2635324714005,759.963267320058,105.586760516006));
#78631=CARTESIAN_POINT('Ctrl Pts',(50.2656408076297,759.963911383872,105.586931029756));
#78632=CARTESIAN_POINT('Ctrl Pts',(50.5437951360706,760.048883190283,105.60942703249));
#78633=CARTESIAN_POINT('Ctrl Pts',(50.8287372405806,760.121019818447,105.628491616469));
#78634=CARTESIAN_POINT('Ctrl Pts',(51.1169098357794,760.178930684446,105.643783944634));
#78635=CARTESIAN_POINT('Ctrl Pts',(51.1183173872021,760.179213544521,105.643858638546));
#78636=CARTESIAN_POINT('Ctrl Pts',(51.1197249553105,760.179496058764,105.643933240885));
#78637=CARTESIAN_POINT('Ctrl Pts',(51.1211325401031,760.179778227198,105.644007751659));
#78638=CARTESIAN_POINT('Ctrl Pts',(51.537483728184,760.263241165698,105.666047382542));
#78639=CARTESIAN_POINT('Ctrl Pts',(51.9553898405354,760.316467744201,105.680080083813));
#78640=CARTESIAN_POINT('Ctrl Pts',(52.3748207884131,760.340038026233,105.686291460172));
#78641=CARTESIAN_POINT('Ctrl Pts',(52.5388480286482,760.349255677751,105.688720548744));
#78642=CARTESIAN_POINT('Ctrl Pts',(52.7031084285715,760.353938347338,105.689953616226));
#78643=CARTESIAN_POINT('Ctrl Pts',(52.8676000187963,760.354122807732,105.690002312588));
#78644=CARTESIAN_POINT('Ctrl Pts',(52.8676121319811,760.354122821316,105.690002316174));
#78645=CARTESIAN_POINT('Ctrl Pts',(52.8676242451673,760.354122834875,105.690002319753));
#78646=CARTESIAN_POINT('Ctrl Pts',(52.8676363583547,760.35412284841,105.690002323327));
#78647=CARTESIAN_POINT('Ctrl Pts',(53.1601792657639,760.354449726949,105.690088617979));
#78648=CARTESIAN_POINT('Ctrl Pts',(53.4534590064905,760.340443962875,105.686396550651));
#78649=CARTESIAN_POINT('Ctrl Pts',(53.7474975400303,760.311678350027,105.678811605977));
#78650=CARTESIAN_POINT('Ctrl Pts',(53.7482265437083,760.311607032036,105.67879280078));
#78651=CARTESIAN_POINT('Ctrl Pts',(53.7489555522463,760.311535623303,105.67877397165));
#78652=CARTESIAN_POINT('Ctrl Pts',(53.7496845656449,760.311464123822,105.678755118587));
#78653=CARTESIAN_POINT('Ctrl Pts',(54.0430101818375,760.28269561375,105.671169405409));
#78654=CARTESIAN_POINT('Ctrl Pts',(54.3353080121679,760.239254752756,105.659713477702));
#78655=CARTESIAN_POINT('Ctrl Pts',(54.621997755479,760.182196535239,105.644647363647));
#78656=CARTESIAN_POINT('Ctrl Pts',(54.6234403711711,760.181909419701,105.644571551334));
#78657=CARTESIAN_POINT('Ctrl Pts',(54.6248828455483,760.18162195925,105.644495647578));
#78658=CARTESIAN_POINT('Ctrl Pts',(54.626325178025,760.181334154021,105.644419652411));
#78659=CARTESIAN_POINT('Ctrl Pts',(55.0237698139674,760.102027443378,105.623478661413));
#78660=CARTESIAN_POINT('Ctrl Pts',(55.4132143245847,759.996489629965,105.595581455059));
#78661=CARTESIAN_POINT('Ctrl Pts',(55.7946463204337,759.864793743759,105.560676652494));
#78662=CARTESIAN_POINT('Ctrl Pts',(55.9633680415354,759.806539698937,105.545236945213));
#78663=CARTESIAN_POINT('Ctrl Pts',(56.130522226761,759.743168128376,105.528426281525));
#78664=CARTESIAN_POINT('Ctrl Pts',(56.2961088088657,759.674688336685,105.51024101466));
#78665=CARTESIAN_POINT('Ctrl Pts',(56.2989309021838,759.6735212351,105.509931083025));
#78666=CARTESIAN_POINT('Ctrl Pts',(56.3017525423132,759.672352648481,105.509620751853));
#78667=CARTESIAN_POINT('Ctrl Pts',(56.3045737292892,759.671182576856,105.50931002112));
#78668=CARTESIAN_POINT('Ctrl Pts',(56.5723103313437,759.56014030856,105.479821018315));
#78669=CARTESIAN_POINT('Ctrl Pts',(56.8368504016774,759.434989847435,105.446537269546));
#78670=CARTESIAN_POINT('Ctrl Pts',(57.0918297542857,759.298919797329,105.410304083083));
#78671=CARTESIAN_POINT('Ctrl Pts',(57.0953207503219,759.297056822933,105.409808004052));
#78672=CARTESIAN_POINT('Ctrl Pts',(57.0988099745461,759.295191792752,105.40931136945));
#78673=CARTESIAN_POINT('Ctrl Pts',(57.102297410318,759.293324715008,105.408814181461));
#78674=CARTESIAN_POINT('Ctrl Pts',(57.3562133100673,759.157385085934,105.372614536862));
#78675=CARTESIAN_POINT('Ctrl Pts',(57.6019269575373,759.010170269504,105.333368585133));
#78676=CARTESIAN_POINT('Ctrl Pts',(57.8395823891179,758.852032502038,105.291209524237));
#78677=CARTESIAN_POINT('Ctrl Pts',(57.8435961886419,758.849361688703,105.290497493305));
#78678=CARTESIAN_POINT('Ctrl Pts',(57.8476076982969,758.846687755669,105.289784630274));
#78679=CARTESIAN_POINT('Ctrl Pts',(57.8516169192593,758.844010704458,105.289070935729));
#78680=CARTESIAN_POINT('Ctrl Pts',(58.0882524163231,758.686003612812,105.246946676398));
#78681=CARTESIAN_POINT('Ctrl Pts',(58.3169134960859,758.517132591522,105.201923457535));
#78682=CARTESIAN_POINT('Ctrl Pts',(58.5376144473366,758.337392970489,105.154098018575));
#78683=CARTESIAN_POINT('Ctrl Pts',(58.5420522017946,758.333778847849,105.153136366377));
#78684=CARTESIAN_POINT('Ctrl Pts',(58.546486708164,758.330160353861,105.152173587515));
#78685=CARTESIAN_POINT('Ctrl Pts',(58.550917968495,758.326537487121,105.151209682423));
#78686=CARTESIAN_POINT('Ctrl Pts',(58.7332547760087,758.177464332762,105.111547066319));
#78687=CARTESIAN_POINT('Ctrl Pts',(58.9107348333014,758.020340398815,105.069804813504));
#78688=CARTESIAN_POINT('Ctrl Pts',(59.0815559882096,757.856699493983,105.026498262851));
#78689=CARTESIAN_POINT('Ctrl Pts',(59.1165412024408,757.823184838755,105.017628817184));
#78690=CARTESIAN_POINT('Ctrl Pts',(59.1512469848355,757.789396703121,105.008693726704));
#78691=CARTESIAN_POINT('Ctrl Pts',(59.1856576422419,757.755348095664,104.999697380079));
#78692=CARTESIAN_POINT('Ctrl Pts',(59.1903858204453,757.750669664742,104.998461241823));
#78693=CARTESIAN_POINT('Ctrl Pts',(59.195108372811,757.745986371901,104.997223961393));
#78694=CARTESIAN_POINT('Ctrl Pts',(59.1998252568978,757.74129825323,104.995985550773));
#78695=CARTESIAN_POINT('Ctrl Pts',(59.4544505926583,757.488225722995,104.929134062762));
#78696=CARTESIAN_POINT('Ctrl Pts',(59.6914823033983,757.222735724059,104.859365942784));
#78697=CARTESIAN_POINT('Ctrl Pts',(59.9114777383397,756.944951075768,104.787414134271));
#78698=CARTESIAN_POINT('Ctrl Pts',(60.043401849949,756.778372651292,104.744266973425));
#78699=CARTESIAN_POINT('Ctrl Pts',(60.1691988731846,756.607372436143,104.700334462475));
#78700=CARTESIAN_POINT('Ctrl Pts',(60.2889819139123,756.431971457055,104.655774342994));
#78701=CARTESIAN_POINT('Ctrl Pts',(60.2933667668142,756.425550619118,104.654143147393));
#78702=CARTESIAN_POINT('Ctrl Pts',(60.2977435424752,756.419123894807,104.652511115576));
#78703=CARTESIAN_POINT('Ctrl Pts',(60.302112246228,756.412691285737,104.650878255422));
#78704=CARTESIAN_POINT('Ctrl Pts',(60.4587645447275,756.182031791949,104.592327410428));
#78705=CARTESIAN_POINT('Ctrl Pts',(60.604959123994,755.94374589697,104.532726165884));
#78706=CARTESIAN_POINT('Ctrl Pts',(60.7404635896536,755.697527263392,104.472591813655));
#78707=CARTESIAN_POINT('Ctrl Pts',(60.7443280641775,755.690505312992,104.470876832005));
#78708=CARTESIAN_POINT('Ctrl Pts',(60.7481838759298,755.683476843825,104.469161401562));
#78709=CARTESIAN_POINT('Ctrl Pts',(60.7520310175676,755.676441850253,104.467445534873));
#78710=CARTESIAN_POINT('Ctrl Pts',(60.8868425647486,755.429921587369,104.407318129921));
#78711=CARTESIAN_POINT('Ctrl Pts',(61.0100891296998,755.176812867826,104.347021350455));
#78712=CARTESIAN_POINT('Ctrl Pts',(61.120367510098,754.920453707401,104.288034421268));
#78713=CARTESIAN_POINT('Ctrl Pts',(61.1234156256758,754.913367891055,104.286404011235));
#78714=CARTESIAN_POINT('Ctrl Pts',(61.1264538819749,754.906279489723,104.284774578093));
#78715=CARTESIAN_POINT('Ctrl Pts',(61.1294822492254,754.899188572816,104.283146152984));
#78716=CARTESIAN_POINT('Ctrl Pts',(61.2851753799673,754.534633364785,104.199426252964));
#78717=CARTESIAN_POINT('Ctrl Pts',(61.4160669876604,754.161503146051,104.117788101251));
#78718=CARTESIAN_POINT('Ctrl Pts',(61.5215771637907,753.779210947047,104.04077912677));
#78719=CARTESIAN_POINT('Ctrl Pts',(61.5667510621108,753.615533569567,104.007807941331));
#78720=CARTESIAN_POINT('Ctrl Pts',(61.6072722405618,753.450176565982,103.975685963823));
#78721=CARTESIAN_POINT('Ctrl Pts',(61.6430949649522,753.28309321559,103.944615964494));
#78722=CARTESIAN_POINT('Ctrl Pts',(61.6442187866902,753.277851517633,103.943641244083));
#78723=CARTESIAN_POINT('Ctrl Pts',(61.6453380248863,753.272607919378,103.942667522459));
#78724=CARTESIAN_POINT('Ctrl Pts',(61.6464526753947,753.267362426993,103.94169480763));
#78725=CARTESIAN_POINT('Ctrl Pts',(61.6800280803303,753.109358165033,103.912394776783));
#78726=CARTESIAN_POINT('Ctrl Pts',(61.7093532644357,752.94940376462,103.884017215441));
#78727=CARTESIAN_POINT('Ctrl Pts',(61.734231455373,752.788230657605,103.856889346437));
#78728=CARTESIAN_POINT('Ctrl Pts',(61.7530337256528,752.666420340786,103.836386829738));
#78729=CARTESIAN_POINT('Ctrl Pts',(61.7692967927551,752.543914606322,103.81659808501));
#78730=CARTESIAN_POINT('Ctrl Pts',(61.7829539548099,752.421035328951,103.79765983892));
#78731=CARTESIAN_POINT('Ctrl Pts',(61.7971811141958,752.293027543925,103.777931183397));
#78732=CARTESIAN_POINT('Ctrl Pts',(61.8085787756287,752.164678612146,103.759133442712));
#78733=CARTESIAN_POINT('Ctrl Pts',(61.8171072456853,752.035968727419,103.741364412261));
#78734=CARTESIAN_POINT('Ctrl Pts',(61.8254209279602,751.910500374928,103.724042891224));
#78735=CARTESIAN_POINT('Ctrl Pts',(61.8310081021847,751.784688356559,103.707698629829));
#78736=CARTESIAN_POINT('Ctrl Pts',(61.8337861166434,751.658514124101,103.692440352553));
#78737=CARTESIAN_POINT('Ctrl Pts',(61.8346337139604,751.620017225506,103.687784914263));
#78738=CARTESIAN_POINT('Ctrl Pts',(61.8352194731405,751.581486643892,103.683230718558));
#78739=CARTESIAN_POINT('Ctrl Pts',(61.8355401657986,751.54292199161,103.678781264903));
#78740=CARTESIAN_POINT('Ctrl Pts',(61.1807573575412,751.59614455564,103.206330589227));
#78741=CARTESIAN_POINT('Ctrl Pts',(61.1807573575412,751.718279376357,103.220917861222));
#78742=CARTESIAN_POINT('Ctrl Pts',(61.1780202994061,751.840070301746,103.236662403929));
#78743=CARTESIAN_POINT('Ctrl Pts',(61.1726298703664,751.961534761204,103.253447745652));
#78744=CARTESIAN_POINT('Ctrl Pts',(61.1671114860814,752.085882481826,103.270631529224));
#78745=CARTESIAN_POINT('Ctrl Pts',(61.1588122816436,752.209888772891,103.288906439657));
#78746=CARTESIAN_POINT('Ctrl Pts',(61.1477725027734,752.333573159067,103.308169159173));
#78747=CARTESIAN_POINT('Ctrl Pts',(61.1452162792684,752.36221186088,103.312629376807));
#78748=CARTESIAN_POINT('Ctrl Pts',(61.1425129174128,752.390833280895,103.317142632079));
#78749=CARTESIAN_POINT('Ctrl Pts',(61.1396625485833,752.419437602569,103.321707772919));
#78750=CARTESIAN_POINT('Ctrl Pts',(61.1242164768869,752.574443649098,103.346446147822));
#78751=CARTESIAN_POINT('Ctrl Pts',(61.1044561303026,752.728875719466,103.37269840247));
#78752=CARTESIAN_POINT('Ctrl Pts',(61.080504106868,752.88200547624,103.40014979494));
#78753=CARTESIAN_POINT('Ctrl Pts',(61.0623131367301,752.998303743913,103.42099844942));
#78754=CARTESIAN_POINT('Ctrl Pts',(61.0417054555287,753.113850750621,103.44253827644));
#78755=CARTESIAN_POINT('Ctrl Pts',(61.0187532924489,753.228333029416,103.464626059596));
#78756=CARTESIAN_POINT('Ctrl Pts',(61.0187372299444,753.228413147012,103.464641517186));
#78757=CARTESIAN_POINT('Ctrl Pts',(61.0187211663153,753.228493264148,103.464656975041));
#78758=CARTESIAN_POINT('Ctrl Pts',(61.0187051015615,753.228573380827,103.464672433162));
#78759=CARTESIAN_POINT('Ctrl Pts',(60.9357145300591,753.642456409306,103.544529137881));
#78760=CARTESIAN_POINT('Ctrl Pts',(60.8224631198419,754.045356768554,103.631716926695));
#78761=CARTESIAN_POINT('Ctrl Pts',(60.6792876136371,754.438138498757,103.722736038756));
#78762=CARTESIAN_POINT('Ctrl Pts',(60.6389128222857,754.548901022487,103.748402982466));
#78763=CARTESIAN_POINT('Ctrl Pts',(60.5961581529625,754.658858791047,103.774374719279));
#78764=CARTESIAN_POINT('Ctrl Pts',(60.5510305085273,754.768030931921,103.800573012368));
#78765=CARTESIAN_POINT('Ctrl Pts',(60.5508956397594,754.768357204482,103.800651308755));
#78766=CARTESIAN_POINT('Ctrl Pts',(60.5507607497986,754.768683470021,103.800729607164));
#78767=CARTESIAN_POINT('Ctrl Pts',(60.5506258386452,754.769009728538,103.800807907594));
#78768=CARTESIAN_POINT('Ctrl Pts',(60.4478944370174,755.017447265838,103.860431687568));
#78769=CARTESIAN_POINT('Ctrl Pts',(60.3322348600846,755.262761506947,103.921524154167));
#78770=CARTESIAN_POINT('Ctrl Pts',(60.2049151155111,755.501632925562,103.982528405725));
#78771=CARTESIAN_POINT('Ctrl Pts',(60.0780610014804,755.73963074968,104.04330955408));
#78772=CARTESIAN_POINT('Ctrl Pts',(59.9405192295365,755.969823047112,104.103622339393));
#78773=CARTESIAN_POINT('Ctrl Pts',(59.7924856214108,756.192526600842,104.162909900451));
#78774=CARTESIAN_POINT('Ctrl Pts',(59.7919434243098,756.19334228873,104.16312705076));
#78775=CARTESIAN_POINT('Ctrl Pts',(59.7914010865019,756.19415787607,104.163344187296));
#78776=CARTESIAN_POINT('Ctrl Pts',(59.7908586079975,756.194973362876,104.163561310031));
#78777=CARTESIAN_POINT('Ctrl Pts',(59.5103527670844,756.616646867508,104.275831556317));
#78778=CARTESIAN_POINT('Ctrl Pts',(59.1925105038488,757.011662044582,104.384358291729));
#78779=CARTESIAN_POINT('Ctrl Pts',(58.8354949001653,757.379387741009,104.486417413724));
#78780=CARTESIAN_POINT('Ctrl Pts',(58.8152435256669,757.40024663545,104.492206621476));
#78781=CARTESIAN_POINT('Ctrl Pts',(58.7948660949876,757.421017715167,104.497975015419));
#78782=CARTESIAN_POINT('Ctrl Pts',(58.7743622687371,757.441700862214,104.503722097022));
#78783=CARTESIAN_POINT('Ctrl Pts',(58.7733336125057,757.442738514788,104.504010422295));
#78784=CARTESIAN_POINT('Ctrl Pts',(58.7723046378064,757.443775946385,104.504298694041));
#78785=CARTESIAN_POINT('Ctrl Pts',(58.771275344601,757.444813156983,104.504586912195));
#78786=CARTESIAN_POINT('Ctrl Pts',(58.5808516562452,757.636701597139,104.557908515421));
#78787=CARTESIAN_POINT('Ctrl Pts',(58.3801742618017,757.820019718356,104.609153555221));
#78788=CARTESIAN_POINT('Ctrl Pts',(58.1725590383603,757.991902528665,104.657313147226));
#78789=CARTESIAN_POINT('Ctrl Pts',(58.1713493088757,757.992904053023,104.657593762865));
#78790=CARTESIAN_POINT('Ctrl Pts',(58.1701393423884,757.993905190394,104.657874274123));
#78791=CARTESIAN_POINT('Ctrl Pts',(58.1689291395544,757.994905940208,104.658154680801));
#78792=CARTESIAN_POINT('Ctrl Pts',(57.9613202248094,758.166583428389,104.70625812639));
#78793=CARTESIAN_POINT('Ctrl Pts',(57.74586879823,758.327772728434,104.751541429878));
#78794=CARTESIAN_POINT('Ctrl Pts',(57.5225977213104,758.478461299949,104.793889430685));
#78795=CARTESIAN_POINT('Ctrl Pts',(57.521283696778,758.479348152301,104.794138662751));
#78796=CARTESIAN_POINT('Ctrl Pts',(57.5199694010075,758.480234641255,104.794387793235));
#78797=CARTESIAN_POINT('Ctrl Pts',(57.5186548339968,758.481120766816,104.794636822115));
#78798=CARTESIAN_POINT('Ctrl Pts',(57.2953041107844,758.631677401157,104.836947925182));
#78799=CARTESIAN_POINT('Ctrl Pts',(57.06412449074,758.771744807745,104.876328247103));
#78800=CARTESIAN_POINT('Ctrl Pts',(56.8248820252568,758.901021457148,104.912646842755));
#78801=CARTESIAN_POINT('Ctrl Pts',(56.8235513819219,758.901740481304,104.912848843253));
#78802=CARTESIAN_POINT('Ctrl Pts',(56.8222204887008,758.902459171897,104.91305074912));
#78803=CARTESIAN_POINT('Ctrl Pts',(56.8208893455624,758.903177528867,104.913252560329));
#78804=CARTESIAN_POINT('Ctrl Pts',(56.581479531921,759.032376037715,104.949548870375));
#78805=CARTESIAN_POINT('Ctrl Pts',(56.3327598991671,759.151183230584,104.982896590313));
#78806=CARTESIAN_POINT('Ctrl Pts',(56.0808986448664,759.25650434361,105.012422175321));
#78807=CARTESIAN_POINT('Ctrl Pts',(56.0796746295836,759.257016191502,105.012565666098));
#78808=CARTESIAN_POINT('Ctrl Pts',(56.0784505393988,759.257527721218,105.012709066717));
#78809=CARTESIAN_POINT('Ctrl Pts',(56.0772263750149,759.258038932408,105.012852377078));
#78810=CARTESIAN_POINT('Ctrl Pts',(55.5718655807993,759.469077658888,105.072013906959));
#78811=CARTESIAN_POINT('Ctrl Pts',(55.0504843965195,759.628654703179,105.116587532522));
#78812=CARTESIAN_POINT('Ctrl Pts',(54.5131113124341,759.736616264493,105.146705257487));
#78813=CARTESIAN_POINT('Ctrl Pts',(54.5123816890383,759.736762850326,105.146746150114));
#78814=CARTESIAN_POINT('Ctrl Pts',(54.5116520360825,759.736909341028,105.146787016095));
#78815=CARTESIAN_POINT('Ctrl Pts',(54.5109223535671,759.737055736599,105.146827855433));
#78816=CARTESIAN_POINT('Ctrl Pts',(54.2422928154709,759.790950648254,105.161862685196));
#78817=CARTESIAN_POINT('Ctrl Pts',(53.9682976582015,759.831974635287,105.173293918456));
#78818=CARTESIAN_POINT('Ctrl Pts',(53.6932892470521,759.859122090062,105.18085779993));
#78819=CARTESIAN_POINT('Ctrl Pts',(53.6929276245361,759.859157787628,105.180867746061));
#78820=CARTESIAN_POINT('Ctrl Pts',(53.6925660003232,759.859193461195,105.180877685505));
#78821=CARTESIAN_POINT('Ctrl Pts',(53.692204374423,759.859229110763,105.180887618259));
#78822=CARTESIAN_POINT('Ctrl Pts',(53.4168449209188,759.886374415834,105.188450898013));
#78823=CARTESIAN_POINT('Ctrl Pts',(53.1422198606357,759.899585894834,105.192131319773));
#78824=CARTESIAN_POINT('Ctrl Pts',(52.8682942728391,759.899278286312,105.19204549995));
#78825=CARTESIAN_POINT('Ctrl Pts',(52.8682575431499,759.899278245066,105.192045488443));
#78826=CARTESIAN_POINT('Ctrl Pts',(52.8682208134732,759.899278203579,105.192045476869));
#78827=CARTESIAN_POINT('Ctrl Pts',(52.868184083809,759.89927816185,105.192045465227));
#78828=CARTESIAN_POINT('Ctrl Pts',(52.3556480524019,759.898695868066,105.191883015616));
#78829=CARTESIAN_POINT('Ctrl Pts',(51.845582323436,759.851133811666,105.178646938558));
#78830=CARTESIAN_POINT('Ctrl Pts',(51.3379868705484,759.755295894061,105.151914842749));
#78831=CARTESIAN_POINT('Ctrl Pts',(51.3030154172992,759.748693015261,105.150073100012));
#78832=CARTESIAN_POINT('Ctrl Pts',(51.2680556907327,759.741860965531,105.148167290173));
#78833=CARTESIAN_POINT('Ctrl Pts',(51.2331076912966,759.734799312132,105.146197272619));
#78834=CARTESIAN_POINT('Ctrl Pts',(51.2323200163315,759.734640153162,105.146152871407));
#78835=CARTESIAN_POINT('Ctrl Pts',(51.23153236758,759.734480879735,105.146108438146));
#78836=CARTESIAN_POINT('Ctrl Pts',(51.230744745125,759.734321491882,105.146063972844));
#78837=CARTESIAN_POINT('Ctrl Pts',(50.960387914189,759.679610513937,105.130800951599));
#78838=CARTESIAN_POINT('Ctrl Pts',(50.6931888913391,759.611430047017,105.111766049666));
#78839=CARTESIAN_POINT('Ctrl Pts',(50.4324905512462,759.531096763007,105.089303880242));
#78840=CARTESIAN_POINT('Ctrl Pts',(50.4314101557122,759.530763842892,105.089210791704));
#78841=CARTESIAN_POINT('Ctrl Pts',(50.4303298528035,759.530430710309,105.089117643243));
#78842=CARTESIAN_POINT('Ctrl Pts',(50.429249642512,759.530097365272,105.089024434863));
#78843=CARTESIAN_POINT('Ctrl Pts',(50.1688396973573,759.449736750779,105.066554375817));
#78844=CARTESIAN_POINT('Ctrl Pts',(49.9138178176667,759.357030872691,105.040602588784));
#78845=CARTESIAN_POINT('Ctrl Pts',(49.6640859638924,759.252209212174,105.011215675376));
#78846=CARTESIAN_POINT('Ctrl Pts',(49.6628163442094,759.251676306013,105.011066274316));
#78847=CARTESIAN_POINT('Ctrl Pts',(49.6615468612612,759.251143086695,105.010916784436));
#78848=CARTESIAN_POINT('Ctrl Pts',(49.660277515055,759.250609554202,105.010767205733));
#78849=CARTESIAN_POINT('Ctrl Pts',(49.4107594812073,759.14573195828,104.981364207807));
#78850=CARTESIAN_POINT('Ctrl Pts',(49.1665103026534,759.028745024005,104.948526855206));
#78851=CARTESIAN_POINT('Ctrl Pts',(48.9276288233629,758.899547810277,104.912230599334));
#78852=CARTESIAN_POINT('Ctrl Pts',(48.9262603815349,758.898807699023,104.912022674823));
#78853=CARTESIAN_POINT('Ctrl Pts',(48.924892075464,758.898067156868,104.911814628255));
#78854=CARTESIAN_POINT('Ctrl Pts',(48.9235239062514,758.897326184491,104.91160645983));
#78855=CARTESIAN_POINT('Ctrl Pts',(48.6847697427405,758.768021827698,104.875279755613));
#78856=CARTESIAN_POINT('Ctrl Pts',(48.4501209010315,758.625579680219,104.835230789));
#78857=CARTESIAN_POINT('Ctrl Pts',(48.2254471982682,758.473601925703,104.792520911464));
#78858=CARTESIAN_POINT('Ctrl Pts',(48.224084691537,758.472680274834,104.792261902533));
#78859=CARTESIAN_POINT('Ctrl Pts',(48.22272252582,758.471758270358,104.792002794067));
#78860=CARTESIAN_POINT('Ctrl Pts',(48.2213607010834,758.470835912327,104.791743586116));
#78861=CARTESIAN_POINT('Ctrl Pts',(47.7707693013975,758.165652297368,104.705978604487));
#78862=CARTESIAN_POINT('Ctrl Pts',(47.357436514095,757.821717855496,104.609307927081));
#78863=CARTESIAN_POINT('Ctrl Pts',(46.9796643865617,757.440479868033,104.503379222176));
#78864=CARTESIAN_POINT('Ctrl Pts',(46.9786124252374,757.439418255519,104.503084248321));
#78865=CARTESIAN_POINT('Ctrl Pts',(46.9775607416614,757.438356351503,104.502789202658));
#78866=CARTESIAN_POINT('Ctrl Pts',(46.9765093358634,757.437294155939,104.502494085233));
#78867=CARTESIAN_POINT('Ctrl Pts',(46.7881027111374,757.246954059582,104.449610528658));
#78868=CARTESIAN_POINT('Ctrl Pts',(46.608619434504,757.047256610765,104.39442382041));
#78869=CARTESIAN_POINT('Ctrl Pts',(46.4382219947662,756.837927719196,104.337189771042));
#78870=CARTESIAN_POINT('Ctrl Pts',(46.2668310118311,756.627378285251,104.279622004803));
#78871=CARTESIAN_POINT('Ctrl Pts',(46.1060960213913,756.408719586273,104.220437312538));
#78872=CARTESIAN_POINT('Ctrl Pts',(45.9575265766773,756.184656946643,104.160811584938));
#78873=CARTESIAN_POINT('Ctrl Pts',(45.956968192286,756.183814828124,104.160587487206));
#78874=CARTESIAN_POINT('Ctrl Pts',(45.9564099695286,756.182972623177,104.160363379714));
#78875=CARTESIAN_POINT('Ctrl Pts',(45.9558519084036,756.182130331792,104.160139262496));
#78876=CARTESIAN_POINT('Ctrl Pts',(45.6869748935028,755.776309565548,104.052158315929));
#78877=CARTESIAN_POINT('Ctrl Pts',(45.4556141963641,755.350424500661,103.941918440707));
#78878=CARTESIAN_POINT('Ctrl Pts',(45.2616365426822,754.903580844173,103.833307486465));
#78879=CARTESIAN_POINT('Ctrl Pts',(45.241747857797,754.857765604591,103.82217151795));
#78880=CARTESIAN_POINT('Ctrl Pts',(45.2222522042453,754.811730014642,103.811052673536));
#78881=CARTESIAN_POINT('Ctrl Pts',(45.2031494655285,754.765473095282,103.799955144725));
#78882=CARTESIAN_POINT('Ctrl Pts',(45.2029977238449,754.765105655674,103.79986699204));
#78883=CARTESIAN_POINT('Ctrl Pts',(45.2028460064544,754.764738199117,103.799778840185));
#78884=CARTESIAN_POINT('Ctrl Pts',(45.2026943133641,754.764370725629,103.799690689167));
#78885=CARTESIAN_POINT('Ctrl Pts',(45.0999909574253,754.515573892939,103.740008304287));
#78886=CARTESIAN_POINT('Ctrl Pts',(45.0084219713795,754.259007028087,103.680706966827));
#78887=CARTESIAN_POINT('Ctrl Pts',(44.9302006255377,754.000446437919,103.624049110639));
#78888=CARTESIAN_POINT('Ctrl Pts',(44.9301647802918,754.00032795149,103.624023146949));
#78889=CARTESIAN_POINT('Ctrl Pts',(44.9301289377625,754.000209464507,103.623997183776));
#78890=CARTESIAN_POINT('Ctrl Pts',(44.9300930979498,754.000090976969,103.623971221122));
#78891=CARTESIAN_POINT('Ctrl Pts',(44.8518477686917,753.741409481043,103.567289661503));
#78892=CARTESIAN_POINT('Ctrl Pts',(44.7865499756604,753.480086321699,103.513075105129));
#78893=CARTESIAN_POINT('Ctrl Pts',(44.7340181312022,753.215987600015,103.462243225474));
#78894=CARTESIAN_POINT('Ctrl Pts',(44.7340063241217,753.21592824107,103.462231800478));
#78895=CARTESIAN_POINT('Ctrl Pts',(44.7339945176863,753.215868881986,103.462220375653));
#78896=CARTESIAN_POINT('Ctrl Pts',(44.7339827118959,753.215809522762,103.462208951));
#78897=CARTESIAN_POINT('Ctrl Pts',(44.6664310985141,752.876161669581,103.39683816619));
#78898=CARTESIAN_POINT('Ctrl Pts',(44.619802503244,752.531965278004,103.337008941954));
#78899=CARTESIAN_POINT('Ctrl Pts',(44.5951181145293,752.182622649644,103.28507900627));
#78900=CARTESIAN_POINT('Ctrl Pts',(44.5814191394018,751.988749670565,103.256259702477));
#78901=CARTESIAN_POINT('Ctrl Pts',(44.5744794255529,751.79329153799,103.229873637158));
#78902=CARTESIAN_POINT('Ctrl Pts',(44.5744794255529,751.59614455564,103.206327301003));
#78903=CARTESIAN_POINT('Origin',(44.0744794081648,738.805700682709,102.677639949919));
#78904=CARTESIAN_POINT('',(43.8756325293234,737.489494249471,103.141409944702));
#78905=CARTESIAN_POINT('Origin',(44.074479425553,737.487748923763,102.682654164686));
#78906=CARTESIAN_POINT('',(43.8756325293234,737.489494249471,103.141409944702));
#78907=CARTESIAN_POINT('Ctrl Pts',(61.1807573575412,752.432433191562,103.304005925674));
#78908=CARTESIAN_POINT('Ctrl Pts',(61.1807573572072,752.352624036457,103.978124555041));
#78909=CARTESIAN_POINT('Ctrl Pts',(61.8291002976553,752.375611223793,103.778088716576));
#78910=CARTESIAN_POINT('Ctrl Pts',(61.1807573575412,750.236642473856,103.038617574031));
#78911=CARTESIAN_POINT('Ctrl Pts',(61.1807573583187,750.098025106155,103.735420913324));
#78912=CARTESIAN_POINT('Ctrl Pts',(61.8481071279839,750.188704031144,103.507887504724));
#78913=CARTESIAN_POINT('Ctrl Pts',(61.1807573575412,748.037926488067,102.841853249379));
#78914=CARTESIAN_POINT('Ctrl Pts',(61.1807573576092,747.955742160344,103.573549866495));
#78915=CARTESIAN_POINT('Ctrl Pts',(61.8641730445071,748.004525375531,103.306069819682));
#78916=CARTESIAN_POINT('Ctrl Pts',(61.1807573575412,744.872422398288,102.704110639652));
#78917=CARTESIAN_POINT('Ctrl Pts',(61.1807573575109,744.843334627062,103.45882252758));
#78918=CARTESIAN_POINT('Ctrl Pts',(61.8760420486351,744.858180968395,103.164229826639));
#78919=CARTESIAN_POINT('Ctrl Pts',(61.1807573575411,743.909613176086,102.680905707402));
#78920=CARTESIAN_POINT('Ctrl Pts',(61.1807573575511,743.893463278854,103.439935530219));
#78921=CARTESIAN_POINT('Ctrl Pts',(61.8782104710529,743.900885214033,103.140202681235));
#78922=CARTESIAN_POINT('Ctrl Pts',(61.1807573575411,741.72559338774,102.658573823938));
#78923=CARTESIAN_POINT('Ctrl Pts',(61.1807573575284,741.72352117949,103.422147088387));
#78924=CARTESIAN_POINT('Ctrl Pts',(61.8806437790432,741.726018999221,103.11691165222));
#78925=CARTESIAN_POINT('Ctrl Pts',(61.1807573575413,740.504024682783,102.667452033055));
#78926=CARTESIAN_POINT('Ctrl Pts',(61.1807573574781,740.51080807793,103.430288184586));
#78927=CARTESIAN_POINT('Ctrl Pts',(61.8802581399683,740.50712798626,103.125906581776));
#78928=CARTESIAN_POINT('Ctrl Pts',(61.1807573575412,739.28265565772,102.671032434937));
#78929=CARTESIAN_POINT('Ctrl Pts',(61.1807573575944,739.283824549444,103.433975186531));
#78930=CARTESIAN_POINT('Ctrl Pts',(61.8803059240399,739.283702376469,103.129490493437));
#78931=CARTESIAN_POINT('',(61.8788481782903,740.125366496447,103.127135084915));
#78932=CARTESIAN_POINT('Origin',(61.6807577676043,740.123614817939,102.668051724002));
#78933=CARTESIAN_POINT('Ctrl Pts',(61.8355401657986,751.54292199161,103.678781264903));
#78934=CARTESIAN_POINT('Ctrl Pts',(61.8384787588597,751.189543606527,103.638009712643));
#78935=CARTESIAN_POINT('Ctrl Pts',(61.8411871116658,750.835827677254,103.599045405492));
#78936=CARTESIAN_POINT('Ctrl Pts',(61.8437662515124,750.481892841926,103.562101738362));
#78937=CARTESIAN_POINT('Ctrl Pts',(61.8461724288251,750.151693619869,103.527635591126));
#78938=CARTESIAN_POINT('Ctrl Pts',(61.8484664081269,749.821304102811,103.494928513058));
#78939=CARTESIAN_POINT('Ctrl Pts',(61.8506962759595,749.490793109622,103.464141507031));
#78940=CARTESIAN_POINT('Ctrl Pts',(61.8527456212718,749.187039163024,103.435846912365));
#78941=CARTESIAN_POINT('Ctrl Pts',(61.8547408431025,748.883182682306,103.409174260207));
#78942=CARTESIAN_POINT('Ctrl Pts',(61.8566878402505,748.579251128213,103.384234339186));
#78943=CARTESIAN_POINT('Ctrl Pts',(61.8585623243818,748.286639053391,103.360223268478));
#78944=CARTESIAN_POINT('Ctrl Pts',(61.860392300632,747.993957621667,103.337818478434));
#78945=CARTESIAN_POINT('Ctrl Pts',(61.8621507591059,747.701203844434,103.317102277541));
#78946=CARTESIAN_POINT('Ctrl Pts',(61.8638506124278,747.418206839903,103.297076497333));
#78947=CARTESIAN_POINT('Ctrl Pts',(61.8654837934075,747.135142455684,103.278628807288));
#78948=CARTESIAN_POINT('Ctrl Pts',(61.8669926368471,746.851978532029,103.261814975452));
#78949=CARTESIAN_POINT('Ctrl Pts',(61.8684390595075,746.580529086019,103.245696731016));
#78950=CARTESIAN_POINT('Ctrl Pts',(61.8697712776325,746.308988318233,103.231080061492));
#78951=CARTESIAN_POINT('Ctrl Pts',(61.8709059450773,746.037297746506,103.217994751078));
#78952=CARTESIAN_POINT('Ctrl Pts',(61.8711766714067,745.972473650647,103.214872657399));
#78953=CARTESIAN_POINT('Ctrl Pts',(61.8714359983516,745.907640880863,103.211837646742));
#78954=CARTESIAN_POINT('Ctrl Pts',(61.8716824986774,745.842798358752,103.208889941404));
#78955=CARTESIAN_POINT('Ctrl Pts',(61.8726385106581,745.591317035963,103.197457738992));
#78956=CARTESIAN_POINT('Ctrl Pts',(61.8734562291384,745.339774682026,103.187322776724));
#78957=CARTESIAN_POINT('Ctrl Pts',(61.8741903578932,745.088218203332,103.178420629519));
#78958=CARTESIAN_POINT('Ctrl Pts',(61.874920260042,744.83811001295,103.169569734724));
#78959=CARTESIAN_POINT('Ctrl Pts',(61.8755674729943,744.587988035432,103.161937492574));
#78960=CARTESIAN_POINT('Ctrl Pts',(61.876151387719,744.337867954568,103.155437940408));
#78961=CARTESIAN_POINT('Ctrl Pts',(61.8767310399504,744.089573714229,103.148985834036));
#78962=CARTESIAN_POINT('Ctrl Pts',(61.8772482273628,743.841281493753,103.14364991165));
#78963=CARTESIAN_POINT('Ctrl Pts',(61.8776890558787,743.59297415862,103.139323989149));
#78964=CARTESIAN_POINT('Ctrl Pts',(61.8780489409083,743.390260201962,103.135792378349));
#78965=CARTESIAN_POINT('Ctrl Pts',(61.8783573098943,743.187535613118,103.132933500598));
#78966=CARTESIAN_POINT('Ctrl Pts',(61.8785908136361,742.98477378795,103.130678769005));
#78967=CARTESIAN_POINT('Ctrl Pts',(61.8788741515892,742.738738670584,103.127942834113));
#78968=CARTESIAN_POINT('Ctrl Pts',(61.8790532116822,742.492644581835,103.126094962502));
#78969=CARTESIAN_POINT('Ctrl Pts',(61.8791721169013,742.246547775394,103.124944588732));
#78970=CARTESIAN_POINT('Ctrl Pts',(61.879292724808,741.996926935346,103.12377774195));
#78971=CARTESIAN_POINT('Ctrl Pts',(61.8793512245671,741.747303367807,103.123328391134));
#78972=CARTESIAN_POINT('Ctrl Pts',(61.8793620402373,741.49769720654,103.123375262688));
#78973=CARTESIAN_POINT('Ctrl Pts',(61.8793731911177,741.240355000058,103.123423586932));
#78974=CARTESIAN_POINT('Ctrl Pts',(61.8793334631664,740.983031397289,103.123999270504));
#78975=CARTESIAN_POINT('Ctrl Pts',(61.8792283444092,740.725706244935,103.124837783144));
#78976=CARTESIAN_POINT('Ctrl Pts',(61.8791466023763,740.525606076093,103.125489824032));
#78977=CARTESIAN_POINT('Ctrl Pts',(61.8790246531794,740.325504073412,103.126300315418));
#78978=CARTESIAN_POINT('Ctrl Pts',(61.8788449024366,740.125373764374,103.127136797834));
#78979=CARTESIAN_POINT('Ctrl Pts',(61.1807573575412,751.190390842625,103.161460170991));
#78980=CARTESIAN_POINT('Ctrl Pts',(61.1807573575412,751.325655907648,103.176136471429));
#78981=CARTESIAN_POINT('Ctrl Pts',(61.1807573575412,751.460907175924,103.191095813468));
#78982=CARTESIAN_POINT('Ctrl Pts',(61.1807573575412,751.59614455564,103.206330589227));
#78983=CARTESIAN_POINT('Origin',(61.6807573751531,738.813605060629,102.677609876716));
#78984=CARTESIAN_POINT('',(61.8796042537708,737.489494249471,103.141409944702));
#78985=CARTESIAN_POINT('Origin',(61.6807573575412,737.487748923763,102.682654164686));
#78986=CARTESIAN_POINT('',(61.8796869430852,740.125382453445,103.131345527102));
#78987=CARTESIAN_POINT('Origin',(52.8776183915471,737.487748923763,112.60871186179));
#78988=CARTESIAN_POINT('Ctrl Pts',(47.4333208409147,731.218654873935,103.766631507276));
#78989=CARTESIAN_POINT('Ctrl Pts',(47.4903874665928,731.169089705094,103.783146874125));
#78990=CARTESIAN_POINT('Ctrl Pts',(47.5481332189328,731.120299570413,103.799578343581));
#78991=CARTESIAN_POINT('Ctrl Pts',(47.6065015949763,731.072342124072,103.815890137194));
#78992=CARTESIAN_POINT('Ctrl Pts',(47.7742018602631,730.934553872641,103.862756133846));
#78993=CARTESIAN_POINT('Ctrl Pts',(47.9463966762133,730.80405183503,103.908474318674));
#78994=CARTESIAN_POINT('Ctrl Pts',(48.1231892969836,730.680578747284,103.952726980298));
#78995=CARTESIAN_POINT('Ctrl Pts',(48.1670582502311,730.649940392074,103.963707743723));
#78996=CARTESIAN_POINT('Ctrl Pts',(48.211210436374,730.619735036351,103.974598241531));
#78997=CARTESIAN_POINT('Ctrl Pts',(48.2556476994714,730.589959161072,103.985393549995));
#78998=CARTESIAN_POINT('Ctrl Pts',(48.3758656235744,730.509405282078,104.014598534351));
#78999=CARTESIAN_POINT('Ctrl Pts',(48.4981525688067,730.431967570665,104.043110482607));
#79000=CARTESIAN_POINT('Ctrl Pts',(48.6226013076915,730.357666854282,104.070828813816));
#79001=CARTESIAN_POINT('Ctrl Pts',(48.8327809759369,730.232181453146,104.117641900956));
#79002=CARTESIAN_POINT('Ctrl Pts',(49.049022413504,730.1157090445,104.162170387175));
#79003=CARTESIAN_POINT('Ctrl Pts',(49.2715626044912,730.008466747415,104.203884195918));
#79004=CARTESIAN_POINT('Ctrl Pts',(49.4070320348871,729.943183919914,104.22927711881));
#79005=CARTESIAN_POINT('Ctrl Pts',(49.5448501968965,729.881314641415,104.253629756634));
#79006=CARTESIAN_POINT('Ctrl Pts',(49.6850608216465,729.822914101572,104.276820177489));
#79007=CARTESIAN_POINT('Ctrl Pts',(49.7751789073598,729.785378109812,104.291725441182));
#79008=CARTESIAN_POINT('Ctrl Pts',(49.8657653920901,729.749494357006,104.306061555955));
#79009=CARTESIAN_POINT('Ctrl Pts',(49.9568153069889,729.715260451392,104.319811060496));
#79010=CARTESIAN_POINT('Ctrl Pts',(50.292244015169,729.589142434159,104.370464359309));
#79011=CARTESIAN_POINT('Ctrl Pts',(50.6338992149115,729.485434904179,104.413149724166));
#79012=CARTESIAN_POINT('Ctrl Pts',(50.9817695313361,729.403915246444,104.447033878752));
#79013=CARTESIAN_POINT('Ctrl Pts',(51.0701525460672,729.383203639933,104.45564278728));
#79014=CARTESIAN_POINT('Ctrl Pts',(51.1589368158667,729.363924516919,104.463683470189));
#79015=CARTESIAN_POINT('Ctrl Pts',(51.2481222818587,729.346074702995,104.471142049786));
#79016=CARTESIAN_POINT('Ctrl Pts',(51.2949743914626,729.336697598451,104.475060291226));
#79017=CARTESIAN_POINT('Ctrl Pts',(51.3419389862517,729.32771747114,104.478817985273));
#79018=CARTESIAN_POINT('Ctrl Pts',(51.3890171418665,729.319136999466,104.482412896601));
#79019=CARTESIAN_POINT('Ctrl Pts',(51.6108100758792,729.278712986187,104.499349115119));
#79020=CARTESIAN_POINT('Ctrl Pts',(51.8351262404447,729.247160032436,104.512672795294));
#79021=CARTESIAN_POINT('Ctrl Pts',(52.0620115376169,729.224765071157,104.522147068232));
#79022=CARTESIAN_POINT('Ctrl Pts',(52.3357794585568,729.197742509249,104.53357906509));
#79023=CARTESIAN_POINT('Ctrl Pts',(52.6114066564425,729.18439443935,104.539260772721));
#79024=CARTESIAN_POINT('Ctrl Pts',(52.8842892071817,729.184612644427,104.539167920817));
#79025=CARTESIAN_POINT('Ctrl Pts',(52.8855117861528,729.184613622038,104.539167504818));
#79026=CARTESIAN_POINT('Ctrl Pts',(52.8867343109061,729.184614871909,104.539166972943));
#79027=CARTESIAN_POINT('Ctrl Pts',(52.8879567810331,729.18461639403,104.539166325188));
#79028=CARTESIAN_POINT('Ctrl Pts',(53.3857239796833,729.185236173512,104.538902571453));
#79029=CARTESIAN_POINT('Ctrl Pts',(53.8790018614575,729.230179734849,104.519658858136));
#79030=CARTESIAN_POINT('Ctrl Pts',(54.3677408399323,729.31940537429,104.48229740503));
#79031=CARTESIAN_POINT('Ctrl Pts',(54.4173351519301,729.328459459181,104.478506187951));
#79032=CARTESIAN_POINT('Ctrl Pts',(54.4668853995529,729.337969958316,104.474529220779));
#79033=CARTESIAN_POINT('Ctrl Pts',(54.5163907755215,729.347936778366,104.470366910493));
#79034=CARTESIAN_POINT('Ctrl Pts',(54.7114157407302,729.387200771329,104.453969612161));
#79035=CARTESIAN_POINT('Ctrl Pts',(54.9064965795643,729.433888389138,104.434574530941));
#79036=CARTESIAN_POINT('Ctrl Pts',(55.098754983177,729.487234225264,104.412598792644));
#79037=CARTESIAN_POINT('Ctrl Pts',(55.1714270378057,729.507398501282,104.404292148961));
#79038=CARTESIAN_POINT('Ctrl Pts',(55.2436845065661,729.528510694318,104.395622861317));
#79039=CARTESIAN_POINT('Ctrl Pts',(55.315381563322,729.550531060602,104.386614149159));
#79040=CARTESIAN_POINT('Ctrl Pts',(55.4815118393699,729.601554766387,104.365739933323));
#79041=CARTESIAN_POINT('Ctrl Pts',(55.6450583157892,729.657475260353,104.343033475127));
#79042=CARTESIAN_POINT('Ctrl Pts',(55.8061710715705,729.718206206078,104.318638781474));
#79043=CARTESIAN_POINT('Ctrl Pts',(55.8987084970164,729.753087897072,104.304627338778));
#79044=CARTESIAN_POINT('Ctrl Pts',(55.9904286757707,729.789551686463,104.290061032122));
#79045=CARTESIAN_POINT('Ctrl Pts',(56.0813462694638,729.827576316513,104.274969868601));
#79046=CARTESIAN_POINT('Ctrl Pts',(56.4436427840962,729.979100244693,104.214833257817));
#79047=CARTESIAN_POINT('Ctrl Pts',(56.7932824124638,730.155215020753,104.146356969981));
#79048=CARTESIAN_POINT('Ctrl Pts',(57.1303788166724,730.356323264058,104.071323822942));
#79049=CARTESIAN_POINT('Ctrl Pts',(57.2572760202182,730.432028828896,104.043078204142));
#79050=CARTESIAN_POINT('Ctrl Pts',(57.3824601776219,730.511315078268,104.013889115566));
#79051=CARTESIAN_POINT('Ctrl Pts',(57.5059168719087,730.594203401661,103.983853486297));
#79052=CARTESIAN_POINT('Ctrl Pts',(57.5875886668259,730.649037513236,103.963983654466));
#79053=CARTESIAN_POINT('Ctrl Pts',(57.6681015618492,730.705188433614,103.943841378445));
#79054=CARTESIAN_POINT('Ctrl Pts',(57.7474430225457,730.762630072087,103.923470734033));
#79055=CARTESIAN_POINT('Ctrl Pts',(57.8947007825111,730.869241759545,103.885662815717));
#79056=CARTESIAN_POINT('Ctrl Pts',(58.0376550195572,730.98009982637,103.847138414877));
#79057=CARTESIAN_POINT('Ctrl Pts',(58.17643809902,731.09513910412,103.808134434802));
#79058=CARTESIAN_POINT('Ctrl Pts',(58.225462290879,731.135775957299,103.794356540481));
#79059=CARTESIAN_POINT('Ctrl Pts',(58.2739656903081,731.176934899041,103.780518722733));
#79060=CARTESIAN_POINT('Ctrl Pts',(58.3219531024995,731.218614186682,103.766631207477));
#79061=CARTESIAN_POINT('Ctrl Pts',(18.2205457342854,776.218453213852,107.756965262063));
#79062=CARTESIAN_POINT('Ctrl Pts',(18.2213549247058,776.117573843427,108.040792094665));
#79063=CARTESIAN_POINT('Ctrl Pts',(18.0556468322312,775.880815322444,107.955814427592));
#79064=CARTESIAN_POINT('Ctrl Pts',(17.3544392369962,776.755270180238,107.950249975219));
#79065=CARTESIAN_POINT('Ctrl Pts',(17.3244896481851,776.666856095555,108.259553418174));
#79066=CARTESIAN_POINT('Ctrl Pts',(17.1727637467093,776.406561520024,108.145113036192));
#79067=CARTESIAN_POINT('Ctrl Pts',(16.5030075315832,777.315984535372,108.138886510896));
#79068=CARTESIAN_POINT('Ctrl Pts',(16.488670529682,777.214259844005,108.458076806816));
#79069=CARTESIAN_POINT('Ctrl Pts',(16.3091708822954,776.961315153559,108.329900767511));
#79070=CARTESIAN_POINT('Ctrl Pts',(15.6662338972256,777.89550680801,108.337269960847));
#79071=CARTESIAN_POINT('Ctrl Pts',(15.6646166993499,777.782008928933,108.661951401639));
#79072=CARTESIAN_POINT('Ctrl Pts',(15.4635632798279,777.538177789599,108.526207820323));
#79073=CARTESIAN_POINT('',(15.4635632798629,777.538177785738,108.526207827222));
#79074=CARTESIAN_POINT('Origin',(15.4890368307271,777.667265994068,108.256601934497));
#79075=CARTESIAN_POINT('',(18.0556466141873,775.880815148244,107.955814158127));
#79076=CARTESIAN_POINT('Ctrl Pts',(18.0556467918663,775.880815346481,107.955814436247));
#79077=CARTESIAN_POINT('Ctrl Pts',(17.1738808373735,776.405896305826,108.144873521151));
#79078=CARTESIAN_POINT('Ctrl Pts',(16.3101489074236,776.96064795568,108.329673719029));
#79079=CARTESIAN_POINT('Ctrl Pts',(15.4635632805302,777.53817778912,108.52620782016));
#79080=CARTESIAN_POINT('',(18.2205407156876,776.21798090548,107.758260909884));
#79081=CARTESIAN_POINT('Origin',(18.0555120549653,775.982245018246,107.673481293432));
#79082=CARTESIAN_POINT('Ctrl Pts',(18.2205473657951,776.218126918571,107.757885251456));
#79083=CARTESIAN_POINT('Ctrl Pts',(17.4395547310011,776.702515187951,107.931255171408));
#79084=CARTESIAN_POINT('Ctrl Pts',(16.670513723768,777.206050004925,108.101619406009));
#79085=CARTESIAN_POINT('Ctrl Pts',(15.9133489649393,777.722889497859,108.285610804169));
#79086=CARTESIAN_POINT('Ctrl Pts',(87.534693420407,776.218613999725,107.756513650752));
#79087=CARTESIAN_POINT('Ctrl Pts',(87.5336178514962,776.117952853449,108.0409278003));
#79088=CARTESIAN_POINT('Ctrl Pts',(87.699590784449,775.880815944701,107.955814324766));
#79089=CARTESIAN_POINT('Ctrl Pts',(86.259537844912,775.428266754528,107.471942382034));
#79090=CARTESIAN_POINT('Ctrl Pts',(86.2555670717131,775.325475361612,107.756754598578));
#79091=CARTESIAN_POINT('Ctrl Pts',(86.4183730487532,775.085504287272,107.66948244197));
#79092=CARTESIAN_POINT('Ctrl Pts',(84.9560677605553,774.684903718524,107.197696734793));
#79093=CARTESIAN_POINT('Ctrl Pts',(84.9508894325089,774.58120275026,107.483989729736));
#79094=CARTESIAN_POINT('Ctrl Pts',(85.1091907908226,774.337094526585,107.393435206673));
#79095=CARTESIAN_POINT('Ctrl Pts',(82.2927499621516,773.285117635406,106.689234302032));
#79096=CARTESIAN_POINT('Ctrl Pts',(82.2887487103214,773.181142922102,106.978515953765));
#79097=CARTESIAN_POINT('Ctrl Pts',(82.4355140915199,772.928856409756,106.881939604336));
#79098=CARTESIAN_POINT('Ctrl Pts',(80.9329000613502,772.628392057774,106.455863954993));
#79099=CARTESIAN_POINT('Ctrl Pts',(80.9331460203576,772.526276326062,106.74708687405));
#79100=CARTESIAN_POINT('Ctrl Pts',(81.0710134534976,772.268715768294,106.647338926234));
#79101=CARTESIAN_POINT('Ctrl Pts',(78.1562200818106,771.392761835475,106.058942628791));
#79102=CARTESIAN_POINT('Ctrl Pts',(78.1613397634359,771.292476595305,106.351216827985));
#79103=CARTESIAN_POINT('Ctrl Pts',(78.2856477557455,771.028649273413,106.248771326341));
#79104=CARTESIAN_POINT('Ctrl Pts',(76.7382747560354,770.813290309123,105.895701125155));
#79105=CARTESIAN_POINT('Ctrl Pts',(76.7523463957842,770.716575263587,106.188097519309));
#79106=CARTESIAN_POINT('Ctrl Pts',(76.8636742037813,770.448155127505,106.085112151117));
#79107=CARTESIAN_POINT('Ctrl Pts',(73.8483529833387,769.729793727005,105.659592442164));
#79108=CARTESIAN_POINT('Ctrl Pts',(73.8695654291816,769.63647611085,105.948354019399));
#79109=CARTESIAN_POINT('Ctrl Pts',(73.9654526952167,769.365276516662,105.848948952432));
#79110=CARTESIAN_POINT('Ctrl Pts',(72.3942858815777,769.232288195398,105.58842925458));
#79111=CARTESIAN_POINT('Ctrl Pts',(72.4254204189451,769.142497596095,105.873763703825));
#79112=CARTESIAN_POINT('Ctrl Pts',(72.5071730554801,768.869421251228,105.778146304558));
#79113=CARTESIAN_POINT('Ctrl Pts',(69.4682809012006,768.323985331645,105.531976527412));
#79114=CARTESIAN_POINT('Ctrl Pts',(69.505130570297,768.237853395557,105.808378836195));
#79115=CARTESIAN_POINT('Ctrl Pts',(69.5714410518175,767.966563923016,105.72289441824));
#79116=CARTESIAN_POINT('Ctrl Pts',(67.9963263139418,767.913184640725,105.546636240739));
#79117=CARTESIAN_POINT('Ctrl Pts',(68.039107434635,767.829022250898,105.81678292199));
#79118=CARTESIAN_POINT('Ctrl Pts',(68.0939695200466,767.559560119585,105.738387788275));
#79119=CARTESIAN_POINT('Ctrl Pts',(65.0323690485381,767.186623681901,105.630322411241));
#79120=CARTESIAN_POINT('Ctrl Pts',(65.0760847078406,767.105299652801,105.88863578277));
#79121=CARTESIAN_POINT('Ctrl Pts',(65.116643660827,766.841456434063,105.823831389765));
#79122=CARTESIAN_POINT('Ctrl Pts',(63.5403268572924,766.870997823238,105.698903803921));
#79123=CARTESIAN_POINT('Ctrl Pts',(63.582537797136,766.789660577686,105.950808131252));
#79124=CARTESIAN_POINT('Ctrl Pts',(63.6167373626631,766.530467814802,105.893331175143));
#79125=CARTESIAN_POINT('Ctrl Pts',(60.5319701718021,766.351593356512,105.842003024112));
#79126=CARTESIAN_POINT('Ctrl Pts',(60.5693321518246,766.271904121821,106.083181145775));
#79127=CARTESIAN_POINT('Ctrl Pts',(60.5900264012593,766.019480612874,106.038035999016));
#79128=CARTESIAN_POINT('Ctrl Pts',(59.0156050355678,766.148059099485,105.915801308287));
#79129=CARTESIAN_POINT('Ctrl Pts',(59.0440098927689,766.067318380161,106.152731837784));
#79130=CARTESIAN_POINT('Ctrl Pts',(59.06316201519,765.819700469343,106.112522123908));
#79131=CARTESIAN_POINT('Ctrl Pts',(56.7192697416383,765.941250026258,105.99565564567));
#79132=CARTESIAN_POINT('Ctrl Pts',(56.7344612356701,765.860453468508,106.228099156722));
#79133=CARTESIAN_POINT('Ctrl Pts',(56.7496613191456,765.616810173469,106.19308711179));
#79134=CARTESIAN_POINT('Ctrl Pts',(55.9501937298133,765.888725246282,106.017218851542));
#79135=CARTESIAN_POINT('Ctrl Pts',(55.9619069202598,765.807911798399,106.248500301597));
#79136=CARTESIAN_POINT('Ctrl Pts',(55.9746367498585,765.565310282087,106.214834552912));
#79137=CARTESIAN_POINT('Ctrl Pts',(54.4042994258696,765.818508090254,106.046441318916));
#79138=CARTESIAN_POINT('Ctrl Pts',(54.4107850600319,765.737853040583,106.276099275293));
#79139=CARTESIAN_POINT('Ctrl Pts',(54.4165611592209,765.496472547381,106.244304592913));
#79140=CARTESIAN_POINT('Ctrl Pts',(53.630716477118,765.801038717635,106.05399145759));
#79141=CARTESIAN_POINT('Ctrl Pts',(53.6333631037709,765.720370934785,106.283261246584));
#79142=CARTESIAN_POINT('Ctrl Pts',(53.6367679636054,765.479352894896,106.25191739984));
#79143=CARTESIAN_POINT('Ctrl Pts',(51.320944157274,765.801809480288,106.053661913636));
#79144=CARTESIAN_POINT('Ctrl Pts',(51.3154236794076,765.721140016323,106.282949676225));
#79145=CARTESIAN_POINT('Ctrl Pts',(51.308435374231,765.480108275012,106.251585096457));
#79146=CARTESIAN_POINT('Ctrl Pts',(49.7905213129482,765.873238298318,106.021911621623));
#79147=CARTESIAN_POINT('Ctrl Pts',(49.7713984809396,765.793164808446,106.252609550755));
#79148=CARTESIAN_POINT('Ctrl Pts',(49.765754962707,765.55008826985,106.219576265668));
#79149=CARTESIAN_POINT('Ctrl Pts',(46.7466364047402,766.14748500395,105.916026945306));
#79150=CARTESIAN_POINT('Ctrl Pts',(46.7183488694763,766.066737371129,106.152947518903));
#79151=CARTESIAN_POINT('Ctrl Pts',(46.6991326128801,765.819137212082,106.112749731659));
#79152=CARTESIAN_POINT('Ctrl Pts',(45.233155034996,766.350078747165,105.842479913589));
#79153=CARTESIAN_POINT('Ctrl Pts',(45.1957740955227,766.270398907609,106.083623748225));
#79154=CARTESIAN_POINT('Ctrl Pts',(45.1751630890169,766.017991986964,106.03851775086));
#79155=CARTESIAN_POINT('Ctrl Pts',(42.2198738993365,766.869948931633,105.699133802545));
#79156=CARTESIAN_POINT('Ctrl Pts',(42.1776265700307,766.78862042883,105.95101607769));
#79157=CARTESIAN_POINT('Ctrl Pts',(42.1434897954953,766.529434177947,105.893564182041));
#79158=CARTESIAN_POINT('Ctrl Pts',(40.7200336640549,767.186966131458,105.6300621503));
#79159=CARTESIAN_POINT('Ctrl Pts',(40.6760645500492,767.105704617896,105.888384255489));
#79160=CARTESIAN_POINT('Ctrl Pts',(40.6357383690942,766.841788106103,105.823569143026));
#79161=CARTESIAN_POINT('Ctrl Pts',(38.4781056808001,767.737064430316,105.567037591417));
#79162=CARTESIAN_POINT('Ctrl Pts',(38.4461641720026,767.650888832438,105.834581014409));
#79163=CARTESIAN_POINT('Ctrl Pts',(38.3837285294506,767.38548886143,105.759216213041));
#79164=CARTESIAN_POINT('Ctrl Pts',(37.7308829200252,767.933261549124,105.552759622542));
#79165=CARTESIAN_POINT('Ctrl Pts',(37.7000110194929,767.846293937843,105.823313156379));
#79166=CARTESIAN_POINT('Ctrl Pts',(37.6334210776661,767.579653875514,105.744505442416));
#79167=CARTESIAN_POINT('Ctrl Pts',(36.2480250617279,768.346763858315,105.542525881567));
#79168=CARTESIAN_POINT('Ctrl Pts',(36.2190919362398,768.258082697861,105.818526797865));
#79169=CARTESIAN_POINT('Ctrl Pts',(36.1448885168633,767.98950585078,105.73348100182));
#79170=CARTESIAN_POINT('Ctrl Pts',(35.5117601149707,768.564176759389,105.546532407994));
#79171=CARTESIAN_POINT('Ctrl Pts',(35.4847637878845,768.474492412453,105.825126547508));
#79172=CARTESIAN_POINT('Ctrl Pts',(35.4060306581063,768.205298543414,105.737129671795));
#79173=CARTESIAN_POINT('Ctrl Pts',(33.3181340307008,769.246512188562,105.590106103946));
#79174=CARTESIAN_POINT('Ctrl Pts',(33.2871615303783,769.156654004714,105.875553753093));
#79175=CARTESIAN_POINT('Ctrl Pts',(33.2051169048726,768.88358612718,105.779810199754));
#79176=CARTESIAN_POINT('Ctrl Pts',(31.8758516711713,769.741242509528,105.661953891397));
#79177=CARTESIAN_POINT('Ctrl Pts',(31.8548850892463,769.647824959646,105.950746346646));
#79178=CARTESIAN_POINT('Ctrl Pts',(31.7586628738894,769.376713512273,105.851309487688));
#79179=CARTESIAN_POINT('Ctrl Pts',(29.0310841033454,770.80817936637,105.894731397872));
#79180=CARTESIAN_POINT('Ctrl Pts',(29.0171468783213,770.711418792167,106.187091334568));
#79181=CARTESIAN_POINT('Ctrl Pts',(28.905725568513,770.443052104303,106.084143587));
#79182=CARTESIAN_POINT('Ctrl Pts',(27.6285945736765,771.380493418822,106.055391376126));
#79183=CARTESIAN_POINT('Ctrl Pts',(27.6233671814146,771.280254931325,106.347667830369));
#79184=CARTESIAN_POINT('Ctrl Pts',(27.4992526397927,771.016354716152,106.245209657368));
#79185=CARTESIAN_POINT('Ctrl Pts',(24.8642886953906,772.608850120777,106.449213695433));
#79186=CARTESIAN_POINT('Ctrl Pts',(24.863940674956,772.506772873493,106.740473669186));
#79187=CARTESIAN_POINT('Ctrl Pts',(24.7263127094394,772.249086217425,106.640656841136));
#79188=CARTESIAN_POINT('Ctrl Pts',(23.5024732025465,773.265020652559,106.682018558467));
#79189=CARTESIAN_POINT('Ctrl Pts',(23.5064761400537,773.16103442948,106.971337918364));
#79190=CARTESIAN_POINT('Ctrl Pts',(23.3598548361072,772.90864623969,106.874683104988));
#79191=CARTESIAN_POINT('Ctrl Pts',(20.8213555103874,774.672343951284,107.193055298186));
#79192=CARTESIAN_POINT('Ctrl Pts',(20.8265704347935,774.568617899291,107.479369892601));
#79193=CARTESIAN_POINT('Ctrl Pts',(20.6683281599921,774.324450877034,107.388763799337));
#79194=CARTESIAN_POINT('Ctrl Pts',(19.498862029959,775.42630609411,107.471237036644));
#79195=CARTESIAN_POINT('Ctrl Pts',(19.5028455397015,775.323505963338,107.75604902853));
#79196=CARTESIAN_POINT('Ctrl Pts',(19.3400444664692,775.083529671144,107.668772140042));
#79197=CARTESIAN_POINT('Ctrl Pts',(18.2205442368837,776.218613355413,107.756513745616));
#79198=CARTESIAN_POINT('Ctrl Pts',(18.2216197623594,776.117952235154,108.040927907501));
#79199=CARTESIAN_POINT('Ctrl Pts',(18.055646832231,775.880815322444,107.955814427592));
#79200=CARTESIAN_POINT('',(87.6995909938491,775.880815775522,107.955814071221));
#79201=CARTESIAN_POINT('',(87.5347015018662,776.217932075331,107.758391194347));
#79202=CARTESIAN_POINT('Origin',(87.6997256064195,775.9822456651,107.673481199464));
#79203=CARTESIAN_POINT('',(72.9143353470373,769.422151368467,105.625740702768));
#79204=CARTESIAN_POINT('Ctrl Pts',(72.9143353591496,769.422151372559,105.625740703389));
#79205=CARTESIAN_POINT('Ctrl Pts',(73.5595632056107,769.640073855905,105.658870605513));
#79206=CARTESIAN_POINT('Ctrl Pts',(74.2034293583074,769.866876365016,105.700518523386));
#79207=CARTESIAN_POINT('Ctrl Pts',(74.8434686433405,770.101754837589,105.750415037215));
#79208=CARTESIAN_POINT('Ctrl Pts',(75.4835079283737,770.336633310163,105.800311551044));
#79209=CARTESIAN_POINT('Ctrl Pts',(76.1197187903174,770.579587235218,105.858456457505));
#79210=CARTESIAN_POINT('Ctrl Pts',(76.7496513514779,770.829776339044,105.924543673933));
#79211=CARTESIAN_POINT('Ctrl Pts',(76.7924259359966,770.846765038513,105.929031222917));
#79212=CARTESIAN_POINT('Ctrl Pts',(76.8351735163699,770.863787902504,105.933555445468));
#79213=CARTESIAN_POINT('Ctrl Pts',(76.8778934067034,770.880844703162,105.93811626543));
#79214=CARTESIAN_POINT('Ctrl Pts',(77.7781956810092,771.240309025396,106.034233473409));
#79215=CARTESIAN_POINT('Ctrl Pts',(78.668175288905,771.615443511941,106.146422411895));
#79216=CARTESIAN_POINT('Ctrl Pts',(79.5476437017226,772.006933824121,106.27197850604));
#79217=CARTESIAN_POINT('Ctrl Pts',(79.8555809468298,772.144010319947,106.315940741834));
#79218=CARTESIAN_POINT('Ctrl Pts',(80.1622296910544,772.283091693059,106.361541443976));
#79219=CARTESIAN_POINT('Ctrl Pts',(80.4675823874359,772.424206324646,106.408663614685));
#79220=CARTESIAN_POINT('Ctrl Pts',(80.7735702594751,772.565614494099,106.455883805998));
#79221=CARTESIAN_POINT('Ctrl Pts',(81.0782698798938,772.709073078691,106.504626295143));
#79222=CARTESIAN_POINT('Ctrl Pts',(81.3816836495893,772.854616733058,106.554771887758));
#79223=CARTESIAN_POINT('Ctrl Pts',(82.8526350110214,773.560213043846,106.797877953118));
#79224=CARTESIAN_POINT('Ctrl Pts',(84.2933577349007,774.31508394129,107.073196647605));
#79225=CARTESIAN_POINT('Ctrl Pts',(85.7035661425854,775.124749342466,107.365756396725));
#79226=CARTESIAN_POINT('Ctrl Pts',(86.31979169175,775.47855272625,107.493597637128));
#79227=CARTESIAN_POINT('Ctrl Pts',(86.9301910915229,775.842921633408,107.624435383555));
#79228=CARTESIAN_POINT('Ctrl Pts',(87.5347015018662,776.217932075331,107.758391194347));
#79229=CARTESIAN_POINT('',(32.8408501865509,769.421912550842,105.626344597616));
#79230=CARTESIAN_POINT('Ctrl Pts',(32.8408501865664,769.421912550837,105.626344597615));
#79231=CARTESIAN_POINT('Ctrl Pts',(33.0236782934409,769.360223677481,105.616839744328));
#79232=CARTESIAN_POINT('Ctrl Pts',(33.2068891034353,769.299142362413,105.608032051533));
#79233=CARTESIAN_POINT('Ctrl Pts',(33.3904861083511,769.238669866531,105.599921157552));
#79234=CARTESIAN_POINT('Ctrl Pts',(34.0174987635566,769.03214677958,105.572221178602));
#79235=CARTESIAN_POINT('Ctrl Pts',(34.6501640698298,768.832460864523,105.552522928579));
#79236=CARTESIAN_POINT('Ctrl Pts',(35.2846233311591,768.64112189397,105.540132327312));
#79237=CARTESIAN_POINT('Ctrl Pts',(35.4438452852828,768.593104051614,105.537022819946));
#79238=CARTESIAN_POINT('Ctrl Pts',(35.6031689190437,768.545616536284,105.534370539334));
#79239=CARTESIAN_POINT('Ctrl Pts',(35.7625331951534,768.498681780911,105.532168229936));
#79240=CARTESIAN_POINT('Ctrl Pts',(36.4241388190288,768.303830721013,105.523025275701));
#79241=CARTESIAN_POINT('Ctrl Pts',(37.0868545409594,768.118322885106,105.521569713914));
#79242=CARTESIAN_POINT('Ctrl Pts',(37.7508739084941,767.942395758076,105.526470077786));
#79243=CARTESIAN_POINT('Ctrl Pts',(37.8841707688899,767.90707971936,105.527453788731));
#79244=CARTESIAN_POINT('Ctrl Pts',(38.0175179372388,767.872150705027,105.528692784248));
#79245=CARTESIAN_POINT('Ctrl Pts',(38.15091594521,767.837610987588,105.530176143381));
#79246=CARTESIAN_POINT('Ctrl Pts',(39.6666985187674,767.445141095529,105.54703134203));
#79247=CARTESIAN_POINT('Ctrl Pts',(41.1890080909103,767.102716903944,105.595773740223));
#79248=CARTESIAN_POINT('Ctrl Pts',(42.7192171003575,766.817008028999,105.653936404576));
#79249=CARTESIAN_POINT('Ctrl Pts',(42.8000135837808,766.801922330094,105.657007448281));
#79250=CARTESIAN_POINT('Ctrl Pts',(42.8808320901257,766.786994821904,105.660104552257));
#79251=CARTESIAN_POINT('Ctrl Pts',(42.9616728208353,766.772226487832,105.663224405103));
#79252=CARTESIAN_POINT('Ctrl Pts',(44.5466204718882,766.482681400938,105.724391633511));
#79253=CARTESIAN_POINT('Ctrl Pts',(46.1401706839877,766.254624596373,105.793419872345));
#79254=CARTESIAN_POINT('Ctrl Pts',(47.7440902907559,766.097195410041,105.845350382395));
#79255=CARTESIAN_POINT('Ctrl Pts',(47.7713529131537,766.094519507556,105.846233071203));
#79256=CARTESIAN_POINT('Ctrl Pts',(47.7986185487758,766.091864008652,105.84711082102));
#79257=CARTESIAN_POINT('Ctrl Pts',(47.8258872054595,766.089228958453,105.847983508994));
#79258=CARTESIAN_POINT('Ctrl Pts',(49.3118883269248,765.945632315735,105.895540501731));
#79259=CARTESIAN_POINT('Ctrl Pts',(50.8069096666398,765.863014317756,105.927387474233));
#79260=CARTESIAN_POINT('Ctrl Pts',(52.3117085411413,765.846417767268,105.933827740143));
#79261=CARTESIAN_POINT('Ctrl Pts',(52.459091258596,765.844792271161,105.934458511408));
#79262=CARTESIAN_POINT('Ctrl Pts',(52.6065677619598,765.843800053509,105.934845580706));
#79263=CARTESIAN_POINT('Ctrl Pts',(52.754138758307,765.843445826145,105.934979848475));
#79264=CARTESIAN_POINT('Ctrl Pts',(52.7818089890395,765.843379406909,105.93500502429));
#79265=CARTESIAN_POINT('Ctrl Pts',(52.8094831122868,765.843335361707,105.935021625747));
#79266=CARTESIAN_POINT('Ctrl Pts',(52.8371610676647,765.843313695639,105.935029674915));
#79267=CARTESIAN_POINT('Ctrl Pts',(53.636861059485,765.842687697291,105.935262239763));
#79268=CARTESIAN_POINT('Ctrl Pts',(54.4398528135242,765.860749498513,105.928342777723));
#79269=CARTESIAN_POINT('Ctrl Pts',(55.244613964507,765.897618906657,105.914824361016));
#79270=CARTESIAN_POINT('Ctrl Pts',(55.3003085386821,765.900170503469,105.913888800867));
#79271=CARTESIAN_POINT('Ctrl Pts',(55.3559839602243,765.902810734082,105.912922266593));
#79272=CARTESIAN_POINT('Ctrl Pts',(55.4116402817597,765.905539243272,105.911925431088));
#79273=CARTESIAN_POINT('Ctrl Pts',(56.1880255318818,765.943600944657,105.898019941792));
#79274=CARTESIAN_POINT('Ctrl Pts',(56.960722155325,765.99885130209,105.878192146322));
#79275=CARTESIAN_POINT('Ctrl Pts',(57.7299521592197,766.070328053399,105.854281130698));
#79276=CARTESIAN_POINT('Ctrl Pts',(57.8126622929001,766.078013468198,105.851710139852));
#79277=CARTESIAN_POINT('Ctrl Pts',(57.8953323483527,766.085886453703,105.849091074128));
#79278=CARTESIAN_POINT('Ctrl Pts',(57.9779626577588,766.093945617801,105.846427342593));
#79279=CARTESIAN_POINT('Ctrl Pts',(59.5424882901759,766.246538157971,105.795992141575));
#79280=CARTESIAN_POINT('Ctrl Pts',(61.0927572405591,766.465921133663,105.729413145712));
#79281=CARTESIAN_POINT('Ctrl Pts',(62.630986689335,766.742742837056,105.669539025615));
#79282=CARTESIAN_POINT('Ctrl Pts',(62.7663823010022,766.767108801369,105.664268880046));
#79283=CARTESIAN_POINT('Ctrl Pts',(62.9016851664723,766.791917627592,105.659057180489));
#79284=CARTESIAN_POINT('Ctrl Pts',(63.0368965356465,766.817164168077,105.653919296428));
#79285=CARTESIAN_POINT('Ctrl Pts',(64.5189523589357,767.093892246284,105.597602797022));
#79286=CARTESIAN_POINT('Ctrl Pts',(65.990029631157,767.423147191921,105.550338785539));
#79287=CARTESIAN_POINT('Ctrl Pts',(67.451755462978,767.798254419419,105.532062337455));
#79288=CARTESIAN_POINT('Ctrl Pts',(67.6384506822806,767.846164037334,105.529728024542));
#79289=CARTESIAN_POINT('Ctrl Pts',(67.8249938600168,767.894819691892,105.52787330476));
#79290=CARTESIAN_POINT('Ctrl Pts',(68.0113863289532,767.944216390829,105.526521579779));
#79291=CARTESIAN_POINT('Ctrl Pts',(68.8926978463568,768.177776684027,105.52013027652));
#79292=CARTESIAN_POINT('Ctrl Pts',(69.7707970311868,768.427894891168,105.52513974266));
#79293=CARTESIAN_POINT('Ctrl Pts',(70.6455470696625,768.69398372115,105.543974097712));
#79294=CARTESIAN_POINT('Ctrl Pts',(71.166422612617,768.852428028317,105.555189135703));
#79295=CARTESIAN_POINT('Ctrl Pts',(71.6861109237649,769.016534162042,105.571305670155));
#79296=CARTESIAN_POINT('Ctrl Pts',(72.2045860049618,769.186171538845,105.592830330109));
#79297=CARTESIAN_POINT('Ctrl Pts',(72.4413593070117,769.263640260705,105.602660049989));
#79298=CARTESIAN_POINT('Ctrl Pts',(72.6779786088689,769.342312155877,105.61363557759));
#79299=CARTESIAN_POINT('Ctrl Pts',(72.914335334925,769.422151364376,105.625740702148));
#79300=CARTESIAN_POINT('Ctrl Pts',(18.2205382491878,776.217926749776,107.758400240177));
#79301=CARTESIAN_POINT('Ctrl Pts',(18.8176899041017,775.847482616211,107.626072229285));
#79302=CARTESIAN_POINT('Ctrl Pts',(19.42029013547,775.487607707795,107.496852123233));
#79303=CARTESIAN_POINT('Ctrl Pts',(20.0282637453734,775.13819782016,107.370606446288));
#79304=CARTESIAN_POINT('Ctrl Pts',(21.4287261468346,774.333334907756,107.079800528026));
#79305=CARTESIAN_POINT('Ctrl Pts',(22.8577001927037,773.583478723244,106.806304167243));
#79306=CARTESIAN_POINT('Ctrl Pts',(24.3145822062801,772.88293906295,106.564536635338));
#79307=CARTESIAN_POINT('Ctrl Pts',(24.6415401841664,772.725721780682,106.510278416338));
#79308=CARTESIAN_POINT('Ctrl Pts',(24.9699031440383,772.570975547355,106.457655516378));
#79309=CARTESIAN_POINT('Ctrl Pts',(25.2996699862003,772.418653078543,106.406814871278));
#79310=CARTESIAN_POINT('Ctrl Pts',(26.4393021087457,771.892246065315,106.231116089962));
#79311=CARTESIAN_POINT('Ctrl Pts',(27.595697848614,771.394747224638,106.076817314253));
#79312=CARTESIAN_POINT('Ctrl Pts',(28.768817589677,770.924268391335,105.949795981634));
#79313=CARTESIAN_POINT('Ctrl Pts',(28.8500363924492,770.891695648559,105.941001891652));
#79314=CARTESIAN_POINT('Ctrl Pts',(28.931335326977,770.859251953746,105.932339804482));
#79315=CARTESIAN_POINT('Ctrl Pts',(29.0127144902168,770.826937363433,105.923810175765));
#79316=CARTESIAN_POINT('Ctrl Pts',(30.0912177658905,770.398677964881,105.810768554961));
#79317=CARTESIAN_POINT('Ctrl Pts',(31.183803955927,769.993060962209,105.721095643046));
#79318=CARTESIAN_POINT('Ctrl Pts',(32.2906732771414,769.610038346885,105.656385894741));
#79319=CARTESIAN_POINT('Ctrl Pts',(32.4736749782796,769.546712181063,105.645687256886));
#79320=CARTESIAN_POINT('Ctrl Pts',(32.6570670106512,769.484003647625,105.635671053798));
#79321=CARTESIAN_POINT('Ctrl Pts',(32.8408501865509,769.421912550842,105.626344597616));
#79322=CARTESIAN_POINT('Ctrl Pts',(87.699590784449,775.880815944701,107.955814324766));
#79323=CARTESIAN_POINT('Ctrl Pts',(86.8582777839384,775.358573691995,107.767794186879));
#79324=CARTESIAN_POINT('Ctrl Pts',(86.0060117989125,774.857236858343,107.584458176575));
#79325=CARTESIAN_POINT('Ctrl Pts',(85.1428195414831,774.375835906652,107.408556668802));
#79326=CARTESIAN_POINT('Ctrl Pts',(84.6890166633739,774.122750761921,107.316080618647));
#79327=CARTESIAN_POINT('Ctrl Pts',(84.2321935891412,773.875176311381,107.225658799374));
#79328=CARTESIAN_POINT('Ctrl Pts',(83.7723522027849,773.632975867124,107.137687555858));
#79329=CARTESIAN_POINT('Ctrl Pts',(83.7596177450129,773.626268573216,107.13525135477));
#79330=CARTESIAN_POINT('Ctrl Pts',(83.7468809718159,773.619565372531,107.132817109852));
#79331=CARTESIAN_POINT('Ctrl Pts',(83.7341418825031,773.612866261111,107.130384833086));
#79332=CARTESIAN_POINT('Ctrl Pts',(82.8766542607943,773.161938806444,106.966664556956));
#79333=CARTESIAN_POINT('Ctrl Pts',(82.008669068268,772.729536592449,106.811865103256));
#79334=CARTESIAN_POINT('Ctrl Pts',(81.1301611010632,772.314552117029,106.669650327641));
#79335=CARTESIAN_POINT('Ctrl Pts',(80.6493702975054,772.0874389583,106.591818869306));
#79336=CARTESIAN_POINT('Ctrl Pts',(80.1654278484269,771.865542814205,106.517755856902));
#79337=CARTESIAN_POINT('Ctrl Pts',(79.6783303541909,771.648683021283,106.448055320323));
#79338=CARTESIAN_POINT('Ctrl Pts',(79.6565647520409,771.638992796983,106.44494080184));
#79339=CARTESIAN_POINT('Ctrl Pts',(79.6347925795945,771.629312489993,106.441835068224));
#79340=CARTESIAN_POINT('Ctrl Pts',(79.6130138468199,771.619642097175,106.438738156145));
#79341=CARTESIAN_POINT('Ctrl Pts',(78.5915534579615,771.166083880045,106.29348760144));
#79342=CARTESIAN_POINT('Ctrl Pts',(77.5557294924615,770.734362664327,106.167655588074));
#79343=CARTESIAN_POINT('Ctrl Pts',(76.5063986710057,770.324083567929,106.064972094903));
#79344=CARTESIAN_POINT('Ctrl Pts',(76.1440527569051,770.182409511301,106.029514312252));
#79345=CARTESIAN_POINT('Ctrl Pts',(75.7800960624704,770.043292390726,105.996816390673));
#79346=CARTESIAN_POINT('Ctrl Pts',(75.4145631715615,769.906716507234,105.967030809491));
#79347=CARTESIAN_POINT('Ctrl Pts',(75.3880786252614,769.896820953647,105.964872706558));
#79348=CARTESIAN_POINT('Ctrl Pts',(75.361591806201,769.886940921773,105.962730460533));
#79349=CARTESIAN_POINT('Ctrl Pts',(75.3351027106994,769.877076401201,105.960604043418));
#79350=CARTESIAN_POINT('Ctrl Pts',(74.2930654068928,769.489022440684,105.876954303209));
#79351=CARTESIAN_POINT('Ctrl Pts',(73.246276649245,769.124516422601,105.817703826413));
#79352=CARTESIAN_POINT('Ctrl Pts',(72.194795767384,768.783191202966,105.781328240662));
#79353=CARTESIAN_POINT('Ctrl Pts',(71.8102591048826,768.658365290246,105.768025339409));
#79354=CARTESIAN_POINT('Ctrl Pts',(71.4250949828742,768.536639299448,105.757781452103));
#79355=CARTESIAN_POINT('Ctrl Pts',(71.0393065916545,768.417994044972,105.750520851269));
#79356=CARTESIAN_POINT('Ctrl Pts',(71.0112581482468,768.409368034491,105.749992974961));
#79357=CARTESIAN_POINT('Ctrl Pts',(70.98320639808,768.400758307566,105.749480846806));
#79358=CARTESIAN_POINT('Ctrl Pts',(70.9551513342617,768.392164889373,105.748984355338));
#79359=CARTESIAN_POINT('Ctrl Pts',(69.8779620116377,768.062215958136,105.729921297378));
#79360=CARTESIAN_POINT('Ctrl Pts',(68.795896327465,767.756312172852,105.733909550365));
#79361=CARTESIAN_POINT('Ctrl Pts',(67.7085751978045,767.475856479629,105.754634331229));
#79362=CARTESIAN_POINT('Ctrl Pts',(67.3414226561117,767.381155826997,105.761632407292));
#79363=CARTESIAN_POINT('Ctrl Pts',(66.9736710071267,767.289356325921,105.770538728799));
#79364=CARTESIAN_POINT('Ctrl Pts',(66.6053060211355,767.200510675188,105.781110245067));
#79365=CARTESIAN_POINT('Ctrl Pts',(66.5767807618794,767.193630691158,105.781928876733));
#79366=CARTESIAN_POINT('Ctrl Pts',(66.5482518057202,767.186768460588,105.782757328545));
#79367=CARTESIAN_POINT('Ctrl Pts',(66.5197191417406,767.179924035241,105.783595431181));
#79368=CARTESIAN_POINT('Ctrl Pts',(65.5464684356867,766.946460317778,105.81218315726));
#79369=CARTESIAN_POINT('Ctrl Pts',(64.5689095968792,766.733710819704,105.851994672493));
#79370=CARTESIAN_POINT('Ctrl Pts',(63.5865249767008,766.543694768022,105.896332474997));
#79371=CARTESIAN_POINT('Ctrl Pts',(63.093381349984,766.448309312126,105.9185894447));
#79372=CARTESIAN_POINT('Ctrl Pts',(62.5990218002459,766.358652022941,105.941987598611));
#79373=CARTESIAN_POINT('Ctrl Pts',(62.1033816701624,766.274975514481,105.965683853526));
#79374=CARTESIAN_POINT('Ctrl Pts',(62.0766203065504,766.27045752384,105.966963298138));
#79375=CARTESIAN_POINT('Ctrl Pts',(62.0498551911242,766.265957036811,105.968243387741));
#79376=CARTESIAN_POINT('Ctrl Pts',(62.0230863151129,766.261474100584,105.969523995523));
#79377=CARTESIAN_POINT('Ctrl Pts',(60.993793818126,766.0891003102,106.01876476236));
#79378=CARTESIAN_POINT('Ctrl Pts',(59.9589403298854,765.942670793626,106.068766207129));
#79379=CARTESIAN_POINT('Ctrl Pts',(58.9178662167072,765.824834760521,106.112355741571));
#79380=CARTESIAN_POINT('Ctrl Pts',(58.4534442810074,765.772268244941,106.131800981546));
#79381=CARTESIAN_POINT('Ctrl Pts',(57.9877844352259,765.725391859862,106.149970946558));
#79382=CARTESIAN_POINT('Ctrl Pts',(57.52082820375,765.684440438175,106.166232140873));
#79383=CARTESIAN_POINT('Ctrl Pts',(57.4987351198496,765.682502904989,106.167001506193));
#79384=CARTESIAN_POINT('Ctrl Pts',(57.4766391419228,765.680578635084,106.167766670019));
#79385=CARTESIAN_POINT('Ctrl Pts',(57.4545402658822,765.678667649798,106.168527587898));
#79386=CARTESIAN_POINT('Ctrl Pts',(56.7926258462055,765.621429050229,106.19131890613));
#79387=CARTESIAN_POINT('Ctrl Pts',(56.1282177310631,765.576115938076,106.210298714617));
#79388=CARTESIAN_POINT('Ctrl Pts',(55.4608823872178,765.54328039121,106.22428065565));
#79389=CARTESIAN_POINT('Ctrl Pts',(55.3725062494401,765.53893193456,106.226132303339));
#79390=CARTESIAN_POINT('Ctrl Pts',(55.2840787559664,765.534802380145,106.227896276555));
#79391=CARTESIAN_POINT('Ctrl Pts',(55.1955988834149,765.530893075335,106.229569797693));
#79392=CARTESIAN_POINT('Ctrl Pts',(55.17689430288,765.530066651149,106.229923578841));
#79393=CARTESIAN_POINT('Ctrl Pts',(55.1581892595765,765.529250195679,106.230273254402));
#79394=CARTESIAN_POINT('Ctrl Pts',(55.1394838074096,765.528443709585,106.230618816138));
#79395=CARTESIAN_POINT('Ctrl Pts',(54.5347612060503,765.502371077699,106.241790371378));
#79396=CARTESIAN_POINT('Ctrl Pts',(53.9299116628076,765.486731543858,106.248659101124));
#79397=CARTESIAN_POINT('Ctrl Pts',(53.3266615204972,765.481538125481,106.250951479058));
#79398=CARTESIAN_POINT('Ctrl Pts',(53.1712106389157,765.480199839074,106.251542199467));
#79399=CARTESIAN_POINT('Ctrl Pts',(53.0158659657042,765.479555459939,106.251828930165));
#79400=CARTESIAN_POINT('Ctrl Pts',(52.8606571008079,765.479605727691,106.251806767246));
#79401=CARTESIAN_POINT('Ctrl Pts',(52.8459297524962,765.479610497461,106.251804664267));
#79402=CARTESIAN_POINT('Ctrl Pts',(52.8312031599683,765.479621520867,106.251799699673));
#79403=CARTESIAN_POINT('Ctrl Pts',(52.8164773180528,765.479638793933,106.251791882204));
#79404=CARTESIAN_POINT('Ctrl Pts',(51.7356232332715,765.480906610322,106.25121809205));
#79405=CARTESIAN_POINT('Ctrl Pts',(50.6591814899032,765.515843034854,106.235276753435));
#79406=CARTESIAN_POINT('Ctrl Pts',(49.5868625183453,765.582849136413,106.20744904546));
#79407=CARTESIAN_POINT('Ctrl Pts',(49.1346634480453,765.611105744411,106.195714044953));
#79408=CARTESIAN_POINT('Ctrl Pts',(48.6831976373843,765.645066027333,106.181865118927));
#79409=CARTESIAN_POINT('Ctrl Pts',(48.2324437882054,765.684612745822,106.166162999396));
#79410=CARTESIAN_POINT('Ctrl Pts',(48.2248448904869,765.68527943224,106.165898289953));
#79411=CARTESIAN_POINT('Ctrl Pts',(48.2172461944353,765.685947701091,106.165633068221));
#79412=CARTESIAN_POINT('Ctrl Pts',(48.209647699823,765.686617551509,106.165367336933));
#79413=CARTESIAN_POINT('Ctrl Pts',(47.1353654230241,765.781321630261,106.127797998829));
#79414=CARTESIAN_POINT('Ctrl Pts',(46.0651042888957,765.907638791474,106.08003928013));
#79415=CARTESIAN_POINT('Ctrl Pts',(44.9983540051326,766.063114396604,106.029843226538));
#79416=CARTESIAN_POINT('Ctrl Pts',(44.5514076839244,766.12825546177,106.00881211754));
#79417=CARTESIAN_POINT('Ctrl Pts',(44.1050776793143,766.198515194267,105.987353729809));
#79418=CARTESIAN_POINT('Ctrl Pts',(43.6593264839041,766.273713338407,105.966041018857));
#79419=CARTESIAN_POINT('Ctrl Pts',(43.6565741099716,766.27417766338,105.965909419547));
#79420=CARTESIAN_POINT('Ctrl Pts',(43.6538217579502,766.274642175869,105.965777828192));
#79421=CARTESIAN_POINT('Ctrl Pts',(43.6510694278281,766.275106875837,105.965646244939));
#79422=CARTESIAN_POINT('Ctrl Pts',(42.6536499926894,766.443509923196,105.917961669528));
#79423=CARTESIAN_POINT('Ctrl Pts',(41.6591048139389,766.636536152419,105.871336956417));
#79424=CARTESIAN_POINT('Ctrl Pts',(40.6670269579103,766.852398103184,105.832815900152));
#79425=CARTESIAN_POINT('Ctrl Pts',(40.1555137236564,766.963696066259,105.812954525405));
#79426=CARTESIAN_POINT('Ctrl Pts',(39.6446563246227,767.081064302483,105.795248236246));
#79427=CARTESIAN_POINT('Ctrl Pts',(39.1343984934061,767.204255349575,105.780667209758));
#79428=CARTESIAN_POINT('Ctrl Pts',(39.1337133432591,767.204420764702,105.780647631044));
#79429=CARTESIAN_POINT('Ctrl Pts',(39.1330281931599,767.204586190663,105.780628057937));
#79430=CARTESIAN_POINT('Ctrl Pts',(39.1323430431126,767.204751627457,105.78060849044));
#79431=CARTESIAN_POINT('Ctrl Pts',(38.382626037155,767.385778802471,105.759196997366));
#79432=CARTESIAN_POINT('Ctrl Pts',(37.632946947243,767.579784422389,105.744501930844));
#79433=CARTESIAN_POINT('Ctrl Pts',(36.8891547984958,767.784579867596,105.738993223485));
#79434=CARTESIAN_POINT('Ctrl Pts',(36.8885834704922,767.78473717683,105.73898899209));
#79435=CARTESIAN_POINT('Ctrl Pts',(36.8880121455897,767.784894492491,105.738984766092));
#79436=CARTESIAN_POINT('Ctrl Pts',(36.8874408237884,767.785051814578,105.738980545492));
#79437=CARTESIAN_POINT('Ctrl Pts',(36.1438767224033,767.989803420957,105.733487517914));
#79438=CARTESIAN_POINT('Ctrl Pts',(35.4055582568506,768.205444130159,105.737138832528));
#79439=CARTESIAN_POINT('Ctrl Pts',(34.6723927466888,768.431394424583,105.75135652115));
#79440=CARTESIAN_POINT('Ctrl Pts',(34.6716125182536,768.431634878944,105.751371651492));
#79441=CARTESIAN_POINT('Ctrl Pts',(34.6708322956372,768.431875344902,105.751386794007));
#79442=CARTESIAN_POINT('Ctrl Pts',(34.6700520788396,768.432115822456,105.751401948695));
#79443=CARTESIAN_POINT('Ctrl Pts',(33.6254395721809,768.754085127844,105.771692176961));
#79444=CARTESIAN_POINT('Ctrl Pts',(32.5912678029789,769.096841452481,105.813806788475));
#79445=CARTESIAN_POINT('Ctrl Pts',(31.5674456454017,769.459993643089,105.878413923118));
#79446=CARTESIAN_POINT('Ctrl Pts',(31.1540099390576,769.606640286086,105.904503313886));
#79447=CARTESIAN_POINT('Ctrl Pts',(30.7422617233729,769.75661244681,105.934260091256));
#79448=CARTESIAN_POINT('Ctrl Pts',(30.3321942334713,769.909882838522,105.967726548718));
#79449=CARTESIAN_POINT('Ctrl Pts',(30.3308081024758,769.910400930899,105.96783967374));
#79450=CARTESIAN_POINT('Ctrl Pts',(30.3294219906938,769.910919061048,105.967952840895));
#79451=CARTESIAN_POINT('Ctrl Pts',(30.3280358981258,769.91143722897,105.968066050175));
#79452=CARTESIAN_POINT('Ctrl Pts',(29.1299440841663,770.359324159757,106.065920345501));
#79453=CARTESIAN_POINT('Ctrl Pts',(27.9462089779132,770.835436553784,106.195249342647));
#79454=CARTESIAN_POINT('Ctrl Pts',(26.7770031279921,771.341380969508,106.351250345135));
#79455=CARTESIAN_POINT('Ctrl Pts',(26.5550725248336,771.437415854515,106.380861381188));
#79456=CARTESIAN_POINT('Ctrl Pts',(26.3336653434522,771.534525429352,106.411433324955));
#79457=CARTESIAN_POINT('Ctrl Pts',(26.1127826892852,771.63272049615,106.442933260637));
#79458=CARTESIAN_POINT('Ctrl Pts',(26.1114327061628,771.633320641432,106.443125780877));
#79459=CARTESIAN_POINT('Ctrl Pts',(26.110082742642,771.633920827386,106.443318335444));
#79460=CARTESIAN_POINT('Ctrl Pts',(26.1087327987236,771.634521054016,106.443510924326));
#79461=CARTESIAN_POINT('Ctrl Pts',(24.8834028164008,772.179340490833,106.618321839375));
#79462=CARTESIAN_POINT('Ctrl Pts',(23.6742287046315,772.75767287839,106.821400751351));
#79463=CARTESIAN_POINT('Ctrl Pts',(22.4816817734695,773.372951908832,107.043515560356));
#79464=CARTESIAN_POINT('Ctrl Pts',(22.3255329513332,773.453514856401,107.072598663838));
#79465=CARTESIAN_POINT('Ctrl Pts',(22.1696691850727,773.534711197042,107.102008189595));
#79466=CARTESIAN_POINT('Ctrl Pts',(22.0140915237079,773.616548601358,107.131723468372));
#79467=CARTESIAN_POINT('Ctrl Pts',(22.0139887749509,773.616602649551,107.131743093349));
#79468=CARTESIAN_POINT('Ctrl Pts',(22.0138860262999,773.616656698041,107.131762718459));
#79469=CARTESIAN_POINT('Ctrl Pts',(22.0137832777549,773.616710746827,107.131782343701));
#79470=CARTESIAN_POINT('Ctrl Pts',(21.5862139423887,773.84162491469,107.213449213102));
#79471=CARTESIAN_POINT('Ctrl Pts',(21.1607365610572,774.071528113583,107.297369892082));
#79472=CARTESIAN_POINT('Ctrl Pts',(20.7377097588874,774.306260864954,107.383126887167));
#79473=CARTESIAN_POINT('Ctrl Pts',(20.3168766744112,774.539776347379,107.468439166606));
#79474=CARTESIAN_POINT('Ctrl Pts',(19.898467575598,774.778072073164,107.555569538841));
#79475=CARTESIAN_POINT('Ctrl Pts',(19.4828625856908,775.021031750083,107.64412093627));
#79476=CARTESIAN_POINT('Ctrl Pts',(19.0865928171878,775.252688196147,107.728552650547));
#79477=CARTESIAN_POINT('Ctrl Pts',(18.6928715455575,775.488585453396,107.81427690553));
#79478=CARTESIAN_POINT('Ctrl Pts',(18.3020670071316,775.728649501869,107.900951830872));
#79479=CARTESIAN_POINT('Ctrl Pts',(18.2197962836763,775.779186895889,107.919198315014));
#79480=CARTESIAN_POINT('Ctrl Pts',(18.1376549866794,775.829909027471,107.937486919332));
#79481=CARTESIAN_POINT('Ctrl Pts',(18.0556468322311,775.880815322444,107.955814427592));
#79482=CARTESIAN_POINT('Ctrl Pts',(11.8385912118569,780.22624452509,109.46295982623));
#79483=CARTESIAN_POINT('Ctrl Pts',(12.0670832072855,780.458609040937,109.611864051783));
#79484=CARTESIAN_POINT('Ctrl Pts',(12.0670501393615,780.578030861977,109.274058255276));
#79485=CARTESIAN_POINT('Ctrl Pts',(13.0097844767455,779.287129064763,109.130812234977));
#79486=CARTESIAN_POINT('Ctrl Pts',(13.2324907967292,779.524274195338,109.281682936946));
#79487=CARTESIAN_POINT('Ctrl Pts',(13.231839594492,779.644266255903,108.943836855405));
#79488=CARTESIAN_POINT('Ctrl Pts',(14.2171090900043,778.388492815856,108.815571055468));
#79489=CARTESIAN_POINT('Ctrl Pts',(14.4032018227789,778.651087036577,108.97403106638));
#79490=CARTESIAN_POINT('Ctrl Pts',(14.4327918077321,778.749748784589,108.629696114708));
#79491=CARTESIAN_POINT('Ctrl Pts',(15.4635632812157,777.538177788623,108.526207819986));
#79492=CARTESIAN_POINT('Ctrl Pts',(15.6646167008071,777.782008927919,108.661951401308));
#79493=CARTESIAN_POINT('Ctrl Pts',(15.6662338981911,777.895506807342,108.337269960618));
#79494=CARTESIAN_POINT('Ctrl Pts',(15.4635632805302,777.53817778912,108.52620782016));
#79495=CARTESIAN_POINT('Ctrl Pts',(14.7152684519203,778.048654902706,108.699923801311));
#79496=CARTESIAN_POINT('Ctrl Pts',(13.9814260101745,778.576348492687,108.882905465017));
#79497=CARTESIAN_POINT('Ctrl Pts',(13.2611376128576,779.119610429859,109.073211560677));
#79498=CARTESIAN_POINT('Ctrl Pts',(12.7881788749144,779.476329323478,109.198171134039));
#79499=CARTESIAN_POINT('Ctrl Pts',(12.3210644993871,779.839761579878,109.326288922373));
#79500=CARTESIAN_POINT('Ctrl Pts',(11.859543044092,780.20945181141,109.457020834635));
#79501=CARTESIAN_POINT('Ctrl Pts',(90.0889078210223,777.895440968217,108.337247425881));
#79502=CARTESIAN_POINT('Ctrl Pts',(90.0905250557564,777.781943458107,108.661927889749));
#79503=CARTESIAN_POINT('Ctrl Pts',(90.2915774330859,777.538112255547,108.526185523131));
#79504=CARTESIAN_POINT('Ctrl Pts',(89.2520735400448,777.315878912135,108.138850533236));
#79505=CARTESIAN_POINT('Ctrl Pts',(89.2664127847706,777.214156416844,108.458039407528));
#79506=CARTESIAN_POINT('Ctrl Pts',(89.445908281308,776.961210264209,108.329865285142));
#79507=CARTESIAN_POINT('Ctrl Pts',(88.4006672002774,776.755189453486,107.950220772475));
#79508=CARTESIAN_POINT('Ctrl Pts',(88.4306076665784,776.666770743405,108.259519276078));
#79509=CARTESIAN_POINT('Ctrl Pts',(88.5823401442266,776.406482463236,108.145084435913));
#79510=CARTESIAN_POINT('Ctrl Pts',(87.5346919229366,776.218453858122,107.756965167182));
#79511=CARTESIAN_POINT('Ctrl Pts',(87.5338826891535,776.117574461731,108.040791987471));
#79512=CARTESIAN_POINT('Ctrl Pts',(87.6995907844487,775.880815944701,107.955814324766));
#79513=CARTESIAN_POINT('',(90.2915774337827,777.538112255959,108.526185523262));
#79514=CARTESIAN_POINT('Origin',(90.2661044385266,777.667199844411,108.256579289987));
#79515=CARTESIAN_POINT('Ctrl Pts',(89.8418878191544,777.722889498519,108.285610804474));
#79516=CARTESIAN_POINT('Ctrl Pts',(89.0846481267868,777.205998632613,108.101601829559));
#79517=CARTESIAN_POINT('Ctrl Pts',(88.3156024019357,776.702465886418,107.93123726532));
#79518=CARTESIAN_POINT('Ctrl Pts',(87.5346940946149,776.217967276064,107.758346187656));
#79519=CARTESIAN_POINT('Ctrl Pts',(90.2915774337827,777.538112255959,108.526185523262));
#79520=CARTESIAN_POINT('Ctrl Pts',(89.4450227738296,776.960606185036,108.329659716473));
#79521=CARTESIAN_POINT('Ctrl Pts',(88.5813231070643,776.405876829861,108.144866373145));
#79522=CARTESIAN_POINT('Ctrl Pts',(87.6995908232158,775.880815967783,107.955814333077));
#79523=CARTESIAN_POINT('Ctrl Pts',(93.6887548566012,780.578486380469,109.274219348021));
#79524=CARTESIAN_POINT('Ctrl Pts',(93.6887212389462,780.45906415542,109.612024882815));
#79525=CARTESIAN_POINT('Ctrl Pts',(93.9172164533292,780.22670229016,109.463121730127));
#79526=CARTESIAN_POINT('Ctrl Pts',(92.5237579617488,779.644534103879,108.943928297855));
#79527=CARTESIAN_POINT('Ctrl Pts',(92.5231064640288,779.52454057462,109.281777811047));
#79528=CARTESIAN_POINT('Ctrl Pts',(92.7458176037906,779.287396872426,109.130903091125));
#79529=CARTESIAN_POINT('Ctrl Pts',(91.322583073976,778.74984115456,108.62972748294));
#79530=CARTESIAN_POINT('Ctrl Pts',(91.352184971522,778.65118685501,108.97406731076));
#79531=CARTESIAN_POINT('Ctrl Pts',(91.5382669500913,778.388583935177,108.815601759781));
#79532=CARTESIAN_POINT('Ctrl Pts',(90.0889078212206,777.895440968355,108.337247425928));
#79533=CARTESIAN_POINT('Ctrl Pts',(90.0905250557281,777.781943458083,108.661927889755));
#79534=CARTESIAN_POINT('Ctrl Pts',(90.2915774330965,777.538112255541,108.526185523126));
#79535=CARTESIAN_POINT('Ctrl Pts',(93.8960334963338,780.209723961161,109.457117026756));
#79536=CARTESIAN_POINT('Ctrl Pts',(93.1510424308948,779.612954242215,109.246081306523));
#79537=CARTESIAN_POINT('Ctrl Pts',(92.3913732828177,779.0324108185,109.041831100158));
#79538=CARTESIAN_POINT('Ctrl Pts',(91.6160271246919,778.470077943857,108.846679892652));
#79539=CARTESIAN_POINT('Ctrl Pts',(91.1795712666005,778.153530973496,108.736825878626));
#79540=CARTESIAN_POINT('Ctrl Pts',(90.7381479858848,777.842755555208,108.629855897371));
#79541=CARTESIAN_POINT('Ctrl Pts',(90.2915774337562,777.538112255991,108.526185523279));
#79542=CARTESIAN_POINT('Ctrl Pts',(68.80511438861,640.627119090081,98.0546383469682));
#79543=CARTESIAN_POINT('Ctrl Pts',(68.8068658173116,640.125373764374,98.0546383469682));
#79544=CARTESIAN_POINT('Ctrl Pts',(68.3051174347811,640.125373764374,98.0546383469682));
#79545=CARTESIAN_POINT('Ctrl Pts',(68.8051141943977,640.627174727561,98.1965353136778));
#79546=CARTESIAN_POINT('Ctrl Pts',(68.8069216424176,640.125373764374,98.1966675010902));
#79547=CARTESIAN_POINT('Ctrl Pts',(68.305117426757,640.125373764374,98.1610611371843));
#79548=CARTESIAN_POINT('Ctrl Pts',(68.7901809021704,640.62721634467,98.3359104357707));
#79549=CARTESIAN_POINT('Ctrl Pts',(68.7920160644509,640.125373764374,98.3361724571032));
#79550=CARTESIAN_POINT('Ctrl Pts',(68.2939175755223,640.125373764374,98.2655925281767));
#79551=CARTESIAN_POINT('Ctrl Pts',(68.7316262194072,640.627272620042,98.6097537558797));
#79552=CARTESIAN_POINT('Ctrl Pts',(68.7334618482997,640.125373764374,98.610284735857));
#79553=CARTESIAN_POINT('Ctrl Pts',(68.2500017088632,640.125373764374,98.4709750840453));
#79554=CARTESIAN_POINT('Ctrl Pts',(68.687173049619,640.627287130011,98.7456950617399));
#79555=CARTESIAN_POINT('Ctrl Pts',(68.6889804824384,640.125373764374,98.7463587242848));
#79556=CARTESIAN_POINT('Ctrl Pts',(68.2166618686685,640.125373764374,98.5729310799066));
#79557=CARTESIAN_POINT('Ctrl Pts',(68.5146759823964,640.627287252338,99.1299181624823));
#79558=CARTESIAN_POINT('Ctrl Pts',(68.516317865413,640.125373764374,99.1309508939863));
#79559=CARTESIAN_POINT('Ctrl Pts',(68.0872890739678,640.125373764374,98.8610984080293));
#79560=CARTESIAN_POINT('Ctrl Pts',(68.3463456555463,640.627230853324,99.3607167776682));
#79561=CARTESIAN_POINT('Ctrl Pts',(68.3477940984104,640.125373764374,99.3619233451112));
#79562=CARTESIAN_POINT('Ctrl Pts',(67.9610411711621,640.125373764374,99.0341972964163));
#79563=CARTESIAN_POINT('Ctrl Pts',(68.1332263705067,640.627119090081,99.5499985678032));
#79564=CARTESIAN_POINT('Ctrl Pts',(68.134389413644,640.125373764374,99.5513080841862));
#79565=CARTESIAN_POINT('Ctrl Pts',(67.8012014212036,640.125373764374,99.1761585125944));
#79566=CARTESIAN_POINT('',(68.1332263705066,640.627119090085,99.5499985678032));
#79567=CARTESIAN_POINT('Origin',(66.8051226640402,640.625373779613,98.0546365904861));
#79568=CARTESIAN_POINT('',(67.8012014212036,640.125373764374,99.1761585125944));
#79569=CARTESIAN_POINT('Origin',(67.8012014212036,640.625373764374,99.1761585125944));
#79570=CARTESIAN_POINT('Ctrl Pts',(68.3051174347811,640.125373764374,98.0546383469682));
#79571=CARTESIAN_POINT('Ctrl Pts',(68.3051174347811,640.125373764374,98.16106912087));
#79572=CARTESIAN_POINT('Ctrl Pts',(68.2939175755208,640.125373764374,98.2655925281833));
#79573=CARTESIAN_POINT('Ctrl Pts',(68.2719596426717,640.125373764374,98.3682838062134));
#79574=CARTESIAN_POINT('Ctrl Pts',(68.2500017098227,640.125373764374,98.4709750842436));
#79575=CARTESIAN_POINT('Ctrl Pts',(68.2166618704369,640.125373764374,98.5729310807814));
#79576=CARTESIAN_POINT('Ctrl Pts',(68.1735376049674,640.125373764374,98.6689868564858));
#79577=CARTESIAN_POINT('Ctrl Pts',(68.1453423196876,640.125373764374,98.7317895493379));
#79578=CARTESIAN_POINT('Ctrl Pts',(68.1128287472829,640.125373764374,98.7926468994039));
#79579=CARTESIAN_POINT('Ctrl Pts',(68.0762480466093,640.125373764374,98.8510410845592));
#79580=CARTESIAN_POINT('Ctrl Pts',(68.0385887645426,640.125373764374,98.9111570213597));
#79581=CARTESIAN_POINT('Ctrl Pts',(67.9966191995703,640.125373764374,98.9686613932213));
#79582=CARTESIAN_POINT('Ctrl Pts',(67.9506628544449,640.125373764374,99.0230191503698));
#79583=CARTESIAN_POINT('Ctrl Pts',(67.9047065093195,640.125373764374,99.0773769075182));
#79584=CARTESIAN_POINT('Ctrl Pts',(67.8547638793613,640.125373764374,99.1285871723741));
#79585=CARTESIAN_POINT('Ctrl Pts',(67.8012014212036,640.125373764374,99.1761585125944));
#79586=CARTESIAN_POINT('Origin',(52.8776183915471,640.625373764374,82.3731046594733));
#79587=CARTESIAN_POINT('',(37.6220104125875,640.627119090081,99.5499985678032));
#79588=CARTESIAN_POINT('',(37.9540353618906,640.125373764374,99.1761585125945));
#79589=CARTESIAN_POINT('Origin',(37.9540353618906,640.625373764375,99.1761585125944));
#79590=CARTESIAN_POINT('Origin',(52.8776183915471,640.125373764374,82.3731046594733));
#79591=CARTESIAN_POINT('Origin',(52.8776183915471,640.627119090082,82.3731046594733));
#79592=CARTESIAN_POINT('Ctrl Pts',(37.6220104125875,640.627119090081,99.5499985678032));
#79593=CARTESIAN_POINT('Ctrl Pts',(37.6208473694502,640.125373764374,99.5513080841862));
#79594=CARTESIAN_POINT('Ctrl Pts',(37.9540353618906,640.125373764374,99.1761585125945));
#79595=CARTESIAN_POINT('Ctrl Pts',(37.5159163554561,640.627174727549,99.4557711821737));
#79596=CARTESIAN_POINT('Ctrl Pts',(37.5146172779777,640.125373764374,99.4570348037583));
#79597=CARTESIAN_POINT('Ctrl Pts',(37.8744646789089,640.125373764374,99.1054880329923));
#79598=CARTESIAN_POINT('Ctrl Pts',(37.4216242255084,640.627216344653,99.3520531890113));
#79599=CARTESIAN_POINT('Ctrl Pts',(37.4202096694391,640.125373764374,99.3532513153967));
#79600=CARTESIAN_POINT('Ctrl Pts',(37.8037454661792,640.125373764374,99.0276995934824));
#79601=CARTESIAN_POINT('Ctrl Pts',(37.2557592423392,640.627272620036,99.1264260137889));
#79602=CARTESIAN_POINT('Ctrl Pts',(37.25414328015,640.125373764374,99.1274458860118));
#79603=CARTESIAN_POINT('Ctrl Pts',(37.6793465830514,640.125373764374,98.8584792771019));
#79604=CARTESIAN_POINT('Ctrl Pts',(37.1836373152616,640.627287130011,99.0029167000581));
#79605=CARTESIAN_POINT('Ctrl Pts',(37.181940872061,640.125373764374,99.0038273821317));
#79606=CARTESIAN_POINT('Ctrl Pts',(37.6252551007653,640.125373764374,98.7658473086436));
#79607=CARTESIAN_POINT('Ctrl Pts',(37.0109069525407,640.627287252338,98.6187984225216));
#79608=CARTESIAN_POINT('Ctrl Pts',(37.0090444961387,640.125373764374,98.6193402438448));
#79609=CARTESIAN_POINT('Ctrl Pts',(37.495707323009,640.125373764374,98.4777586030618));
#79610=CARTESIAN_POINT('Ctrl Pts',(36.9501227846132,640.627230853348,98.3396776876425));
#79611=CARTESIAN_POINT('Ctrl Pts',(36.9482588084213,640.125373764374,98.3399594403062));
#79612=CARTESIAN_POINT('Ctrl Pts',(37.4501193563501,640.125373764374,98.2684179824933));
#79613=CARTESIAN_POINT('Ctrl Pts',(36.9501223944842,640.627119090081,98.0546383469683));
#79614=CARTESIAN_POINT('Ctrl Pts',(36.9483709657826,640.125373764374,98.0546383469683));
#79615=CARTESIAN_POINT('Ctrl Pts',(37.4501193483131,640.125373764374,98.0546383469682));
#79616=CARTESIAN_POINT('',(36.9501223944842,640.627119090084,98.0546383469682));
#79617=CARTESIAN_POINT('',(37.4501193483131,640.125373764374,98.0546383469682));
#79618=CARTESIAN_POINT('Origin',(37.4501193483131,640.625373764374,98.0546383469682));
#79619=CARTESIAN_POINT('Ctrl Pts',(37.9540353618906,640.125373764374,99.1761585125945));
#79620=CARTESIAN_POINT('Ctrl Pts',(37.8744587042996,640.125373764374,99.1054827373954));
#79621=CARTESIAN_POINT('Ctrl Pts',(37.8037454661753,640.125373764374,99.0276995934772));
#79622=CARTESIAN_POINT('Ctrl Pts',(37.7415460242206,640.125373764374,98.9430894355824));
#79623=CARTESIAN_POINT('Ctrl Pts',(37.6793465822659,640.125373764374,98.8584792776875));
#79624=CARTESIAN_POINT('Ctrl Pts',(37.6252550989367,640.125373764374,98.7658473093854));
#79625=CARTESIAN_POINT('Ctrl Pts',(37.5820725069809,640.125373764374,98.6698177406556));
#79626=CARTESIAN_POINT('Ctrl Pts',(37.5538390869676,640.125373764374,98.6070321822894));
#79627=CARTESIAN_POINT('Ctrl Pts',(37.5299277455258,640.125373764374,98.5423097194069));
#79628=CARTESIAN_POINT('Ctrl Pts',(37.5105588672889,640.125373764374,98.4761820014583));
#79629=CARTESIAN_POINT('Ctrl Pts',(37.490618897988,640.125373764374,98.4081045088073));
#79630=CARTESIAN_POINT('Ctrl Pts',(37.4754938161077,640.125373764374,98.3385385037225));
#79631=CARTESIAN_POINT('Ctrl Pts',(37.4653688468807,640.125373764374,98.268081166164));
#79632=CARTESIAN_POINT('Ctrl Pts',(37.4552438776536,640.125373764374,98.1976238286054));
#79633=CARTESIAN_POINT('Ctrl Pts',(37.450119348313,640.125373764374,98.1262761116766));
#79634=CARTESIAN_POINT('Ctrl Pts',(37.4501193483131,640.125373764374,98.0546383469682));
#79635=CARTESIAN_POINT('Origin',(38.9501141189669,640.625373779629,98.0546365905253));
#79636=CARTESIAN_POINT('Ctrl Pts',(68.1332263705066,640.627119090081,81.6674251557765));
#79637=CARTESIAN_POINT('Ctrl Pts',(68.134389413644,640.125373764374,81.6661156393935));
#79638=CARTESIAN_POINT('Ctrl Pts',(67.8012014212035,640.125373764374,82.0412652109852));
#79639=CARTESIAN_POINT('Ctrl Pts',(68.2393204276379,640.62717472755,81.7616525414059));
#79640=CARTESIAN_POINT('Ctrl Pts',(68.2406195051122,640.125373764374,81.7603889198256));
#79641=CARTESIAN_POINT('Ctrl Pts',(67.8807721041838,640.125373764374,82.1119356905887));
#79642=CARTESIAN_POINT('Ctrl Pts',(68.3336125575859,640.627216344653,81.8653705345686));
#79643=CARTESIAN_POINT('Ctrl Pts',(68.3350271136558,640.125373764374,81.864172408183));
#79644=CARTESIAN_POINT('Ctrl Pts',(67.9514913169153,640.125373764374,82.1897241300973));
#79645=CARTESIAN_POINT('Ctrl Pts',(68.4994775407548,640.627272620036,82.0909977097906));
#79646=CARTESIAN_POINT('Ctrl Pts',(68.5010935029434,640.125373764374,82.0899778375679));
#79647=CARTESIAN_POINT('Ctrl Pts',(68.0758902000424,640.125373764374,82.3589444464778));
#79648=CARTESIAN_POINT('Ctrl Pts',(68.5715994678325,640.627287130011,82.2145070235214));
#79649=CARTESIAN_POINT('Ctrl Pts',(68.5732959110343,640.125373764374,82.2135963414472));
#79650=CARTESIAN_POINT('Ctrl Pts',(68.1299816823292,640.125373764374,82.4515764149354));
#79651=CARTESIAN_POINT('Ctrl Pts',(68.7443298305536,640.627287252338,82.5986253010585));
#79652=CARTESIAN_POINT('Ctrl Pts',(68.7461922869533,640.125373764374,82.5980834797364));
#79653=CARTESIAN_POINT('Ctrl Pts',(68.2595294600845,640.125373764374,82.7396651205193));
#79654=CARTESIAN_POINT('Ctrl Pts',(68.805113998481,640.627230853348,82.877746035937));
#79655=CARTESIAN_POINT('Ctrl Pts',(68.8069779746714,640.125373764374,82.8774642832724));
#79656=CARTESIAN_POINT('Ctrl Pts',(68.3051174267426,640.125373764374,82.9490057410853));
#79657=CARTESIAN_POINT('Ctrl Pts',(68.80511438861,640.627119090081,83.1627853766115));
#79658=CARTESIAN_POINT('Ctrl Pts',(68.8068658173116,640.125373764374,83.1627853766115));
#79659=CARTESIAN_POINT('Ctrl Pts',(68.3051174347811,640.125373764374,83.1627853766115));
#79660=CARTESIAN_POINT('Origin',(66.8051226640255,640.625373779627,83.1627871331001));
#79661=CARTESIAN_POINT('Ctrl Pts',(67.8012014212036,640.125373764374,82.0412652109852));
#79662=CARTESIAN_POINT('Ctrl Pts',(67.8807780787945,640.125373764374,82.1119409861843));
#79663=CARTESIAN_POINT('Ctrl Pts',(67.951491316919,640.125373764374,82.1897241301024));
#79664=CARTESIAN_POINT('Ctrl Pts',(68.0136907588737,640.125373764374,82.2743342879973));
#79665=CARTESIAN_POINT('Ctrl Pts',(68.0758902008283,640.125373764374,82.3589444458922));
#79666=CARTESIAN_POINT('Ctrl Pts',(68.1299816841575,640.125373764374,82.4515764141943));
#79667=CARTESIAN_POINT('Ctrl Pts',(68.173164276113,640.125373764374,82.5476059829244));
#79668=CARTESIAN_POINT('Ctrl Pts',(68.2013976961101,640.125373764374,82.6103915412553));
#79669=CARTESIAN_POINT('Ctrl Pts',(68.2253090375408,640.125373764374,82.6751140041001));
#79670=CARTESIAN_POINT('Ctrl Pts',(68.244677915772,640.125373764374,82.7412417220098));
#79671=CARTESIAN_POINT('Ctrl Pts',(68.2646178850837,640.125373764374,82.8093192146777));
#79672=CARTESIAN_POINT('Ctrl Pts',(68.2797429669723,640.125373764374,82.8788852197806));
#79673=CARTESIAN_POINT('Ctrl Pts',(68.289867936205,640.125373764374,82.9493425573579));
#79674=CARTESIAN_POINT('Ctrl Pts',(68.2999929054377,640.125373764374,83.0197998949352));
#79675=CARTESIAN_POINT('Ctrl Pts',(68.3051174347812,640.125373764374,83.0911476118835));
#79676=CARTESIAN_POINT('Ctrl Pts',(68.3051174347811,640.125373764374,83.1627853766115));
#79677=CARTESIAN_POINT('Origin',(37.4501193483131,640.625373764374,82.287785267134));
#79678=CARTESIAN_POINT('',(36.9501223944842,640.627119090078,83.1627853766115));
#79679=CARTESIAN_POINT('',(37.4501193483131,640.125373764374,83.1627853766115));
#79680=CARTESIAN_POINT('Origin',(37.4501193483131,640.62537376437,83.1627853766115));
#79681=CARTESIAN_POINT('',(37.4501193483131,640.125373764374,83.1619984528873));
#79682=CARTESIAN_POINT('',(36.9501223944842,640.627119090081,98.0554252706924));
#79683=CARTESIAN_POINT('Ctrl Pts',(36.9501223944842,640.627119090081,83.1627853766114));
#79684=CARTESIAN_POINT('Ctrl Pts',(36.9483709657826,640.125373764374,83.1627853766115));
#79685=CARTESIAN_POINT('Ctrl Pts',(37.4501193483131,640.125373764374,83.1627853766115));
#79686=CARTESIAN_POINT('Ctrl Pts',(36.9501225886964,640.627174727561,83.0208884099024));
#79687=CARTESIAN_POINT('Ctrl Pts',(36.9483151406832,640.125373764374,83.0207562224895));
#79688=CARTESIAN_POINT('Ctrl Pts',(37.4501193563416,640.125373764374,83.0563625863953));
#79689=CARTESIAN_POINT('Ctrl Pts',(36.9650558809238,640.62721634467,82.8815132878083));
#79690=CARTESIAN_POINT('Ctrl Pts',(36.9632207186425,640.125373764374,82.8812512664765));
#79691=CARTESIAN_POINT('Ctrl Pts',(37.4613192075715,640.125373764374,82.951831195403));
#79692=CARTESIAN_POINT('Ctrl Pts',(37.0236105636868,640.627272620042,82.6076699677006));
#79693=CARTESIAN_POINT('Ctrl Pts',(37.0217749347951,640.125373764374,82.6071389877227));
#79694=CARTESIAN_POINT('Ctrl Pts',(37.5052350742313,640.125373764374,82.7464486395343));
#79695=CARTESIAN_POINT('Ctrl Pts',(37.0680637334749,640.627287130011,82.4717286618402));
#79696=CARTESIAN_POINT('Ctrl Pts',(37.066256300655,640.125373764374,82.4710649992963));
#79697=CARTESIAN_POINT('Ctrl Pts',(37.5385749144261,640.125373764374,82.6444926436739));
#79698=CARTESIAN_POINT('Ctrl Pts',(37.2405608006982,640.627287252338,82.0875055610965));
#79699=CARTESIAN_POINT('Ctrl Pts',(37.2389189176825,640.125373764374,82.0864728295907));
#79700=CARTESIAN_POINT('Ctrl Pts',(37.6679477091256,640.125373764374,82.356325315549));
#79701=CARTESIAN_POINT('Ctrl Pts',(37.4088911275473,640.627230853324,81.856706945912));
#79702=CARTESIAN_POINT('Ctrl Pts',(37.4074426846854,640.125373764374,81.8555003784741));
#79703=CARTESIAN_POINT('Ctrl Pts',(37.794195611936,640.125373764374,82.1832264271683));
#79704=CARTESIAN_POINT('Ctrl Pts',(37.6220104125875,640.627119090081,81.6674251557765));
#79705=CARTESIAN_POINT('Ctrl Pts',(37.6208473694501,640.125373764374,81.6661156393935));
#79706=CARTESIAN_POINT('Ctrl Pts',(37.9540353618906,640.125373764374,82.0412652109853));
#79707=CARTESIAN_POINT('Origin',(38.9501141190175,640.62537377961,83.1627871330772));
#79708=CARTESIAN_POINT('Ctrl Pts',(37.4501193483131,640.125373764374,83.1627853766115));
#79709=CARTESIAN_POINT('Ctrl Pts',(37.4501193483131,640.125373764374,83.0563546027096));
#79710=CARTESIAN_POINT('Ctrl Pts',(37.4613192075729,640.125373764374,82.9518311953963));
#79711=CARTESIAN_POINT('Ctrl Pts',(37.4832771404222,640.125373764374,82.8491399173662));
#79712=CARTESIAN_POINT('Ctrl Pts',(37.5052350732715,640.125373764374,82.7464486393361));
#79713=CARTESIAN_POINT('Ctrl Pts',(37.5385749126573,640.125373764374,82.6444926427984));
#79714=CARTESIAN_POINT('Ctrl Pts',(37.5816991781264,640.125373764374,82.5484368670937));
#79715=CARTESIAN_POINT('Ctrl Pts',(37.6098944633952,640.125373764374,82.4856341742655));
#79716=CARTESIAN_POINT('Ctrl Pts',(37.6424080357855,640.125373764374,82.4247768242222));
#79717=CARTESIAN_POINT('Ctrl Pts',(37.6789887364421,640.125373764374,82.3663826390874));
#79718=CARTESIAN_POINT('Ctrl Pts',(37.7166480185124,640.125373764374,82.3062667022739));
#79719=CARTESIAN_POINT('Ctrl Pts',(37.7586175834904,640.125373764374,82.2487623304001));
#79720=CARTESIAN_POINT('Ctrl Pts',(37.8045739286231,640.125373764374,82.1944045732403));
#79721=CARTESIAN_POINT('Ctrl Pts',(37.8505302737557,640.125373764374,82.1400468160806));
#79722=CARTESIAN_POINT('Ctrl Pts',(37.9004729037229,640.125373764374,82.0888365512145));
#79723=CARTESIAN_POINT('Ctrl Pts',(37.9540353618905,640.125373764374,82.0412652109853));
#79724=CARTESIAN_POINT('Ctrl Pts',(10.5317017736754,779.984261556367,107.006332650571));
#79725=CARTESIAN_POINT('Ctrl Pts',(10.3604849461703,779.152731480618,108.803696199278));
#79726=CARTESIAN_POINT('Ctrl Pts',(11.5614808152667,780.530792792794,109.582854450735));
#79727=CARTESIAN_POINT('Ctrl Pts',(10.5733299874904,779.865842760521,107.219090474412));
#79728=CARTESIAN_POINT('Ctrl Pts',(10.5582433475702,779.256981704553,108.887216975226));
#79729=CARTESIAN_POINT('Ctrl Pts',(11.7093120354819,780.435428829693,109.551490669409));
#79730=CARTESIAN_POINT('Ctrl Pts',(10.7318267936817,779.743920761265,107.158653158791));
#79731=CARTESIAN_POINT('Ctrl Pts',(10.7068785033582,779.120077753409,108.835843568229));
#79732=CARTESIAN_POINT('Ctrl Pts',(11.8566239029334,780.315075067507,109.508795773261));
#79733=CARTESIAN_POINT('Ctrl Pts',(10.9216035979647,779.592391477705,107.105565628044));
#79734=CARTESIAN_POINT('Ctrl Pts',(10.8970342369242,778.968863920289,108.782484477585));
#79735=CARTESIAN_POINT('Ctrl Pts',(12.0415407060361,780.167617208107,109.456683482087));
#79736=CARTESIAN_POINT('Ctrl Pts',(10.9595078561701,779.562175400004,107.095035038181));
#79737=CARTESIAN_POINT('Ctrl Pts',(10.9350411255372,778.938762360073,108.771872584246));
#79738=CARTESIAN_POINT('Ctrl Pts',(12.0784988928585,780.138215973205,109.446293459633));
#79739=CARTESIAN_POINT('Ctrl Pts',(11.0732462957153,779.471645605594,107.063645836025));
#79740=CARTESIAN_POINT('Ctrl Pts',(11.0491718823668,778.848720729622,108.74015903354));
#79741=CARTESIAN_POINT('Ctrl Pts',(12.1894723235861,780.050134608815,109.415168109637));
#79742=CARTESIAN_POINT('Ctrl Pts',(11.1491060843021,779.411450286746,107.042989781577));
#79743=CARTESIAN_POINT('Ctrl Pts',(11.125405322853,778.789043900988,108.719179562979));
#79744=CARTESIAN_POINT('Ctrl Pts',(12.26358634686,779.991576829024,109.394477502784));
#79745=CARTESIAN_POINT('Ctrl Pts',(11.3767577611053,779.231301369849,106.981776204739));
#79746=CARTESIAN_POINT('Ctrl Pts',(11.3544757071218,778.611001152522,108.656698819988));
#79747=CARTESIAN_POINT('Ctrl Pts',(12.4862824988523,779.816350545124,109.33256920393));
#79748=CARTESIAN_POINT('Ctrl Pts',(11.5286209740312,779.111784371392,106.941972898753));
#79749=CARTESIAN_POINT('Ctrl Pts',(11.50768553079,778.493617265097,108.615653000625));
#79750=CARTESIAN_POINT('Ctrl Pts',(12.635218701962,779.70012801209,109.291514647201));
#79751=CARTESIAN_POINT('Ctrl Pts',(11.9842915999363,778.754706931681,106.82514494408));
#79752=CARTESIAN_POINT('Ctrl Pts',(11.9682792420486,778.144895323507,108.494096092455));
#79753=CARTESIAN_POINT('Ctrl Pts',(13.0831312259875,779.352924298943,109.168887274619));
#79754=CARTESIAN_POINT('Ctrl Pts',(12.2881684816843,778.51861469024,106.750692042409));
#79755=CARTESIAN_POINT('Ctrl Pts',(12.2767214939561,777.916865625875,108.415119273732));
#79756=CARTESIAN_POINT('Ctrl Pts',(13.3832175329536,779.123384899081,109.087842851556));
#79757=CARTESIAN_POINT('Ctrl Pts',(13.3131173672748,777.725974089015,106.507342906962));
#79758=CARTESIAN_POINT('Ctrl Pts',(13.3177396755757,777.158567029708,108.153655030184));
#79759=CARTESIAN_POINT('Ctrl Pts',(14.3987831512332,778.352459845658,108.815709181203));
#79760=CARTESIAN_POINT('Ctrl Pts',(14.0325982015706,777.175560053502,106.349270625002));
#79761=CARTESIAN_POINT('Ctrl Pts',(14.0533667512555,776.640899205561,107.977072247212));
#79762=CARTESIAN_POINT('Ctrl Pts',(15.1179090626436,777.816088388095,108.626470714689));
#79763=CARTESIAN_POINT('Ctrl Pts',(14.7464540540325,776.626446606295,106.193899773879));
#79764=CARTESIAN_POINT('Ctrl Pts',(14.7919275351275,776.119102455067,107.799271902089));
#79765=CARTESIAN_POINT('Ctrl Pts',(15.8356919568668,777.277268015822,108.43638579439));
#79766=CARTESIAN_POINT('',(14.3866390709116,776.891105572714,106.313407256592));
#79767=CARTESIAN_POINT('Ctrl Pts',(14.3866390402624,776.891105535654,106.313407246381));
#79768=CARTESIAN_POINT('Ctrl Pts',(14.3889611516474,776.87128206777,106.378381133509));
#79769=CARTESIAN_POINT('Ctrl Pts',(14.3934547660474,776.854060889204,106.444094869398));
#79770=CARTESIAN_POINT('Ctrl Pts',(14.400093388946,776.839542736536,106.51017865051));
#79771=CARTESIAN_POINT('Ctrl Pts',(14.4069781065082,776.824486393953,106.578712166474));
#79772=CARTESIAN_POINT('Ctrl Pts',(14.416169310853,776.812336724029,106.64764312285));
#79773=CARTESIAN_POINT('Ctrl Pts',(14.4276103046054,776.80316153864,106.716583175345));
#79774=CARTESIAN_POINT('Ctrl Pts',(14.4399117991466,776.793296268593,106.790708351689));
#79775=CARTESIAN_POINT('Ctrl Pts',(14.4548137441145,776.78686922282,106.864843683666));
#79776=CARTESIAN_POINT('Ctrl Pts',(14.472222712476,776.78392174325,106.938541809043));
#79777=CARTESIAN_POINT('Ctrl Pts',(14.4758003829653,776.783316014613,106.953687313521));
#79778=CARTESIAN_POINT('Ctrl Pts',(14.4794838753247,776.782857120754,106.96881447167));
#79779=CARTESIAN_POINT('Ctrl Pts',(14.4832722978711,776.782545250895,106.983919577223));
#79780=CARTESIAN_POINT('Ctrl Pts',(14.5008198470155,776.781100704622,107.053884735218));
#79781=CARTESIAN_POINT('Ctrl Pts',(14.5206170789698,776.782814197739,107.123360471363));
#79782=CARTESIAN_POINT('Ctrl Pts',(14.5425448232576,776.787676006415,107.191926901758));
#79783=CARTESIAN_POINT('Ctrl Pts',(14.5650401209042,776.792663652742,107.262268029421));
#79784=CARTESIAN_POINT('Ctrl Pts',(14.5897774106074,776.800964417161,107.331652085065));
#79785=CARTESIAN_POINT('Ctrl Pts',(14.6166037709663,776.812526033795,107.39965284292));
#79786=CARTESIAN_POINT('Ctrl Pts',(14.6442355350974,776.824434763102,107.469695177276));
#79787=CARTESIAN_POINT('Ctrl Pts',(14.6740836141183,776.83980295605,107.538269973234));
#79788=CARTESIAN_POINT('Ctrl Pts',(14.7059579927268,776.85853302803,107.604939969069));
#79789=CARTESIAN_POINT('Ctrl Pts',(14.7090669241534,776.860359903155,107.611442760789));
#79790=CARTESIAN_POINT('Ctrl Pts',(14.7121951155176,776.862218731124,107.617927452371));
#79791=CARTESIAN_POINT('Ctrl Pts',(14.7153423794039,776.864109401912,107.624393651513));
#79792=CARTESIAN_POINT('Ctrl Pts',(14.7471339629307,776.883207710938,107.689710929489));
#79793=CARTESIAN_POINT('Ctrl Pts',(14.7808684292452,776.905555339565,107.753128713198));
#79794=CARTESIAN_POINT('Ctrl Pts',(14.8163336489197,776.931011584379,107.814248718621));
#79795=CARTESIAN_POINT('Ctrl Pts',(14.8528604552702,776.957229815458,107.877198239947));
#79796=CARTESIAN_POINT('Ctrl Pts',(14.8912233634063,776.986745851564,107.937710200034));
#79797=CARTESIAN_POINT('Ctrl Pts',(14.9311656072414,777.019362440652,107.995378735158));
#79798=CARTESIAN_POINT('Ctrl Pts',(14.968877269302,777.050157550468,108.04982676059));
#79799=CARTESIAN_POINT('Ctrl Pts',(15.0079966692538,777.083716400361,108.101740112061));
#79800=CARTESIAN_POINT('Ctrl Pts',(15.0482858219991,777.119834762961,108.150803170287));
#79801=CARTESIAN_POINT('Ctrl Pts',(15.0506688580393,777.121971103736,108.15370516817));
#79802=CARTESIAN_POINT('Ctrl Pts',(15.0530559801051,777.12411638773,108.156597202236));
#79803=CARTESIAN_POINT('Ctrl Pts',(15.0554471365295,777.126270568379,108.159479210262));
#79804=CARTESIAN_POINT('Ctrl Pts',(15.0974465589804,777.164107634247,108.210100186517));
#79805=CARTESIAN_POINT('Ctrl Pts',(15.1406848085548,777.204685542196,108.257617141791));
#79806=CARTESIAN_POINT('Ctrl Pts',(15.1848969486944,777.247755041553,108.301740662617));
#79807=CARTESIAN_POINT('Ctrl Pts',(15.2271686575255,777.288934259085,108.343927641556));
#79808=CARTESIAN_POINT('Ctrl Pts',(15.2703307319288,777.33239141631,108.38301211459));
#79809=CARTESIAN_POINT('Ctrl Pts',(15.3141296941221,777.377872296008,108.418761739622));
#79810=CARTESIAN_POINT('Ctrl Pts',(15.35581599226,777.421159383548,108.452786964257));
#79811=CARTESIAN_POINT('Ctrl Pts',(15.3980790830262,777.466279671584,108.483790788085));
#79812=CARTESIAN_POINT('Ctrl Pts',(15.4406805907297,777.512978560241,108.511598648713));
#79813=CARTESIAN_POINT('Ctrl Pts',(15.4482978589518,777.521328451589,108.516570771637));
#79814=CARTESIAN_POINT('Ctrl Pts',(15.4559258968458,777.529728716795,108.52144079969));
#79815=CARTESIAN_POINT('Ctrl Pts',(15.4635632778611,777.538177775594,108.526207848409));
#79816=CARTESIAN_POINT('Ctrl Pts',(14.3866390862365,776.891105591244,106.313407261698));
#79817=CARTESIAN_POINT('Ctrl Pts',(14.1635282499457,777.062166931795,106.362258830835));
#79818=CARTESIAN_POINT('Ctrl Pts',(13.9402770911972,777.233217022154,106.411497164547));
#79819=CARTESIAN_POINT('Ctrl Pts',(13.7171561772671,777.404295799324,106.461350719229));
#79820=CARTESIAN_POINT('Ctrl Pts',(13.5059079782952,777.566271128857,106.508551465469));
#79821=CARTESIAN_POINT('Ctrl Pts',(13.2947768511875,777.728271930287,106.556303545477));
#79822=CARTESIAN_POINT('Ctrl Pts',(13.0839822957079,777.890366583229,106.604830521648));
#79823=CARTESIAN_POINT('Ctrl Pts',(12.8883440114655,778.040806520893,106.649868375382));
#79824=CARTESIAN_POINT('Ctrl Pts',(12.6929958066475,778.191327236408,106.695573695199));
#79825=CARTESIAN_POINT('Ctrl Pts',(12.4981009461385,778.342015811371,106.742152379873));
#79826=CARTESIAN_POINT('Ctrl Pts',(12.3101448643633,778.487339469698,106.78707273869));
#79827=CARTESIAN_POINT('Ctrl Pts',(12.1226106083063,778.632819007354,106.832805230861));
#79828=CARTESIAN_POINT('Ctrl Pts',(11.9356302264546,778.778566284359,106.87956213152));
#79829=CARTESIAN_POINT('Ctrl Pts',(11.7548581546475,778.919474314193,106.924766562699));
#79830=CARTESIAN_POINT('Ctrl Pts',(11.5746039399841,779.060632360689,106.970928362183));
#79831=CARTESIAN_POINT('Ctrl Pts',(11.3949707652917,779.202177093405,107.018267738977));
#79832=CARTESIAN_POINT('Ctrl Pts',(11.2229617632804,779.337714241574,107.063597890114));
#79833=CARTESIAN_POINT('Ctrl Pts',(11.051522286338,779.47360579314,107.110007706059));
#79834=CARTESIAN_POINT('Ctrl Pts',(10.8807262369361,779.610007641348,107.15771846644));
#79835=CARTESIAN_POINT('Ctrl Pts',(10.8510478741863,779.6337094983,107.166008923149));
#79836=CARTESIAN_POINT('Ctrl Pts',(10.8213888951291,779.65742685787,107.174338733481));
#79837=CARTESIAN_POINT('Ctrl Pts',(10.791749630326,779.68116066072,107.182709152208));
#79838=CARTESIAN_POINT('Ctrl Pts',(93.9784435005612,780.377188811389,109.530513700775));
#79839=CARTESIAN_POINT('Ctrl Pts',(95.1084144693317,779.190184574876,108.861662561019));
#79840=CARTESIAN_POINT('Ctrl Pts',(95.0949273018122,779.794272325681,107.197683299583));
#79841=CARTESIAN_POINT('Ctrl Pts',(93.9029214534442,780.319268354671,109.510319941364));
#79842=CARTESIAN_POINT('Ctrl Pts',(95.0270033001491,779.15409027672,108.854135188967));
#79843=CARTESIAN_POINT('Ctrl Pts',(95.0299861041092,779.732879674436,107.2059504738));
#79844=CARTESIAN_POINT('Ctrl Pts',(93.8271635469066,780.258099564455,109.488660207096));
#79845=CARTESIAN_POINT('Ctrl Pts',(94.9497485946087,779.087848677435,108.829971302735));
#79846=CARTESIAN_POINT('Ctrl Pts',(94.9503799339584,779.670399483667,107.179461492168));
#79847=CARTESIAN_POINT('Ctrl Pts',(93.7145339590534,780.168283129866,109.456918645028));
#79848=CARTESIAN_POINT('Ctrl Pts',(94.8340030377784,778.995794648529,108.797486372228));
#79849=CARTESIAN_POINT('Ctrl Pts',(94.8347839700442,779.578107160797,107.147122444466));
#79850=CARTESIAN_POINT('Ctrl Pts',(93.6777850797537,780.139047238446,109.446587044326));
#79851=CARTESIAN_POINT('Ctrl Pts',(94.7962349321268,778.965876172659,108.786938170426));
#79852=CARTESIAN_POINT('Ctrl Pts',(94.797091755628,779.548063554189,107.13664949813));
#79853=CARTESIAN_POINT('Ctrl Pts',(93.5674424188274,780.051462002609,109.415636978074));
#79854=CARTESIAN_POINT('Ctrl Pts',(94.6828244381048,778.87637858051,108.755412779786));
#79855=CARTESIAN_POINT('Ctrl Pts',(94.6839894976143,779.458054320114,107.105430896486));
#79856=CARTESIAN_POINT('Ctrl Pts',(93.4937527041494,779.993235106026,109.395063251624));
#79857=CARTESIAN_POINT('Ctrl Pts',(94.6070763781049,778.81705748974,108.734554862737));
#79858=CARTESIAN_POINT('Ctrl Pts',(94.608553905792,779.398210244639,107.084885469161));
#79859=CARTESIAN_POINT('Ctrl Pts',(93.2723395706119,779.819001952487,109.33350570485));
#79860=CARTESIAN_POINT('Ctrl Pts',(94.3794751460829,778.640062134937,108.672427820456));
#79861=CARTESIAN_POINT('Ctrl Pts',(94.3821747887695,779.219127121472,107.023995285396));
#79862=CARTESIAN_POINT('Ctrl Pts',(93.1242721691852,779.703442160639,109.292685135209));
#79863=CARTESIAN_POINT('Ctrl Pts',(94.2272622385821,778.523350322706,108.631603283016));
#79864=CARTESIAN_POINT('Ctrl Pts',(94.2311597815261,779.10033662908,106.984396198984));
#79865=CARTESIAN_POINT('Ctrl Pts',(92.6789965002652,779.358229445953,109.170760515774));
#79866=CARTESIAN_POINT('Ctrl Pts',(93.7696917507482,778.176575029635,108.510672591972));
#79867=CARTESIAN_POINT('Ctrl Pts',(93.7780323027825,778.745482414722,106.868153397216));
#79868=CARTESIAN_POINT('Ctrl Pts',(92.3807087316349,779.130021392018,109.090185763539));
#79869=CARTESIAN_POINT('Ctrl Pts',(93.463312097639,777.949755097055,108.432064949768));
#79870=CARTESIAN_POINT('Ctrl Pts',(93.4758459227127,778.510928031655,106.794052998108));
#79871=CARTESIAN_POINT('Ctrl Pts',(91.436392783065,778.413053495081,108.837097455752));
#79872=CARTESIAN_POINT('Ctrl Pts',(92.4955494384007,777.24368808485,108.188425098313));
#79873=CARTESIAN_POINT('Ctrl Pts',(92.522429303692,777.774489190713,106.567468299851));
#79874=CARTESIAN_POINT('Ctrl Pts',(90.7875519064439,777.928254343851,108.666045113778));
#79875=CARTESIAN_POINT('Ctrl Pts',(91.8317630359771,776.774133286743,108.027925378993));
#79876=CARTESIAN_POINT('Ctrl Pts',(91.8723885912789,777.277552943272,106.423405302575));
#79877=CARTESIAN_POINT('Ctrl Pts',(90.1393011458404,777.442136168392,108.494548400935));
#79878=CARTESIAN_POINT('Ctrl Pts',(91.1655083296893,776.302751793624,107.867095841556));
#79879=CARTESIAN_POINT('Ctrl Pts',(91.2264327071444,776.782084773983,106.282319498487));
#79880=CARTESIAN_POINT('',(91.3685977607863,776.891105610866,106.313407267717));
#79881=CARTESIAN_POINT('Origin',(90.121757461417,778.398696175795,106.728810633623));
#79882=CARTESIAN_POINT('Ctrl Pts',(94.9634854797312,779.681065915379,107.182982656498));
#79883=CARTESIAN_POINT('Ctrl Pts',(94.9335364154961,779.65678741413,107.175391806428));
#79884=CARTESIAN_POINT('Ctrl Pts',(94.9028729284262,779.632469682793,107.166170964834));
#79885=CARTESIAN_POINT('Ctrl Pts',(94.8724662944701,779.608192893332,107.157664425742));
#79886=CARTESIAN_POINT('Ctrl Pts',(94.8347859453406,779.578108737883,107.147122997074));
#79887=CARTESIAN_POINT('Ctrl Pts',(94.7970943095949,779.548065586691,107.136650203078));
#79888=CARTESIAN_POINT('Ctrl Pts',(94.7593910029568,779.518060476164,107.126243297582));
#79889=CARTESIAN_POINT('Ctrl Pts',(94.6840066344572,779.458067957986,107.105435626615));
#79890=CARTESIAN_POINT('Ctrl Pts',(94.6085756769736,779.398227467302,107.084891325052));
#79891=CARTESIAN_POINT('Ctrl Pts',(94.5330942001178,779.33851587025,107.064588741239));
#79892=CARTESIAN_POINT('Ctrl Pts',(94.3823169310425,779.219239566836,107.024033518026));
#79893=CARTESIAN_POINT('Ctrl Pts',(94.2313389024036,779.100476902626,106.984442149658));
#79894=CARTESIAN_POINT('Ctrl Pts',(94.0801172886116,778.982051890961,106.945648598395));
#79895=CARTESIAN_POINT('Ctrl Pts',(93.7791781886844,778.746379783477,106.868447356408));
#79896=CARTESIAN_POINT('Ctrl Pts',(93.4772813584262,778.512036792077,106.794394137293));
#79897=CARTESIAN_POINT('Ctrl Pts',(93.1739656948357,778.277749460308,106.722309503209));
#79898=CARTESIAN_POINT('Ctrl Pts',(93.0983585117683,778.219348898419,106.704341040714));
#79899=CARTESIAN_POINT('Ctrl Pts',(93.0226642310308,778.16095067228,106.686492238259));
#79900=CARTESIAN_POINT('Ctrl Pts',(92.9468736313629,778.10253749141,106.668748929446));
#79901=CARTESIAN_POINT('Ctrl Pts',(92.6334775012801,777.860997446724,106.595379879182));
#79902=CARTESIAN_POINT('Ctrl Pts',(92.3192632623904,777.61984344963,106.524012845445));
#79903=CARTESIAN_POINT('Ctrl Pts',(92.0047568357767,777.37872161051,106.453859054074));
#79904=CARTESIAN_POINT('Ctrl Pts',(91.7927819712388,777.216207382311,106.40657594898));
#79905=CARTESIAN_POINT('Ctrl Pts',(91.580674607973,777.053707086829,106.359842876413));
#79906=CARTESIAN_POINT('Ctrl Pts',(91.3685977607864,776.891105610866,106.313407267717));
#79907=CARTESIAN_POINT('Origin',(52.8776183915471,825.72084445736,125.575299673618));
#79908=CARTESIAN_POINT('',(109.287160197048,801.327730363652,97.6776808736006));
#79909=CARTESIAN_POINT('Ctrl Pts',(94.9631204076456,779.681651525798,107.182848479366));
#79910=CARTESIAN_POINT('Ctrl Pts',(97.9566175222976,782.913141020044,105.674139401781));
#79911=CARTESIAN_POINT('Ctrl Pts',(100.611942429969,786.348058684875,104.108803322329));
#79912=CARTESIAN_POINT('Ctrl Pts',(105.362756559923,793.572374302806,100.924218762755));
#79913=CARTESIAN_POINT('Ctrl Pts',(107.456885361,797.362462511322,99.3044501680741));
#79914=CARTESIAN_POINT('Ctrl Pts',(109.287160197048,801.327730363652,97.6776808736006));
#79915=CARTESIAN_POINT('',(110.414493061984,803.264712503322,98.3625359087414));
#79916=CARTESIAN_POINT('Ctrl Pts',(109.286997799662,801.327818017083,97.6777118772549));
#79917=CARTESIAN_POINT('Ctrl Pts',(109.602099673755,801.846665738832,97.8613333644607));
#79918=CARTESIAN_POINT('Ctrl Pts',(109.909319285169,802.370215427769,98.0464022479971));
#79919=CARTESIAN_POINT('Ctrl Pts',(110.20842933104,802.89807608039,98.2329603445207));
#79920=CARTESIAN_POINT('Ctrl Pts',(110.277550970416,803.020059926052,98.2760722414585));
#79921=CARTESIAN_POINT('Ctrl Pts',(110.346239709757,803.142273864574,98.3192636277638));
#79922=CARTESIAN_POINT('Ctrl Pts',(110.414493061994,803.264712840779,98.3625349539297));
#79923=CARTESIAN_POINT('',(-4.65925699042498,803.26469939074,98.3625770753546));
#79924=CARTESIAN_POINT('Origin',(52.8776183915471,831.777100559639,108.439826246791));
#79925=CARTESIAN_POINT('',(-3.53191933480331,801.327721522442,97.6776844983083));
#79926=CARTESIAN_POINT('Ctrl Pts',(-4.65925699042498,803.264699682484,98.3625762498996));
#79927=CARTESIAN_POINT('Ctrl Pts',(-4.29564935142747,802.612431997225,98.132044141205));
#79928=CARTESIAN_POINT('Ctrl Pts',(-3.91967758749859,801.966556600686,97.9037821557117));
#79929=CARTESIAN_POINT('Ctrl Pts',(-3.53175694823092,801.327809177577,97.6777154785989));
#79930=CARTESIAN_POINT('Ctrl Pts',(-3.53191933480331,801.327721522442,97.6776844983083));
#79931=CARTESIAN_POINT('Ctrl Pts',(-1.70164478141682,797.362455407221,99.3044531792666));
#79932=CARTESIAN_POINT('Ctrl Pts',(0.39248354271191,793.572368800321,100.924221150267));
#79933=CARTESIAN_POINT('Ctrl Pts',(5.14328675973971,786.348070686369,104.108798069958));
#79934=CARTESIAN_POINT('Ctrl Pts',(7.79859897771313,782.91316749669,105.674127349588));
#79935=CARTESIAN_POINT('Ctrl Pts',(10.7920801946104,779.681690583154,107.182830244375));
#79936=CARTESIAN_POINT('Ctrl Pts',(37.9812496537119,740.125372558701,99.4034193855844));
#79937=CARTESIAN_POINT('Ctrl Pts',(37.2974432564443,740.126812599378,98.8057432472127));
#79938=CARTESIAN_POINT('Ctrl Pts',(37.2974382339422,740.125373764374,97.8975538623548));
#79939=CARTESIAN_POINT('Ctrl Pts',(37.9848781973332,741.131801150289,99.40192578217));
#79940=CARTESIAN_POINT('Ctrl Pts',(37.3009560358114,741.133144619624,98.8042413548037));
#79941=CARTESIAN_POINT('Ctrl Pts',(37.3009513751051,741.131810483968,97.8959593541246));
#79942=CARTESIAN_POINT('Ctrl Pts',(37.9866262292947,742.10800476726,99.4028220357934));
#79943=CARTESIAN_POINT('Ctrl Pts',(37.3013602990247,742.104570379522,98.8049161509109));
#79944=CARTESIAN_POINT('Ctrl Pts',(37.3017025845383,742.109496105312,97.8954725494215));
#79945=CARTESIAN_POINT('Ctrl Pts',(37.932153261221,744.017093575077,99.4504961368679));
#79946=CARTESIAN_POINT('Ctrl Pts',(37.2320445091758,743.994011092838,98.8508878191548));
#79947=CARTESIAN_POINT('Ctrl Pts',(37.2320605227026,744.020040901463,97.9291756497104));
#79948=CARTESIAN_POINT('Ctrl Pts',(37.8766679946406,744.950872239177,99.4961335269924));
#79949=CARTESIAN_POINT('Ctrl Pts',(37.1633838585167,744.915439122629,98.8953866888645));
#79950=CARTESIAN_POINT('Ctrl Pts',(37.1628307039845,744.953765972469,97.9629589076155));
#79951=CARTESIAN_POINT('Ctrl Pts',(37.6873075163571,746.798808429708,99.6375574552887));
#79952=CARTESIAN_POINT('Ctrl Pts',(36.9403996269704,746.729163892062,99.0355904635441));
#79953=CARTESIAN_POINT('Ctrl Pts',(36.9342019053666,746.7964768367,98.076166342412));
#79954=CARTESIAN_POINT('Ctrl Pts',(37.5538636559385,747.712920381025,99.7328632917094));
#79955=CARTESIAN_POINT('Ctrl Pts',(36.7859775201029,747.62350503362,99.1313049156982));
#79956=CARTESIAN_POINT('Ctrl Pts',(36.7753843913839,747.705400843227,98.1553201925244));
#79957=CARTESIAN_POINT('Ctrl Pts',(37.2017809758576,749.533161016737,99.9688263843864));
#79958=CARTESIAN_POINT('Ctrl Pts',(36.3903788991122,749.39639674591,99.3709651407066));
#79959=CARTESIAN_POINT('Ctrl Pts',(36.3652226953077,749.50796954038,98.3603489337074));
#79960=CARTESIAN_POINT('Ctrl Pts',(36.9833127647707,750.439165145003,100.109343103989));
#79961=CARTESIAN_POINT('Ctrl Pts',(36.148555591448,750.275876693628,99.5152612287328));
#79962=CARTESIAN_POINT('Ctrl Pts',(36.1141069873064,750.401487464794,98.4860982992872));
#79963=CARTESIAN_POINT('Ctrl Pts',(36.4594369785795,752.247460839569,100.429869034596));
#79964=CARTESIAN_POINT('Ctrl Pts',(35.5806904318709,752.02583524078,99.8466826136125));
#79965=CARTESIAN_POINT('Ctrl Pts',(35.522610606527,752.177098593973,98.781314739587));
#79966=CARTESIAN_POINT('Ctrl Pts',(36.1573629783603,753.137997262295,100.607797664768));
#79967=CARTESIAN_POINT('Ctrl Pts',(35.2576419586772,752.884926267611,100.031972820423));
#79968=CARTESIAN_POINT('Ctrl Pts',(35.1860607782106,753.047665087694,98.9488503591591));
#79969=CARTESIAN_POINT('Ctrl Pts',(35.4833922952658,754.885078669401,100.989350703394));
#79970=CARTESIAN_POINT('Ctrl Pts',(34.5471212341506,754.568275972171,100.430525778272));
#79971=CARTESIAN_POINT('Ctrl Pts',(34.446248605843,754.749366369677,99.3142469989865));
#79972=CARTESIAN_POINT('Ctrl Pts',(35.1109298655096,755.743586990137,101.193363601259));
#79973=CARTESIAN_POINT('Ctrl Pts',(34.1586862018381,755.393720711171,100.644289501562));
#79974=CARTESIAN_POINT('Ctrl Pts',(34.0423388546041,755.582452785822,99.5124350021307));
#79975=CARTESIAN_POINT('Ctrl Pts',(33.8962272695194,758.278760713144,101.836914643919));
#79976=CARTESIAN_POINT('Ctrl Pts',(32.8995224205562,757.840128068945,101.321091231123));
#79977=CARTESIAN_POINT('Ctrl Pts',(32.7411531447682,758.03610031727,100.143047832541));
#79978=CARTESIAN_POINT('Ctrl Pts',(32.9572524321006,759.915278556649,102.307851274058));
#79979=CARTESIAN_POINT('Ctrl Pts',(31.9441149171027,759.409670588889,101.814372592625));
#79980=CARTESIAN_POINT('Ctrl Pts',(31.7554250151974,759.611504553537,100.61146803336));
#79981=CARTESIAN_POINT('Ctrl Pts',(30.8570361245727,763.093346528461,103.30000026461));
#79982=CARTESIAN_POINT('Ctrl Pts',(29.825466232898,762.462865228477,102.845341032932));
#79983=CARTESIAN_POINT('Ctrl Pts',(29.5870230864445,762.666413683269,101.592593895766));
#79984=CARTESIAN_POINT('Ctrl Pts',(29.7125386287475,764.609757915344,103.813459947128));
#79985=CARTESIAN_POINT('Ctrl Pts',(28.6759889607061,763.920191194033,103.375458895112));
#79986=CARTESIAN_POINT('Ctrl Pts',(28.421165172366,764.121697471862,102.097362675171));
#79987=CARTESIAN_POINT('Ctrl Pts',(27.2672007424541,767.51635281373,104.842469498997));
#79988=CARTESIAN_POINT('Ctrl Pts',(26.225714610018,766.706197784119,104.425707712909));
#79989=CARTESIAN_POINT('Ctrl Pts',(25.9520288338402,766.91296491144,103.085302829331));
#79990=CARTESIAN_POINT('Ctrl Pts',(25.9651032199003,768.907107240029,105.358419148589));
#79991=CARTESIAN_POINT('Ctrl Pts',(24.9148601580403,768.039581315371,104.948653383042));
#79992=CARTESIAN_POINT('Ctrl Pts',(24.6473500139942,768.249130815112,103.568680493393));
#79993=CARTESIAN_POINT('Ctrl Pts',(23.2176003801495,771.582105405033,106.362164464073));
#79994=CARTESIAN_POINT('Ctrl Pts',(22.1528427787513,770.579303463978,105.9503202526));
#79995=CARTESIAN_POINT('Ctrl Pts',(21.9084442478426,770.82737375778,104.47103030333));
#79996=CARTESIAN_POINT('Ctrl Pts',(21.7706855706201,772.865970272614,106.849323966766));
#79997=CARTESIAN_POINT('Ctrl Pts',(20.6827182904449,771.793794132029,106.432116222091));
#79998=CARTESIAN_POINT('Ctrl Pts',(20.4732983628028,772.068583075469,104.888224483132));
#79999=CARTESIAN_POINT('Ctrl Pts',(19.5143472122575,774.730385301656,107.538946728448));
#80000=CARTESIAN_POINT('Ctrl Pts',(18.4132817282156,773.523297302945,107.095600274954));
#80001=CARTESIAN_POINT('Ctrl Pts',(18.2396670183582,773.892291450409,105.45248981662));
#80002=CARTESIAN_POINT('Ctrl Pts',(18.7480232299384,775.341818771779,107.762053723911));
#80003=CARTESIAN_POINT('Ctrl Pts',(17.6323627611125,774.094371854445,107.310495542271));
#80004=CARTESIAN_POINT('Ctrl Pts',(17.4816920982757,774.494237769663,105.630707165859));
#80005=CARTESIAN_POINT('Ctrl Pts',(17.1984668818591,776.548230578555,108.195765565376));
#80006=CARTESIAN_POINT('Ctrl Pts',(16.049679031786,775.22424377604,107.7256534537));
#80007=CARTESIAN_POINT('Ctrl Pts',(15.9460577282015,775.693942761,105.975651051878));
#80008=CARTESIAN_POINT('Ctrl Pts',(16.4159441921319,777.142527752461,108.406078863569));
#80009=CARTESIAN_POINT('Ctrl Pts',(15.2486973592712,775.781848806884,107.925169073805));
#80010=CARTESIAN_POINT('Ctrl Pts',(15.1690942862755,776.291189365633,106.142083265953));
#80011=CARTESIAN_POINT('Ctrl Pts',(15.6333869345031,777.732299565987,108.614524175997));
#80012=CARTESIAN_POINT('Ctrl Pts',(14.451947512053,776.338746499521,108.121995372869));
#80013=CARTESIAN_POINT('Ctrl Pts',(14.386546670293,776.891176447478,106.31342749679));
#80014=CARTESIAN_POINT('',(37.9809447552159,740.125373764374,99.4032758153525));
#80015=CARTESIAN_POINT('Ctrl Pts',(18.0556461947237,775.880814855153,107.955813432072));
#80016=CARTESIAN_POINT('Ctrl Pts',(18.6359399718752,775.428232050397,107.792932399321));
#80017=CARTESIAN_POINT('Ctrl Pts',(19.2109756852516,774.971301297233,107.626641737905));
#80018=CARTESIAN_POINT('Ctrl Pts',(19.7787947443054,774.508909152344,107.456599405267));
#80019=CARTESIAN_POINT('Ctrl Pts',(19.9419616392958,774.376037440226,107.407736516656));
#80020=CARTESIAN_POINT('Ctrl Pts',(20.1045324232678,774.242714570337,107.358563696084));
#80021=CARTESIAN_POINT('Ctrl Pts',(20.2664599983784,774.108913625309,107.309072474554));
#80022=CARTESIAN_POINT('Ctrl Pts',(20.7762113255627,773.687705506431,107.153273094234));
#80023=CARTESIAN_POINT('Ctrl Pts',(21.2795378908958,773.261673546964,106.994279935223));
#80024=CARTESIAN_POINT('Ctrl Pts',(21.776120368853,772.830028841967,106.832474695738));
#80025=CARTESIAN_POINT('Ctrl Pts',(21.901530240627,772.721018738896,106.791611444945));
#80026=CARTESIAN_POINT('Ctrl Pts',(22.026509775505,772.611650510322,106.750568787163));
#80027=CARTESIAN_POINT('Ctrl Pts',(22.1510534016441,772.501911135818,106.70935277429));
#80028=CARTESIAN_POINT('Ctrl Pts',(22.7300047215739,771.991778600838,106.517756738467));
#80029=CARTESIAN_POINT('Ctrl Pts',(23.299430327368,771.473724094565,106.322450258449));
#80030=CARTESIAN_POINT('Ctrl Pts',(23.8584057417782,770.946731145025,106.124160150832));
#80031=CARTESIAN_POINT('Ctrl Pts',(24.1047781349485,770.714455250925,106.0367623743));
#80032=CARTESIAN_POINT('Ctrl Pts',(24.3491198830283,770.480442524666,105.948785039611));
#80033=CARTESIAN_POINT('Ctrl Pts',(24.5913492318159,770.244603979373,105.860290778658));
#80034=CARTESIAN_POINT('Ctrl Pts',(25.0521007996099,769.796008546848,105.691963242467));
#80035=CARTESIAN_POINT('Ctrl Pts',(25.5053803166802,769.34085066765,105.521836468159));
#80036=CARTESIAN_POINT('Ctrl Pts',(25.9509163291252,768.878635306682,105.350453253166));
#80037=CARTESIAN_POINT('Ctrl Pts',(26.5018720881807,768.30705364339,105.138518489941));
#80038=CARTESIAN_POINT('Ctrl Pts',(27.0409759418072,767.724707271522,104.924672333782));
#80039=CARTESIAN_POINT('Ctrl Pts',(27.5676119325008,767.130683387953,104.709978953184));
#80040=CARTESIAN_POINT('Ctrl Pts',(27.8794361966021,766.778958356572,104.582857741198));
#80041=CARTESIAN_POINT('Ctrl Pts',(28.1868887145181,766.423138784951,104.455439922943));
#80042=CARTESIAN_POINT('Ctrl Pts',(28.4898357301289,766.063030294278,104.327950500425));
#80043=CARTESIAN_POINT('Ctrl Pts',(28.8000158409975,765.69432393374,104.197417168939));
#80044=CARTESIAN_POINT('Ctrl Pts',(29.1055538570495,765.321084701143,104.066782989571));
#80045=CARTESIAN_POINT('Ctrl Pts',(29.4061629237366,764.943095807458,103.936306435134));
#80046=CARTESIAN_POINT('Ctrl Pts',(29.7677270420684,764.488461412724,103.779372910514));
#80047=CARTESIAN_POINT('Ctrl Pts',(30.1222178891466,764.026933172879,103.622662560985));
#80048=CARTESIAN_POINT('Ctrl Pts',(30.469238091311,763.557975992853,103.466594024389));
#80049=CARTESIAN_POINT('Ctrl Pts',(30.6453260113138,763.320013782336,103.387400410254));
#80050=CARTESIAN_POINT('Ctrl Pts',(30.8194897665024,763.080138267366,103.308372271751));
#80051=CARTESIAN_POINT('Ctrl Pts',(30.9916735359252,762.838276475935,103.229565859888));
#80052=CARTESIAN_POINT('Ctrl Pts',(31.3035038206331,762.400257076461,103.086844940661));
#80053=CARTESIAN_POINT('Ctrl Pts',(31.6088768919138,761.955597818807,102.944803289155));
#80054=CARTESIAN_POINT('Ctrl Pts',(31.9071207213202,761.504299136386,102.8039146946));
#80055=CARTESIAN_POINT('Ctrl Pts',(32.098100365209,761.215311223952,102.71369705734));
#80056=CARTESIAN_POINT('Ctrl Pts',(32.2856033689663,760.924432957779,102.62420875733));
#80057=CARTESIAN_POINT('Ctrl Pts',(32.4694461051648,760.631695630178,102.535578116741));
#80058=CARTESIAN_POINT('Ctrl Pts',(32.7850951211746,760.129079909168,102.383403627454));
#80059=CARTESIAN_POINT('Ctrl Pts',(33.0901687852529,759.620779524475,102.233712226929));
#80060=CARTESIAN_POINT('Ctrl Pts',(33.384057549731,759.106366696422,102.087002002915));
#80061=CARTESIAN_POINT('Ctrl Pts',(33.6704511511639,758.605073145063,101.944033388593));
#80062=CARTESIAN_POINT('Ctrl Pts',(33.9462231170835,758.097974964884,101.803895702305));
#80063=CARTESIAN_POINT('Ctrl Pts',(34.210766568814,757.584662151294,101.667069515409));
#80064=CARTESIAN_POINT('Ctrl Pts',(34.380532980657,757.255252090504,101.579263558984));
#80065=CARTESIAN_POINT('Ctrl Pts',(34.5456743815257,756.923282422653,101.492821749334));
#80066=CARTESIAN_POINT('Ctrl Pts',(34.7060206085897,756.588641542112,101.40787591758));
#80067=CARTESIAN_POINT('Ctrl Pts',(34.804502824199,756.383110199388,101.355703478783));
#80068=CARTESIAN_POINT('Ctrl Pts',(34.9011674635956,756.17656816369,101.304097107596));
#80069=CARTESIAN_POINT('Ctrl Pts',(34.9959622034492,755.968977218687,101.253097355651));
#80070=CARTESIAN_POINT('Ctrl Pts',(35.2891642151148,755.326894305936,101.095354110744));
#80071=CARTESIAN_POINT('Ctrl Pts',(35.5645845671724,754.674582533358,100.94337441152));
#80072=CARTESIAN_POINT('Ctrl Pts',(35.8203705047122,754.011535722312,100.798569763282));
#80073=CARTESIAN_POINT('Ctrl Pts',(35.8858189728303,753.841880586103,100.761518303398));
#80074=CARTESIAN_POINT('Ctrl Pts',(35.9500034519668,753.671448552098,100.724922033871));
#80075=CARTESIAN_POINT('Ctrl Pts',(36.0128772187498,753.500267400008,100.688820064372));
#80076=CARTESIAN_POINT('Ctrl Pts',(36.1327878772717,753.173796667875,100.619967645342));
#80077=CARTESIAN_POINT('Ctrl Pts',(36.2479329813418,752.844593841339,100.552907119306));
#80078=CARTESIAN_POINT('Ctrl Pts',(36.3580946322322,752.512498828401,100.487847755715));
#80079=CARTESIAN_POINT('Ctrl Pts',(36.3896867780702,752.417260657984,100.469190038751));
#80080=CARTESIAN_POINT('Ctrl Pts',(36.4208687868851,752.321784548089,100.450697037795));
#80081=CARTESIAN_POINT('Ctrl Pts',(36.4516348136901,752.226066545188,100.432374031466));
#80082=CARTESIAN_POINT('Ctrl Pts',(36.5455194837096,751.933976403869,100.376460103615));
#80083=CARTESIAN_POINT('Ctrl Pts',(36.6355420462419,751.639583202857,100.32212010209));
#80084=CARTESIAN_POINT('Ctrl Pts',(36.7213730733827,751.343312580103,100.269604830608));
#80085=CARTESIAN_POINT('Ctrl Pts',(36.7617470615855,751.203950078844,100.244902214062));
#80086=CARTESIAN_POINT('Ctrl Pts',(36.8011148436526,751.064451733841,100.220652624616));
#80087=CARTESIAN_POINT('Ctrl Pts',(36.839467518245,750.924843089873,100.196873854367));
#80088=CARTESIAN_POINT('Ctrl Pts',(36.9440720163877,750.544069329141,100.132018760044));
#80089=CARTESIAN_POINT('Ctrl Pts',(37.041311835785,750.161767483015,100.070543566056));
#80090=CARTESIAN_POINT('Ctrl Pts',(37.1310665907186,749.778084619037,100.012767251748));
#80091=CARTESIAN_POINT('Ctrl Pts',(37.2208213456522,749.394401755058,99.9549909374389));
#80092=CARTESIAN_POINT('Ctrl Pts',(37.3030910876506,749.009337679417,99.9009137567967));
#80093=CARTESIAN_POINT('Ctrl Pts',(37.3778087353439,748.623038694641,99.8508345064501));
#80094=CARTESIAN_POINT('Ctrl Pts',(37.450080637764,748.249384499219,99.8023945085907));
#80095=CARTESIAN_POINT('Ctrl Pts',(37.5152581745136,747.874595933607,99.7577188420942));
#80096=CARTESIAN_POINT('Ctrl Pts',(37.5735213054274,747.498556700093,99.7169961397917));
#80097=CARTESIAN_POINT('Ctrl Pts',(37.6323548151807,747.118836153572,99.6758747742641));
#80098=CARTESIAN_POINT('Ctrl Pts',(37.6841380810966,746.737839878748,99.6387843384986));
#80099=CARTESIAN_POINT('Ctrl Pts',(37.7291029119305,746.355452828044,99.6058939719244));
#80100=CARTESIAN_POINT('Ctrl Pts',(37.7479124219616,746.195494190758,99.592135403983));
#80101=CARTESIAN_POINT('Ctrl Pts',(37.7655293233452,746.035292279684,99.5791114827409));
#80102=CARTESIAN_POINT('Ctrl Pts',(37.7819728263361,745.874839208236,99.5668331851581));
#80103=CARTESIAN_POINT('Ctrl Pts',(37.7913011847699,745.783814579051,99.5598677374143));
#80104=CARTESIAN_POINT('Ctrl Pts',(37.800247750642,745.692709568112,99.5531469001629));
#80105=CARTESIAN_POINT('Ctrl Pts',(37.8088230074611,745.601517934398,99.5466675895096));
#80106=CARTESIAN_POINT('Ctrl Pts',(37.8378956419644,745.292351562745,99.5247008269473));
#80107=CARTESIAN_POINT('Ctrl Pts',(37.8626795852361,744.982343338724,99.5055209995584));
#80108=CARTESIAN_POINT('Ctrl Pts',(37.8835913732746,744.671551091498,99.4890037412289));
#80109=CARTESIAN_POINT('Ctrl Pts',(37.9046205324492,744.359014467413,99.4723937768443));
#80110=CARTESIAN_POINT('Ctrl Pts',(37.9217347366429,744.045684201553,99.4584761186185));
#80111=CARTESIAN_POINT('Ctrl Pts',(37.935389011644,743.73165097331,99.4470976139473));
#80112=CARTESIAN_POINT('Ctrl Pts',(37.9450719184635,743.508954822322,99.439028565941));
#80113=CARTESIAN_POINT('Ctrl Pts',(37.9530155354597,743.28590580784,99.4322358706036));
#80114=CARTESIAN_POINT('Ctrl Pts',(37.9593883250465,743.062549141665,99.4266578585726));
#80115=CARTESIAN_POINT('Ctrl Pts',(37.9611590765629,743.000486970937,99.4251079449706));
#80116=CARTESIAN_POINT('Ctrl Pts',(37.9628054655143,742.938397342271,99.4236565976025));
#80117=CARTESIAN_POINT('Ctrl Pts',(37.9643355819159,742.876282072794,99.4222976730097));
#80118=CARTESIAN_POINT('Ctrl Pts',(37.9711642729064,742.599070495545,99.4162329866146));
#80119=CARTESIAN_POINT('Ctrl Pts',(37.9756774229465,742.321457256423,99.4120103254435));
#80120=CARTESIAN_POINT('Ctrl Pts',(37.9785774429603,742.04357831077,99.4090836139286));
#80121=CARTESIAN_POINT('Ctrl Pts',(37.9813521913033,741.777702854617,99.4062833270727));
#80122=CARTESIAN_POINT('Ctrl Pts',(37.9826505919109,741.51158419174,99.4046691230041));
#80123=CARTESIAN_POINT('Ctrl Pts',(37.9830568749844,741.245367381578,99.4037857245824));
#80124=CARTESIAN_POINT('Ctrl Pts',(37.9834441189532,740.991625936664,99.4029437236892));
#80125=CARTESIAN_POINT('Ctrl Pts',(37.9830211040447,740.737795411156,99.4027654800549));
#80126=CARTESIAN_POINT('Ctrl Pts',(37.9822605484979,740.484024606801,99.4028814909415));
#80127=CARTESIAN_POINT('Ctrl Pts',(37.9819021957661,740.364454824696,99.4029361520616));
#80128=CARTESIAN_POINT('Ctrl Pts',(37.9814683990284,740.244898636289,99.4030565185439));
#80129=CARTESIAN_POINT('Ctrl Pts',(37.9810056935186,740.125373441235,99.4032061173321));
#80130=CARTESIAN_POINT('',(37.2974382384014,740.125373959151,97.8976768136687));
#80131=CARTESIAN_POINT('Ctrl Pts',(37.2974382384014,740.125373959151,97.8976768136687));
#80132=CARTESIAN_POINT('Ctrl Pts',(37.2983318605475,740.381377378649,97.8972387441088));
#80133=CARTESIAN_POINT('Ctrl Pts',(37.2990577839814,740.637542123138,97.8968757675639));
#80134=CARTESIAN_POINT('Ctrl Pts',(37.2990427906181,740.89368310615,97.8968686277991));
#80135=CARTESIAN_POINT('Ctrl Pts',(37.2990273004109,741.158311982312,97.8968612514397));
#80136=CARTESIAN_POINT('Ctrl Pts',(37.2982206538606,741.422915451805,97.8972338428727));
#80137=CARTESIAN_POINT('Ctrl Pts',(37.2959428630901,741.687311531574,97.8983197957206));
#80138=CARTESIAN_POINT('Ctrl Pts',(37.2935027332017,741.970551232522,97.8994831448904));
#80139=CARTESIAN_POINT('Ctrl Pts',(37.289373995854,742.253552746991,97.9014653049404));
#80140=CARTESIAN_POINT('Ctrl Pts',(37.2826709803646,742.536119324456,97.904700903467));
#80141=CARTESIAN_POINT('Ctrl Pts',(37.2787647974619,742.700785023872,97.9065864488107));
#80142=CARTESIAN_POINT('Ctrl Pts',(37.2739834986708,742.865303533007,97.9088981060954));
#80143=CARTESIAN_POINT('Ctrl Pts',(37.2681456938219,743.02964000767,97.9117249392825));
#80144=CARTESIAN_POINT('Ctrl Pts',(37.2677296940343,743.041350563318,97.9119263783568));
#80145=CARTESIAN_POINT('Ctrl Pts',(37.2673083352308,743.05305998757,97.9121304239047));
#80146=CARTESIAN_POINT('Ctrl Pts',(37.2668815517067,743.064768267401,97.912337108483));
#80147=CARTESIAN_POINT('Ctrl Pts',(37.2549444530568,743.392247852373,97.9181180584528));
#80148=CARTESIAN_POINT('Ctrl Pts',(37.2388984624568,743.71892997045,97.9259165344839));
#80149=CARTESIAN_POINT('Ctrl Pts',(37.2182112729509,744.044672112233,97.9360228946803));
#80150=CARTESIAN_POINT('Ctrl Pts',(37.1978608651249,744.365111262726,97.9459647261492));
#80151=CARTESIAN_POINT('Ctrl Pts',(37.1730184144701,744.68464151184,97.9581403117403));
#80152=CARTESIAN_POINT('Ctrl Pts',(37.1432044022258,745.003166375805,97.9728135962615));
#80153=CARTESIAN_POINT('Ctrl Pts',(37.1159189644583,745.294676632188,97.9862424158504));
#80154=CARTESIAN_POINT('Ctrl Pts',(37.084469352093,745.585345608254,98.0017633380483));
#80155=CARTESIAN_POINT('Ctrl Pts',(37.048516313891,745.875121266209,98.019564990037));
#80156=CARTESIAN_POINT('Ctrl Pts',(37.0475376309818,745.883009291759,98.0200495714085));
#80157=CARTESIAN_POINT('Ctrl Pts',(37.0465556556594,745.890896651898,98.0205358219973));
#80158=CARTESIAN_POINT('Ctrl Pts',(37.0455703870231,745.898783342991,98.0210237422502));
#80159=CARTESIAN_POINT('Ctrl Pts',(37.0005242361305,746.259360208962,98.0433312922155));
#80160=CARTESIAN_POINT('Ctrl Pts',(36.9485888662299,746.61854987502,98.0691300902769));
#80161=CARTESIAN_POINT('Ctrl Pts',(36.8896598941157,746.976332159384,98.0984675551207));
#80162=CARTESIAN_POINT('Ctrl Pts',(36.8310145410884,747.332392474381,98.1276638217611));
#80163=CARTESIAN_POINT('Ctrl Pts',(36.7654426559371,747.687059243834,98.1603648150365));
#80164=CARTESIAN_POINT('Ctrl Pts',(36.6928858986749,748.040325201541,98.1965946320511));
#80165=CARTESIAN_POINT('Ctrl Pts',(36.6540288333409,748.229513347716,98.2159971580169));
#80166=CARTESIAN_POINT('Ctrl Pts',(36.6131692518367,748.418299923063,98.2364113721441));
#80167=CARTESIAN_POINT('Ctrl Pts',(36.5703036120726,748.606684822443,98.2578382276742));
#80168=CARTESIAN_POINT('Ctrl Pts',(36.5622919438916,748.641894312199,98.2618429470162));
#80169=CARTESIAN_POINT('Ctrl Pts',(36.5542105589542,748.677089578501,98.2658828432146));
#80170=CARTESIAN_POINT('Ctrl Pts',(36.5460596373825,748.712270459513,98.2699577847131));
#80171=CARTESIAN_POINT('Ctrl Pts',(36.4518792628445,749.118770328411,98.3170419718421));
#80172=CARTESIAN_POINT('Ctrl Pts',(36.3484727645248,749.523118577006,98.3687797969891));
#80173=CARTESIAN_POINT('Ctrl Pts',(36.2359718696286,749.925751497935,98.4250421952344));
#80174=CARTESIAN_POINT('Ctrl Pts',(36.1220206095073,750.333575175681,98.4820299301625));
#80175=CARTESIAN_POINT('Ctrl Pts',(35.9987389341516,750.739638875786,98.5436597116707));
#80176=CARTESIAN_POINT('Ctrl Pts',(35.8662168994976,751.144387313592,98.6098212405897));
#80177=CARTESIAN_POINT('Ctrl Pts',(35.8503959760103,751.192707535077,98.6177198250747));
#80178=CARTESIAN_POINT('Ctrl Pts',(35.8344433014094,751.241009002355,98.6256830246782));
#80179=CARTESIAN_POINT('Ctrl Pts',(35.8183589852451,751.28929246544,98.6337106734054));
#80180=CARTESIAN_POINT('Ctrl Pts',(35.7985042220638,751.348894422736,98.6436201443927));
#80181=CARTESIAN_POINT('Ctrl Pts',(35.7784661312112,751.408416995377,98.6536191168439));
#80182=CARTESIAN_POINT('Ctrl Pts',(35.7582467256096,751.46786022694,98.6637062638557));
#80183=CARTESIAN_POINT('Ctrl Pts',(35.6169690124689,751.883203980482,98.7341875178566));
#80184=CARTESIAN_POINT('Ctrl Pts',(35.4672072907378,752.293604308015,98.8087915984105));
#80185=CARTESIAN_POINT('Ctrl Pts',(35.3097956950983,752.699018411369,98.8869972042913));
#80186=CARTESIAN_POINT('Ctrl Pts',(35.1526148447416,753.103838229457,98.9650881707481));
#80187=CARTESIAN_POINT('Ctrl Pts',(34.9878061137368,753.503686549661,99.0467703748835));
#80188=CARTESIAN_POINT('Ctrl Pts',(34.8161547712006,753.898515570349,99.1315496716264));
#80189=CARTESIAN_POINT('Ctrl Pts',(34.6273932430672,754.332701101294,99.2247797586786));
#80190=CARTESIAN_POINT('Ctrl Pts',(34.4301879091346,754.76132641945,99.3218404923965));
#80191=CARTESIAN_POINT('Ctrl Pts',(34.2251022209785,755.184974100915,99.4222726360482));
#80192=CARTESIAN_POINT('Ctrl Pts',(34.026814638703,755.594578862951,99.5193756914906));
#80193=CARTESIAN_POINT('Ctrl Pts',(33.8211599493022,755.999530207921,99.6196307211958));
#80194=CARTESIAN_POINT('Ctrl Pts',(33.6086106613834,756.400334739729,99.7226425127427));
#80195=CARTESIAN_POINT('Ctrl Pts',(33.5646169352091,756.483293779463,99.7439640264227));
#80196=CARTESIAN_POINT('Ctrl Pts',(33.5203303039215,756.566076272598,99.7654035652552));
#80197=CARTESIAN_POINT('Ctrl Pts',(33.4757529967058,756.648685564578,99.7869579643792));
#80198=CARTESIAN_POINT('Ctrl Pts',(33.2095740132058,757.14196025388,99.9156630927762));
#80199=CARTESIAN_POINT('Ctrl Pts',(32.9332035131286,757.628747618622,100.048378087605));
#80200=CARTESIAN_POINT('Ctrl Pts',(32.6472123512702,758.109614982728,100.184390926258));
#80201=CARTESIAN_POINT('Ctrl Pts',(32.3393089393483,758.627325743886,100.33082488182));
#80202=CARTESIAN_POINT('Ctrl Pts',(32.0202543965417,759.13817469299,100.481081454425));
#80203=CARTESIAN_POINT('Ctrl Pts',(31.6907105830928,759.642842532214,100.634303710862));
#80204=CARTESIAN_POINT('Ctrl Pts',(31.3611667696439,760.147510371438,100.787525967299));
#80205=CARTESIAN_POINT('Ctrl Pts',(31.0211333110752,760.64599686594,100.943714382247));
#80206=CARTESIAN_POINT('Ctrl Pts',(30.6712252726902,761.138957940082,101.102037752359));
#80207=CARTESIAN_POINT('Ctrl Pts',(30.611648803568,761.222891079623,101.128994399066));
#80208=CARTESIAN_POINT('Ctrl Pts',(30.5518367470566,761.306590851968,101.15598902283));
#80209=CARTESIAN_POINT('Ctrl Pts',(30.4917908266565,761.390060526202,101.183017748532));
#80210=CARTESIAN_POINT('Ctrl Pts',(30.1140681869024,761.915131763029,101.353043647931));
#80211=CARTESIAN_POINT('Ctrl Pts',(29.7273147134851,762.430793603965,101.52431280613));
#80212=CARTESIAN_POINT('Ctrl Pts',(29.3320083504767,762.937818247023,101.695852328439));
#80213=CARTESIAN_POINT('Ctrl Pts',(28.9175690820682,763.469382982118,101.875694397228));
#80214=CARTESIAN_POINT('Ctrl Pts',(28.4937289681027,763.991454179029,102.05583405897));
#80215=CARTESIAN_POINT('Ctrl Pts',(28.0609982131296,764.504885059978,102.235171026141));
#80216=CARTESIAN_POINT('Ctrl Pts',(27.7734124900033,764.846102755915,102.354355416884));
#80217=CARTESIAN_POINT('Ctrl Pts',(27.4818991808668,765.183503509633,102.473185705651));
#80218=CARTESIAN_POINT('Ctrl Pts',(27.1865989652666,765.517329651811,102.591342117818));
#80219=CARTESIAN_POINT('Ctrl Pts',(27.1237204576095,765.58841151538,102.61650125579));
#80220=CARTESIAN_POINT('Ctrl Pts',(27.0606665961456,765.659331758786,102.641630381738));
#80221=CARTESIAN_POINT('Ctrl Pts',(26.9974376972065,765.730092673734,102.666726864875));
#80222=CARTESIAN_POINT('Ctrl Pts',(26.3736370873112,766.428202282502,102.914322533149));
#80223=CARTESIAN_POINT('Ctrl Pts',(25.7329957515788,767.110586820099,103.158643462115));
#80224=CARTESIAN_POINT('Ctrl Pts',(25.0762978115619,767.778941189329,103.397017695192));
#80225=CARTESIAN_POINT('Ctrl Pts',(24.4894741349809,768.376181022608,103.610028328136));
#80226=CARTESIAN_POINT('Ctrl Pts',(23.8898288617463,768.962217177825,103.818291018878));
#80227=CARTESIAN_POINT('Ctrl Pts',(23.2779107817818,769.538240064334,104.01992680827));
#80228=CARTESIAN_POINT('Ctrl Pts',(23.2208829292338,769.591922655701,104.038718304129));
#80229=CARTESIAN_POINT('Ctrl Pts',(23.1637468817857,769.645516760381,104.0574491783));
#80230=CARTESIAN_POINT('Ctrl Pts',(23.1065035427576,769.699024062558,104.076118974889));
#80231=CARTESIAN_POINT('Ctrl Pts',(22.521837427674,770.245531429594,104.26680661866));
#80232=CARTESIAN_POINT('Ctrl Pts',(21.9259462054306,770.783010238342,104.451060584945));
#80233=CARTESIAN_POINT('Ctrl Pts',(21.3201444618659,771.312948153102,104.628323437275));
#80234=CARTESIAN_POINT('Ctrl Pts',(20.7202763727252,771.837695477895,104.803850050778));
#80235=CARTESIAN_POINT('Ctrl Pts',(20.1106918453103,772.355050307892,104.972521471847));
#80236=CARTESIAN_POINT('Ctrl Pts',(19.492693694308,772.866451768922,105.133838046219));
#80237=CARTESIAN_POINT('Ctrl Pts',(19.3238196104963,773.006197256917,105.177919389595));
#80238=CARTESIAN_POINT('Ctrl Pts',(19.1543173848269,773.145498103519,105.221451797222));
#80239=CARTESIAN_POINT('Ctrl Pts',(18.9842138166466,773.28438339178,105.264425669065));
#80240=CARTESIAN_POINT('Ctrl Pts',(18.9443923702578,773.316896601937,105.274485903263));
#80241=CARTESIAN_POINT('Ctrl Pts',(18.9045381239163,773.349388165791,105.284516625319));
#80242=CARTESIAN_POINT('Ctrl Pts',(18.8646517458932,773.38185861452,105.294518478373));
#80243=CARTESIAN_POINT('Ctrl Pts',(18.285662894482,773.853198173206,105.439704922939));
#80244=CARTESIAN_POINT('Ctrl Pts',(17.699937037803,774.32007178252,105.578734506063));
#80245=CARTESIAN_POINT('Ctrl Pts',(17.1099015562802,774.783789023184,105.713499937743));
#80246=CARTESIAN_POINT('Ctrl Pts',(16.9780991288093,774.887374417441,105.74360390876));
#80247=CARTESIAN_POINT('Ctrl Pts',(16.8460816480295,774.990802127088,105.773495035281));
#80248=CARTESIAN_POINT('Ctrl Pts',(16.7138761071789,775.094086374212,105.803194238856));
#80249=CARTESIAN_POINT('Ctrl Pts',(16.6899503361007,775.11277814187,105.808569023766));
#80250=CARTESIAN_POINT('Ctrl Pts',(16.6660190814303,775.131464713226,105.813937236859));
#80251=CARTESIAN_POINT('Ctrl Pts',(16.6420825015631,775.150146217236,105.819299208366));
#80252=CARTESIAN_POINT('Ctrl Pts',(16.2574274119396,775.450353499937,105.905464802704));
#80253=CARTESIAN_POINT('Ctrl Pts',(15.8714060853263,775.749252883057,105.98999114635));
#80254=CARTESIAN_POINT('Ctrl Pts',(15.4846980450322,776.047354453647,106.074219552651));
#80255=CARTESIAN_POINT('Ctrl Pts',(15.119102964531,776.329180680002,106.153849370947));
#80256=CARTESIAN_POINT('Ctrl Pts',(14.7528942828154,776.61029400738,106.23321330142));
#80257=CARTESIAN_POINT('Ctrl Pts',(14.386639086236,776.891105591243,106.313407261698));
#80258=CARTESIAN_POINT('Origin',(39.2974260110815,740.1183815439,97.8977997828924));
#80259=CARTESIAN_POINT('Ctrl Pts',(68.457798550648,740.125373335778,97.8975538630338));
#80260=CARTESIAN_POINT('Ctrl Pts',(68.457793528146,740.126812170783,98.8057432478524));
#80261=CARTESIAN_POINT('Ctrl Pts',(67.7739871309274,740.125372130105,99.4034193862205));
#80262=CARTESIAN_POINT('Ctrl Pts',(68.4543137644914,741.123686977417,97.8959722242474));
#80263=CARTESIAN_POINT('Ctrl Pts',(68.4543091225958,741.125015728932,98.8042534866716));
#80264=CARTESIAN_POINT('Ctrl Pts',(67.770387876316,741.123676987505,99.4019378389631));
#80265=CARTESIAN_POINT('Ctrl Pts',(68.4534660468998,742.089834211708,97.895444103238));
#80266=CARTESIAN_POINT('Ctrl Pts',(68.4537977237444,742.085024899139,98.8048439523186));
#80267=CARTESIAN_POINT('Ctrl Pts',(67.7685829871235,742.088371346622,99.4027417427996));
#80268=CARTESIAN_POINT('Ctrl Pts',(68.5212719805811,743.985087877402,97.9282498249378));
#80269=CARTESIAN_POINT('Ctrl Pts',(68.5213036800754,743.959475863193,98.8496547973229));
#80270=CARTESIAN_POINT('Ctrl Pts',(67.8215691081142,743.982153788961,99.4492253539828));
#80271=CARTESIAN_POINT('Ctrl Pts',(68.5888690257085,744.914529948807,97.961220943636));
#80272=CARTESIAN_POINT('Ctrl Pts',(68.5883730543687,744.876767240832,98.8931590717075));
#80273=CARTESIAN_POINT('Ctrl Pts',(67.8756945555098,744.911598667171,99.493863121479));
#80274=CARTESIAN_POINT('Ctrl Pts',(68.8148134713651,746.756613909965,98.0730736941144));
#80275=CARTESIAN_POINT('Ctrl Pts',(68.8087869122143,746.689940361214,99.0318249317338));
#80276=CARTESIAN_POINT('Ctrl Pts',(68.0627239309321,746.758761162693,99.6337887080991));
#80277=CARTESIAN_POINT('Ctrl Pts',(68.9726401474251,747.669153697586,98.1517196268434));
#80278=CARTESIAN_POINT('Ctrl Pts',(68.9622942131984,747.587911596858,99.1270386428823));
#80279=CARTESIAN_POINT('Ctrl Pts',(68.195245132507,747.676396788027,99.7286309912845));
#80280=CARTESIAN_POINT('Ctrl Pts',(69.3842051708727,749.48685510545,98.3574424080094));
#80281=CARTESIAN_POINT('Ctrl Pts',(69.3592786500214,749.37567200458,99.3676317906573));
#80282=CARTESIAN_POINT('Ctrl Pts',(68.548409408609,749.511762264063,99.9655665671925));
#80283=CARTESIAN_POINT('Ctrl Pts',(69.6397214138926,750.396327035182,98.4853933992926));
#80284=CARTESIAN_POINT('Ctrl Pts',(69.6053161375638,750.270768604279,99.5144439610128));
#80285=CARTESIAN_POINT('Ctrl Pts',(68.7707035402597,750.433935418948,100.108551651481));
#80286=CARTESIAN_POINT('Ctrl Pts',(70.5222777867757,753.048462277384,98.9258874811848));
#80287=CARTESIAN_POINT('Ctrl Pts',(70.4561632372631,752.895496196554,100.011085429209));
#80288=CARTESIAN_POINT('Ctrl Pts',(69.5522866245713,753.134812078005,100.586887702835));
#80289=CARTESIAN_POINT('Ctrl Pts',(71.2666661634435,754.737397951853,99.2960490283313));
#80290=CARTESIAN_POINT('Ctrl Pts',(71.170949083334,754.563260077608,100.415280341793));
#80291=CARTESIAN_POINT('Ctrl Pts',(70.2279620290083,754.870567597945,100.972451671599));
#80292=CARTESIAN_POINT('Ctrl Pts',(72.9942145650824,758.002166447748,100.133539302775));
#80293=CARTESIAN_POINT('Ctrl Pts',(72.8364708956345,757.80629690058,101.310996337131));
#80294=CARTESIAN_POINT('Ctrl Pts',(71.8402373204914,758.243588198102,101.82729685542));
#80295=CARTESIAN_POINT('Ctrl Pts',(73.9775035669035,759.577384533899,100.601048495267));
#80296=CARTESIAN_POINT('Ctrl Pts',(73.7894427854517,759.375625735358,101.803417053148));
#80297=CARTESIAN_POINT('Ctrl Pts',(72.776593891794,759.879822520825,102.297356153672));
#80298=CARTESIAN_POINT('Ctrl Pts',(76.1447884375183,762.636049603697,101.582311656938));
#80299=CARTESIAN_POINT('Ctrl Pts',(75.9067736606732,762.432506681983,102.834553788344));
#80300=CARTESIAN_POINT('Ctrl Pts',(74.8752981911426,763.061721698698,103.289564156708));
#80301=CARTESIAN_POINT('Ctrl Pts',(77.3113370175406,764.094348930254,102.087808588578));
#80302=CARTESIAN_POINT('Ctrl Pts',(77.0568033578485,763.892857490299,103.365391981035));
#80303=CARTESIAN_POINT('Ctrl Pts',(76.0203013175091,764.581271199176,103.803653935234));
#80304=CARTESIAN_POINT('Ctrl Pts',(79.782400865438,766.891062887789,103.077422528602));
#80305=CARTESIAN_POINT('Ctrl Pts',(79.5087647074557,766.684405458065,104.417255532439));
#80306=CARTESIAN_POINT('Ctrl Pts',(78.46730944119,767.493556992294,104.834121508641));
#80307=CARTESIAN_POINT('Ctrl Pts',(81.0886284163067,768.230099673479,103.561888384961));
#80308=CARTESIAN_POINT('Ctrl Pts',(80.8210769288954,768.020758453429,104.941255173866));
#80309=CARTESIAN_POINT('Ctrl Pts',(79.7708698338623,768.887323474605,105.35104305306));
#80310=CARTESIAN_POINT('Ctrl Pts',(83.831887455577,770.81423378035,104.4665568788));
#80311=CARTESIAN_POINT('Ctrl Pts',(83.5872932985924,770.566505473212,105.94524619932));
#80312=CARTESIAN_POINT('Ctrl Pts',(82.5226269516004,771.568512635756,106.357013415668));
#80313=CARTESIAN_POINT('Ctrl Pts',(85.2698557482559,772.058456227081,104.884970895144));
#80314=CARTESIAN_POINT('Ctrl Pts',(85.060286287709,771.784116881193,106.428343407822));
#80315=CARTESIAN_POINT('Ctrl Pts',(83.9723523533647,772.855556135977,106.845426196585));
#80316=CARTESIAN_POINT('Ctrl Pts',(87.5086332117794,773.886757355081,105.450835609297));
#80317=CARTESIAN_POINT('Ctrl Pts',(87.3348509098558,773.518063834734,107.093622744994));
#80318=CARTESIAN_POINT('Ctrl Pts',(86.2338780036532,774.724758211298,107.536886595124));
#80319=CARTESIAN_POINT('Ctrl Pts',(88.2686884844878,774.490412833172,105.629591813404));
#80320=CARTESIAN_POINT('Ctrl Pts',(88.1178962276606,774.090775432108,107.309158083682));
#80321=CARTESIAN_POINT('Ctrl Pts',(87.0023075858948,775.337952653219,107.760653532829));
#80322=CARTESIAN_POINT('Ctrl Pts',(89.8066747417754,775.692017030682,105.975112203932));
#80323=CARTESIAN_POINT('Ctrl Pts',(89.7029989420519,775.222460255136,107.72501381451));
#80324=CARTESIAN_POINT('Ctrl Pts',(88.5542478926562,776.546313317911,108.19508593578));
#80325=CARTESIAN_POINT('Ctrl Pts',(90.5848365181571,776.290187893291,106.141797634399));
#80326=CARTESIAN_POINT('Ctrl Pts',(90.5052198785861,775.780926684455,107.92484290776));
#80327=CARTESIAN_POINT('Ctrl Pts',(89.3379859242012,777.141542501245,108.405730641429));
#80328=CARTESIAN_POINT('Ctrl Pts',(91.3685977607865,776.891105610866,106.313407267717));
#80329=CARTESIAN_POINT('Ctrl Pts',(91.30319437909,776.338680147618,108.121971920454));
#80330=CARTESIAN_POINT('Ctrl Pts',(90.121757463342,777.732229909622,108.614499557081));
#80331=CARTESIAN_POINT('',(67.7742920278783,740.125373764374,99.4032758153525));
#80332=CARTESIAN_POINT('Ctrl Pts',(67.7742310895756,740.125373441235,99.4032061173321));
#80333=CARTESIAN_POINT('Ctrl Pts',(67.7732877224663,740.369027246431,99.4029012766841));
#80334=CARTESIAN_POINT('Ctrl Pts',(67.7724586522842,740.612704432908,99.4027119719534));
#80335=CARTESIAN_POINT('Ctrl Pts',(67.7721484590144,740.856295764963,99.4029559530873));
#80336=CARTESIAN_POINT('Ctrl Pts',(67.7718267965963,741.108893691921,99.4032089552288));
#80337=CARTESIAN_POINT('Ctrl Pts',(67.7720634371067,741.361399339847,99.4039281453025));
#80338=CARTESIAN_POINT('Ctrl Pts',(67.773344281289,741.613730131199,99.4054937540533));
#80339=CARTESIAN_POINT('Ctrl Pts',(67.774726999303,741.886130424322,99.4071838858059));
#80340=CARTESIAN_POINT('Ctrl Pts',(67.7773270520541,742.158326800835,99.4098607599035));
#80341=CARTESIAN_POINT('Ctrl Pts',(67.7817898558437,742.430261486565,99.4140279754738));
#80342=CARTESIAN_POINT('Ctrl Pts',(67.7841872781943,742.576345052909,99.4162666075578));
#80343=CARTESIAN_POINT('Ctrl Pts',(67.7871227905514,742.72235387932,99.4189357188471));
#80344=CARTESIAN_POINT('Ctrl Pts',(67.7906992152466,742.868283965283,99.4221154035058));
#80345=CARTESIAN_POINT('Ctrl Pts',(67.7920636549196,742.923957666184,99.4233284831219));
#80346=CARTESIAN_POINT('Ctrl Pts',(67.7935213617819,742.979617114786,99.4246157929733));
#80347=CARTESIAN_POINT('Ctrl Pts',(67.7950781312413,743.035262525335,99.4259817466451));
#80348=CARTESIAN_POINT('Ctrl Pts',(67.8039732671529,743.353211651789,99.4337865911499));
#80349=CARTESIAN_POINT('Ctrl Pts',(67.8160290747519,743.670739140473,99.4440434513336));
#80350=CARTESIAN_POINT('Ctrl Pts',(67.8317599909462,743.987754340686,99.4569482517995));
#80351=CARTESIAN_POINT('Ctrl Pts',(67.8472830920453,744.300581574783,99.4696825719004));
#80352=CARTESIAN_POINT('Ctrl Pts',(67.8663857089031,744.612910887329,99.4849956039512));
#80353=CARTESIAN_POINT('Ctrl Pts',(67.8895371977891,744.924690182995,99.503051025853));
#80354=CARTESIAN_POINT('Ctrl Pts',(67.9060712787972,745.147353362738,99.5159456526232));
#80355=CARTESIAN_POINT('Ctrl Pts',(67.9246699523343,745.369736771215,99.5302385027949));
#80356=CARTESIAN_POINT('Ctrl Pts',(67.9454925408185,745.591828666883,99.5459802086122));
#80357=CARTESIAN_POINT('Ctrl Pts',(67.9531016634615,745.672986899129,99.5517326428144));
#80358=CARTESIAN_POINT('Ctrl Pts',(67.9610071024784,745.754102616515,99.5576783730213));
#80359=CARTESIAN_POINT('Ctrl Pts',(67.9692166012849,745.835179366707,99.563819843913));
#80360=CARTESIAN_POINT('Ctrl Pts',(68.0044365618116,746.183010581337,99.5901676597151));
#80361=CARTESIAN_POINT('Ctrl Pts',(68.0452020240616,746.530112578135,99.6200570912663));
#80362=CARTESIAN_POINT('Ctrl Pts',(68.0917401161303,746.876470855017,99.6533875148075));
#80363=CARTESIAN_POINT('Ctrl Pts',(68.1374417447843,747.216603779416,99.6861188660909));
#80364=CARTESIAN_POINT('Ctrl Pts',(68.1887105364043,747.55601987355,99.7221684631195));
#80365=CARTESIAN_POINT('Ctrl Pts',(68.2457178514693,747.894706722461,99.7614164359059));
#80366=CARTESIAN_POINT('Ctrl Pts',(68.2677433897189,748.025562914106,99.7765804148591));
#80367=CARTESIAN_POINT('Ctrl Pts',(68.2906250723667,748.156310229622,99.7922215858955));
#80368=CARTESIAN_POINT('Ctrl Pts',(68.3143709022457,748.286947818455,99.8083321054578));
#80369=CARTESIAN_POINT('Ctrl Pts',(68.3329980045785,748.38942474801,99.8209697895502));
#80370=CARTESIAN_POINT('Ctrl Pts',(68.352148729185,748.491793122839,99.8338915643058));
#80371=CARTESIAN_POINT('Ctrl Pts',(68.3718306053814,748.594079036638,99.8470962397665));
#80372=CARTESIAN_POINT('Ctrl Pts',(68.4249845802106,748.870318091961,99.8827575242933));
#80373=CARTESIAN_POINT('Ctrl Pts',(68.4821587598131,749.146356983718,99.9205610463555));
#80374=CARTESIAN_POINT('Ctrl Pts',(68.5431875418258,749.421829357746,99.9603143446058));
#80375=CARTESIAN_POINT('Ctrl Pts',(68.5580569543216,749.488947072135,99.9700000727206));
#80376=CARTESIAN_POINT('Ctrl Pts',(68.5731553965728,749.556031213665,99.9798016632362));
#80377=CARTESIAN_POINT('Ctrl Pts',(68.5884808649365,749.623076561152,99.989716548589));
#80378=CARTESIAN_POINT('Ctrl Pts',(68.6560448371755,749.918653171852,100.03342738488));
#80379=CARTESIAN_POINT('Ctrl Pts',(68.727998815401,750.213369552359,100.079327842352));
#80380=CARTESIAN_POINT('Ctrl Pts',(68.8039642538315,750.505968120847,100.127062363807));
#80381=CARTESIAN_POINT('Ctrl Pts',(68.8421391725935,750.653007706384,100.151050397264));
#80382=CARTESIAN_POINT('Ctrl Pts',(68.8813264975892,750.799512856937,100.175501330819));
#80383=CARTESIAN_POINT('Ctrl Pts',(68.921474642866,750.945327316819,100.200368733094));
#80384=CARTESIAN_POINT('Ctrl Pts',(68.9572967666306,751.075430054879,100.222556636317));
#80385=CARTESIAN_POINT('Ctrl Pts',(68.9939077941583,751.205085505603,100.245096046841));
#80386=CARTESIAN_POINT('Ctrl Pts',(69.0312825981136,751.334215880537,100.267961608868));
#80387=CARTESIAN_POINT('Ctrl Pts',(69.2398705795402,752.054889740941,100.395573821447));
#80388=CARTESIAN_POINT('Ctrl Pts',(69.4725174329772,752.762848064153,100.53347495977));
#80389=CARTESIAN_POINT('Ctrl Pts',(69.7271516357318,753.459062406438,100.679829134532));
#80390=CARTESIAN_POINT('Ctrl Pts',(69.9667703347098,754.114221741294,100.81755296176));
#80391=CARTESIAN_POINT('Ctrl Pts',(70.2258594541185,754.758981441764,100.962762134576));
#80392=CARTESIAN_POINT('Ctrl Pts',(70.5027061196983,755.394128388056,101.113965705465));
#80393=CARTESIAN_POINT('Ctrl Pts',(70.5855287331775,755.584141621284,101.159200402015));
#80394=CARTESIAN_POINT('Ctrl Pts',(70.6699407413637,755.773294352767,101.204971877759));
#80395=CARTESIAN_POINT('Ctrl Pts',(70.7558965790219,755.961607205061,101.251240971544));
#80396=CARTESIAN_POINT('Ctrl Pts',(70.8469099664253,756.161000184593,101.300232489423));
#80397=CARTESIAN_POINT('Ctrl Pts',(70.9396654517017,756.359475081021,101.349787412258));
#80398=CARTESIAN_POINT('Ctrl Pts',(71.0341165657173,756.557071161423,101.399864795737));
#80399=CARTESIAN_POINT('Ctrl Pts',(71.2796304629115,757.070697541326,101.530034711754));
#80400=CARTESIAN_POINT('Ctrl Pts',(71.5365755788152,757.578291245017,101.663805397549));
#80401=CARTESIAN_POINT('Ctrl Pts',(71.8043655001815,758.080232588601,101.80070691016));
#80402=CARTESIAN_POINT('Ctrl Pts',(72.0790115985549,758.595025045778,101.941113487481));
#80403=CARTESIAN_POINT('Ctrl Pts',(72.365064950169,759.103871994686,102.084813401217));
#80404=CARTESIAN_POINT('Ctrl Pts',(72.6619410691463,759.607169089028,102.231322895338));
#80405=CARTESIAN_POINT('Ctrl Pts',(72.861480151622,759.945449718549,102.329796191646));
#80406=CARTESIAN_POINT('Ctrl Pts',(73.065909504308,760.281222856161,102.429539216931));
#80407=CARTESIAN_POINT('Ctrl Pts',(73.2750632326797,760.614605117607,102.530410239635));
#80408=CARTESIAN_POINT('Ctrl Pts',(73.4551718214064,760.901690645955,102.617273322038));
#80409=CARTESIAN_POINT('Ctrl Pts',(73.6388660691381,761.187093199647,102.70499474763));
#80410=CARTESIAN_POINT('Ctrl Pts',(73.8259682109547,761.470759519602,102.793449721858));
#80411=CARTESIAN_POINT('Ctrl Pts',(74.1273614208162,761.927702993742,102.93593728695));
#80412=CARTESIAN_POINT('Ctrl Pts',(74.4361683805267,762.377984729352,103.079663214883));
#80413=CARTESIAN_POINT('Ctrl Pts',(74.751624296169,762.821500601673,103.224103473275));
#80414=CARTESIAN_POINT('Ctrl Pts',(75.0805888348608,763.28400894945,103.374729030172));
#80415=CARTESIAN_POINT('Ctrl Pts',(75.4168296426776,763.73930700147,103.526184694805));
#80416=CARTESIAN_POINT('Ctrl Pts',(75.759965128326,764.187892650595,103.678080246159));
#80417=CARTESIAN_POINT('Ctrl Pts',(75.9501426745341,764.436514322159,103.762266010805));
#80418=CARTESIAN_POINT('Ctrl Pts',(76.1424388529362,764.683073556509,103.846587192504));
#80419=CARTESIAN_POINT('Ctrl Pts',(76.3367939550992,764.927651198528,103.930979227673));
#80420=CARTESIAN_POINT('Ctrl Pts',(76.6343722691297,765.30212555784,104.060192401207));
#80421=CARTESIAN_POINT('Ctrl Pts',(76.9368184677876,765.671978786484,104.189577407643));
#80422=CARTESIAN_POINT('Ctrl Pts',(77.2438372520424,766.037390595207,104.318874365421));
#80423=CARTESIAN_POINT('Ctrl Pts',(77.7681161939748,766.661384064896,104.539667605755));
#80424=CARTESIAN_POINT('Ctrl Pts',(78.3060132783773,767.272616928675,104.760302519951));
#80425=CARTESIAN_POINT('Ctrl Pts',(78.8568288139819,767.872053720357,104.979603558284));
#80426=CARTESIAN_POINT('Ctrl Pts',(79.1650161183708,768.207445148229,105.102304882929));
#80427=CARTESIAN_POINT('Ctrl Pts',(79.4772482099342,768.539143253834,105.224589148224));
#80428=CARTESIAN_POINT('Ctrl Pts',(79.7934071938624,768.867313120509,105.346254087456));
#80429=CARTESIAN_POINT('Ctrl Pts',(80.2368843417532,769.327637969384,105.516913859885));
#80430=CARTESIAN_POINT('Ctrl Pts',(80.6880872333938,769.781011256299,105.686350506972));
#80431=CARTESIAN_POINT('Ctrl Pts',(81.1467510511712,770.227915631652,105.854027170534));
#80432=CARTESIAN_POINT('Ctrl Pts',(81.6973635034992,770.764411218467,106.055318084148));
#80433=CARTESIAN_POINT('Ctrl Pts',(82.2589714532759,771.291524419039,106.253970999396));
#80434=CARTESIAN_POINT('Ctrl Pts',(82.8306295792313,771.810281649119,106.44924471571));
#80435=CARTESIAN_POINT('Ctrl Pts',(83.0843259953669,772.040501152946,106.535905325864));
#80436=CARTESIAN_POINT('Ctrl Pts',(83.3400023623642,772.269074524743,106.621900498031));
#80437=CARTESIAN_POINT('Ctrl Pts',(83.5975786343429,772.496089563158,106.707165791572));
#80438=CARTESIAN_POINT('Ctrl Pts',(84.1242886014654,772.960305783469,106.88152222438));
#80439=CARTESIAN_POINT('Ctrl Pts',(84.6589209701514,773.417991363861,107.052821094596));
#80440=CARTESIAN_POINT('Ctrl Pts',(85.2009816334199,773.870020876545,107.220562746921));
#80441=CARTESIAN_POINT('Ctrl Pts',(85.2937827633958,773.947408616335,107.249280224382));
#80442=CARTESIAN_POINT('Ctrl Pts',(85.3868017127355,774.024630507358,107.277893419594));
#80443=CARTESIAN_POINT('Ctrl Pts',(85.4800361202237,774.101690852858,107.306399795611));
#80444=CARTESIAN_POINT('Ctrl Pts',(86.0719655882021,774.590933939642,107.487381950637));
#80445=CARTESIAN_POINT('Ctrl Pts',(86.6726364164098,775.073886492312,107.664146507473));
#80446=CARTESIAN_POINT('Ctrl Pts',(87.2790233367975,775.551280939275,107.836892391151));
#80447=CARTESIAN_POINT('Ctrl Pts',(87.4189205946676,775.66141882617,107.876745947721));
#80448=CARTESIAN_POINT('Ctrl Pts',(87.5591222556294,775.771260752326,107.916385519452));
#80449=CARTESIAN_POINT('Ctrl Pts',(87.6995913966809,775.880815488401,107.955813389664));
#80450=CARTESIAN_POINT('',(68.4577985453727,740.125373764361,97.8976768139577));
#80451=CARTESIAN_POINT('Origin',(66.4578107338363,740.118392461545,97.897799765561));
#80452=CARTESIAN_POINT('Ctrl Pts',(91.3685977607861,776.891105610866,106.313407267717));
#80453=CARTESIAN_POINT('Ctrl Pts',(90.9807645122238,776.59374991394,106.228488649706));
#80454=CARTESIAN_POINT('Ctrl Pts',(90.5929827521625,776.296055513399,106.144500887552));
#80455=CARTESIAN_POINT('Ctrl Pts',(90.2059289296751,775.997535867259,106.060142229145));
#80456=CARTESIAN_POINT('Ctrl Pts',(89.840429621133,775.715640384224,105.980481392523));
#80457=CARTESIAN_POINT('Ctrl Pts',(89.4755797478288,775.433008439386,105.900488671419));
#80458=CARTESIAN_POINT('Ctrl Pts',(89.1119557798394,775.149210594843,105.819030848735));
#80459=CARTESIAN_POINT('Ctrl Pts',(89.0871916323187,775.129882903857,105.813483267401));
#80460=CARTESIAN_POINT('Ctrl Pts',(89.0624331052717,775.110549722594,105.807928988557));
#80461=CARTESIAN_POINT('Ctrl Pts',(89.03768037791,775.091210911155,105.802367647203));
#80462=CARTESIAN_POINT('Ctrl Pts',(88.3981541217163,774.591561822048,105.65868150855));
#80463=CARTESIAN_POINT('Ctrl Pts',(87.762336284931,774.088004973204,105.510337467111));
#80464=CARTESIAN_POINT('Ctrl Pts',(87.1340806565533,773.579504623176,105.355121991748));
#80465=CARTESIAN_POINT('Ctrl Pts',(87.0514946058935,773.512660756172,105.334718460872));
#80466=CARTESIAN_POINT('Ctrl Pts',(86.9690392655668,773.445731408773,105.314196174729));
#80467=CARTESIAN_POINT('Ctrl Pts',(86.886723406743,773.378714186383,105.293550101408));
#80468=CARTESIAN_POINT('Ctrl Pts',(86.8452368118931,773.344937993156,105.283144630441));
#80469=CARTESIAN_POINT('Ctrl Pts',(86.803785640428,773.311139432702,105.272708072074));
#80470=CARTESIAN_POINT('Ctrl Pts',(86.7623708602348,773.277318075086,105.262239751732));
#80471=CARTESIAN_POINT('Ctrl Pts',(86.1451910388785,772.773298511194,105.106236603869));
#80472=CARTESIAN_POINT('Ctrl Pts',(85.535985930652,772.263834583666,104.942883567379));
#80473=CARTESIAN_POINT('Ctrl Pts',(84.9360365702387,771.747549276272,104.772668100744));
#80474=CARTESIAN_POINT('Ctrl Pts',(84.3294429878634,771.225546296015,104.60056755944));
#80475=CARTESIAN_POINT('Ctrl Pts',(83.7323121895133,770.696568606511,104.42145207513));
#80476=CARTESIAN_POINT('Ctrl Pts',(83.145943842104,770.15918257094,104.235869825657));
#80477=CARTESIAN_POINT('Ctrl Pts',(82.9764651492521,770.003861289926,104.18223078256));
#80478=CARTESIAN_POINT('Ctrl Pts',(82.8078853384044,769.847837593609,104.12805177399));
#80479=CARTESIAN_POINT('Ctrl Pts',(82.6402352490262,769.691076967123,104.073346646529));
#80480=CARTESIAN_POINT('Ctrl Pts',(82.5801185630709,769.634865071338,104.053730247994));
#80481=CARTESIAN_POINT('Ctrl Pts',(82.5201210385646,769.578558067279,104.034046834186));
#80482=CARTESIAN_POINT('Ctrl Pts',(82.4602437160975,769.522154014666,104.01429694718));
#80483=CARTESIAN_POINT('Ctrl Pts',(81.775386691458,768.877023102676,103.788404267034));
#80484=CARTESIAN_POINT('Ctrl Pts',(81.1060195434944,768.219416764147,103.554258150673));
#80485=CARTESIAN_POINT('Ctrl Pts',(80.4528992274308,767.547678951716,103.314503189542));
#80486=CARTESIAN_POINT('Ctrl Pts',(79.8714268663558,766.949631452334,103.101049588575));
#80487=CARTESIAN_POINT('Ctrl Pts',(79.3028325727198,766.340382487871,102.883150733177));
#80488=CARTESIAN_POINT('Ctrl Pts',(78.7476614911316,765.718744550908,102.662699893706));
#80489=CARTESIAN_POINT('Ctrl Pts',(78.6805303972213,765.643576307985,102.636043054944));
#80490=CARTESIAN_POINT('Ctrl Pts',(78.6135988172079,765.56823053418,102.609350414184));
#80491=CARTESIAN_POINT('Ctrl Pts',(78.5468669476994,765.492704343741,102.582625076989));
#80492=CARTESIAN_POINT('Ctrl Pts',(78.1183922109045,765.007762668828,102.411025930964));
#80493=CARTESIAN_POINT('Ctrl Pts',(77.6979420020796,764.515310703848,102.238036237578));
#80494=CARTESIAN_POINT('Ctrl Pts',(77.2859484879984,764.01461866131,102.064638291515));
#80495=CARTESIAN_POINT('Ctrl Pts',(76.8937139601728,763.537939538511,101.899556417225));
#80496=CARTESIAN_POINT('Ctrl Pts',(76.5091443987673,763.053791770041,101.734104044716));
#80497=CARTESIAN_POINT('Ctrl Pts',(76.1326468908731,762.561516463863,101.569139898605));
#80498=CARTESIAN_POINT('Ctrl Pts',(75.8347136960172,762.171965001654,101.438599074146));
#80499=CARTESIAN_POINT('Ctrl Pts',(75.5418358252766,761.777323557447,101.308364096761));
#80500=CARTESIAN_POINT('Ctrl Pts',(75.254231642613,761.377251511711,101.178868608371));
#80501=CARTESIAN_POINT('Ctrl Pts',(75.1895924136379,761.287335056633,101.149764412292));
#80502=CARTESIAN_POINT('Ctrl Pts',(75.1252294081678,761.197157836843,101.120702138367));
#80503=CARTESIAN_POINT('Ctrl Pts',(75.0611448173126,761.106715923497,101.091686671466));
#80504=CARTESIAN_POINT('Ctrl Pts',(74.7252379190504,760.632654028437,100.939598699018));
#80505=CARTESIAN_POINT('Ctrl Pts',(74.3986534810529,760.153737745643,100.789588600975));
#80506=CARTESIAN_POINT('Ctrl Pts',(74.0818958041657,759.669396971228,100.642377223156));
#80507=CARTESIAN_POINT('Ctrl Pts',(73.7599137942162,759.17706788996,100.492737865451));
#80508=CARTESIAN_POINT('Ctrl Pts',(73.4480848800937,758.679134181147,100.34598977661));
#80509=CARTESIAN_POINT('Ctrl Pts',(73.1469854009512,758.174974131377,100.202914164611));
#80510=CARTESIAN_POINT('Ctrl Pts',(72.8687762443246,757.709141567831,100.070715512321));
#80511=CARTESIAN_POINT('Ctrl Pts',(72.5997274327346,757.23799325803,99.9416521346038));
#80512=CARTESIAN_POINT('Ctrl Pts',(72.3403334658204,756.761018795067,99.8163640668633));
#80513=CARTESIAN_POINT('Ctrl Pts',(72.3189912079547,756.721774582471,99.8060556919961));
#80514=CARTESIAN_POINT('Ctrl Pts',(72.2977143320303,756.682490917786,99.7957728888851));
#80515=CARTESIAN_POINT('Ctrl Pts',(72.2765031258968,756.643167510428,99.7855160220318));
#80516=CARTESIAN_POINT('Ctrl Pts',(72.227461953983,756.552250192083,99.7618017283947));
#80517=CARTESIAN_POINT('Ctrl Pts',(72.1787729826753,756.461122589529,99.7382267680948));
#80518=CARTESIAN_POINT('Ctrl Pts',(72.1304401703867,756.36978191241,99.7147958362881));
#80519=CARTESIAN_POINT('Ctrl Pts',(71.8690884406554,755.875872230153,99.5880969278873));
#80520=CARTESIAN_POINT('Ctrl Pts',(71.6181356407634,755.375790462634,99.4655907782217));
#80521=CARTESIAN_POINT('Ctrl Pts',(71.3787125423155,754.86877041419,99.3480968719145));
#80522=CARTESIAN_POINT('Ctrl Pts',(71.1430487323805,754.369711312941,99.2324477896664));
#80523=CARTESIAN_POINT('Ctrl Pts',(70.918555297956,753.86393017412,99.1216546996797));
#80524=CARTESIAN_POINT('Ctrl Pts',(70.7063483157787,753.350674498194,99.0165239863566));
#80525=CARTESIAN_POINT('Ctrl Pts',(70.4985310074892,752.84803593305,98.9135679872786));
#80526=CARTESIAN_POINT('Ctrl Pts',(70.3024970383778,752.338228909847,98.8160424711298));
#80527=CARTESIAN_POINT('Ctrl Pts',(70.1193322626677,751.82052474662,98.724729886038));
#80528=CARTESIAN_POINT('Ctrl Pts',(70.0806268960185,751.711126368161,98.7054342159401));
#80529=CARTESIAN_POINT('Ctrl Pts',(70.0424963259886,751.601375271595,98.6864160694099));
#80530=CARTESIAN_POINT('Ctrl Pts',(70.0049510239408,751.49126444936,98.6676829807012));
#80531=CARTESIAN_POINT('Ctrl Pts',(69.9810239029901,751.421092288852,98.6557446327624));
#80532=CARTESIAN_POINT('Ctrl Pts',(69.9573427321779,751.350798301254,98.6439264166418));
#80533=CARTESIAN_POINT('Ctrl Pts',(69.9339067018654,751.280371607074,98.6322285107702));
#80534=CARTESIAN_POINT('Ctrl Pts',(69.8522878701283,751.03510206162,98.5914891279363));
#80535=CARTESIAN_POINT('Ctrl Pts',(69.7736131636686,750.787790163411,98.5521884983569));
#80536=CARTESIAN_POINT('Ctrl Pts',(69.6980134816527,750.538580321834,98.514405391234));
#80537=CARTESIAN_POINT('Ctrl Pts',(69.6558192522898,750.399489561998,98.4933176161869));
#80538=CARTESIAN_POINT('Ctrl Pts',(69.6145836640669,750.259807269986,98.4727029314975));
#80539=CARTESIAN_POINT('Ctrl Pts',(69.5743357876118,750.119557537408,98.452578198471));
#80540=CARTESIAN_POINT('Ctrl Pts',(69.4412691722878,749.655867055873,98.386042263063));
#80541=CARTESIAN_POINT('Ctrl Pts',(69.3196158156649,749.18811805896,98.3251703911877));
#80542=CARTESIAN_POINT('Ctrl Pts',(69.2109107377535,748.719717791463,98.2708381534396));
#80543=CARTESIAN_POINT('Ctrl Pts',(69.1999501987674,748.672489828504,98.265359930881));
#80544=CARTESIAN_POINT('Ctrl Pts',(69.1891200775681,748.625249855634,98.2599472155666));
#80545=CARTESIAN_POINT('Ctrl Pts',(69.1784222872972,748.578002387959,98.2546010785117));
#80546=CARTESIAN_POINT('Ctrl Pts',(69.1033489490578,748.246436239071,98.2170837646336));
#80547=CARTESIAN_POINT('Ctrl Pts',(69.0345597878175,747.913927214286,98.1827308961769));
#80548=CARTESIAN_POINT('Ctrl Pts',(68.9719999552296,747.580534775366,98.1515240467797));
#80549=CARTESIAN_POINT('Ctrl Pts',(68.9085608240518,747.242456398371,98.1198785750663));
#80550=CARTESIAN_POINT('Ctrl Pts',(68.8515272981591,746.903469292199,98.0914681468127));
#80551=CARTESIAN_POINT('Ctrl Pts',(68.8007944554575,746.563639967713,98.0662489751074));
#80552=CARTESIAN_POINT('Ctrl Pts',(68.7672748745265,746.33911210887,98.0495864736197));
#80553=CARTESIAN_POINT('Ctrl Pts',(68.7365047781278,746.1142166938,98.0343165602586));
#80554=CARTESIAN_POINT('Ctrl Pts',(68.7084429883808,745.888974959709,98.0204209926115));
#80555=CARTESIAN_POINT('Ctrl Pts',(68.7062255233766,745.871176178258,98.0193229537747));
#80556=CARTESIAN_POINT('Ctrl Pts',(68.7040249428091,745.85337505384,98.0182334644857));
#80557=CARTESIAN_POINT('Ctrl Pts',(68.7018412289294,745.83557162853,98.0171525161574));
#80558=CARTESIAN_POINT('Ctrl Pts',(68.6632110913049,745.520627085521,97.9980304218781));
#80559=CARTESIAN_POINT('Ctrl Pts',(68.6299239732758,745.204972885799,97.9816106203079));
#80560=CARTESIAN_POINT('Ctrl Pts',(68.6015127569383,744.888652305022,97.967637146246));
#80561=CARTESIAN_POINT('Ctrl Pts',(68.5720603542791,744.560739518615,97.9531515860457));
#80562=CARTESIAN_POINT('Ctrl Pts',(68.5478470658136,744.232109684,97.9412945386335));
#80563=CARTESIAN_POINT('Ctrl Pts',(68.5283084725441,743.902839265685,97.9317593780112));
#80564=CARTESIAN_POINT('Ctrl Pts',(68.5112191275066,743.614844336287,97.9234194915304));
#80565=CARTESIAN_POINT('Ctrl Pts',(68.497704854417,743.32635947197,97.9168553037103));
#80566=CARTESIAN_POINT('Ctrl Pts',(68.4873690146543,743.037460938716,97.9118529049428));
#80567=CARTESIAN_POINT('Ctrl Pts',(68.4871628646808,743.031698811367,97.911753131301));
#80568=CARTESIAN_POINT('Ctrl Pts',(68.4869580177625,743.025936507947,97.9116539921842));
#80569=CARTESIAN_POINT('Ctrl Pts',(68.4867544660922,743.020174028313,97.9115554837351));
#80570=CARTESIAN_POINT('Ctrl Pts',(68.4769948303666,742.743882008606,97.9068323263289));
#80571=CARTESIAN_POINT('Ctrl Pts',(68.4702128160218,742.467233873008,97.9035600998517));
#80572=CARTESIAN_POINT('Ctrl Pts',(68.4655567364647,742.190285780326,97.9013210273558));
#80573=CARTESIAN_POINT('Ctrl Pts',(68.4611688045257,741.929287366015,97.8992109049669));
#80574=CARTESIAN_POINT('Ctrl Pts',(68.4586682871477,741.668022513426,97.898018015762));
#80575=CARTESIAN_POINT('Ctrl Pts',(68.4573689622943,741.406570728667,97.8974060106253));
#80576=CARTESIAN_POINT('Ctrl Pts',(68.4561510499872,741.161500879099,97.8968323522473));
#80577=CARTESIAN_POINT('Ctrl Pts',(68.4559881997955,740.916266870814,97.896768909083));
#80578=CARTESIAN_POINT('Ctrl Pts',(68.4563461801979,740.670963156096,97.8969540896854));
#80579=CARTESIAN_POINT('Ctrl Pts',(68.4566115484957,740.489121276497,97.8970913627342));
#80580=CARTESIAN_POINT('Ctrl Pts',(68.4571637055702,740.307241660318,97.8973655500502));
#80581=CARTESIAN_POINT('Ctrl Pts',(68.4577985453727,740.125373764361,97.8976768139577));
#80582=CARTESIAN_POINT('Ctrl Pts',(37.2974370684329,740.1250398719,82.4370095290715));
#80583=CARTESIAN_POINT('Ctrl Pts',(37.3424884707948,753.031264614585,82.4563563944262));
#80584=CARTESIAN_POINT('Ctrl Pts',(37.3879041226833,765.937472681678,82.4756378033222));
#80585=CARTESIAN_POINT('Ctrl Pts',(13.9672995497186,779.915230707551,88.5489395495829));
#80586=CARTESIAN_POINT('Ctrl Pts',(2.77065801251735,790.645214141688,92.3412787532726));
#80587=CARTESIAN_POINT('Ctrl Pts',(-4.44817956388518,803.379710979161,96.8420808181083));
#80588=CARTESIAN_POINT('Ctrl Pts',(37.2974370944911,740.125047336989,83.2541797519407));
#80589=CARTESIAN_POINT('Ctrl Pts',(37.3414812482621,752.742717755302,83.2719940286304));
#80590=CARTESIAN_POINT('Ctrl Pts',(37.3858793646116,765.36036823179,83.2897413519787));
#80591=CARTESIAN_POINT('Ctrl Pts',(14.6269734057586,779.259941132568,89.4579435538414));
#80592=CARTESIAN_POINT('Ctrl Pts',(3.52773834636104,789.585631506022,93.0954993990444));
#80593=CARTESIAN_POINT('Ctrl Pts',(-3.81134624434443,801.905170120104,97.4384971415098));
#80594=CARTESIAN_POINT('Ctrl Pts',(37.297437120366,740.125054749569,84.07134997481));
#80595=CARTESIAN_POINT('Ctrl Pts',(37.3404811104892,752.456200521121,84.0876316628422));
#80596=CARTESIAN_POINT('Ctrl Pts',(37.3838684935262,764.787322986573,84.1038448845999));
#80597=CARTESIAN_POINT('Ctrl Pts',(15.3048815505885,778.617102553909,90.3217738647409));
#80598=CARTESIAN_POINT('Ctrl Pts',(4.3028141604402,788.543880887858,93.8278683544787));
#80599=CARTESIAN_POINT('Ctrl Pts',(-3.14516449837338,800.450285635656,98.0345313843018));
#80600=CARTESIAN_POINT('Ctrl Pts',(37.2974371460461,740.125062106342,84.8885201976793));
#80601=CARTESIAN_POINT('Ctrl Pts',(37.3394885023999,752.171840373793,84.9032692970658));
#80602=CARTESIAN_POINT('Ctrl Pts',(37.3818727361078,764.21859183176,84.9179478797552));
#80603=CARTESIAN_POINT('Ctrl Pts',(15.9793268060979,777.989735996571,91.1817234896819));
#80604=CARTESIAN_POINT('Ctrl Pts',(5.08782990810792,787.523121454333,94.5593122958652));
#80605=CARTESIAN_POINT('Ctrl Pts',(-2.44951120227387,799.014953473008,98.6297577392777));
#80606=CARTESIAN_POINT('Ctrl Pts',(37.2974371715198,740.125069404011,85.7056904205486));
#80607=CARTESIAN_POINT('Ctrl Pts',(37.3385038689179,751.88976477507,85.7189069313054));
#80608=CARTESIAN_POINT('Ctrl Pts',(37.37989331662,763.654429651608,85.7320498163745));
#80609=CARTESIAN_POINT('Ctrl Pts',(16.6287677270449,777.38095747515,92.07906222547));
#80610=CARTESIAN_POINT('Ctrl Pts',(5.87488577558581,786.526607362185,95.3107346888993));
#80611=CARTESIAN_POINT('Ctrl Pts',(-1.72410749947928,797.599164568951,99.2237271886367));
#80612=CARTESIAN_POINT('Ctrl Pts',(37.2974372094038,740.125080256911,86.9314457548525));
#80613=CARTESIAN_POINT('Ctrl Pts',(37.3370395479918,751.470269392525,86.9423633826947));
#80614=CARTESIAN_POINT('Ctrl Pts',(37.376950526235,762.815422167125,86.9532003527393));
#80615=CARTESIAN_POINT('Ctrl Pts',(17.5333967744215,776.500515238856,93.5430042314188));
#80616=CARTESIAN_POINT('Ctrl Pts',(7.04696637151271,785.073254941205,96.4991366952518));
#80617=CARTESIAN_POINT('Ctrl Pts',(-0.590671714732331,795.504951976006,
100.112068018336));
#80618=CARTESIAN_POINT('Ctrl Pts',(37.2974372219773,740.125083858944,87.3400308662872));
#80619=CARTESIAN_POINT('Ctrl Pts',(37.3365535459,751.331040600932,87.3501821998278));
#80620=CARTESIAN_POINT('Ctrl Pts',(37.3759739088114,762.536959012098,87.3602503005129));
#80621=CARTESIAN_POINT('Ctrl Pts',(17.8283182521832,776.209771644634,94.040091612404));
#80622=CARTESIAN_POINT('Ctrl Pts',(7.43772026798971,784.59385178339,96.9000225008642));
#80623=CARTESIAN_POINT('Ctrl Pts',(-0.205304748057507,794.811792905548,
100.407746070846));
#80624=CARTESIAN_POINT('Ctrl Pts',(37.2974372344949,740.125087444965,87.7486159777218));
#80625=CARTESIAN_POINT('Ctrl Pts',(37.3360697043082,751.192430744648,87.7580010169631));
#80626=CARTESIAN_POINT('Ctrl Pts',(37.37500167387,762.259733741229,87.7673000996059));
#80627=CARTESIAN_POINT('Ctrl Pts',(18.1192890407701,775.921049293556,94.5419441749148));
#80628=CARTESIAN_POINT('Ctrl Pts',(7.82954922493632,784.118890694556,97.3033652604152));
#80629=CARTESIAN_POINT('Ctrl Pts',(0.187675975419192,794.123558618551,100.702927900473));
#80630=CARTESIAN_POINT('Ctrl Pts',(37.2974372469552,740.12509101456,88.1572010891565));
#80631=CARTESIAN_POINT('Ctrl Pts',(37.3355880788326,751.05445575639,88.1658198340999));
#80632=CARTESIAN_POINT('Ctrl Pts',(37.3740338910031,761.9837782321,88.1743498323877));
#80633=CARTESIAN_POINT('Ctrl Pts',(18.4089919196902,775.633639338812,95.0442181190076));
#80634=CARTESIAN_POINT('Ctrl Pts',(8.22347986897346,783.647773155753,97.7068678552149));
#80635=CARTESIAN_POINT('Ctrl Pts',(0.588341104726402,793.440269165873,100.99755057259));
#80636=CARTESIAN_POINT('Ctrl Pts',(37.2974372717582,740.125098120077,88.9743713120258));
#80637=CARTESIAN_POINT('Ctrl Pts',(37.3346293713467,750.779807381366,88.9814574683739));
#80638=CARTESIAN_POINT('Ctrl Pts',(37.3721073681987,761.434470492247,88.9884493301505));
#80639=CARTESIAN_POINT('Ctrl Pts',(18.9912534758669,775.060041775275,96.0409158137305));
#80640=CARTESIAN_POINT('Ctrl Pts',(9.01762384312406,782.712043387227,98.5095931211922));
#80641=CARTESIAN_POINT('Ctrl Pts',(1.40520753171264,792.083635277775,101.585546375814));
#80642=CARTESIAN_POINT('Ctrl Pts',(37.297437284101,740.125101655998,89.3829564234604));
#80643=CARTESIAN_POINT('Ctrl Pts',(37.3341522893364,750.6431339946,89.3892762855112));
#80644=CARTESIAN_POINT('Ctrl Pts',(37.3711486282413,761.161118261416,89.3954990950289));
#80645=CARTESIAN_POINT('Ctrl Pts',(19.2838134375432,774.773861036257,96.5353461798798));
#80646=CARTESIAN_POINT('Ctrl Pts',(9.41783717323752,782.247431157503,98.9088157923697));
#80647=CARTESIAN_POINT('Ctrl Pts',(1.82140882939167,791.410290842356,101.87891950692));
#80648=CARTESIAN_POINT('Ctrl Pts',(37.2974372963835,740.125105174671,89.7915415348951));
#80649=CARTESIAN_POINT('Ctrl Pts',(37.333677534675,750.507127341298,89.7970951026478));
#80650=CARTESIAN_POINT('Ctrl Pts',(37.3701944834603,760.889099547344,89.8025489584973));
#80651=CARTESIAN_POINT('Ctrl Pts',(19.5802186903287,774.487584241543,97.0214998392773));
#80652=CARTESIAN_POINT('Ctrl Pts',(9.8222315023368,781.785480686826,99.3035987046764));
#80653=CARTESIAN_POINT('Ctrl Pts',(2.24546188961201,790.741946589879,102.171602254524));
#80654=CARTESIAN_POINT('Ctrl Pts',(37.2974373086044,740.125108675681,90.2001266463297));
#80655=CARTESIAN_POINT('Ctrl Pts',(37.3332051629788,750.37180335418,90.2049139197827));
#80656=CARTESIAN_POINT('Ctrl Pts',(37.3692450073853,760.618446227576,90.2095990031906));
#80657=CARTESIAN_POINT('Ctrl Pts',(19.8828983710714,774.200504916139,97.4950158880135));
#80658=CARTESIAN_POINT('Ctrl Pts',(10.2318595156963,781.325608703157,99.6916393826827));
#80659=CARTESIAN_POINT('Ctrl Pts',(2.67746342005582,790.078637818108,102.463526327259));
#80660=CARTESIAN_POINT('Ctrl Pts',(37.2974373450777,740.125119124492,91.4258819806337));
#80661=CARTESIAN_POINT('Ctrl Pts',(37.3317953636346,749.967927189533,91.4283703711791));
#80662=CARTESIAN_POINT('Ctrl Pts',(37.3664108052091,759.810678083431,91.4307499289936));
#80663=CARTESIAN_POINT('Ctrl Pts',(20.8170904917175,773.334764479849,98.8645592276937));
#80664=CARTESIAN_POINT('Ctrl Pts',(11.4796450483815,779.950502954021,100.828618024696));
#80665=CARTESIAN_POINT('Ctrl Pts',(3.99764592910691,788.103948395176,103.336808383945));
#80666=CARTESIAN_POINT('Ctrl Pts',(37.297437369141,740.125126018071,92.243052203503));
#80667=CARTESIAN_POINT('Ctrl Pts',(37.3308652517341,749.701470808714,92.244008005429));
#80668=CARTESIAN_POINT('Ctrl Pts',(37.3645400286259,759.277754923748,92.2448519400639));
#80669=CARTESIAN_POINT('Ctrl Pts',(21.4925708184156,772.761294515867,99.6877915698248));
#80670=CARTESIAN_POINT('Ctrl Pts',(12.345371211636,779.043417932929,101.539440317288));
#80671=CARTESIAN_POINT('Ctrl Pts',(4.91000482543385,786.807804636397,103.915676206375));
#80672=CARTESIAN_POINT('Ctrl Pts',(37.2974373929403,740.125132836058,93.0602224263723));
#80673=CARTESIAN_POINT('Ctrl Pts',(37.329945339088,749.437936285258,93.0596456396654));
#80674=CARTESIAN_POINT('Ctrl Pts',(37.3626890028486,758.750675605608,93.0589551285022));
#80675=CARTESIAN_POINT('Ctrl Pts',(22.2098244807151,772.193286281927,100.442875982628));
#80676=CARTESIAN_POINT('Ctrl Pts',(13.2416248126661,778.147949114238,102.213865617469));
#80677=CARTESIAN_POINT('Ctrl Pts',(5.85548763085168,785.532324601494,104.490652781672));
#80678=CARTESIAN_POINT('Ctrl Pts',(37.2974374164643,740.125139575155,93.8773926492416));
#80679=CARTESIAN_POINT('Ctrl Pts',(37.3290360706217,749.177451080918,93.8752832738895));
#80680=CARTESIAN_POINT('Ctrl Pts',(37.3608587836402,758.229695032105,93.8730592785752));
#80681=CARTESIAN_POINT('Ctrl Pts',(22.9581652826313,771.632642151683,101.151411686076));
#80682=CARTESIAN_POINT('Ctrl Pts',(14.1652901957973,777.266191525838,102.862610999887));
#80683=CARTESIAN_POINT('Ctrl Pts',(6.83520707883987,784.277987128319,105.061117676372));
#80684=CARTESIAN_POINT('Ctrl Pts',(37.2974374629385,740.125152888974,95.5117330949803));
#80685=CARTESIAN_POINT('Ctrl Pts',(37.3272397119003,748.662834233973,95.5065585423147));
#80686=CARTESIAN_POINT('Ctrl Pts',(37.3572420617776,757.200441175945,95.501269072464));
#80687=CARTESIAN_POINT('Ctrl Pts',(24.4961711849034,770.530184767746,102.51845911973));
#80688=CARTESIAN_POINT('Ctrl Pts',(16.0617356260895,775.534586787255,104.13005108402));
#80689=CARTESIAN_POINT('Ctrl Pts',(8.86586713809172,781.812852902991,106.191658243183));
#80690=CARTESIAN_POINT('Ctrl Pts',(37.2974374858887,740.125159463696,96.3289033178496));
#80691=CARTESIAN_POINT('Ctrl Pts',(37.3263526216414,748.408702591369,96.3221961765227));
#80692=CARTESIAN_POINT('Ctrl Pts',(37.3554559164072,756.692167907054,96.3153740553816));
#80693=CARTESIAN_POINT('Ctrl Pts',(25.2628191432126,769.98748460851,103.21954759762));
#80694=CARTESIAN_POINT('Ctrl Pts',(17.0243325801041,774.68595208428,104.770644970324));
#80695=CARTESIAN_POINT('Ctrl Pts',(9.91680774935538,780.602056150836,106.751733915294));
#80696=CARTESIAN_POINT('Ctrl Pts',(37.2974375085405,740.125165952933,97.146073540719));
#80697=CARTESIAN_POINT('Ctrl Pts',(37.3254770654129,748.157875191384,97.1378338107217));
#80698=CARTESIAN_POINT('Ctrl Pts',(37.353692747676,756.190503271047,97.1294794255097));
#80699=CARTESIAN_POINT('Ctrl Pts',(26.0354102597506,769.450667095891,103.92649548435));
#80700=CARTESIAN_POINT('Ctrl Pts',(18.0055779592141,773.852731336532,105.411629333519));
#80701=CARTESIAN_POINT('Ctrl Pts',(11.0047328813242,779.413657557974,107.305932045411));
#80702=CARTESIAN_POINT('Ctrl Pts',(37.2974375308824,740.125172353387,97.9632437635883));
#80703=CARTESIAN_POINT('Ctrl Pts',(37.3246134881434,747.91047949577,97.9534714449075));
#80704=CARTESIAN_POINT('Ctrl Pts',(37.3519533126077,755.695702239311,97.9435854850557));
#80705=CARTESIAN_POINT('Ctrl Pts',(26.8225038911607,768.9172353047,104.627534930461));
#80706=CARTESIAN_POINT('Ctrl Pts',(19.0100071552343,773.033319793847,106.046458309024));
#80707=CARTESIAN_POINT('Ctrl Pts',(12.1312776786533,778.248433884114,107.853507205599));
#80708=CARTESIAN_POINT('Ctrl Pts',(37.2974375529029,740.125178661761,98.7804139864576));
#80709=CARTESIAN_POINT('Ctrl Pts',(37.3237623347616,747.666642966279,98.7691090790754));
#80710=CARTESIAN_POINT('Ctrl Pts',(37.3502383636256,755.208019780636,98.7576925374003));
#80711=CARTESIAN_POINT('Ctrl Pts',(27.6329557572476,768.384859261124,105.310822493709));
#80712=CARTESIAN_POINT('Ctrl Pts',(20.0424519231406,772.226279657433,106.668510439474));
#80713=CARTESIAN_POINT('Ctrl Pts',(13.2983736491593,777.107328840337,108.39363837514));
#80714=CARTESIAN_POINT('',(37.297438237489,740.125373936259,83.3197325254973));
#80715=CARTESIAN_POINT('Ctrl Pts',(-3.53207921104705,801.327714069793,97.6774171598034));
#80716=CARTESIAN_POINT('Ctrl Pts',(-3.52587249025034,801.317418707077,97.6740101620181));
#80717=CARTESIAN_POINT('Ctrl Pts',(-3.51962667648031,801.307146848781,97.6703505307767));
#80718=CARTESIAN_POINT('Ctrl Pts',(-3.51334807640392,801.296826345139,97.6666767907112));
#80719=CARTESIAN_POINT('Ctrl Pts',(-3.5106008964837,801.292310644183,97.6650693583509));
#80720=CARTESIAN_POINT('Ctrl Pts',(-3.50784744134078,801.287785628975,97.6634592331446));
#80721=CARTESIAN_POINT('Ctrl Pts',(-3.50508824012168,801.283252220773,97.6618466990113));
#80722=CARTESIAN_POINT('Ctrl Pts',(-3.49201375725401,801.261770653046,97.6542057014094));
#80723=CARTESIAN_POINT('Ctrl Pts',(-3.47868041561161,801.239995695538,97.646128608076));
#80724=CARTESIAN_POINT('Ctrl Pts',(-3.46537855240211,801.218215478767,97.6383364608635));
#80725=CARTESIAN_POINT('Ctrl Pts',(-3.46229474298644,801.213166108127,97.636529984841));
#80726=CARTESIAN_POINT('Ctrl Pts',(-3.4592126975727,801.208116512442,97.6347390358641));
#80727=CARTESIAN_POINT('Ctrl Pts',(-3.45613613830592,801.203070365482,97.6329729068014));
#80728=CARTESIAN_POINT('Ctrl Pts',(-3.4304744809274,801.160980328153,97.6182415803537));
#80729=CARTESIAN_POINT('Ctrl Pts',(-3.40459867550778,801.118642251537,97.6034680866934));
#80730=CARTESIAN_POINT('Ctrl Pts',(-3.37884385789892,801.076686597832,97.5886127519183));
#80731=CARTESIAN_POINT('Ctrl Pts',(-3.32744721036587,800.992959351992,97.5589672534716));
#80732=CARTESIAN_POINT('Ctrl Pts',(-3.27586200981757,800.909393845096,97.529356289513));
#80733=CARTESIAN_POINT('Ctrl Pts',(-3.22408722923495,800.825990597834,97.4997811184006));
#80734=CARTESIAN_POINT('Ctrl Pts',(-3.19288321141107,800.775724495596,97.4819565297466));
#80735=CARTESIAN_POINT('Ctrl Pts',(-3.16161031478435,800.725517304614,97.464144933854));
#80736=CARTESIAN_POINT('Ctrl Pts',(-3.13026831930153,800.675369158711,97.4463466147331));
#80737=CARTESIAN_POINT('Ctrl Pts',(-3.05760287905582,800.559102244513,97.4050817662566));
#80738=CARTESIAN_POINT('Ctrl Pts',(-2.98456554311726,800.443153214223,97.3638884681123));
#80739=CARTESIAN_POINT('Ctrl Pts',(-2.91115554479481,800.3275217629,97.3227696504956));
#80740=CARTESIAN_POINT('Ctrl Pts',(-2.76326137054251,800.094566873895,97.2399303409108));
#80741=CARTESIAN_POINT('Ctrl Pts',(-2.61385506024094,799.86290132501,97.1573933949809));
#80742=CARTESIAN_POINT('Ctrl Pts',(-2.46292804567857,799.632522498369,97.0751821615028));
#80743=CARTESIAN_POINT('Ctrl Pts',(-2.39939935499147,799.535550692089,97.0405775412644));
#80744=CARTESIAN_POINT('Ctrl Pts',(-2.3356003334188,799.438808100775,97.0060312761693));
#80745=CARTESIAN_POINT('Ctrl Pts',(-2.27153217997277,799.342292332637,96.9715441428051));
#80746=CARTESIAN_POINT('Ctrl Pts',(-1.92974275328136,798.827402059012,96.7875629148974));
#80747=CARTESIAN_POINT('Ctrl Pts',(-1.58030992268464,798.318982584886,96.6052745778218));
#80748=CARTESIAN_POINT('Ctrl Pts',(-1.22344040148274,797.816762200364,96.4248254346384));
#80749=CARTESIAN_POINT('Ctrl Pts',(-1.17154198831683,797.743725867845,96.3985832827258));
#80750=CARTESIAN_POINT('Ctrl Pts',(-1.11948623212914,797.670820699189,96.3723800465563));
#80751=CARTESIAN_POINT('Ctrl Pts',(-1.06727370425656,797.59804591967,96.3462161961521));
#80752=CARTESIAN_POINT('Ctrl Pts',(-1.02414389435495,797.537930799138,96.3246037222842));
#80753=CARTESIAN_POINT('Ctrl Pts',(-0.980906989626348,797.477905472924,
96.3030187351991));
#80754=CARTESIAN_POINT('Ctrl Pts',(-0.937563757151817,797.417968716901,
96.2814610407467));
#80755=CARTESIAN_POINT('Ctrl Pts',(-0.405606907320748,796.682357501429,
96.0168807919786));
#80756=CARTESIAN_POINT('Ctrl Pts',(0.1423611097153,795.960080192847,95.7564278130585));
#80757=CARTESIAN_POINT('Ctrl Pts',(0.704521420287423,795.249490032763,95.4999771464207));
#80758=CARTESIAN_POINT('Ctrl Pts',(1.10745352353966,794.740169857773,95.3161644429169));
#80759=CARTESIAN_POINT('Ctrl Pts',(1.51767785039838,794.236855021861,95.1344083618379));
#80760=CARTESIAN_POINT('Ctrl Pts',(1.93453138702115,793.738951725696,94.954670179249));
#80761=CARTESIAN_POINT('Ctrl Pts',(1.93694797209831,793.736065278612,94.9536282003003));
#80762=CARTESIAN_POINT('Ctrl Pts',(1.93936478014842,793.73317901318,94.9525862891865));
#80763=CARTESIAN_POINT('Ctrl Pts',(1.9417818110133,793.730292929321,94.9515444459138));
#80764=CARTESIAN_POINT('Ctrl Pts',(2.46152573053298,793.10968664788,94.727512674564));
#80765=CARTESIAN_POINT('Ctrl Pts',(2.99136899894459,792.497326343745,94.5065323530685));
#80766=CARTESIAN_POINT('Ctrl Pts',(3.52988153404372,791.89198649273,94.288351414471));
#80767=CARTESIAN_POINT('Ctrl Pts',(4.07175701103376,791.282866371786,94.0688079638234));
#80768=CARTESIAN_POINT('Ctrl Pts',(4.62241032479021,790.680854621645,93.8520989609514));
#80769=CARTESIAN_POINT('Ctrl Pts',(5.18034579587942,790.084667031274,93.6379591178906));
#80770=CARTESIAN_POINT('Ctrl Pts',(5.74430546766639,789.482042220322,93.4215071411534));
#80771=CARTESIAN_POINT('Ctrl Pts',(6.31570537878925,788.885367999664,93.2076801009325));
#80772=CARTESIAN_POINT('Ctrl Pts',(6.8929619902048,788.293282271603,92.996195468457));
#80773=CARTESIAN_POINT('Ctrl Pts',(7.35536276565974,787.819002905412,92.8267895991787));
#80774=CARTESIAN_POINT('Ctrl Pts',(7.82152073377076,787.347667044819,92.6588865708896));
#80775=CARTESIAN_POINT('Ctrl Pts',(8.29060449945157,786.878558472934,92.4923373092731));
#80776=CARTESIAN_POINT('Ctrl Pts',(8.37840289062202,786.790755438787,92.4611642901017));
#80777=CARTESIAN_POINT('Ctrl Pts',(8.4663027434857,786.70303137381,92.4300390763354));
#80778=CARTESIAN_POINT('Ctrl Pts',(8.55429849135774,786.615381572838,92.3989606884239));
#80779=CARTESIAN_POINT('Ctrl Pts',(9.2020771922392,785.970149552205,92.1701778411428));
#80780=CARTESIAN_POINT('Ctrl Pts',(9.85516593914095,785.328922519864,91.9438905224339));
#80781=CARTESIAN_POINT('Ctrl Pts',(10.5119316825118,784.690249367814,91.7199934851448));
#80782=CARTESIAN_POINT('Ctrl Pts',(11.1784195477638,784.042121919023,91.492782093678));
#80783=CARTESIAN_POINT('Ctrl Pts',(11.8486939692838,783.396624421051,91.2680322692314));
#80784=CARTESIAN_POINT('Ctrl Pts',(12.5210102394924,782.752202308121,91.0456283092697));
#80785=CARTESIAN_POINT('Ctrl Pts',(13.2092167288867,782.092549255413,90.8179678237289));
#80786=CARTESIAN_POINT('Ctrl Pts',(13.8995626461569,781.434022950849,90.5927654025733));
#80787=CARTESIAN_POINT('Ctrl Pts',(14.5901383989481,780.77491761496,90.3698910252198));
#80788=CARTESIAN_POINT('Ctrl Pts',(14.7454939012683,780.626641860816,90.3197520495779));
#80789=CARTESIAN_POINT('Ctrl Pts',(14.9008608885752,780.478336654654,90.2697308715161));
#80790=CARTESIAN_POINT('Ctrl Pts',(15.0562173685823,780.329982323209,90.2198259708646));
#80791=CARTESIAN_POINT('Ctrl Pts',(15.2025918930187,780.190205117184,90.172806328687));
#80792=CARTESIAN_POINT('Ctrl Pts',(15.3489560630232,780.050385112899,90.1258907692892));
#80793=CARTESIAN_POINT('Ctrl Pts',(15.4952926315725,779.910504634489,90.0790775852241));
#80794=CARTESIAN_POINT('Ctrl Pts',(16.1928584000468,779.2437141365,89.855925743953));
#80795=CARTESIAN_POINT('Ctrl Pts',(16.889954019786,778.575674525802,89.6351177879038));
#80796=CARTESIAN_POINT('Ctrl Pts',(17.5847563840439,777.904658212687,89.4168036934157));
#80797=CARTESIAN_POINT('Ctrl Pts',(18.2975118197521,777.216303438401,89.1928485580525));
#80798=CARTESIAN_POINT('Ctrl Pts',(19.0078543826094,776.524816528801,88.9715177779207));
#80799=CARTESIAN_POINT('Ctrl Pts',(19.7137724683992,775.828294175026,88.7529787110537));
#80800=CARTESIAN_POINT('Ctrl Pts',(20.3772626986632,775.173634964287,88.54757451655));
#80801=CARTESIAN_POINT('Ctrl Pts',(21.0368441158626,774.514527240835,88.3446365659295));
#80802=CARTESIAN_POINT('Ctrl Pts',(21.6908079933751,773.849356636992,88.1443086044901));
#80803=CARTESIAN_POINT('Ctrl Pts',(21.7326266723076,773.806821327514,88.1314983392924));
#80804=CARTESIAN_POINT('Ctrl Pts',(21.7744223670276,773.764261214263,88.1186987483769));
#80805=CARTESIAN_POINT('Ctrl Pts',(21.8161946252474,773.721675870246,88.1059098700103));
#80806=CARTESIAN_POINT('Ctrl Pts',(21.9874035471954,773.547134412572,88.053493022768));
#80807=CARTESIAN_POINT('Ctrl Pts',(22.1582247673597,773.372162484028,88.0012561601995));
#80808=CARTESIAN_POINT('Ctrl Pts',(22.3286263866547,773.196731155624,87.9492018283233));
#80809=CARTESIAN_POINT('Ctrl Pts',(22.9217001552904,772.586151752073,87.7680294961155));
#80810=CARTESIAN_POINT('Ctrl Pts',(23.5096391298023,771.969986601658,87.5891234565314));
#80811=CARTESIAN_POINT('Ctrl Pts',(24.0901190310581,771.347652427082,87.4129600323426));
#80812=CARTESIAN_POINT('Ctrl Pts',(24.4191223749035,770.994926994243,87.3131144468262));
#80813=CARTESIAN_POINT('Ctrl Pts',(24.7457287032067,770.640219608101,87.2141500896773));
#80814=CARTESIAN_POINT('Ctrl Pts',(25.0695077938623,770.283422208196,87.1161552851402));
#80815=CARTESIAN_POINT('Ctrl Pts',(25.2378156931276,770.097950624099,87.0652153073388));
#80816=CARTESIAN_POINT('Ctrl Pts',(25.4053776088423,769.911894013562,87.0145331826002));
#80817=CARTESIAN_POINT('Ctrl Pts',(25.5721341822133,769.725234149169,86.9641212714148));
#80818=CARTESIAN_POINT('Ctrl Pts',(26.0657199242206,769.172736302715,86.8149061605171));
#80819=CARTESIAN_POINT('Ctrl Pts',(26.5524710659009,768.614757993071,86.667993036751));
#80820=CARTESIAN_POINT('Ctrl Pts',(27.0309765036493,768.050324506237,86.5236723647956));
#80821=CARTESIAN_POINT('Ctrl Pts',(27.4081607721694,767.605407029726,86.4099108841739));
#80822=CARTESIAN_POINT('Ctrl Pts',(27.7802208709166,767.15647821111,86.2977603859367));
#80823=CARTESIAN_POINT('Ctrl Pts',(28.1464464456118,766.703049004253,86.1873675997798));
#80824=CARTESIAN_POINT('Ctrl Pts',(28.2997018283907,766.513301287377,86.14117123921));
#80825=CARTESIAN_POINT('Ctrl Pts',(28.4519381960058,766.322761541815,86.0952825656747));
#80826=CARTESIAN_POINT('Ctrl Pts',(28.6031049900163,766.131389970733,86.049711726047));
#80827=CARTESIAN_POINT('Ctrl Pts',(29.0146873705057,765.610341897316,85.9256358350576));
#80828=CARTESIAN_POINT('Ctrl Pts',(29.4183518970935,765.083145013738,85.8039128044781));
#80829=CARTESIAN_POINT('Ctrl Pts',(29.8128239835195,764.548824944325,85.6848253174677));
#80830=CARTESIAN_POINT('Ctrl Pts',(30.1808879757273,764.050275149214,85.5737101906962));
#80831=CARTESIAN_POINT('Ctrl Pts',(30.5409489517119,763.545523878989,85.4648895910462));
#80832=CARTESIAN_POINT('Ctrl Pts',(30.8919292568867,763.033753666233,85.3586037439776));
#80833=CARTESIAN_POINT('Ctrl Pts',(30.9171116196388,762.997034844825,85.3509778780335));
#80834=CARTESIAN_POINT('Ctrl Pts',(30.9422472176289,762.960279879347,85.3433650653162));
#80835=CARTESIAN_POINT('Ctrl Pts',(30.9673356440519,762.923488462468,85.3357653967386));
#80836=CARTESIAN_POINT('Ctrl Pts',(31.0931562269573,762.738976391463,85.2976524153105));
#80837=CARTESIAN_POINT('Ctrl Pts',(31.2177928973397,762.553543736145,85.2598702174453));
#80838=CARTESIAN_POINT('Ctrl Pts',(31.3411923375727,762.367153525296,85.2224307953528));
#80839=CARTESIAN_POINT('Ctrl Pts',(31.67162055091,761.868054143339,85.1221787899384));
#80840=CARTESIAN_POINT('Ctrl Pts',(31.9931781805276,761.362119302838,85.0243785666424));
#80841=CARTESIAN_POINT('Ctrl Pts',(32.3046347587608,760.848393719462,84.9293386946084));
#80842=CARTESIAN_POINT('Ctrl Pts',(32.6103846810005,760.344080861276,84.8360401884446));
#80843=CARTESIAN_POINT('Ctrl Pts',(32.9064003732124,759.83226018293,84.745401791375));
#80844=CARTESIAN_POINT('Ctrl Pts',(33.191477489211,759.311999617512,84.6577259631547));
#80845=CARTESIAN_POINT('Ctrl Pts',(33.2722338246568,759.164620770238,84.6328892498695));
#80846=CARTESIAN_POINT('Ctrl Pts',(33.3521121179694,759.016564468346,84.6082903403824));
#80847=CARTESIAN_POINT('Ctrl Pts',(33.4310843780547,758.867809091466,84.5839362708936));
#80848=CARTESIAN_POINT('Ctrl Pts',(33.5184886981044,758.703170741799,84.5569818582706));
#80849=CARTESIAN_POINT('Ctrl Pts',(33.604784507844,758.537673273943,84.5303280434968));
#80850=CARTESIAN_POINT('Ctrl Pts',(33.6899309478928,758.371291959995,84.5039849906636));
#80851=CARTESIAN_POINT('Ctrl Pts',(33.9690198476379,757.825935303612,84.4176390010139));
#80852=CARTESIAN_POINT('Ctrl Pts',(34.235731054912,757.271036232819,84.3346450446765));
#80853=CARTESIAN_POINT('Ctrl Pts',(34.4885049018037,756.705379129562,84.2554525761138));
#80854=CARTESIAN_POINT('Ctrl Pts',(34.5543284959757,756.558079145551,84.2348304548925));
#80855=CARTESIAN_POINT('Ctrl Pts',(34.6192302660274,756.409996636499,84.2144591104201));
#80856=CARTESIAN_POINT('Ctrl Pts',(34.683162161741,756.261152515248,84.1943530418467));
#80857=CARTESIAN_POINT('Ctrl Pts',(34.7794358499984,756.037011304225,84.1640757388463));
#80858=CARTESIAN_POINT('Ctrl Pts',(34.8731112642366,755.81203754227,84.134524996995));
#80859=CARTESIAN_POINT('Ctrl Pts',(34.9640667158625,755.586434948884,84.1057441504196));
#80860=CARTESIAN_POINT('Ctrl Pts',(35.1154224134244,755.211017782751,84.0578509781911));
#80861=CARTESIAN_POINT('Ctrl Pts',(35.2592674497983,754.833824929926,84.0120879836128));
#80862=CARTESIAN_POINT('Ctrl Pts',(35.3954459345825,754.454814897335,83.968523258549));
#80863=CARTESIAN_POINT('Ctrl Pts',(35.4390765570408,754.33338276607,83.9545654290521));
#80864=CARTESIAN_POINT('Ctrl Pts',(35.4819193465824,754.211765261265,83.9408333754645));
#80865=CARTESIAN_POINT('Ctrl Pts',(35.5239629769602,754.08997669971,83.9273314983401));
#80866=CARTESIAN_POINT('Ctrl Pts',(35.6660146583664,753.678492967467,83.8817130698071));
#80867=CARTESIAN_POINT('Ctrl Pts',(35.7989765135005,753.264811291308,83.8387082730724));
#80868=CARTESIAN_POINT('Ctrl Pts',(35.92285624938,752.848949522755,83.7983768427954));
#80869=CARTESIAN_POINT('Ctrl Pts',(36.0471797986685,752.431597881562,83.7579009205283));
#80870=CARTESIAN_POINT('Ctrl Pts',(36.1623561247641,752.012050272139,83.7201175790626));
#80871=CARTESIAN_POINT('Ctrl Pts',(36.268442795898,751.590333930163,83.6850727875611));
#80872=CARTESIAN_POINT('Ctrl Pts',(36.3750616706859,751.166501969178,83.6498521872997));
#80873=CARTESIAN_POINT('Ctrl Pts',(36.4724995532146,750.740479226775,83.6173977076522));
#80874=CARTESIAN_POINT('Ctrl Pts',(36.5608637350915,750.312306102992,83.5877411049482));
#80875=CARTESIAN_POINT('Ctrl Pts',(36.5947655315134,750.148033229442,83.5763630546332));
#80876=CARTESIAN_POINT('Ctrl Pts',(36.6273322267701,749.983443982138,83.5653966803727));
#80877=CARTESIAN_POINT('Ctrl Pts',(36.6585717280759,749.818541249099,83.5548431863892));
#80878=CARTESIAN_POINT('Ctrl Pts',(36.6697841668005,749.759354587583,83.5510553408836));
#80879=CARTESIAN_POINT('Ctrl Pts',(36.6808256450559,749.700127543216,83.547320581778));
#80880=CARTESIAN_POINT('Ctrl Pts',(36.6916965257908,749.640860451538,83.5436389647139));
#80881=CARTESIAN_POINT('Ctrl Pts',(36.7715340805677,749.205593080501,83.5166005571378));
#80882=CARTESIAN_POINT('Ctrl Pts',(36.8420681306053,748.768117375119,83.4924835988422));
#80883=CARTESIAN_POINT('Ctrl Pts',(36.9040112041995,748.328578403737,83.4710984305574));
#80884=CARTESIAN_POINT('Ctrl Pts',(36.9678585923859,747.875526695119,83.4490558184996));
#80885=CARTESIAN_POINT('Ctrl Pts',(37.0225793411126,747.420282447104,83.4299153750923));
#80886=CARTESIAN_POINT('Ctrl Pts',(37.0689991241824,746.963034706298,83.4134539836569));
#80887=CARTESIAN_POINT('Ctrl Pts',(37.117061798547,746.489604030473,83.3964099898287));
#80888=CARTESIAN_POINT('Ctrl Pts',(37.1562263895217,746.014024962391,83.3822378239292));
#80889=CARTESIAN_POINT('Ctrl Pts',(37.1874453911839,745.536547323445,83.3706765172477));
#80890=CARTESIAN_POINT('Ctrl Pts',(37.1988089751989,745.362747490762,83.3664682507177));
#80891=CARTESIAN_POINT('Ctrl Pts',(37.209120094727,745.188696526882,83.3626057969649));
#80892=CARTESIAN_POINT('Ctrl Pts',(37.2184254531716,745.014407957878,83.3590762444424));
#80893=CARTESIAN_POINT('Ctrl Pts',(37.2187740305499,745.00787913335,83.3589440279166));
#80894=CARTESIAN_POINT('Ctrl Pts',(37.2191211971741,745.00134996549,83.3588122778083));
#80895=CARTESIAN_POINT('Ctrl Pts',(37.2194669555068,744.994820454777,83.3586809934331));
#80896=CARTESIAN_POINT('Ctrl Pts',(37.2425322364403,744.559241656856,83.3499231105201));
#80897=CARTESIAN_POINT('Ctrl Pts',(37.2594390596283,744.122700322152,83.343187806879));
#80898=CARTESIAN_POINT('Ctrl Pts',(37.2716207511684,743.685890065863,83.3380039330951));
#80899=CARTESIAN_POINT('Ctrl Pts',(37.2818457931714,743.31924121392,83.3336527042856));
#80900=CARTESIAN_POINT('Ctrl Pts',(37.2887414425155,742.952402928708,83.3303946352932));
#80901=CARTESIAN_POINT('Ctrl Pts',(37.293128367296,742.585781657886,83.3279600207453));
#80902=CARTESIAN_POINT('Ctrl Pts',(37.2931885805528,742.580749554113,83.3279266041543));
#80903=CARTESIAN_POINT('Ctrl Pts',(37.2932483203103,742.575717439987,83.3278933422545));
#80904=CARTESIAN_POINT('Ctrl Pts',(37.2933075895563,742.570685315405,83.3278602340709));
#80905=CARTESIAN_POINT('Ctrl Pts',(37.2974212094887,742.221427489737,83.3255623394062));
#80906=CARTESIAN_POINT('Ctrl Pts',(37.2992717289621,741.872143582838,83.3240043233008));
#80907=CARTESIAN_POINT('Ctrl Pts',(37.2998365932158,741.522834600892,83.3228583018915));
#80908=CARTESIAN_POINT('Ctrl Pts',(37.3003789001298,741.187474955125,83.3217580458038));
#80909=CARTESIAN_POINT('Ctrl Pts',(37.299736351987,740.852092203344,83.3210374820026));
#80910=CARTESIAN_POINT('Ctrl Pts',(37.2987309819122,740.516704184972,83.320420517403));
#80911=CARTESIAN_POINT('Ctrl Pts',(37.2983399605194,740.386260785713,83.3201805596371));
#80912=CARTESIAN_POINT('Ctrl Pts',(37.2978935698031,740.255816775995,83.3199564322173));
#80913=CARTESIAN_POINT('Ctrl Pts',(37.297438237489,740.125373936259,83.3197325254973));
#80914=CARTESIAN_POINT('',(37.2974382339422,740.125373764374,83.3197325252249));
#80915=CARTESIAN_POINT('Ctrl Pts',(68.4577991911175,740.125189855522,98.7804139696777));
#80916=CARTESIAN_POINT('Ctrl Pts',(68.4314744168991,747.666651921185,98.7691090655225));
#80917=CARTESIAN_POINT('Ctrl Pts',(68.4050070734591,755.208031515623,98.7576983734677));
#80918=CARTESIAN_POINT('Ctrl Pts',(78.1222855324702,768.384861541845,105.310823299793));
#80919=CARTESIAN_POINT('Ctrl Pts',(85.7127868619961,772.226281106417,106.668510951594));
#80920=CARTESIAN_POINT('Ctrl Pts',(92.4568631339348,777.107328840337,108.39363837514));
#80921=CARTESIAN_POINT('Ctrl Pts',(68.4577992118746,740.125183909083,97.9632437490832));
#80922=CARTESIAN_POINT('Ctrl Pts',(68.430623262492,747.910488740229,97.953471433172));
#80923=CARTESIAN_POINT('Ctrl Pts',(68.4032928480487,755.695714014116,97.9435914375012));
#80924=CARTESIAN_POINT('Ctrl Pts',(78.9327187735727,768.917219170172,104.62754444939));
#80925=CARTESIAN_POINT('Ctrl Pts',(86.7452316640843,773.033321350878,106.046458844125));
#80926=CARTESIAN_POINT('Ctrl Pts',(93.6239591044408,778.248433884114,107.853507205599));
#80927=CARTESIAN_POINT('Ctrl Pts',(68.4577992329346,740.125177875847,97.1460735284887));
#80928=CARTESIAN_POINT('Ctrl Pts',(68.4297596841829,748.157884729622,97.1378338008051));
#80929=CARTESIAN_POINT('Ctrl Pts',(68.4015541154982,756.190515080161,97.1294854786493));
#80930=CARTESIAN_POINT('Ctrl Pts',(79.7198124540396,769.450651027237,103.926505090804));
#80931=CARTESIAN_POINT('Ctrl Pts',(87.7496608967702,773.852732995686,105.411629894754));
#80932=CARTESIAN_POINT('Ctrl Pts',(94.75050390177,779.413657557974,107.305932045411));
#80933=CARTESIAN_POINT('Ctrl Pts',(68.4577992542868,740.125171758922,96.3289033078942));
#80934=CARTESIAN_POINT('Ctrl Pts',(68.4288841269008,748.408712427461,96.3221961684255));
#80935=CARTESIAN_POINT('Ctrl Pts',(68.3997916362531,756.69217974737,96.3153802040162));
#80936=CARTESIAN_POINT('Ctrl Pts',(80.4924129928722,769.987477901082,103.219552953207));
#80937=CARTESIAN_POINT('Ctrl Pts',(88.7309063108587,774.685953843899,104.770645558223));
#80938=CARTESIAN_POINT('Ctrl Pts',(95.8384290337387,780.602056150837,106.751733915294));
#80939=CARTESIAN_POINT('Ctrl Pts',(68.4577992759202,740.125165561416,95.5117330872998));
#80940=CARTESIAN_POINT('Ctrl Pts',(68.4279970355747,748.662844371844,95.5065585360376));
#80941=CARTESIAN_POINT('Ctrl Pts',(68.3980061750953,757.200453046912,95.5012753218122));
#80942=CARTESIAN_POINT('Ctrl Pts',(81.2590704459109,770.530187531119,102.518460172987));
#80943=CARTESIAN_POINT('Ctrl Pts',(89.6935032939934,775.534588649946,104.130051696489));
#80944=CARTESIAN_POINT('Ctrl Pts',(96.8893696450024,781.812852902992,106.191658243183));
#80945=CARTESIAN_POINT('Ctrl Pts',(68.457799319728,740.125153011461,93.8773926461109));
#80946=CARTESIAN_POINT('Ctrl Pts',(68.4262006746925,749.177461829888,93.8752832712527));
#80947=CARTESIAN_POINT('Ctrl Pts',(68.3943908261618,758.229706968641,93.8730657605118));
#80948=CARTESIAN_POINT('Ctrl Pts',(82.7970768809045,771.632645704261,101.151412605607));
#80949=CARTESIAN_POINT('Ctrl Pts',(91.5899487624662,777.266193608426,102.862611652065));
#80950=CARTESIAN_POINT('Ctrl Pts',(98.9200297042542,784.277987128321,105.061117676372));
#80951=CARTESIAN_POINT('Ctrl Pts',(68.4577993419023,740.125146659012,93.0602224255164));
#80952=CARTESIAN_POINT('Ctrl Pts',(68.4252914051331,749.437947343551,93.0596456388496));
#80953=CARTESIAN_POINT('Ctrl Pts',(68.3925612750287,758.750687577726,93.0589617044525));
#80954=CARTESIAN_POINT('Ctrl Pts',(83.5454184581273,772.193289626093,100.442877153979));
#80955=CARTESIAN_POINT('Ctrl Pts',(92.5136141758915,778.147951298143,102.213866283972));
#80956=CARTESIAN_POINT('Ctrl Pts',(99.8997491522424,785.532324601496,104.490652781672));
#80957=CARTESIAN_POINT('Ctrl Pts',(68.4577993643362,740.125140232198,92.2430522049219));
#80958=CARTESIAN_POINT('Ctrl Pts',(68.4243714913817,749.70148217995,92.2440080064353));
#80959=CARTESIAN_POINT('Ctrl Pts',(68.3907108896609,759.277766932611,92.2448585685712));
#80960=CARTESIAN_POINT('Ctrl Pts',(84.2626728179383,772.761297551471,99.6877930536026));
#80961=CARTESIAN_POINT('Ctrl Pts',(93.4098678056052,779.043420219821,101.539441004633));
#80962=CARTESIAN_POINT('Ctrl Pts',(100.84523195766,786.807804636399,103.915676206375));
#80963=CARTESIAN_POINT('Ctrl Pts',(68.4577993870189,740.125133734129,91.4258819843274));
#80964=CARTESIAN_POINT('Ctrl Pts',(68.4234413783645,749.967938877182,91.4283703740089));
#80965=CARTESIAN_POINT('Ctrl Pts',(68.3888407163122,759.810690128692,91.430756549369));
#80966=CARTESIAN_POINT('Ctrl Pts',(84.9381531776121,773.334767609609,98.8645608264283));
#80967=CARTESIAN_POINT('Ctrl Pts',(94.275593983119,779.950505355874,100.828618751446));
#80968=CARTESIAN_POINT('Ctrl Pts',(101.757590853987,788.103948395178,103.336808383945));
#80969=CARTESIAN_POINT('Ctrl Pts',(68.4577994213996,740.125123884805,90.2001266534357));
#80970=CARTESIAN_POINT('Ctrl Pts',(68.4220315773295,750.371815521424,90.20491392535));
#80971=CARTESIAN_POINT('Ctrl Pts',(68.3860073486596,760.618458324829,90.2096054914207));
#80972=CARTESIAN_POINT('Ctrl Pts',(85.8723434708061,774.20050954551,97.4950169758646));
#80973=CARTESIAN_POINT('Ctrl Pts',(95.5233794963349,781.325611310863,99.6916402144542));
#80974=CARTESIAN_POINT('Ctrl Pts',(103.077773363038,790.07863781811,102.463526327259));
#80975=CARTESIAN_POINT('Ctrl Pts',(68.4577994329193,740.12512058466,89.7915415431385));
#80976=CARTESIAN_POINT('Ctrl Pts',(68.4215592050669,750.507139669237,89.797095109128));
#80977=CARTESIAN_POINT('Ctrl Pts',(68.3850581429893,760.889111659347,89.8025553875324));
#80978=CARTESIAN_POINT('Ctrl Pts',(86.1750232524054,774.487588917475,97.0215011063112));
#80979=CARTESIAN_POINT('Ctrl Pts',(95.933007509302,781.785483359929,99.3035995687804));
#80980=CARTESIAN_POINT('Ctrl Pts',(103.509774893482,790.741946589881,102.171602254524));
#80981=CARTESIAN_POINT('Ctrl Pts',(68.4577994444972,740.125117267868,89.3829564328412));
#80982=CARTESIAN_POINT('Ctrl Pts',(68.4210844498364,750.643146484044,89.3892762929044));
#80983=CARTESIAN_POINT('Ctrl Pts',(68.3841042630244,761.161130386228,89.3955054536124));
#80984=CARTESIAN_POINT('Ctrl Pts',(86.4714289387005,774.773865563578,96.5353477393156));
#80985=CARTESIAN_POINT('Ctrl Pts',(96.3374018422195,782.247433893577,98.9088166869112));
#80986=CARTESIAN_POINT('Ctrl Pts',(103.933827953702,791.410290842359,101.87891950692));
#80987=CARTESIAN_POINT('Ctrl Pts',(68.4577994561318,740.125113934815,88.9743713225439));
#80988=CARTESIAN_POINT('Ctrl Pts',(68.4206073672543,750.779820033107,88.9814574766802));
#80989=CARTESIAN_POINT('Ctrl Pts',(68.3831457844632,761.434482628579,88.9884556109133));
#80990=CARTESIAN_POINT('Ctrl Pts',(86.763989289185,775.060046216945,96.0409175425288));
#80991=CARTESIAN_POINT('Ctrl Pts',(96.7376151784749,782.712046184646,98.5095940450559));
#80992=CARTESIAN_POINT('Ctrl Pts',(104.350029251381,792.083635277778,101.585546375814));
#80993=CARTESIAN_POINT('Ctrl Pts',(68.4577994795118,740.125107236968,88.1572011019495));
#80994=CARTESIAN_POINT('Ctrl Pts',(68.4196486586195,751.054468734271,88.1658198442325));
#80995=CARTESIAN_POINT('Ctrl Pts',(68.3812197819262,761.983790390204,88.17435595054));
#80996=CARTESIAN_POINT('Ctrl Pts',(87.3462507788668,775.633644251365,95.0442194679357));
#80997=CARTESIAN_POINT('Ctrl Pts',(97.5317591657831,783.647776074199,97.7068688370514));
#80998=CARTESIAN_POINT('Ctrl Pts',(105.166895678368,793.440269165875,100.99755057259));
#80999=CARTESIAN_POINT('Ctrl Pts',(68.4577994912571,740.125103872174,87.7486159916522));
#81000=CARTESIAN_POINT('Ctrl Pts',(68.4191670325668,751.192443886372,87.758001028009));
#81001=CARTESIAN_POINT('Ctrl Pts',(68.3802522579229,762.259745909587,87.767306132953));
#81002=CARTESIAN_POINT('Ctrl Pts',(87.6359537956839,775.921054293985,94.5419456284517));
#81003=CARTESIAN_POINT('Ctrl Pts',(97.9256898168359,784.118893672684,97.3033662709022));
#81004=CARTESIAN_POINT('Ctrl Pts',(105.567560807675,794.123558618553,100.702927900473));
#81005=CARTESIAN_POINT('Ctrl Pts',(68.4577995030566,740.125100491896,87.3400308813549));
#81006=CARTESIAN_POINT('Ctrl Pts',(68.4186831903952,751.331053907253,87.3501822117867));
#81007=CARTESIAN_POINT('Ctrl Pts',(68.3792802829773,762.536971190724,87.3602562494283));
#81008=CARTESIAN_POINT('Ctrl Pts',(87.9269247718117,776.209776667823,94.0400932925943));
#81009=CARTESIAN_POINT('Ctrl Pts',(98.3175187793482,784.593854821168,96.9000235404456));
#81010=CARTESIAN_POINT('Ctrl Pts',(105.960541531152,794.81179290555,100.407746070846));
#81011=CARTESIAN_POINT('Ctrl Pts',(68.4577995149088,740.125097096526,86.9314457710577));
#81012=CARTESIAN_POINT('Ctrl Pts',(68.418197187721,751.470282864177,86.9423633955665));
#81013=CARTESIAN_POINT('Ctrl Pts',(68.3783039290729,762.815434356689,86.9532062214676));
#81014=CARTESIAN_POINT('Ctrl Pts',(88.2218463652581,776.500520302144,93.543006087808));
#81015=CARTESIAN_POINT('Ctrl Pts',(98.7082726780542,785.073258039394,96.4991377651511));
#81016=CARTESIAN_POINT('Ctrl Pts',(106.345908497826,795.504951976008,100.112068018336));
#81017=CARTESIAN_POINT('Ctrl Pts',(68.4577995506192,740.125086866296,85.7056904401659));
#81018=CARTESIAN_POINT('Ctrl Pts',(68.4167328650399,751.889778744866,85.7189069469152));
#81019=CARTESIAN_POINT('Ctrl Pts',(68.3753619469564,763.654441877978,85.7320554688825));
#81020=CARTESIAN_POINT('Ctrl Pts',(89.126475179618,777.380962958098,92.079063941594));
#81021=CARTESIAN_POINT('Ctrl Pts',(99.8803532649971,786.526610646288,95.310735855761));
#81022=CARTESIAN_POINT('Ctrl Pts',(107.479344282573,797.599164568952,99.2237271886368));
#81023=CARTESIAN_POINT('Ctrl Pts',(68.4577995746314,740.125079987321,84.8885202195714));
#81024=CARTESIAN_POINT('Ctrl Pts',(68.415748230377,752.171854678547,84.9032693144991));
#81025=CARTESIAN_POINT('Ctrl Pts',(68.3733831076234,764.218604097713,84.9179534581158));
#81026=CARTESIAN_POINT('Ctrl Pts',(89.7759151781224,777.989739099571,91.1817265572392));
#81027=CARTESIAN_POINT('Ctrl Pts',(100.667408968764,787.523124895316,94.5593136514548));
#81028=CARTESIAN_POINT('Ctrl Pts',(108.204747985368,799.014953473009,98.6297577392777));
#81029=CARTESIAN_POINT('Ctrl Pts',(68.4577995988381,740.125073052633,84.0713499989769));
#81030=CARTESIAN_POINT('Ctrl Pts',(68.4147556210969,752.456215163547,84.0876316820978));
#81031=CARTESIAN_POINT('Ctrl Pts',(68.3713879526406,764.787335304437,84.1038504221104));
#81032=CARTESIAN_POINT('Ctrl Pts',(90.4503596257349,778.617103253815,90.3217783746812));
#81033=CARTESIAN_POINT('Ctrl Pts',(101.452424543665,788.543884485768,93.8278698898637));
#81034=CARTESIAN_POINT('Ctrl Pts',(108.900401281468,800.450285635657,98.0345313843018));
#81035=CARTESIAN_POINT('Ctrl Pts',(68.4577996232285,740.12506606534,83.2541797783824));
#81036=CARTESIAN_POINT('Ctrl Pts',(68.4137554821241,752.742732737961,83.2719940497075));
#81037=CARTESIAN_POINT('Ctrl Pts',(68.3693776870735,765.36038061127,83.289746845202));
#81038=CARTESIAN_POINT('Ctrl Pts',(91.1282679588575,779.259942042811,89.4579482431207));
#81039=CARTESIAN_POINT('Ctrl Pts',(102.227500324588,789.585635228018,93.0955009722738));
#81040=CARTESIAN_POINT('Ctrl Pts',(109.566583027439,801.905170120104,97.4384971415098));
#81041=CARTESIAN_POINT('Ctrl Pts',(68.4577996477916,740.125059028551,82.4370095577878));
#81042=CARTESIAN_POINT('Ctrl Pts',(68.4127482583835,753.031279939886,82.4563564173248));
#81043=CARTESIAN_POINT('Ctrl Pts',(68.3673535182661,765.937485129951,82.4756432120661));
#81044=CARTESIAN_POINT('Ctrl Pts',(91.7879438810236,779.915237078138,88.5489418011639));
#81045=CARTESIAN_POINT('Ctrl Pts',(102.984580913554,790.645217922039,92.3412800893767));
#81046=CARTESIAN_POINT('Ctrl Pts',(110.203416346979,803.379710979161,96.8420808181083));
#81047=CARTESIAN_POINT('',(68.4577985491519,740.125373764374,83.3197325252249));
#81048=CARTESIAN_POINT('',(68.4577985491519,740.125373764374,83.3197325252249));
#81049=CARTESIAN_POINT('Ctrl Pts',(68.4577985491519,740.125373764374,83.3197325252249));
#81050=CARTESIAN_POINT('Ctrl Pts',(68.4521142211524,741.75380716905,83.3224194785555));
#81051=CARTESIAN_POINT('Ctrl Pts',(68.4499256999464,743.382130664584,83.3261020865078));
#81052=CARTESIAN_POINT('Ctrl Pts',(68.5797134472817,745.820412963062,83.3752834133531));
#81053=CARTESIAN_POINT('Ctrl Pts',(68.6448130821809,746.634567916206,83.3988648178505));
#81054=CARTESIAN_POINT('Ctrl Pts',(68.8296879542825,748.245163355258,83.4636594090421));
#81055=CARTESIAN_POINT('Ctrl Pts',(68.9493582190413,749.04253454444,83.5048356188137));
#81056=CARTESIAN_POINT('Ctrl Pts',(69.3984362959591,751.408519901678,83.656381909957));
#81057=CARTESIAN_POINT('Ctrl Pts',(69.8191726784943,752.950650995558,83.7950334335352));
#81058=CARTESIAN_POINT('Ctrl Pts',(70.6317188459528,755.211605983176,84.0548612189204));
#81059=CARTESIAN_POINT('Ctrl Pts',(70.9324330224284,755.95665758029,84.1500172544934));
#81060=CARTESIAN_POINT('Ctrl Pts',(71.4258868704458,757.062054538247,84.3045997067613));
#81061=CARTESIAN_POINT('Ctrl Pts',(71.5976113189271,757.428799566548,84.3581584224953));
#81062=CARTESIAN_POINT('Ctrl Pts',(71.9513538712402,758.15192384479,84.4680386926666));
#81063=CARTESIAN_POINT('Ctrl Pts',(72.1337262198999,758.509139597191,84.5244719529524));
#81064=CARTESIAN_POINT('Ctrl Pts',(73.0709910162594,760.27515071812,84.813518540632));
#81065=CARTESIAN_POINT('Ctrl Pts',(73.9015561965611,761.624180220335,85.0665674297279));
#81066=CARTESIAN_POINT('Ctrl Pts',(75.6790516558849,764.230121938606,85.6050503921944));
#81067=CARTESIAN_POINT('Ctrl Pts',(76.6261100820584,765.486924428665,85.8905575072476));
#81068=CARTESIAN_POINT('Ctrl Pts',(78.6034328418404,767.934229456814,86.4866793099093));
#81069=CARTESIAN_POINT('Ctrl Pts',(79.6338181982263,769.124636451881,86.7973264992592));
#81070=CARTESIAN_POINT('Ctrl Pts',(81.7524708372019,771.458757542837,87.4386664033878));
#81071=CARTESIAN_POINT('Ctrl Pts',(82.8414898324954,772.603045483691,87.7695806430336));
#81072=CARTESIAN_POINT('Ctrl Pts',(86.1553991306081,775.980737157317,88.7843870404448));
#81073=CARTESIAN_POINT('Ctrl Pts',(88.4295363397,778.162606809164,89.4905766503777));
#81074=CARTESIAN_POINT('Ctrl Pts',(92.9793970190661,782.507828567648,90.9525504249873));
#81075=CARTESIAN_POINT('Ctrl Pts',(95.256518702732,784.669931234052,91.708224027398));
#81076=CARTESIAN_POINT('Ctrl Pts',(99.6798110453827,789.094244285017,93.2790928565411));
#81077=CARTESIAN_POINT('Ctrl Pts',(101.826042863888,791.356276291902,94.0946429907112));
#81078=CARTESIAN_POINT('Ctrl Pts',(104.820439166947,794.933117908512,95.3858318597951));
#81079=CARTESIAN_POINT('Ctrl Pts',(105.780609774061,796.156382916215,95.827771932233));
#81080=CARTESIAN_POINT('Ctrl Pts',(107.150002788981,798.050254358706,96.5089305255182));
#81081=CARTESIAN_POINT('Ctrl Pts',(107.594705916051,798.691342353046,96.7389844066105));
#81082=CARTESIAN_POINT('Ctrl Pts',(108.243331370894,799.668541513458,97.0881426854701));
#81083=CARTESIAN_POINT('Ctrl Pts',(108.456477837002,799.996861973796,97.2052035713835));
#81084=CARTESIAN_POINT('Ctrl Pts',(108.771609297049,800.493252018569,97.3817121458909));
#81085=CARTESIAN_POINT('Ctrl Pts',(108.875889222769,800.65936627551,97.4407009280924));
#81086=CARTESIAN_POINT('Ctrl Pts',(109.082932430931,800.992892849213,97.5589647600582));
#81087=CARTESIAN_POINT('Ctrl Pts',(109.186653881671,801.161883674408,97.6187977856326));
#81088=CARTESIAN_POINT('Ctrl Pts',(109.28716016657,801.327730313361,97.677680855745));
#81089=CARTESIAN_POINT('Origin',(52.8776183915471,763.53825870998,301.513705792983));
#81090=CARTESIAN_POINT('',(109.164743594634,804.5210255586,96.7791116555879));
#81091=CARTESIAN_POINT('',(-3.40942206489524,804.520974706055,96.7791223637616));
#81092=CARTESIAN_POINT('Ctrl Pts',(109.164743594634,804.5210255586,96.7791116555879));
#81093=CARTESIAN_POINT('Ctrl Pts',(108.81785985458,804.8963810802,96.7588565871085));
#81094=CARTESIAN_POINT('Ctrl Pts',(108.468245873048,805.269049622901,96.7392277597907));
#81095=CARTESIAN_POINT('Ctrl Pts',(108.11577894047,805.639042885829,96.720204176775));
#81096=CARTESIAN_POINT('Ctrl Pts',(107.74545819184,806.027777741361,96.7002169755574));
#81097=CARTESIAN_POINT('Ctrl Pts',(107.37198808282,806.413559445882,96.6808978891222));
#81098=CARTESIAN_POINT('Ctrl Pts',(106.995272778489,806.7963641143,96.6622233680472));
#81099=CARTESIAN_POINT('Ctrl Pts',(106.613731311482,807.184072957255,96.643309604564));
#81100=CARTESIAN_POINT('Ctrl Pts',(106.228861219377,807.568727757392,96.6250570349512));
#81101=CARTESIAN_POINT('Ctrl Pts',(105.840607577229,807.950268251547,96.6074419190684));
#81102=CARTESIAN_POINT('Ctrl Pts',(105.434092518505,808.349754410979,96.5889982804513));
#81103=CARTESIAN_POINT('Ctrl Pts',(105.023868199041,808.74582631095,96.5712534762176));
#81104=CARTESIAN_POINT('Ctrl Pts',(104.609918091164,809.138378549129,96.5541809523683));
#81105=CARTESIAN_POINT('Ctrl Pts',(104.248161472504,809.481435278985,96.5392610420162));
#81106=CARTESIAN_POINT('Ctrl Pts',(103.883560272872,809.821803233661,96.5248545843592));
#81107=CARTESIAN_POINT('Ctrl Pts',(103.516129310237,810.159392437004,96.5109442003283));
#81108=CARTESIAN_POINT('Ctrl Pts',(103.06479988911,810.574066090609,96.4938575467505));
#81109=CARTESIAN_POINT('Ctrl Pts',(102.60906554779,810.98464433311,96.4775075766846));
#81110=CARTESIAN_POINT('Ctrl Pts',(102.148842854877,811.391053015295,96.4618608159888));
#81111=CARTESIAN_POINT('Ctrl Pts',(101.653703754645,811.828295316299,96.4450269589631));
#81112=CARTESIAN_POINT('Ctrl Pts',(101.153369718894,812.260711381115,96.4290070688144));
#81113=CARTESIAN_POINT('Ctrl Pts',(100.64777226437,812.688159362852,96.4137620187931));
#81114=CARTESIAN_POINT('Ctrl Pts',(100.087326977579,813.161977426152,96.3968631670388));
#81115=CARTESIAN_POINT('Ctrl Pts',(99.5204148958492,813.629691121572,96.3809163971792));
#81116=CARTESIAN_POINT('Ctrl Pts',(98.9469783994167,814.09104744428,96.3658713278112));
#81117=CARTESIAN_POINT('Ctrl Pts',(98.4269437329283,814.509439511936,96.3522273451213));
#81118=CARTESIAN_POINT('Ctrl Pts',(97.901544405208,814.922601805145,96.3393250150671));
#81119=CARTESIAN_POINT('Ctrl Pts',(97.3707511754493,815.330311529557,96.3271282343743));
#81120=CARTESIAN_POINT('Ctrl Pts',(96.666210865658,815.87147882303,96.310939023273));
#81121=CARTESIAN_POINT('Ctrl Pts',(95.9550708055675,816.40080863672,96.2960592932168));
#81122=CARTESIAN_POINT('Ctrl Pts',(95.2375484879537,816.917927766701,96.2823758101844));
#81123=CARTESIAN_POINT('Ctrl Pts',(94.6380435770987,817.349991620758,96.2709429737775));
#81124=CARTESIAN_POINT('Ctrl Pts',(94.0340839728432,817.773530116061,96.2603453667684));
#81125=CARTESIAN_POINT('Ctrl Pts',(93.4257633003275,818.18833773882,96.250518440248));
#81126=CARTESIAN_POINT('Ctrl Pts',(92.8704692631059,818.566987043239,96.2415481159642));
#81127=CARTESIAN_POINT('Ctrl Pts',(92.3115417089347,818.938360749592,96.2332200210036));
#81128=CARTESIAN_POINT('Ctrl Pts',(91.74901452317,819.302323611573,96.2254853180879));
#81129=CARTESIAN_POINT('Ctrl Pts',(91.2207405796963,819.644124152493,96.2182215944595));
#81130=CARTESIAN_POINT('Ctrl Pts',(90.6892923056537,819.979388560072,96.2114812282335));
#81131=CARTESIAN_POINT('Ctrl Pts',(90.154658713138,820.3080299507,96.2052234643063));
#81132=CARTESIAN_POINT('Ctrl Pts',(89.6564796614257,820.614262590454,96.1993923924419));
#81133=CARTESIAN_POINT('Ctrl Pts',(89.1555349269183,820.914744481525,96.1939803706782));
#81134=CARTESIAN_POINT('Ctrl Pts',(88.6517785687755,821.209430866217,96.188953827893));
#81135=CARTESIAN_POINT('Ctrl Pts',(88.164171040949,821.494670540519,96.1840884201193));
#81136=CARTESIAN_POINT('Ctrl Pts',(87.6739294792162,821.774480098891,96.1795841890942));
#81137=CARTESIAN_POINT('Ctrl Pts',(87.1809740020025,822.048846495541,96.1754098686499));
#81138=CARTESIAN_POINT('Ctrl Pts',(86.7101113032903,822.310916617355,96.1714226286647));
#81139=CARTESIAN_POINT('Ctrl Pts',(86.236772571269,822.568020427466,96.167736400845));
#81140=CARTESIAN_POINT('Ctrl Pts',(85.7608508452064,822.820174359809,96.1643229932653));
#81141=CARTESIAN_POINT('Ctrl Pts',(85.3585836922947,823.03330445853,96.1614378512899));
#81142=CARTESIAN_POINT('Ctrl Pts',(84.9544706744878,823.242898585414,96.1587476093714));
#81143=CARTESIAN_POINT('Ctrl Pts',(84.5484240257377,823.448984348812,96.1562345944108));
#81144=CARTESIAN_POINT('Ctrl Pts',(84.3196278766203,823.56510802376,96.15481857941));
#81145=CARTESIAN_POINT('Ctrl Pts',(84.0902168468878,823.680118401631,96.1534588149677));
#81146=CARTESIAN_POINT('Ctrl Pts',(83.860148425969,823.794016828468,96.1521530930805));
#81147=CARTESIAN_POINT('Ctrl Pts',(83.4412841428411,824.001381153896,96.1497758860737));
#81148=CARTESIAN_POINT('Ctrl Pts',(83.0206056486588,824.204892507276,96.1475840276166));
#81149=CARTESIAN_POINT('Ctrl Pts',(82.5979699841252,824.404530042682,96.1455626897761));
#81150=CARTESIAN_POINT('Ctrl Pts',(82.1749665556623,824.604341296235,96.1435395930324));
#81151=CARTESIAN_POINT('Ctrl Pts',(81.7500025546443,824.800271983972,96.1416873134641));
#81152=CARTESIAN_POINT('Ctrl Pts',(81.3229848179643,824.992286687618,96.1399910525799));
#81153=CARTESIAN_POINT('Ctrl Pts',(80.8953263404622,825.184589509646,96.1382922464535));
#81154=CARTESIAN_POINT('Ctrl Pts',(80.465607961045,825.372964584677,96.1367499272253));
#81155=CARTESIAN_POINT('Ctrl Pts',(80.0337863500513,825.5573618177,96.135349303189));
#81156=CARTESIAN_POINT('Ctrl Pts',(79.6015643180971,825.741930039194,96.1339473803775));
#81157=CARTESIAN_POINT('Ctrl Pts',(79.1672351601097,825.922513033928,96.132687415312));
#81158=CARTESIAN_POINT('Ctrl Pts',(78.7308056556793,826.099046084197,96.1315546539312));
#81159=CARTESIAN_POINT('Ctrl Pts',(78.293687855145,826.275857546007,96.1304201060643));
#81160=CARTESIAN_POINT('Ctrl Pts',(77.8544630820329,826.448606275714,96.1294131630575));
#81161=CARTESIAN_POINT('Ctrl Pts',(77.4131884314279,826.617212779452,96.1285190853947));
#81162=CARTESIAN_POINT('Ctrl Pts',(77.1269068793251,826.72659801497,96.1279390431452));
#81163=CARTESIAN_POINT('Ctrl Pts',(76.839763575618,826.834239534435,96.1274065065369));
#81164=CARTESIAN_POINT('Ctrl Pts',(76.5517853843881,826.94011239358,96.1269174709266));
#81165=CARTESIAN_POINT('Ctrl Pts',(76.1094254387221,827.102742459485,96.1261662690211));
#81166=CARTESIAN_POINT('Ctrl Pts',(75.6649961893313,827.261246404981,96.1255203741796));
#81167=CARTESIAN_POINT('Ctrl Pts',(75.2184220958277,827.415588632804,96.1249665290083));
#81168=CARTESIAN_POINT('Ctrl Pts',(74.777972940969,827.567813996506,96.1244202800404));
#81169=CARTESIAN_POINT('Ctrl Pts',(74.3354373538775,827.715991025202,96.1239635813572));
#81170=CARTESIAN_POINT('Ctrl Pts',(73.8907836577821,827.860056255693,96.1235840476201));
#81171=CARTESIAN_POINT('Ctrl Pts',(73.5114595775302,827.982955067808,96.1232602759142));
#81172=CARTESIAN_POINT('Ctrl Pts',(73.1305946682942,828.102861107367,96.122992668282));
#81173=CARTESIAN_POINT('Ctrl Pts',(72.7481937098735,828.219717553959,96.1227736657644));
#81174=CARTESIAN_POINT('Ctrl Pts',(72.3376562878923,828.345172114858,96.1225385493846));
#81175=CARTESIAN_POINT('Ctrl Pts',(71.925008210908,828.467179924549,96.1223492899608));
#81176=CARTESIAN_POINT('Ctrl Pts',(71.5109237265998,828.585474558666,96.122201589357));
#81177=CARTESIAN_POINT('Ctrl Pts',(71.0891856621001,828.705955648695,96.1220511587827));
#81178=CARTESIAN_POINT('Ctrl Pts',(70.665957780851,828.822584769025,96.1219438236296));
#81179=CARTESIAN_POINT('Ctrl Pts',(70.242000467664,828.935106602914,96.1218746129595));
#81180=CARTESIAN_POINT('Ctrl Pts',(69.9067472443637,829.024085625872,96.1218198831565));
#81181=CARTESIAN_POINT('Ctrl Pts',(69.571038934021,829.110496760903,96.1217889821186));
#81182=CARTESIAN_POINT('Ctrl Pts',(69.2352705986298,829.194226670312,96.1217793560992));
#81183=CARTESIAN_POINT('Ctrl Pts',(69.1074681048227,829.226096534444,96.1217756921764));
#81184=CARTESIAN_POINT('Ctrl Pts',(68.979657110544,829.257578070376,96.1217751100857));
#81185=CARTESIAN_POINT('Ctrl Pts',(68.8518554245239,829.288669335678,96.1217775923678));
#81186=CARTESIAN_POINT('Ctrl Pts',(68.3162220814629,829.418976837027,96.121787995932));
#81187=CARTESIAN_POINT('Ctrl Pts',(67.7796819487752,829.542652600751,96.1218398401812));
#81188=CARTESIAN_POINT('Ctrl Pts',(67.2424596078188,829.659711642437,96.1219241710703));
#81189=CARTESIAN_POINT('Ctrl Pts',(66.7045825480914,829.776913345263,96.1220086047345));
#81190=CARTESIAN_POINT('Ctrl Pts',(66.1660216083883,829.887482190453,96.1221256049698));
#81191=CARTESIAN_POINT('Ctrl Pts',(65.6269501649236,829.991428532487,96.1222666012994));
#81192=CARTESIAN_POINT('Ctrl Pts',(65.0870382729811,830.095536933828,96.1224078174518));
#81193=CARTESIAN_POINT('Ctrl Pts',(64.5466142815548,830.193002168601,96.1225731052528));
#81194=CARTESIAN_POINT('Ctrl Pts',(64.0058002959459,830.283829877612,96.1227542611935));
#81195=CARTESIAN_POINT('Ctrl Pts',(63.4645517895842,830.374730562776,96.1229355626852));
#81196=CARTESIAN_POINT('Ctrl Pts',(62.9229126551899,830.458983054191,96.1231327585445));
#81197=CARTESIAN_POINT('Ctrl Pts',(62.3809532481644,830.536588205254,96.1233380223962));
#81198=CARTESIAN_POINT('Ctrl Pts',(61.8386286725166,830.614245646149,96.1235434245533));
#81199=CARTESIAN_POINT('Ctrl Pts',(61.2959833867929,830.685246788226,96.1237569062999));
#81200=CARTESIAN_POINT('Ctrl Pts',(60.7530358914191,830.749587646318,96.1239710119053));
#81201=CARTESIAN_POINT('Ctrl Pts',(60.2097935247798,830.813963447514,96.12418523379));
#81202=CARTESIAN_POINT('Ctrl Pts',(59.6662486156575,830.871671731051,96.1244000809341));
#81203=CARTESIAN_POINT('Ctrl Pts',(59.1223677365911,830.922703623813,96.1246084613678));
#81204=CARTESIAN_POINT('Ctrl Pts',(58.5781800982875,830.97376429954,96.124816959332));
#81205=CARTESIAN_POINT('Ctrl Pts',(58.0336561089993,831.01814105406,96.1250189840038));
#81206=CARTESIAN_POINT('Ctrl Pts',(57.4887103301528,831.055820072134,96.1252077968563));
#81207=CARTESIAN_POINT('Ctrl Pts',(56.943659265322,831.093506369965,96.1253966461883));
#81208=CARTESIAN_POINT('Ctrl Pts',(56.3981862451516,831.124492345937,96.1255722793249));
#81209=CARTESIAN_POINT('Ctrl Pts',(55.8521538618925,831.148759205987,96.1257283084493));
#81210=CARTESIAN_POINT('Ctrl Pts',(55.3060711495201,831.173028302772,96.1258843519552));
#81211=CARTESIAN_POINT('Ctrl Pts',(54.7594289696607,831.190577048051,96.1260207885621));
#81212=CARTESIAN_POINT('Ctrl Pts',(54.2120379841324,831.201381626344,96.1261315723995));
#81213=CARTESIAN_POINT('Ctrl Pts',(53.8259906871007,831.209001551326,96.1262097026613));
#81214=CARTESIAN_POINT('Ctrl Pts',(53.4395698705124,831.213266977978,96.1262750810007));
#81215=CARTESIAN_POINT('Ctrl Pts',(53.0526936028336,831.214168039196,96.1263256865));
#81216=CARTESIAN_POINT('Ctrl Pts',(53.0507674189968,831.21417252541,96.1263259384553));
#81217=CARTESIAN_POINT('Ctrl Pts',(53.0488412238427,831.214176928223,96.1263261900445));
#81218=CARTESIAN_POINT('Ctrl Pts',(53.0469150173836,831.214181247634,96.126326441268));
#81219=CARTESIAN_POINT('Ctrl Pts',(52.3346198024729,831.215778530047,96.1264193416725));
#81220=CARTESIAN_POINT('Ctrl Pts',(51.6215169228228,831.205826030126,96.1264155205298));
#81221=CARTESIAN_POINT('Ctrl Pts',(50.9075293471847,831.184317742721,96.1263391289961));
#81222=CARTESIAN_POINT('Ctrl Pts',(50.1715641524487,831.162147397649,96.1262603860152));
#81223=CARTESIAN_POINT('Ctrl Pts',(49.4346598209972,831.127701084149,96.1261044758506));
#81224=CARTESIAN_POINT('Ctrl Pts',(48.6967885724123,831.080969582942,96.125896924031));
#81225=CARTESIAN_POINT('Ctrl Pts',(48.000718975506,831.036885500157,96.1257011303723));
#81226=CARTESIAN_POINT('Ctrl Pts',(47.3037901271249,830.981870161356,96.1254593251443));
#81227=CARTESIAN_POINT('Ctrl Pts',(46.6060121350389,830.915887966615,96.125192980259));
#81228=CARTESIAN_POINT('Ctrl Pts',(46.0831370663034,830.866444669461,96.1249933965779));
#81229=CARTESIAN_POINT('Ctrl Pts',(45.5597859324478,830.810842890367,96.124780029375));
#81230=CARTESIAN_POINT('Ctrl Pts',(45.0359707212101,830.749049777422,96.1245622001286));
#81231=CARTESIAN_POINT('Ctrl Pts',(44.4025671667175,830.674328813725,96.1242987984251));
#81232=CARTESIAN_POINT('Ctrl Pts',(43.7714150067874,830.590901454991,96.1240300924934));
#81233=CARTESIAN_POINT('Ctrl Pts',(43.1426290306698,830.498910823778,96.1237662142207));
#81234=CARTESIAN_POINT('Ctrl Pts',(42.5654376360675,830.414468417718,96.12352398829));
#81235=CARTESIAN_POINT('Ctrl Pts',(41.9902401605419,830.322810512071,96.1232858165673));
#81236=CARTESIAN_POINT('Ctrl Pts',(41.4171018972515,830.224010399001,96.1230601152048));
#81237=CARTESIAN_POINT('Ctrl Pts',(40.8646821681992,830.128781838654,96.1228425727836));
#81238=CARTESIAN_POINT('Ctrl Pts',(40.3141756799341,830.026918383084,96.1226366023955));
#81239=CARTESIAN_POINT('Ctrl Pts',(39.7656155656075,829.918446237259,96.1224504934597));
#81240=CARTESIAN_POINT('Ctrl Pts',(39.2433139742531,829.815166445487,96.1222732932026));
#81241=CARTESIAN_POINT('Ctrl Pts',(38.7227769897778,829.705895614109,96.1221140905957));
#81242=CARTESIAN_POINT('Ctrl Pts',(38.2040076146669,829.590617471609,96.1219808803541));
#81243=CARTESIAN_POINT('Ctrl Pts',(37.8404778949911,829.509835851031,96.1218875327432));
#81244=CARTESIAN_POINT('Ctrl Pts',(37.4778156605375,829.426103522171,96.1218069655784));
#81245=CARTESIAN_POINT('Ctrl Pts',(37.1160133445364,829.339402126673,96.1217422273291));
#81246=CARTESIAN_POINT('Ctrl Pts',(36.9923124132681,829.30975874715,96.1217200931929));
#81247=CARTESIAN_POINT('Ctrl Pts',(36.8687142495218,829.279774758988,96.1217017401159));
#81248=CARTESIAN_POINT('Ctrl Pts',(36.7452224780983,829.249449924558,96.1216872005585));
#81249=CARTESIAN_POINT('Ctrl Pts',(36.2993203358342,829.139953490261,96.121634701354));
#81250=CARTESIAN_POINT('Ctrl Pts',(35.8548008687036,829.02601443886,96.1216319013983));
#81251=CARTESIAN_POINT('Ctrl Pts',(35.4115522887877,828.907694732824,96.1216850275004));
#81252=CARTESIAN_POINT('Ctrl Pts',(34.9603240819995,828.787244964451,96.1217391100104));
#81253=CARTESIAN_POINT('Ctrl Pts',(34.5104129852087,828.662255071877,96.1218511518375));
#81254=CARTESIAN_POINT('Ctrl Pts',(34.0617533635338,828.532776578757,96.1220280134034));
#81255=CARTESIAN_POINT('Ctrl Pts',(33.6002876660254,828.399602385552,96.1222099231228));
#81256=CARTESIAN_POINT('Ctrl Pts',(33.1401459038875,828.261679322302,96.1224604071805));
#81257=CARTESIAN_POINT('Ctrl Pts',(32.6813112387729,828.119054297259,96.1227872133734));
#81258=CARTESIAN_POINT('Ctrl Pts',(32.2149424150519,827.974087340269,96.1231193857905));
#81259=CARTESIAN_POINT('Ctrl Pts',(31.749924115111,827.824262281401,96.1235304099026));
#81260=CARTESIAN_POINT('Ctrl Pts',(31.2862929699484,827.669625492323,96.1240286780445));
#81261=CARTESIAN_POINT('Ctrl Pts',(30.812451946628,827.511583360892,96.1245379188251));
#81262=CARTESIAN_POINT('Ctrl Pts',(30.3400599943064,827.348514711429,96.1251382913234));
#81263=CARTESIAN_POINT('Ctrl Pts',(29.8692102824549,827.180473645186,96.1258389792862));
#81264=CARTESIAN_POINT('Ctrl Pts',(29.7316433704635,827.131377532374,96.1260436974307));
#81265=CARTESIAN_POINT('Ctrl Pts',(29.5942084434188,827.081857023802,96.1262569799536));
#81266=CARTESIAN_POINT('Ctrl Pts',(29.4569086376803,827.031913643688,96.1264790588299));
#81267=CARTESIAN_POINT('Ctrl Pts',(28.9763315010338,826.857101694897,96.1272563798895));
#81268=CARTESIAN_POINT('Ctrl Pts',(28.4972902395431,826.677116185297,96.1281568157707));
#81269=CARTESIAN_POINT('Ctrl Pts',(28.0197389778897,826.491962153884,96.1291981422069));
#81270=CARTESIAN_POINT('Ctrl Pts',(27.5380280346519,826.305195349401,96.1302485390545));
#81271=CARTESIAN_POINT('Ctrl Pts',(27.0578334044021,826.113168931253,96.1314422860078));
#81272=CARTESIAN_POINT('Ctrl Pts',(26.5791611724838,825.915895118084,96.1327981858621));
#81273=CARTESIAN_POINT('Ctrl Pts',(26.2452186745877,825.778268354828,96.1337441203744));
#81274=CARTESIAN_POINT('Ctrl Pts',(25.9120209680096,825.638088956988,96.1347689780978));
#81275=CARTESIAN_POINT('Ctrl Pts',(25.579575465666,825.495361925563,96.1358793542484));
#81276=CARTESIAN_POINT('Ctrl Pts',(25.1043935615804,825.291354645937,96.1374664734899));
#81277=CARTESIAN_POINT('Ctrl Pts',(24.6307299666174,825.082134386464,96.1392283111973));
#81278=CARTESIAN_POINT('Ctrl Pts',(24.1585815459311,824.867703385282,96.1411851424814));
#81279=CARTESIAN_POINT('Ctrl Pts',(24.0645301183577,824.824988974106,96.1415749410442));
#81280=CARTESIAN_POINT('Ctrl Pts',(23.9705389615557,824.782067872531,96.1419724803075));
#81281=CARTESIAN_POINT('Ctrl Pts',(23.8766082699099,824.738940216866,96.142377925612));
#81282=CARTESIAN_POINT('Ctrl Pts',(23.5242791952853,824.57717065311,96.1438987295842));
#81283=CARTESIAN_POINT('Ctrl Pts',(23.1726904806387,824.412439784918,96.1455313567798));
#81284=CARTESIAN_POINT('Ctrl Pts',(22.8225264021466,824.245069168157,96.1472764201388));
#81285=CARTESIAN_POINT('Ctrl Pts',(22.5641059405136,824.121549953298,96.1485642737667));
#81286=CARTESIAN_POINT('Ctrl Pts',(22.3064613514965,823.996594101978,96.1499133413435));
#81287=CARTESIAN_POINT('Ctrl Pts',(22.0498649176053,823.870348867314,96.1513233720859));
#81288=CARTESIAN_POINT('Ctrl Pts',(21.8205654519541,823.757533718598,96.1525834024413));
#81289=CARTESIAN_POINT('Ctrl Pts',(21.5919627696193,823.643633984308,96.1538967179459));
#81290=CARTESIAN_POINT('Ctrl Pts',(21.3640843664886,823.528679500814,96.1552654445697));
#81291=CARTESIAN_POINT('Ctrl Pts',(20.6897210395786,823.188493301213,96.1593159338962));
#81292=CARTESIAN_POINT('Ctrl Pts',(20.0216970167957,822.839071979066,96.1638516478053));
#81293=CARTESIAN_POINT('Ctrl Pts',(19.3597612622417,822.48059179808,96.1689367561272));
#81294=CARTESIAN_POINT('Ctrl Pts',(18.6797438547955,822.11231925559,96.174160770926));
#81295=CARTESIAN_POINT('Ctrl Pts',(18.0061520763646,821.734486260633,96.1799646020606));
#81296=CARTESIAN_POINT('Ctrl Pts',(17.3387696085509,821.34728998514,96.1864183552341));
#81297=CARTESIAN_POINT('Ctrl Pts',(16.6518654105832,820.94876775853,96.1930608883562));
#81298=CARTESIAN_POINT('Ctrl Pts',(15.9715393097476,820.540326539864,96.2003919176625));
#81299=CARTESIAN_POINT('Ctrl Pts',(15.2976106450826,820.122186493828,96.2084884921846));
#81300=CARTESIAN_POINT('Ctrl Pts',(14.5906904817536,819.683576823195,96.2169814263535));
#81301=CARTESIAN_POINT('Ctrl Pts',(13.8908095443592,819.234295555008,96.2263166860551));
#81302=CARTESIAN_POINT('Ctrl Pts',(13.1978169881674,818.774601332847,96.2365839510869));
#81303=CARTESIAN_POINT('Ctrl Pts',(12.4824725211103,818.300080047702,96.2471823783956));
#81304=CARTESIAN_POINT('Ctrl Pts',(11.7744682831821,817.814463333678,96.258773896731));
#81305=CARTESIAN_POINT('Ctrl Pts',(11.0736948546628,817.318039228885,96.2714580313752));
#81306=CARTESIAN_POINT('Ctrl Pts',(10.334954086467,816.794719266112,96.2848293822136));
#81307=CARTESIAN_POINT('Ctrl Pts',(9.60424912359563,816.259389196666,96.2994149405681));
#81308=CARTESIAN_POINT('Ctrl Pts',(8.88150935089614,815.712389091413,96.3153324022128));
#81309=CARTESIAN_POINT('Ctrl Pts',(8.737364605695,815.603294236287,96.318507014348));
#81310=CARTESIAN_POINT('Ctrl Pts',(8.59353685960559,815.493735186086,96.3217346094189));
#81311=CARTESIAN_POINT('Ctrl Pts',(8.45002579119955,815.38371464605,96.3250161265263));
#81312=CARTESIAN_POINT('Ctrl Pts',(7.73485923702806,814.835443273122,96.3413690901561));
#81313=CARTESIAN_POINT('Ctrl Pts',(7.02744314731507,814.275599585686,96.3590559958425));
#81314=CARTESIAN_POINT('Ctrl Pts',(6.32763648910812,813.704382912701,96.3781977036289));
#81315=CARTESIAN_POINT('Ctrl Pts',(5.98839153239689,813.427474464879,96.387477020642));
#81316=CARTESIAN_POINT('Ctrl Pts',(5.65093560132485,813.147893119755,96.3970982758466));
#81317=CARTESIAN_POINT('Ctrl Pts',(5.31525674903631,812.865660336836,96.4070755760922));
#81318=CARTESIAN_POINT('Ctrl Pts',(4.88604189826204,812.504784157183,96.4198330238934));
#81319=CARTESIAN_POINT('Ctrl Pts',(4.45941044659712,812.139296345883,96.4331827773792));
#81320=CARTESIAN_POINT('Ctrl Pts',(4.03593287282361,811.769745606281,96.4471373618657));
#81321=CARTESIAN_POINT('Ctrl Pts',(3.60939542391928,811.397524644717,96.461192776452));
#81322=CARTESIAN_POINT('Ctrl Pts',(3.18605779243993,811.021182033279,96.4758618462414));
#81323=CARTESIAN_POINT('Ctrl Pts',(2.76646984314789,810.641319253384,96.4911510252356));
#81324=CARTESIAN_POINT('Ctrl Pts',(2.60477662834758,810.494934605856,96.4970428925007));
#81325=CARTESIAN_POINT('Ctrl Pts',(2.44363989332385,810.348027610871,96.5030267777089));
#81326=CARTESIAN_POINT('Ctrl Pts',(2.28308971551838,810.200634184955,96.5091027768158));
#81327=CARTESIAN_POINT('Ctrl Pts',(1.59637390937374,809.57019330546,96.5350914408076));
#81328=CARTESIAN_POINT('Ctrl Pts',(0.920061146645233,808.930567192885,96.562778850032));
#81329=CARTESIAN_POINT('Ctrl Pts',(0.253832209561208,808.28208074038,96.5922727164801));
#81330=CARTESIAN_POINT('Ctrl Pts',(-0.434923194360932,807.611667728168,
96.6227638266195));
#81331=CARTESIAN_POINT('Ctrl Pts',(-1.11290049535978,806.931785155324,96.6551855659363));
#81332=CARTESIAN_POINT('Ctrl Pts',(-1.78043670077545,806.242737817501,96.6896592282327));
#81333=CARTESIAN_POINT('Ctrl Pts',(-2.33045840547436,805.674991846132,96.7180640733178));
#81334=CARTESIAN_POINT('Ctrl Pts',(-2.87339101909581,805.101022796369,96.7478620175358));
#81335=CARTESIAN_POINT('Ctrl Pts',(-3.40942206489524,804.520974706055,96.7791223637616));
#81336=CARTESIAN_POINT('Origin',(52.8776183915471,832.414102583906,106.637502983816));
#81337=CARTESIAN_POINT('Ctrl Pts',(68.4577985491519,740.125373764374,82.4370100295875));
#81338=CARTESIAN_POINT('Ctrl Pts',(68.4127473761225,753.031531728391,82.4563567944567));
#81339=CARTESIAN_POINT('Ctrl Pts',(68.3676962032424,765.937689649662,82.4757320753115));
#81340=CARTESIAN_POINT('Ctrl Pts',(91.7880530990439,779.91534174428,88.5489787937199));
#81341=CARTESIAN_POINT('Ctrl Pts',(102.984616121786,790.64528003164,92.3413020410111));
#81342=CARTESIAN_POINT('Ctrl Pts',(110.203416346979,803.379710979161,96.8420808181083));
#81343=CARTESIAN_POINT('Ctrl Pts',(68.146245887415,740.125373764374,82.1411634292565));
#81344=CARTESIAN_POINT('Ctrl Pts',(68.1013386355289,753.27209360235,82.1623170532707));
#81345=CARTESIAN_POINT('Ctrl Pts',(68.0564326571535,766.41881340126,82.1834984289274));
#81346=CARTESIAN_POINT('Ctrl Pts',(90.6389575804412,780.789138080197,88.3851212990028));
#81347=CARTESIAN_POINT('Ctrl Pts',(101.882701838135,791.724397584064,92.2074425549413));
#81348=CARTESIAN_POINT('Ctrl Pts',(109.112490425402,804.596520123409,96.7733914942943));
#81349=CARTESIAN_POINT('Ctrl Pts',(67.8275991955539,740.125373764374,81.8527984530498));
#81350=CARTESIAN_POINT('Ctrl Pts',(67.7829212500557,753.508784911136,81.8757450226982));
#81351=CARTESIAN_POINT('Ctrl Pts',(67.7382457320547,766.892196022395,81.8987186035317));
#81352=CARTESIAN_POINT('Ctrl Pts',(89.4941280640034,781.614609851677,88.2295744554866));
#81353=CARTESIAN_POINT('Ctrl Pts',(100.768263665002,792.773015962468,92.0801584109773));
#81354=CARTESIAN_POINT('Ctrl Pts',(107.999153078758,805.790564251154,96.7101361882138));
#81355=CARTESIAN_POINT('Ctrl Pts',(67.5021302853703,740.125373764374,81.5720908670709));
#81356=CARTESIAN_POINT('Ctrl Pts',(67.4577640330222,753.741304019782,81.5968129309024));
#81357=CARTESIAN_POINT('Ctrl Pts',(67.4134012477569,767.357234243137,81.6215612893473));
#81358=CARTESIAN_POINT('Ctrl Pts',(88.3519233861698,782.395636392562,88.0819107242408));
#81359=CARTESIAN_POINT('Ctrl Pts',(99.6387825034722,793.793017584272,91.9592106396445));
#81360=CARTESIAN_POINT('Ctrl Pts',(106.860546215042,806.962773547768,96.6519976135905));
#81361=CARTESIAN_POINT('Ctrl Pts',(67.1701109686658,740.125373764374,81.2992164374233));
#81362=CARTESIAN_POINT('Ctrl Pts',(67.1261357977477,753.969349293325,81.3256930060463));
#81363=CARTESIAN_POINT('Ctrl Pts',(67.0821650240712,767.813324793557,81.3521951765969));
#81364=CARTESIAN_POINT('Ctrl Pts',(87.2125822519353,783.134553009413,87.941736205412));
#81365=CARTESIAN_POINT('Ctrl Pts',(98.4936191231884,794.784740839621,91.8443939105452));
#81366=CARTESIAN_POINT('Ctrl Pts',(105.695691610809,808.11253417135,96.598692123225));
#81367=CARTESIAN_POINT('Ctrl Pts',(66.4935151458177,740.125373764374,80.7694854229978));
#81368=CARTESIAN_POINT('Ctrl Pts',(66.4504749173554,754.415888900274,80.7994219465401));
#81369=CARTESIAN_POINT('Ctrl Pts',(66.4074407375454,768.706404013894,80.8293827344099));
#81370=CARTESIAN_POINT('Ctrl Pts',(84.9422477192991,784.531226837734,87.6756031833855));
#81371=CARTESIAN_POINT('Ctrl Pts',(96.1727927030411,796.71069722726,91.6266372665226));
#81372=CARTESIAN_POINT('Ctrl Pts',(103.313673713057,810.364320218198,96.501205407115));
#81373=CARTESIAN_POINT('Ctrl Pts',(66.1489386396743,740.125373764374,80.5126288382199));
#81374=CARTESIAN_POINT('Ctrl Pts',(66.1064422722375,754.63438323368,80.5442708118899));
#81375=CARTESIAN_POINT('Ctrl Pts',(66.0639526747054,769.143392683811,80.5759364049731));
#81376=CARTESIAN_POINT('Ctrl Pts',(83.8113135756256,785.189269489409,87.5495985783604));
#81377=CARTESIAN_POINT('Ctrl Pts',(94.9971296631777,797.644930359551,91.5236973515995));
#81378=CARTESIAN_POINT('Ctrl Pts',(102.096510419537,811.466345641466,96.4570241813705));
#81379=CARTESIAN_POINT('Ctrl Pts',(65.798355350613,740.125373764374,80.2639569419803));
#81380=CARTESIAN_POINT('Ctrl Pts',(65.7564762355172,754.847800462054,80.2972763005058));
#81381=CARTESIAN_POINT('Ctrl Pts',(65.7146045120992,769.570227143548,80.330618657416));
#81382=CARTESIAN_POINT('Ctrl Pts',(82.6856346728155,785.808275750055,87.4303886685735));
#81383=CARTESIAN_POINT('Ctrl Pts',(93.8066491824885,798.549951735236,91.4265032086189));
#81384=CARTESIAN_POINT('Ctrl Pts',(100.853286177248,812.543084537451,96.4171341359893));
#81385=CARTESIAN_POINT('Ctrl Pts',(65.4420370904355,740.125373764374,80.0236455003826));
#81386=CARTESIAN_POINT('Ctrl Pts',(65.4008456205139,755.05583895043,80.058610640551));
#81387=CARTESIAN_POINT('Ctrl Pts',(65.3596620695378,769.986304123174,80.0935981819611));
#81388=CARTESIAN_POINT('Ctrl Pts',(81.5673047484096,786.388698405906,87.317718938527));
#81389=CARTESIAN_POINT('Ctrl Pts',(92.60285526926,799.424489574021,91.3348748976876));
#81390=CARTESIAN_POINT('Ctrl Pts',(99.5851660013872,813.592312893813,96.3812770142762));
#81391=CARTESIAN_POINT('Ctrl Pts',(64.3566928319587,740.125373764374,79.3283198378255));
#81392=CARTESIAN_POINT('Ctrl Pts',(64.3177664806126,755.662913290672,79.3681168994633));
#81393=CARTESIAN_POINT('Ctrl Pts',(64.2788493614205,771.200452811937,79.4079346425718));
#81394=CARTESIAN_POINT('Ctrl Pts',(78.241433233292,788.015375488293,86.9985419953978));
#81395=CARTESIAN_POINT('Ctrl Pts',(88.9568353670791,801.952638709294,91.0761228956451));
#81396=CARTESIAN_POINT('Ctrl Pts',(95.7104028289416,816.650595877495,96.2850049043395));
#81397=CARTESIAN_POINT('Ctrl Pts',(63.6112773557153,740.125373764374,78.8989142791022));
#81398=CARTESIAN_POINT('Ctrl Pts',(63.5741306608233,756.044908017652,78.9417920571076));
#81399=CARTESIAN_POINT('Ctrl Pts',(63.5369937154316,771.964442270956,78.9846894656125));
#81400=CARTESIAN_POINT('Ctrl Pts',(76.0642641288587,788.948173418263,86.8103724461283));
#81401=CARTESIAN_POINT('Ctrl Pts',(86.4799712156315,803.510785624701,90.925132135285));
#81402=CARTESIAN_POINT('Ctrl Pts',(93.0333571874941,818.570248419414,96.2358891713181));
#81403=CARTESIAN_POINT('Ctrl Pts',(62.8461837366256,740.125373764374,78.5050597321885));
#81404=CARTESIAN_POINT('Ctrl Pts',(62.8110622877333,756.401768165066,78.5508493584264));
#81405=CARTESIAN_POINT('Ctrl Pts',(62.7759507873526,772.678162570383,78.5966576597357));
#81406=CARTESIAN_POINT('Ctrl Pts',(73.9439429760598,789.735427319849,86.6451094909407));
#81407=CARTESIAN_POINT('Ctrl Pts',(83.9710618745184,804.930943310987,90.7941464415347));
#81408=CARTESIAN_POINT('Ctrl Pts',(90.273868435174,820.35237693673,96.1997070697605));
#81409=CARTESIAN_POINT('Ctrl Pts',(62.0635864691022,740.125373764374,78.1481623259125));
#81410=CARTESIAN_POINT('Ctrl Pts',(62.030711867897,756.731080653197,78.1966666287248));
#81411=CARTESIAN_POINT('Ctrl Pts',(61.9978471356711,773.336787550785,78.2451887467233));
#81412=CARTESIAN_POINT('Ctrl Pts',(71.9014530756279,790.382188332322,86.5009126672756));
#81413=CARTESIAN_POINT('Ctrl Pts',(81.4484602921453,806.201350089842,90.6815283295111));
#81414=CARTESIAN_POINT('Ctrl Pts',(87.4475775756694,821.977601894745,96.1741945803691));
#81415=CARTESIAN_POINT('Ctrl Pts',(60.8666968367854,740.125373764374,77.6703611206971));
#81416=CARTESIAN_POINT('Ctrl Pts',(60.8374889278549,757.180108276895,77.7225992255993));
#81417=CARTESIAN_POINT('Ctrl Pts',(60.8082904104759,774.2348428037,77.7748539991746));
#81418=CARTESIAN_POINT('Ctrl Pts',(68.9534649735206,791.183049009015,86.3122526659036));
#81419=CARTESIAN_POINT('Ctrl Pts',(77.6390738981942,807.898573162258,90.5364930374217));
#81420=CARTESIAN_POINT('Ctrl Pts',(83.0989245500585,824.184896473511,96.1473309662659));
#81421=CARTESIAN_POINT('Ctrl Pts',(60.4639013375078,740.125373764374,77.5206848696584));
#81422=CARTESIAN_POINT('Ctrl Pts',(60.4359650627929,757.322293966711,77.574111206462));
#81423=CARTESIAN_POINT('Ctrl Pts',(60.4080379607987,774.519214185056,77.6275538536533));
#81424=CARTESIAN_POINT('Ctrl Pts',(67.9937609712978,791.419007894659,86.2538360757553));
#81425=CARTESIAN_POINT('Ctrl Pts',(76.3668683465713,808.42881848167,90.4919822112373));
#81426=CARTESIAN_POINT('Ctrl Pts',(81.6311707521293,824.882237523391,96.1402772815622));
#81427=CARTESIAN_POINT('Ctrl Pts',(60.0575929071003,740.125373764374,77.3806599983877));
#81428=CARTESIAN_POINT('Ctrl Pts',(60.0309746715761,757.456687836812,77.435214660357));
#81429=CARTESIAN_POINT('Ctrl Pts',(60.0043653352274,774.788001926869,77.4897852983144));
#81430=CARTESIAN_POINT('Ctrl Pts',(67.0520671834915,791.628107124824,86.1997490225217));
#81431=CARTESIAN_POINT('Ctrl Pts',(75.0880088655532,808.924844429388,90.4511382932003));
#81432=CARTESIAN_POINT('Ctrl Pts',(80.1413037501949,825.541048987406,96.1348595437315));
#81433=CARTESIAN_POINT('Ctrl Pts',(59.6480909029385,740.125373764374,77.2503470692863));
#81434=CARTESIAN_POINT('Ctrl Pts',(59.6228341130978,757.582988252235,77.3059666117453));
#81435=CARTESIAN_POINT('Ctrl Pts',(59.5975858991469,775.040602759208,77.3616018196785));
#81436=CARTESIAN_POINT('Ctrl Pts',(66.1262266721434,791.81364749282,86.1498551125073));
#81437=CARTESIAN_POINT('Ctrl Pts',(73.801043158822,809.387093113981,90.4137980666451));
#81438=CARTESIAN_POINT('Ctrl Pts',(78.6282046757473,826.160390864936,96.1308169926819));
#81439=CARTESIAN_POINT('Ctrl Pts',(58.8233384618568,740.125373764374,77.0092662202253));
#81440=CARTESIAN_POINT('Ctrl Pts',(58.8008853794041,757.818798903791,77.066881558431));
#81441=CARTESIAN_POINT('Ctrl Pts',(58.7784401367371,775.51222406508,77.1245119888545));
#81442=CARTESIAN_POINT('Ctrl Pts',(64.307521418656,792.142543642154,86.0581890842577));
#81443=CARTESIAN_POINT('Ctrl Pts',(71.2135777935067,810.243251725114,90.3458068558984));
#81444=CARTESIAN_POINT('Ctrl Pts',(75.5588877370191,827.316586996844,96.1249690366928));
#81445=CARTESIAN_POINT('Ctrl Pts',(58.4080880249371,740.125373764374,76.8984983002657));
#81446=CARTESIAN_POINT('Ctrl Pts',(58.3870772041889,757.928309139926,76.9570445537283));
#81447=CARTESIAN_POINT('Ctrl Pts',(58.3660738104078,775.731244538614,77.0156056366663));
#81448=CARTESIAN_POINT('Ctrl Pts',(63.4143078482157,792.286216796038,86.0164198990661));
#81449=CARTESIAN_POINT('Ctrl Pts',(69.9130781349227,810.637161651653,90.315155871707));
#81450=CARTESIAN_POINT('Ctrl Pts',(74.0026698727384,827.853441251222,96.1231636317532));
#81451=CARTESIAN_POINT('Ctrl Pts',(57.9902827290137,740.125373764374,76.7975634472785));
#81452=CARTESIAN_POINT('Ctrl Pts',(57.9707515794984,758.029122651452,76.8569700954413));
#81453=CARTESIAN_POINT('Ctrl Pts',(57.9512274043388,775.932871562816,76.9163913342226));
#81454=CARTESIAN_POINT('Ctrl Pts',(62.5378525327461,792.410646110844,85.9786120728594));
#81455=CARTESIAN_POINT('Ctrl Pts',(68.6071507501991,810.996510083265,90.2876904383976));
#81456=CARTESIAN_POINT('Ctrl Pts',(72.4265652911377,828.347277468934,96.1222201861425));
#81457=CARTESIAN_POINT('Ctrl Pts',(57.5702419314624,740.125373764374,76.7065222236651));
#81458=CARTESIAN_POINT('Ctrl Pts',(57.5522248642258,758.120937803404,76.7667152080309));
#81459=CARTESIAN_POINT('Ctrl Pts',(57.534214283915,776.116501867756,76.8269225680443));
#81460=CARTESIAN_POINT('Ctrl Pts',(61.6815662170187,792.516528443811,85.9446672820555));
#81461=CARTESIAN_POINT('Ctrl Pts',(67.2999264352273,811.320070679581,90.2632556320363));
#81462=CARTESIAN_POINT('Ctrl Pts',(70.8350382159185,828.795487200422,96.1218862325003));
#81463=CARTESIAN_POINT('Ctrl Pts',(56.3043711060502,740.125373764374,76.4632611281508));
#81464=CARTESIAN_POINT('Ctrl Pts',(56.2909905233413,758.368483275649,76.5255803318131));
#81465=CARTESIAN_POINT('Ctrl Pts',(56.2776148757333,776.611592815006,76.5879133378671));
#81466=CARTESIAN_POINT('Ctrl Pts',(59.1918211416932,792.778122395503,85.8541394842021));
#81467=CARTESIAN_POINT('Ctrl Pts',(63.3951297255563,812.177207268129,90.198590761091));
#81468=CARTESIAN_POINT('Ctrl Pts',(66.0359568188235,829.992908914138,96.1219678844952));
#81469=CARTESIAN_POINT('Ctrl Pts',(55.4527926454315,740.125373764374,76.3409038315759));
#81470=CARTESIAN_POINT('Ctrl Pts',(55.4426287026627,758.496313612328,76.4043301290191));
#81471=CARTESIAN_POINT('Ctrl Pts',(55.4324685410653,776.867253489743,76.4677699422263));
#81472=CARTESIAN_POINT('Ctrl Pts',(57.5776163014075,792.896237715016,85.8093161318793));
#81473=CARTESIAN_POINT('Ctrl Pts',(60.7859907751168,812.60335257697,90.1671799470646));
#81474=CARTESIAN_POINT('Ctrl Pts',(62.8039023255101,830.594913415615,96.1234670030539));
#81475=CARTESIAN_POINT('Ctrl Pts',(54.5961044668057,740.125373764374,76.2588478013141));
#81476=CARTESIAN_POINT('Ctrl Pts',(54.5892588263739,758.584530891138,76.3230425032652));
#81477=CARTESIAN_POINT('Ctrl Pts',(54.5824157335954,777.043688048284,76.3872505298953));
#81478=CARTESIAN_POINT('Ctrl Pts',(56.0185052693372,792.968126815447,85.7796391878122));
#81479=CARTESIAN_POINT('Ctrl Pts',(58.1928767330255,812.887876650848,90.1467431470515));
#81480=CARTESIAN_POINT('Ctrl Pts',(59.5658196544964,831.000797356562,96.1253259192129));
#81481=CARTESIAN_POINT('Ctrl Pts',(53.7368614291764,740.125373764374,76.2175775365774));
#81482=CARTESIAN_POINT('Ctrl Pts',(53.7334117656202,758.630722032363,76.2821736502402));
#81483=CARTESIAN_POINT('Ctrl Pts',(53.7299633764019,777.136070331194,76.3467829930399));
#81484=CARTESIAN_POINT('Ctrl Pts',(54.4988708269895,793.001912967943,85.7649011332908));
#81485=CARTESIAN_POINT('Ctrl Pts',(55.6126678348459,813.032506180276,90.1367298610748));
#81486=CARTESIAN_POINT('Ctrl Pts',(56.3232617065557,831.208785659394,96.126634332624));
#81487=CARTESIAN_POINT('Ctrl Pts',(52.0183753539178,740.125373764373,76.2175775365774));
#81488=CARTESIAN_POINT('Ctrl Pts',(52.0218250174741,758.634225880209,76.2821858810255));
#81489=CARTESIAN_POINT('Ctrl Pts',(52.0252734087246,777.143078026885,76.3468074546121));
#81490=CARTESIAN_POINT('Ctrl Pts',(51.4571490512008,793.00566360327,85.7652369378129));
#81491=CARTESIAN_POINT('Ctrl Pts',(50.4216491638841,813.041567215157,90.1367984891347));
#81492=CARTESIAN_POINT('Ctrl Pts',(49.782129424813,831.22155851757,96.126678725148));
#81493=CARTESIAN_POINT('Ctrl Pts',(51.1591323162885,740.125373764374,76.2588478013141));
#81494=CARTESIAN_POINT('Ctrl Pts',(51.1659789780672,758.5910875414,76.3230649827209));
#81495=CARTESIAN_POINT('Ctrl Pts',(51.1728230942121,777.056801348808,76.3872954888097));
#81496=CARTESIAN_POINT('Ctrl Pts',(49.8704945841611,792.973408011051,85.7797762908131));
#81497=CARTESIAN_POINT('Ctrl Pts',(47.7800644164022,812.905202797824,90.1466343865574));
#81498=CARTESIAN_POINT('Ctrl Pts',(46.4835550910109,831.026343072914,96.1254147042609));
#81499=CARTESIAN_POINT('Ctrl Pts',(50.3024441376628,740.125373764374,76.3409038315759));
#81500=CARTESIAN_POINT('Ctrl Pts',(50.3126108891353,758.505475285689,76.404360988347));
#81501=CARTESIAN_POINT('Ctrl Pts',(50.3227738614307,776.885576836465,76.4678316608864));
#81502=CARTESIAN_POINT('Ctrl Pts',(48.2415589467887,792.894397192007,85.8089306098157));
#81503=CARTESIAN_POINT('Ctrl Pts',(45.1221815361918,812.620221612385,90.1667651019422));
#81504=CARTESIAN_POINT('Ctrl Pts',(43.1856486711625,830.624454929622,96.1236765570555));
#81505=CARTESIAN_POINT('Ctrl Pts',(49.450865677044,740.125373764374,76.4632611281508));
#81506=CARTESIAN_POINT('Ctrl Pts',(49.464251366487,758.379805458904,76.5256178155316));
#81507=CARTESIAN_POINT('Ctrl Pts',(49.4776321227852,776.634237181515,76.5879883053097));
#81508=CARTESIAN_POINT('Ctrl Pts',(46.6096800057099,792.777563498267,85.8527801984682));
#81509=CARTESIAN_POINT('Ctrl Pts',(42.4936032603387,812.200458494583,90.1975206582424));
#81510=CARTESIAN_POINT('Ctrl Pts',(39.9329117299652,830.032379931876,96.122113162747));
#81511=CARTESIAN_POINT('Ctrl Pts',(48.1849948516318,740.125373764374,76.706522223665));
#81512=CARTESIAN_POINT('Ctrl Pts',(48.2030208556531,758.134838880861,76.7667601650879));
#81513=CARTESIAN_POINT('Ctrl Pts',(48.2210403746284,776.14430402267,76.8270124821659));
#81514=CARTESIAN_POINT('Ctrl Pts',(44.1793258575781,792.534315599669,85.9415459155213));
#81515=CARTESIAN_POINT('Ctrl Pts',(38.6259692778301,811.364731598803,90.2609142626241));
#81516=CARTESIAN_POINT('Ctrl Pts',(35.1511853022989,828.859054345708,96.1218314935801));
#81517=CARTESIAN_POINT('Ctrl Pts',(47.7649540540804,740.125373764374,76.7975634472784));
#81518=CARTESIAN_POINT('Ctrl Pts',(47.7844954808982,758.043773048535,76.8570171330699));
#81519=CARTESIAN_POINT('Ctrl Pts',(47.8040299352114,775.962172356984,76.9164854094881));
#81520=CARTESIAN_POINT('Ctrl Pts',(43.3440936170016,792.434158289661,85.9750736900068));
#81521=CARTESIAN_POINT('Ctrl Pts',(37.3360276518998,811.04929213267,90.2849869594039));
#81522=CARTESIAN_POINT('Ctrl Pts',(33.5735063237651,828.420410302061,96.1220815075737));
#81523=CARTESIAN_POINT('Ctrl Pts',(47.3471487581571,740.125373764374,76.8984983002657));
#81524=CARTESIAN_POINT('Ctrl Pts',(47.3681712286424,757.943598953128,76.957093275552));
#81525=CARTESIAN_POINT('Ctrl Pts',(47.3891862739802,775.761824165019,77.0157030803224));
#81526=CARTESIAN_POINT('Ctrl Pts',(42.4812723007942,792.314724749067,86.0125874141734));
#81527=CARTESIAN_POINT('Ctrl Pts',(36.0421742699118,810.6977140878,90.3121448688152));
#81528=CARTESIAN_POINT('Ctrl Pts',(32.0080856465946,827.935994030087,96.122920038645));
#81529=CARTESIAN_POINT('Ctrl Pts',(46.9318983212373,740.125373764374,77.0092662202253));
#81530=CARTESIAN_POINT('Ctrl Pts',(46.954364425862,757.834618637866,77.0669315822377));
#81531=CARTESIAN_POINT('Ctrl Pts',(46.9768226924855,775.543863533231,77.124612036477));
#81532=CARTESIAN_POINT('Ctrl Pts',(41.5917117805538,792.174400912347,86.0541498402097));
#81533=CARTESIAN_POINT('Ctrl Pts',(34.7445524302651,810.309310207566,90.3425477128121));
#81534=CARTESIAN_POINT('Ctrl Pts',(30.4542764974918,827.40615630429,96.1246077047976));
#81535=CARTESIAN_POINT('Ctrl Pts',(46.1071458801556,740.125373764374,77.2503470692862));
#81536=CARTESIAN_POINT('Ctrl Pts',(46.1324183732037,757.599649654093,77.3060185034231));
#81537=CARTESIAN_POINT('Ctrl Pts',(46.1576822920703,775.073925562926,77.361705603044));
#81538=CARTESIAN_POINT('Ctrl Pts',(39.7649974382762,791.849864134419,86.1455125141571));
#81539=CARTESIAN_POINT('Ctrl Pts',(32.146243795526,809.458595881956,90.4101776276437));
#81540=CARTESIAN_POINT('Ctrl Pts',(27.3727730719043,826.257459112895,96.1302174570309));
#81541=CARTESIAN_POINT('Ctrl Pts',(45.6976438759937,740.125373764374,77.3806599983876));
#81542=CARTESIAN_POINT('Ctrl Pts',(45.724279123326,757.473660985582,77.4352671179228));
#81543=CARTESIAN_POINT('Ctrl Pts',(45.7509054731498,774.821948224408,77.4898902134563));
#81544=CARTESIAN_POINT('Ctrl Pts',(38.8267914620367,791.663318494346,86.1953136093372));
#81545=CARTESIAN_POINT('Ctrl Pts',(30.8455570004336,808.99628543658,90.4474046984785));
#81546=CARTESIAN_POINT('Ctrl Pts',(25.8450787954196,825.638599647297,96.1341395431115));
#81547=CARTESIAN_POINT('Ctrl Pts',(45.2913354455863,740.125373764374,77.5206848696584));
#81548=CARTESIAN_POINT('Ctrl Pts',(45.3192899768756,757.339470183674,77.574163876033));
#81549=CARTESIAN_POINT('Ctrl Pts',(45.347235337067,774.553566618983,77.627659192806));
#81550=CARTESIAN_POINT('Ctrl Pts',(37.8665259645302,791.450598279842,86.2493786341431));
#81551=CARTESIAN_POINT('Ctrl Pts',(29.5455737075545,808.496894261427,90.4882110615655));
#81552=CARTESIAN_POINT('Ctrl Pts',(24.3318878634854,824.976139895723,96.139446914039));
#81553=CARTESIAN_POINT('Ctrl Pts',(44.8885399463087,740.125373764374,77.6703611206971));
#81554=CARTESIAN_POINT('Ctrl Pts',(44.9177672608288,757.197379291599,77.7226517674573));
#81555=CARTESIAN_POINT('Ctrl Pts',(44.9469851853724,774.269384833108,77.7749590829014));
#81556=CARTESIAN_POINT('Ctrl Pts',(36.8890829111274,791.210365977003,86.3078592168729));
#81557=CARTESIAN_POINT('Ctrl Pts',(28.2506225783616,807.960854718712,90.5327713526171));
#81558=CARTESIAN_POINT('Ctrl Pts',(22.8367388658799,824.271550251516,96.146415101575));
#81559=CARTESIAN_POINT('Ctrl Pts',(43.6916503139919,740.125373764374,78.1481623259125));
#81560=CARTESIAN_POINT('Ctrl Pts',(43.7245473848271,756.748312474556,78.1967178107824));
#81561=CARTESIAN_POINT('Ctrl Pts',(43.7574345881057,773.371251193502,78.2452911108501));
#81562=CARTESIAN_POINT('Ctrl Pts',(33.9224488004764,790.410716654602,86.4969992510776));
#81563=CARTESIAN_POINT('Ctrl Pts',(24.3964334873945,806.251684467338,90.6782346441511));
#81564=CARTESIAN_POINT('Ctrl Pts',(18.4186152665191,822.043399213847,96.1731254366424));
#81565=CARTESIAN_POINT('Ctrl Pts',(42.9090530464685,740.125373764375,78.5050597321886));
#81566=CARTESIAN_POINT('Ctrl Pts',(42.9441984970111,756.418542408771,78.5508983317358));
#81567=CARTESIAN_POINT('Ctrl Pts',(42.9793340003503,772.711711057793,78.596755606366));
#81568=CARTESIAN_POINT('Ctrl Pts',(31.8698675756471,789.759693991976,86.6416659528865));
#81569=CARTESIAN_POINT('Ctrl Pts',(21.8539209894605,804.971856467956,90.7911736909535));
#81570=CARTESIAN_POINT('Ctrl Pts',(15.5629640582194,820.40545571534,96.1986733566335));
#81571=CARTESIAN_POINT('Ctrl Pts',(42.1439594273788,740.125373764375,78.8989142791023));
#81572=CARTESIAN_POINT('Ctrl Pts',(42.1811308899313,756.060796501059,78.9418376327706));
#81573=CARTESIAN_POINT('Ctrl Pts',(42.2182926041646,771.99621923777,78.9847806169498));
#81574=CARTESIAN_POINT('Ctrl Pts',(29.7482325355677,788.975322800262,86.8070049453425));
#81575=CARTESIAN_POINT('Ctrl Pts',(19.3392894961986,803.552080430039,90.922021074782));
#81576=CARTESIAN_POINT('Ctrl Pts',(12.7933854819489,818.622207535651,96.2344984406095));
#81577=CARTESIAN_POINT('Ctrl Pts',(41.3985439511354,740.125373764375,79.3283198378255));
#81578=CARTESIAN_POINT('Ctrl Pts',(41.4374948148052,755.67749109725,79.3681580018985));
#81579=CARTESIAN_POINT('Ctrl Pts',(41.4764364473626,771.229608425092,79.4080168474528));
#81580=CARTESIAN_POINT('Ctrl Pts',(27.5697855394546,788.045868489416,86.9951801697774));
#81581=CARTESIAN_POINT('Ctrl Pts',(16.8599436396416,801.99648030487,91.0727866099062));
#81582=CARTESIAN_POINT('Ctrl Pts',(10.1126581685345,816.704550291679,96.2832018189664));
#81583=CARTESIAN_POINT('Ctrl Pts',(39.9514182731664,740.125373764374,80.255420721235));
#81584=CARTESIAN_POINT('Ctrl Pts',(39.9933862308964,754.864593989093,80.2888054523636));
#81585=CARTESIAN_POINT('Ctrl Pts',(40.0353467081538,769.603814197741,80.3222131579999));
#81586=CARTESIAN_POINT('Ctrl Pts',(23.126009607612,785.876577822194,87.421096066829));
#81587=CARTESIAN_POINT('Ctrl Pts',(11.9888907180205,798.625133155414,91.4177387128464));
#81588=CARTESIAN_POINT('Ctrl Pts',(4.93672158308855,812.625462281788,96.4111325267945));
#81589=CARTESIAN_POINT('Ctrl Pts',(39.2497080714407,740.125373764374,80.7531160459211));
#81590=CARTESIAN_POINT('Ctrl Pts',(39.2929137221135,754.435002284747,80.7831325337009));
#81591=CARTESIAN_POINT('Ctrl Pts',(39.3361131257469,768.74463078307,80.8131732380438));
#81592=CARTESIAN_POINT('Ctrl Pts',(20.8607795467825,784.637676843055,87.6588066532497));
#81593=CARTESIAN_POINT('Ctrl Pts',(9.5971836529565,796.809386131128,91.6119252806624));
#81594=CARTESIAN_POINT('Ctrl Pts',(2.44151231105709,810.46403151587,96.4903598562657));
#81595=CARTESIAN_POINT('Ctrl Pts',(38.5720250013864,740.125373764374,81.2835501247607));
#81596=CARTESIAN_POINT('Ctrl Pts',(38.6161732477199,753.984683775961,81.3100852591544));
#81597=CARTESIAN_POINT('Ctrl Pts',(38.6603168783517,767.84399375906,81.3366459477096));
#81598=CARTESIAN_POINT('Ctrl Pts',(18.5683916561005,783.235903460189,87.9242593021168));
#81599=CARTESIAN_POINT('Ctrl Pts',(7.25782974268059,794.869316294976,91.8296147298744));
#81600=CARTESIAN_POINT('Ctrl Pts',(0.0429698175526117,808.193236292288,
96.5872328424701));
#81601=CARTESIAN_POINT('Ctrl Pts',(37.9205435574161,740.125373764374,81.8453168289255));
#81602=CARTESIAN_POINT('Ctrl Pts',(37.9653150589334,753.516054808566,81.8682859167358));
#81603=CARTESIAN_POINT('Ctrl Pts',(38.010084013782,766.906735817371,81.8912819918484));
#81604=CARTESIAN_POINT('Ctrl Pts',(16.2661593276306,781.664267601813,88.2202259887619));
#81605=CARTESIAN_POINT('Ctrl Pts',(4.98049187324324,792.812300971065,92.0723819763127));
#81606=CARTESIAN_POINT('Ctrl Pts',(-2.25386901258056,805.827225600765,96.7039177173643));
#81607=CARTESIAN_POINT('Ctrl Pts',(37.2974382339422,740.125373764374,82.4370100295875));
#81608=CARTESIAN_POINT('Ctrl Pts',(37.3424894069716,753.031531728391,82.4563567944567));
#81609=CARTESIAN_POINT('Ctrl Pts',(37.3875405798517,765.937689649662,82.4757320753115));
#81610=CARTESIAN_POINT('Ctrl Pts',(13.9671836840501,779.915341744281,88.5489787937201));
#81611=CARTESIAN_POINT('Ctrl Pts',(2.77062066130783,790.64528003164,92.3413020410112));
#81612=CARTESIAN_POINT('Ctrl Pts',(-4.44817956388518,803.379710979161,96.8420808181083));
#81613=CARTESIAN_POINT('',(-2.3072174972792,802.626345096273,96.1096278308841));
#81614=CARTESIAN_POINT('Ctrl Pts',(-2.30689020010939,802.626560388343,96.1095808375407));
#81615=CARTESIAN_POINT('Ctrl Pts',(-2.68639626067645,803.251812836745,96.330577960684));
#81616=CARTESIAN_POINT('Ctrl Pts',(-3.05421750819845,803.883231163271,96.5538081011059));
#81617=CARTESIAN_POINT('Ctrl Pts',(-3.40944118612444,804.520983132338,96.7791293074463));
#81618=CARTESIAN_POINT('',(108.062487312194,802.626301820665,96.1096219232672));
#81619=CARTESIAN_POINT('Ctrl Pts',(109.164772626437,804.521007661288,96.7791165021265));
#81620=CARTESIAN_POINT('Ctrl Pts',(108.987923875025,804.201654960381,96.666601644594));
#81621=CARTESIAN_POINT('Ctrl Pts',(108.807152759608,803.884339316512,96.5544638713983));
#81622=CARTESIAN_POINT('Ctrl Pts',(108.623155796259,803.568713813167,96.4428324932515));
#81623=CARTESIAN_POINT('Ctrl Pts',(108.439158832909,803.253088309821,96.3312011151047));
#81624=CARTESIAN_POINT('Ctrl Pts',(108.252007023091,802.939107479159,96.2200864522011));
#81625=CARTESIAN_POINT('Ctrl Pts',(108.062323461338,802.626409591658,96.1095984083762));
#81626=CARTESIAN_POINT('',(67.774347942193,740.125373764374,81.8141824275666));
#81627=CARTESIAN_POINT('Ctrl Pts',(108.062487312194,802.626301820665,96.1096219232672));
#81628=CARTESIAN_POINT('Ctrl Pts',(107.640412981026,801.930681948247,95.8638046150634));
#81629=CARTESIAN_POINT('Ctrl Pts',(107.203256492765,801.24328772892,95.620741919965));
#81630=CARTESIAN_POINT('Ctrl Pts',(106.75236567008,800.565958331003,95.3807586268188));
#81631=CARTESIAN_POINT('Ctrl Pts',(106.325982702208,799.925444698033,95.1538194574609));
#81632=CARTESIAN_POINT('Ctrl Pts',(105.8873187214,799.293931975707,94.9296340745444));
#81633=CARTESIAN_POINT('Ctrl Pts',(105.437552836549,798.67295949173,94.7084711043448));
#81634=CARTESIAN_POINT('Ctrl Pts',(105.42652693745,798.657736505321,94.7030493489913));
#81635=CARTESIAN_POINT('Ctrl Pts',(105.415494274884,798.642519698899,94.697629359652));
#81636=CARTESIAN_POINT('Ctrl Pts',(105.404454864429,798.627309092915,94.6922111394988));
#81637=CARTESIAN_POINT('Ctrl Pts',(104.79826132232,797.79206783104,94.394687093275));
#81638=CARTESIAN_POINT('Ctrl Pts',(104.171417072003,796.974168319304,94.1020990225107));
#81639=CARTESIAN_POINT('Ctrl Pts',(103.526885548805,796.171143140921,93.8138832266392));
#81640=CARTESIAN_POINT('Ctrl Pts',(103.198040541494,795.761433435264,93.6668332809201));
#81641=CARTESIAN_POINT('Ctrl Pts',(102.864592019392,795.35559515563,93.5209213547615));
#81642=CARTESIAN_POINT('Ctrl Pts',(102.52693755488,794.953297460646,93.37607176917));
#81643=CARTESIAN_POINT('Ctrl Pts',(102.504551389322,794.926625511211,93.3664683812544));
#81644=CARTESIAN_POINT('Ctrl Pts',(102.482146735223,794.899969102788,93.3568696590447));
#81645=CARTESIAN_POINT('Ctrl Pts',(102.4597237084,794.873328137208,93.3472755801077));
#81646=CARTESIAN_POINT('Ctrl Pts',(101.728050389849,794.004021604738,93.0342165257061));
#81647=CARTESIAN_POINT('Ctrl Pts',(100.977128069926,793.150865667694,92.7260164575441));
#81648=CARTESIAN_POINT('Ctrl Pts',(100.211177215851,792.310090537155,92.4222827468567));
#81649=CARTESIAN_POINT('Ctrl Pts',(99.380591387708,791.398366365341,92.0929183832238));
#81650=CARTESIAN_POINT('Ctrl Pts',(98.5323338124084,790.501200490887,91.7688059920466));
#81651=CARTESIAN_POINT('Ctrl Pts',(97.6718328280343,789.613743392316,91.4494366429952));
#81652=CARTESIAN_POINT('Ctrl Pts',(97.152518953693,789.07816145512,91.2566966728924));
#81653=CARTESIAN_POINT('Ctrl Pts',(96.6287467376884,788.546114787712,91.0656840262139));
#81654=CARTESIAN_POINT('Ctrl Pts',(96.1017159269538,788.016531543047,90.8762855451684));
#81655=CARTESIAN_POINT('Ctrl Pts',(96.0590994158765,787.973708638289,90.8609704965961));
#81656=CARTESIAN_POINT('Ctrl Pts',(96.0164615787842,787.930901903599,90.8456660040061));
#81657=CARTESIAN_POINT('Ctrl Pts',(95.9738030426657,787.888110760593,90.830372003895));
#81658=CARTESIAN_POINT('Ctrl Pts',(94.8209136774377,786.73163756233,90.4170364400377));
#81659=CARTESIAN_POINT('Ctrl Pts',(93.6527406381072,785.58666301832,90.0114150472833));
#81660=CARTESIAN_POINT('Ctrl Pts',(92.4789028667217,784.444304507527,89.6134588224494));
#81661=CARTESIAN_POINT('Ctrl Pts',(91.4230801131926,783.416796160305,89.2555122242647));
#81662=CARTESIAN_POINT('Ctrl Pts',(90.3626752475194,782.39140318791,88.903766858798));
#81663=CARTESIAN_POINT('Ctrl Pts',(89.3047136290314,781.361636814038,88.5581860807789));
#81664=CARTESIAN_POINT('Ctrl Pts',(89.2467119251352,781.305180886662,88.5392399549379));
#81665=CARTESIAN_POINT('Ctrl Pts',(89.1887176192233,781.248711946809,88.5203123802324));
#81666=CARTESIAN_POINT('Ctrl Pts',(89.1307318277863,781.192228889795,88.5014033367873));
#81667=CARTESIAN_POINT('Ctrl Pts',(88.0211876752418,780.111439198484,88.139583344944));
#81668=CARTESIAN_POINT('Ctrl Pts',(86.9143542908349,779.025811538966,87.7845303670263));
#81669=CARTESIAN_POINT('Ctrl Pts',(85.8179698161622,777.927924518351,87.4370122370397));
#81670=CARTESIAN_POINT('Ctrl Pts',(84.9020308283374,777.010730277063,87.1466894428158));
#81671=CARTESIAN_POINT('Ctrl Pts',(83.9933842451906,776.084980050413,86.8616255566873));
#81672=CARTESIAN_POINT('Ctrl Pts',(83.0965727816879,775.146316117423,86.582276091458));
#81673=CARTESIAN_POINT('Ctrl Pts',(82.9198955321183,774.961393679764,86.5272425674744));
#81674=CARTESIAN_POINT('Ctrl Pts',(82.7436777330877,774.775969931733,86.4724308521597));
#81675=CARTESIAN_POINT('Ctrl Pts',(82.5679542960686,774.590011378811,86.4178444648264));
#81676=CARTESIAN_POINT('Ctrl Pts',(82.5012260278146,774.519396482961,86.3971161251195));
#81677=CARTESIAN_POINT('Ctrl Pts',(82.4345687142384,774.448703746333,86.3764201674801));
#81678=CARTESIAN_POINT('Ctrl Pts',(82.3679844602655,774.377931547985,86.3557568467796));
#81679=CARTESIAN_POINT('Ctrl Pts',(81.4237317729819,773.374288276671,86.0627236604705));
#81680=CARTESIAN_POINT('Ctrl Pts',(80.4945540723926,772.354776636511,85.7764377798638));
#81681=CARTESIAN_POINT('Ctrl Pts',(79.5903226433914,771.317053989318,85.4989930367865));
#81682=CARTESIAN_POINT('Ctrl Pts',(79.5114235124355,771.226507020465,85.4747844675917));
#81683=CARTESIAN_POINT('Ctrl Pts',(79.4327142911312,771.135821426451,85.4506431946544));
#81684=CARTESIAN_POINT('Ctrl Pts',(79.3542015223261,771.044995666001,85.4265705989427));
#81685=CARTESIAN_POINT('Ctrl Pts',(79.2872510851058,770.967545533169,85.406043099627));
#81686=CARTESIAN_POINT('Ctrl Pts',(79.220441547077,770.88999082999,85.3855649455497));
#81687=CARTESIAN_POINT('Ctrl Pts',(79.1537766614075,770.812330210894,85.3651369027868));
#81688=CARTESIAN_POINT('Ctrl Pts',(78.5551663921203,770.114984919695,85.1817054597342));
#81689=CARTESIAN_POINT('Ctrl Pts',(77.9679052424419,769.408810509424,85.0022174634512));
#81690=CARTESIAN_POINT('Ctrl Pts',(77.3946133745915,768.69196912988,84.8272162256116));
#81691=CARTESIAN_POINT('Ctrl Pts',(77.0383014961175,768.246438479898,84.7184496037794));
#81692=CARTESIAN_POINT('Ctrl Pts',(76.687386434515,767.796786822786,84.611416309622));
#81693=CARTESIAN_POINT('Ctrl Pts',(76.3425054304563,767.342566840531,84.5062485763837));
#81694=CARTESIAN_POINT('Ctrl Pts',(76.2787833852224,767.25864274522,84.48681722767));
#81695=CARTESIAN_POINT('Ctrl Pts',(76.2152675101717,767.174562113752,84.467449653553));
#81696=CARTESIAN_POINT('Ctrl Pts',(76.1519616252091,767.090321815678,84.4481466294127));
#81697=CARTESIAN_POINT('Ctrl Pts',(75.705965492299,766.49684070096,84.3121549419864));
#81698=CARTESIAN_POINT('Ctrl Pts',(75.2703804789971,765.89544498154,84.1793611878219));
#81699=CARTESIAN_POINT('Ctrl Pts',(74.8469145710805,765.284861908932,84.0501684628422));
#81700=CARTESIAN_POINT('Ctrl Pts',(74.4554953372686,764.720485995804,83.9307526693148));
#81701=CARTESIAN_POINT('Ctrl Pts',(74.0744302930709,764.148260661885,83.8144134988996));
#81702=CARTESIAN_POINT('Ctrl Pts',(73.7051075794581,763.56715370259,83.7014789981592));
#81703=CARTESIAN_POINT('Ctrl Pts',(73.6748700141567,763.51957672186,83.6922327097099));
#81704=CARTESIAN_POINT('Ctrl Pts',(73.6447111835826,763.471940189732,83.6830092491982));
#81705=CARTESIAN_POINT('Ctrl Pts',(73.6146318625107,763.424243530879,83.6738087998238));
#81706=CARTESIAN_POINT('Ctrl Pts',(73.5590966011547,763.336181489556,83.6568220679962));
#81707=CARTESIAN_POINT('Ctrl Pts',(73.5038324872464,763.247913812902,83.6399138783004));
#81708=CARTESIAN_POINT('Ctrl Pts',(73.4488444080641,763.159436842759,83.6230853925887));
#81709=CARTESIAN_POINT('Ctrl Pts',(73.1132302252477,762.619426599187,83.520374431156));
#81710=CARTESIAN_POINT('Ctrl Pts',(72.7879129157079,762.071637465489,83.4206318480089));
#81711=CARTESIAN_POINT('Ctrl Pts',(72.474219014269,761.515064802767,83.3242202553888));
#81712=CARTESIAN_POINT('Ctrl Pts',(72.1726286046254,760.979966808905,83.2315285850079));
#81713=CARTESIAN_POINT('Ctrl Pts',(71.8817818330543,760.436750090596,83.1419157855282));
#81714=CARTESIAN_POINT('Ctrl Pts',(71.6028966763131,759.884495600035,83.0557144828276));
#81715=CARTESIAN_POINT('Ctrl Pts',(71.4907939020061,759.662507233072,83.0210643591189));
#81716=CARTESIAN_POINT('Ctrl Pts',(71.3806243244004,759.439058250873,82.9869655811785));
#81717=CARTESIAN_POINT('Ctrl Pts',(71.2724690060563,759.214087653493,82.9534402731627));
#81718=CARTESIAN_POINT('Ctrl Pts',(71.2313548746967,759.128567395828,82.9406959722931));
#81719=CARTESIAN_POINT('Ctrl Pts',(71.1905294946928,759.042821726578,82.9280338870646));
#81720=CARTESIAN_POINT('Ctrl Pts',(71.1499985653014,758.956849457591,82.9154556285894));
#81721=CARTESIAN_POINT('Ctrl Pts',(70.9502324773323,758.533115185837,82.8534607637595));
#81722=CARTESIAN_POINT('Ctrl Pts',(70.7572982590349,758.102842316802,82.7934040808962));
#81723=CARTESIAN_POINT('Ctrl Pts',(70.5729745362041,757.668912681433,82.7358431182547));
#81724=CARTESIAN_POINT('Ctrl Pts',(70.4749971365992,757.438257090107,82.7052465496105));
#81725=CARTESIAN_POINT('Ctrl Pts',(70.3794524660278,757.20656932707,82.6753551137604));
#81726=CARTESIAN_POINT('Ctrl Pts',(70.2866057688366,756.974287643936,82.6462520783323));
#81727=CARTESIAN_POINT('Ctrl Pts',(70.2549725135742,756.895148309984,82.6363365533168));
#81728=CARTESIAN_POINT('Ctrl Pts',(70.2236466597481,756.815928101304,82.6265104736713));
#81729=CARTESIAN_POINT('Ctrl Pts',(70.1926389310556,756.736643983384,82.6167772222424));
#81730=CARTESIAN_POINT('Ctrl Pts',(70.0008322429551,756.246210639236,82.5565695643541));
#81731=CARTESIAN_POINT('Ctrl Pts',(69.8207380469322,755.752537000797,82.4997730334338));
#81732=CARTESIAN_POINT('Ctrl Pts',(69.6526436142649,755.25574335944,82.4465134247772));
#81733=CARTESIAN_POINT('Ctrl Pts',(69.5876584443764,755.063683344895,82.4259233037255));
#81734=CARTESIAN_POINT('Ctrl Pts',(69.5244662353335,754.871157182456,82.4058616953423));
#81735=CARTESIAN_POINT('Ctrl Pts',(69.4630816345515,754.678172457831,82.3863354291315));
#81736=CARTESIAN_POINT('Ctrl Pts',(69.4414146562721,754.610054464336,82.3794432252159));
#81737=CARTESIAN_POINT('Ctrl Pts',(69.4199715886117,754.541876553508,82.3726171766097));
#81738=CARTESIAN_POINT('Ctrl Pts',(69.3987530496711,754.473639090163,82.3658575497437));
#81739=CARTESIAN_POINT('Ctrl Pts',(69.2456839785206,753.981378753056,82.31709406944));
#81740=CARTESIAN_POINT('Ctrl Pts',(69.1044146638885,753.486041628445,82.2718223599259));
#81741=CARTESIAN_POINT('Ctrl Pts',(68.9747603029794,752.987670002935,82.2300252477364));
#81742=CARTESIAN_POINT('Ctrl Pts',(68.8429790834064,752.481123056502,82.1875424929695));
#81743=CARTESIAN_POINT('Ctrl Pts',(68.7231969358553,751.971441077823,82.1486492709651));
#81744=CARTESIAN_POINT('Ctrl Pts',(68.6151684215416,751.458678722048,82.1133126209994));
#81745=CARTESIAN_POINT('Ctrl Pts',(68.5098860997668,750.958951296583,82.0788742639066));
#81746=CARTESIAN_POINT('Ctrl Pts',(68.4157670280329,750.456298046548,82.0478138616348));
#81747=CARTESIAN_POINT('Ctrl Pts',(68.3325396635622,749.950780797533,82.020087648334));
#81748=CARTESIAN_POINT('Ctrl Pts',(68.3261422655682,749.911923445082,82.0179564307653));
#81749=CARTESIAN_POINT('Ctrl Pts',(68.3198091607959,749.873049471991,82.0158448547));
#81750=CARTESIAN_POINT('Ctrl Pts',(68.3135402277496,749.834158963291,82.0137529034267));
#81751=CARTESIAN_POINT('Ctrl Pts',(68.2338355712915,749.339696091785,81.9871553538386));
#81752=CARTESIAN_POINT('Ctrl Pts',(68.1644146011459,748.842528149145,81.9637035184728));
#81753=CARTESIAN_POINT('Ctrl Pts',(68.104550932947,748.34284804846,81.9432166527108));
#81754=CARTESIAN_POINT('Ctrl Pts',(68.0718651149346,748.070020583542,81.9320307366772));
#81755=CARTESIAN_POINT('Ctrl Pts',(68.0420276545082,747.796444564669,81.9217284836477));
#81756=CARTESIAN_POINT('Ctrl Pts',(68.0149147410762,747.522154173909,81.9122787837859));
#81757=CARTESIAN_POINT('Ctrl Pts',(68.0125303604343,747.498032358317,81.9114477524222));
#81758=CARTESIAN_POINT('Ctrl Pts',(68.0101670378479,747.473905194498,81.9106232965028));
#81759=CARTESIAN_POINT('Ctrl Pts',(68.0078246793461,747.449772635794,81.9098053910308));
#81760=CARTESIAN_POINT('Ctrl Pts',(67.9624381839498,746.982170318031,81.8939573204166));
#81761=CARTESIAN_POINT('Ctrl Pts',(67.9249638118947,746.512338386814,81.8805821287688));
#81762=CARTESIAN_POINT('Ctrl Pts',(67.8943950412482,746.041844248718,81.8693983373665));
#81763=CARTESIAN_POINT('Ctrl Pts',(67.8731624008485,745.715045603139,81.8616302323322));
#81764=CARTESIAN_POINT('Ctrl Pts',(67.8552623904349,745.387926532362,81.8549196791735));
#81765=CARTESIAN_POINT('Ctrl Pts',(67.8403691802505,745.061004150737,81.8491758738642));
#81766=CARTESIAN_POINT('Ctrl Pts',(67.8398151425495,745.048842412437,81.8489622003412));
#81767=CARTESIAN_POINT('Ctrl Pts',(67.839265268583,745.036681055243,81.8487498640869));
#81768=CARTESIAN_POINT('Ctrl Pts',(67.838719541966,745.024520113673,81.8485388605921));
#81769=CARTESIAN_POINT('Ctrl Pts',(67.809929228428,744.382958368549,81.8374071756329));
#81770=CARTESIAN_POINT('Ctrl Pts',(67.7929166955335,743.741046577285,81.830088040421));
#81771=CARTESIAN_POINT('Ctrl Pts',(67.7832106745823,743.098909519817,81.8251575416515));
#81772=CARTESIAN_POINT('Ctrl Pts',(67.775657710959,742.599215787377,81.8213207605402));
#81773=CARTESIAN_POINT('Ctrl Pts',(67.7725283304721,742.099386023544,81.8189301434773));
#81774=CARTESIAN_POINT('Ctrl Pts',(67.7717437536218,741.599490031252,81.8173236497979));
#81775=CARTESIAN_POINT('Ctrl Pts',(67.770972615075,741.10815630284,81.8157446722878));
#81776=CARTESIAN_POINT('Ctrl Pts',(67.7724654094933,740.616758542271,81.8149227882236));
#81777=CARTESIAN_POINT('Ctrl Pts',(67.774294136204,740.125373479123,81.8142439628221));
#81778=CARTESIAN_POINT('',(37.9808888409178,740.125373764374,81.814182427552));
#81779=CARTESIAN_POINT('Ctrl Pts',(67.774347942193,740.125373764374,81.8141824275666));
#81780=CARTESIAN_POINT('Ctrl Pts',(67.5900718265523,740.125373764374,81.6531996590034));
#81781=CARTESIAN_POINT('Ctrl Pts',(67.0763564188786,740.125373764374,81.2162773885272));
#81782=CARTESIAN_POINT('Ctrl Pts',(66.5464115392411,740.125373764374,80.7985912178955));
#81783=CARTESIAN_POINT('Ctrl Pts',(65.3066539796418,740.125373764381,79.8939539311288));
#81784=CARTESIAN_POINT('Ctrl Pts',(63.9938241652593,740.125373764356,79.0958415525578));
#81785=CARTESIAN_POINT('Ctrl Pts',(62.8461837366256,740.125373764374,78.5050597321885));
#81786=CARTESIAN_POINT('Ctrl Pts',(60.4983919340555,740.125373764374,77.4343675133605));
#81787=CARTESIAN_POINT('Ctrl Pts',(58.0126377452945,740.125373764374,76.7089447197242));
#81788=CARTESIAN_POINT('Ctrl Pts',(56.3145905420647,740.125373764374,76.3826585955248));
#81789=CARTESIAN_POINT('Ctrl Pts',(52.8776183915509,740.125373764374,76.052496477614));
#81790=CARTESIAN_POINT('Ctrl Pts',(49.4406462410274,740.125373764373,76.3826585955353));
#81791=CARTESIAN_POINT('Ctrl Pts',(47.742599037804,740.125373764375,76.7089447197054));
#81792=CARTESIAN_POINT('Ctrl Pts',(45.2568448490267,740.125373764369,77.4343675134104));
#81793=CARTESIAN_POINT('Ctrl Pts',(42.2948993868004,740.125373764376,78.785139739208));
#81794=CARTESIAN_POINT('Ctrl Pts',(40.9539042355239,740.125373764374,79.5398396982121));
#81795=CARTESIAN_POINT('Ctrl Pts',(39.6810271869632,740.125373764374,80.4042681496218));
#81796=CARTESIAN_POINT('Ctrl Pts',(38.4886305678844,740.125373764374,81.3704310402807));
#81797=CARTESIAN_POINT('Ctrl Pts',(37.9808888409178,740.125373764374,81.814182427552));
#81798=CARTESIAN_POINT('Ctrl Pts',(37.9809426469069,740.125373479124,81.8142439628075));
#81799=CARTESIAN_POINT('Ctrl Pts',(37.9827466960379,740.59524704715,81.8148446402991));
#81800=CARTESIAN_POINT('Ctrl Pts',(37.9844092385585,741.06512079536,81.8155325195939));
#81801=CARTESIAN_POINT('Ctrl Pts',(37.9840335952872,741.534967841274,81.8169143815015));
#81802=CARTESIAN_POINT('Ctrl Pts',(37.9837494506095,741.890370287103,81.8179596516719));
#81803=CARTESIAN_POINT('Ctrl Pts',(37.9822977692306,742.245757495851,81.8194024431643));
#81804=CARTESIAN_POINT('Ctrl Pts',(37.97883925489,742.601120543275,81.8215114577564));
#81805=CARTESIAN_POINT('Ctrl Pts',(37.9788240082044,742.602687143306,81.8215207552406));
#81806=CARTESIAN_POINT('Ctrl Pts',(37.9788087225029,742.604253741534,81.8215300656766));
#81807=CARTESIAN_POINT('Ctrl Pts',(37.9787933977119,742.605820337965,81.8215393890886));
#81808=CARTESIAN_POINT('Ctrl Pts',(37.9737782986691,743.118495274342,81.8245905128916));
#81809=CARTESIAN_POINT('Ctrl Pts',(37.9645767685362,743.631503793139,81.8290294628732));
#81810=CARTESIAN_POINT('Ctrl Pts',(37.9492753233026,744.14400294551,81.835443517788));
#81811=CARTESIAN_POINT('Ctrl Pts',(37.940075009395,744.452153777489,81.8393001024266));
#81812=CARTESIAN_POINT('Ctrl Pts',(37.9286685542766,744.760120076633,81.8438710044871));
#81813=CARTESIAN_POINT('Ctrl Pts',(37.9146320060792,745.067715043578,81.8492863515391));
#81814=CARTESIAN_POINT('Ctrl Pts',(37.9145109708903,745.070367391891,81.8493330473181));
#81815=CARTESIAN_POINT('Ctrl Pts',(37.9143897370563,745.073019691594,81.8493798067728));
#81816=CARTESIAN_POINT('Ctrl Pts',(37.9142683044256,745.075671942701,81.8494266299454));
#81817=CARTESIAN_POINT('Ctrl Pts',(37.8866198583192,745.679550993783,81.8600875862031));
#81818=CARTESIAN_POINT('Ctrl Pts',(37.8486433540992,746.281212927868,81.8740631070229));
#81819=CARTESIAN_POINT('Ctrl Pts',(37.7985599020469,746.880257424195,81.8918453024477));
#81820=CARTESIAN_POINT('Ctrl Pts',(37.7539545794202,747.413778416287,81.9076824808256));
#81821=CARTESIAN_POINT('Ctrl Pts',(37.6997452435811,747.945223820169,81.9265392815381));
#81822=CARTESIAN_POINT('Ctrl Pts',(37.6347063987271,748.474332613323,81.9487526687549));
#81823=CARTESIAN_POINT('Ctrl Pts',(37.5766710855168,748.946465760858,81.9685740676049));
#81824=CARTESIAN_POINT('Ctrl Pts',(37.5100128380444,749.416738761758,81.9910680943248));
#81825=CARTESIAN_POINT('Ctrl Pts',(37.4338923550026,749.884978811516,82.0164642440168));
#81826=CARTESIAN_POINT('Ctrl Pts',(37.4299124359474,749.909460494001,82.0177920682246));
#81827=CARTESIAN_POINT('Ctrl Pts',(37.4259068238323,749.93393682343,82.019127764189));
#81828=CARTESIAN_POINT('Ctrl Pts',(37.42187547866,749.958407780289,82.0204713395027));
#81829=CARTESIAN_POINT('Ctrl Pts',(37.3372425300594,750.472144298872,82.048677989048));
#81830=CARTESIAN_POINT('Ctrl Pts',(37.2412646275997,750.983457551872,82.0803621354665));
#81831=CARTESIAN_POINT('Ctrl Pts',(37.1335886143222,751.492258643645,82.115588980578));
#81832=CARTESIAN_POINT('Ctrl Pts',(37.0243826544436,752.008289186781,82.1513163567762));
#81833=CARTESIAN_POINT('Ctrl Pts',(36.903143375796,752.521735767981,82.1906879120542));
#81834=CARTESIAN_POINT('Ctrl Pts',(36.7695549149236,753.032515831067,82.233756080504));
#81835=CARTESIAN_POINT('Ctrl Pts',(36.6359664540512,753.543295894153,82.2768242489537));
#81836=CARTESIAN_POINT('Ctrl Pts',(36.4900285286155,754.051409567256,82.3235890827042));
#81837=CARTESIAN_POINT('Ctrl Pts',(36.3314825399832,754.556782671789,82.3740865194685));
#81838=CARTESIAN_POINT('Ctrl Pts',(36.3162234058514,754.605421909245,82.3789466056022));
#81839=CARTESIAN_POINT('Ctrl Pts',(36.3008472050756,754.654038994412,82.3838413589757));
#81840=CARTESIAN_POINT('Ctrl Pts',(36.2853543869488,754.702633073474,82.388770610727));
#81841=CARTESIAN_POINT('Ctrl Pts',(36.1002458846035,755.283236106727,82.4476654097167));
#81842=CARTESIAN_POINT('Ctrl Pts',(35.8983907512341,755.860820660562,82.5115195397896));
#81843=CARTESIAN_POINT('Ctrl Pts',(35.6804717557189,756.434123844787,82.5800712398139));
#81844=CARTESIAN_POINT('Ctrl Pts',(35.6280069590958,756.572148686965,82.5965753127674));
#81845=CARTESIAN_POINT('Ctrl Pts',(35.5746112583638,756.709925496093,82.6133516164342));
#81846=CARTESIAN_POINT('Ctrl Pts',(35.5202945448795,756.847436900889,82.6303964032376));
#81847=CARTESIAN_POINT('Ctrl Pts',(35.497861482644,756.904229768204,82.6374359816403));
#81848=CARTESIAN_POINT('Ctrl Pts',(35.4752936356645,756.960922884651,82.6445143553775));
#81849=CARTESIAN_POINT('Ctrl Pts',(35.4525923201978,757.017516942744,82.651631118668));
#81850=CARTESIAN_POINT('Ctrl Pts',(35.1875439041849,757.678278891777,82.734722639952));
#81851=CARTESIAN_POINT('Ctrl Pts',(34.9042764143143,758.325612285822,82.8230551210942));
#81852=CARTESIAN_POINT('Ctrl Pts',(34.6047070769484,758.960937830743,82.9160405142498));
#81853=CARTESIAN_POINT('Ctrl Pts',(34.5867726694948,758.998973055872,82.9216072986969));
#81854=CARTESIAN_POINT('Ctrl Pts',(34.5687798227313,759.036965234549,82.9271907631233));
#81855=CARTESIAN_POINT('Ctrl Pts',(34.5507289434783,759.074914668111,82.9327907826882));
#81856=CARTESIAN_POINT('Ctrl Pts',(34.5222206321713,759.134849381028,82.9416350666061));
#81857=CARTESIAN_POINT('Ctrl Pts',(34.4935678348722,759.194677750235,82.950520481513));
#81858=CARTESIAN_POINT('Ctrl Pts',(34.4647721445413,759.254400744103,82.9594465899417));
#81859=CARTESIAN_POINT('Ctrl Pts',(34.1949133510472,759.814094742889,83.0430976093646));
#81860=CARTESIAN_POINT('Ctrl Pts',(33.912510712514,760.364551038498,83.1303190024909));
#81861=CARTESIAN_POINT('Ctrl Pts',(33.618793061381,760.90667060331,83.220776067925));
#81862=CARTESIAN_POINT('Ctrl Pts',(33.3134812904446,761.470189628311,83.3148038076091));
#81863=CARTESIAN_POINT('Ctrl Pts',(32.9959434573165,762.024700696235,83.4123277444519));
#81864=CARTESIAN_POINT('Ctrl Pts',(32.6675131954889,762.571185853467,83.512984538312));
#81865=CARTESIAN_POINT('Ctrl Pts',(32.5238668199846,762.810203450891,83.5570090551986));
#81866=CARTESIAN_POINT('Ctrl Pts',(32.3781362077929,763.047685365439,83.6016330258509));
#81867=CARTESIAN_POINT('Ctrl Pts',(32.230430415535,763.283712134329,83.6468267333961));
#81868=CARTESIAN_POINT('Ctrl Pts',(32.1941831345178,763.341633550198,83.6579173547763));
#81869=CARTESIAN_POINT('Ctrl Pts',(32.1578171062028,763.39946717192,83.6690422855322));
#81870=CARTESIAN_POINT('Ctrl Pts',(32.1213337000335,763.457214005624,83.6802012019161));
#81871=CARTESIAN_POINT('Ctrl Pts',(31.7502871493371,764.044515623252,83.7936905349721));
#81872=CARTESIAN_POINT('Ctrl Pts',(31.3671032562343,764.62286796126,83.910692328112));
#81873=CARTESIAN_POINT('Ctrl Pts',(30.9732032066471,765.193301121279,84.0308718910516));
#81874=CARTESIAN_POINT('Ctrl Pts',(30.5580738785247,765.794477827669,84.1575285423251));
#81875=CARTESIAN_POINT('Ctrl Pts',(30.1310419378069,766.386858621788,84.2877147689403));
#81876=CARTESIAN_POINT('Ctrl Pts',(29.6937240880705,766.971618419196,84.4210507830968));
#81877=CARTESIAN_POINT('Ctrl Pts',(29.6303795406661,767.056319614744,84.4403642171918));
#81878=CARTESIAN_POINT('Ctrl Pts',(29.5668191133517,767.140860866817,84.4597437554177));
#81879=CARTESIAN_POINT('Ctrl Pts',(29.503047648562,767.225245698764,84.4791882620394));
#81880=CARTESIAN_POINT('Ctrl Pts',(29.4655179406033,767.274906438242,84.4906314154517));
#81881=CARTESIAN_POINT('Ctrl Pts',(29.4279150906882,767.32451295757,84.5020971038909));
#81882=CARTESIAN_POINT('Ctrl Pts',(29.3902398839613,767.374065886495,84.5135851689969));
#81883=CARTESIAN_POINT('Ctrl Pts',(28.8372399597301,768.101408038588,84.6822079765435));
#81884=CARTESIAN_POINT('Ctrl Pts',(28.2686639470961,768.817231510892,84.85564644981));
#81885=CARTESIAN_POINT('Ctrl Pts',(27.6870997968389,769.523343990526,85.0333678725965));
#81886=CARTESIAN_POINT('Ctrl Pts',(27.2888276362705,770.006910494313,85.1550767072989));
#81887=CARTESIAN_POINT('Ctrl Pts',(26.8844630765403,770.485921879645,85.278794462455));
#81888=CARTESIAN_POINT('Ctrl Pts',(26.4748262094946,770.960950931432,85.4043528068919));
#81889=CARTESIAN_POINT('Ctrl Pts',(26.4409425167201,771.000243631246,85.4147385429192));
#81890=CARTESIAN_POINT('Ctrl Pts',(26.4070217053255,771.039510056123,85.4251371961802));
#81891=CARTESIAN_POINT('Ctrl Pts',(26.3730642728265,771.078750367021,85.4355486646748));
#81892=CARTESIAN_POINT('Ctrl Pts',(25.7100717721007,771.8448869662,85.638824502258));
#81893=CARTESIAN_POINT('Ctrl Pts',(25.0328724614708,772.601367096943,85.8470613974414));
#81894=CARTESIAN_POINT('Ctrl Pts',(24.3457466839457,773.348724068689,86.0593230190846));
#81895=CARTESIAN_POINT('Ctrl Pts',(23.9775445712505,773.749201572131,86.1730651898625));
#81896=CARTESIAN_POINT('Ctrl Pts',(23.6064930208942,774.147060117326,86.287962674055));
#81897=CARTESIAN_POINT('Ctrl Pts',(23.2332540233972,774.542385963715,86.4038694764088));
#81898=CARTESIAN_POINT('Ctrl Pts',(23.2062709433082,774.570965798742,86.4122488862554));
#81899=CARTESIAN_POINT('Ctrl Pts',(23.1792765535914,774.599532492652,86.4206334784754));
#81900=CARTESIAN_POINT('Ctrl Pts',(23.1522710105224,774.628086137261,86.4290232311268));
#81901=CARTESIAN_POINT('Ctrl Pts',(22.4054414532268,775.417727941851,86.6610391266233));
#81902=CARTESIAN_POINT('Ctrl Pts',(21.6500097546164,776.197495325431,86.8970247415881));
#81903=CARTESIAN_POINT('Ctrl Pts',(20.8885671226297,776.970039421042,87.1367381864585));
#81904=CARTESIAN_POINT('Ctrl Pts',(20.0199236634596,777.851347279813,87.4102000432217));
#81905=CARTESIAN_POINT('Ctrl Pts',(19.143457320241,778.723254574552,87.6885131079581));
#81906=CARTESIAN_POINT('Ctrl Pts',(18.2629623050438,779.589646932752,87.9713327580525));
#81907=CARTESIAN_POINT('Ctrl Pts',(17.6497070459899,780.193079843671,88.1683135867802));
#81908=CARTESIAN_POINT('Ctrl Pts',(17.0344962824946,780.793836325147,88.3674808723051));
#81909=CARTESIAN_POINT('Ctrl Pts',(16.4186020601252,781.39321950309,88.5687220124197));
#81910=CARTESIAN_POINT('Ctrl Pts',(16.4153549874364,781.396379527452,88.5697829813105));
#81911=CARTESIAN_POINT('Ctrl Pts',(16.4121078922666,781.39953951086,88.5708440079859));
#81912=CARTESIAN_POINT('Ctrl Pts',(16.408860774807,781.402699453514,88.5719050924519));
#81913=CARTESIAN_POINT('Ctrl Pts',(15.0040136404545,782.769830897858,89.0309773280409));
#81914=CARTESIAN_POINT('Ctrl Pts',(13.5950748355171,784.129278826655,89.5008398450487));
#81915=CARTESIAN_POINT('Ctrl Pts',(12.1980182279082,785.496799332103,89.9818285700894));
#81916=CARTESIAN_POINT('Ctrl Pts',(11.3291011844497,786.347346022903,90.2809855968148));
#81917=CARTESIAN_POINT('Ctrl Pts',(10.4647792418779,787.201014039128,90.584447359179));
#81918=CARTESIAN_POINT('Ctrl Pts',(9.60890053120187,788.061597029217,90.8923018138587));
#81919=CARTESIAN_POINT('Ctrl Pts',(9.58424946245066,788.0863835909,90.9011686558925));
#81920=CARTESIAN_POINT('Ctrl Pts',(9.55960541231716,788.111175895238,90.9100391396316));
#81921=CARTESIAN_POINT('Ctrl Pts',(9.53496847334693,788.135974031963,90.91891326703));
#81922=CARTESIAN_POINT('Ctrl Pts',(8.59423498486735,789.082862673328,91.2577617268507));
#81923=CARTESIAN_POINT('Ctrl Pts',(7.66378701510754,790.038210513089,91.6018883436517));
#81924=CARTESIAN_POINT('Ctrl Pts',(6.75031466068051,791.008392590562,91.9520631261947));
#81925=CARTESIAN_POINT('Ctrl Pts',(6.60468479907203,791.163063370682,92.0078895613061));
#81926=CARTESIAN_POINT('Ctrl Pts',(6.45948646854013,791.318111255008,92.0638697355003));
#81927=CARTESIAN_POINT('Ctrl Pts',(6.31474687067201,791.473562167901,92.1200067905554));
#81928=CARTESIAN_POINT('Ctrl Pts',(5.82689730392431,791.997514573619,92.309218577727));
#81929=CARTESIAN_POINT('Ctrl Pts',(5.34457107578471,792.525722147699,92.5000943886224));
#81930=CARTESIAN_POINT('Ctrl Pts',(4.86909463668608,793.058804009112,92.6926189943811));
#81931=CARTESIAN_POINT('Ctrl Pts',(4.42763029014315,793.553753109111,92.871371803744));
#81932=CARTESIAN_POINT('Ctrl Pts',(3.99207103417591,794.052904312235,93.0515459213008));
#81933=CARTESIAN_POINT('Ctrl Pts',(3.56344441385697,794.556723524126,93.233121145656));
#81934=CARTESIAN_POINT('Ctrl Pts',(3.43512442690785,794.707554274318,93.2874801829043));
#81935=CARTESIAN_POINT('Ctrl Pts',(3.30742552153365,794.858803170986,93.3419647388763));
#81936=CARTESIAN_POINT('Ctrl Pts',(3.18037457161906,795.0104821055,93.3965741249367));
#81937=CARTESIAN_POINT('Ctrl Pts',(3.13179027251589,795.068484148988,93.4174567609814));
#81938=CARTESIAN_POINT('Ctrl Pts',(3.08329934447481,795.126550660042,93.4383582328862));
#81939=CARTESIAN_POINT('Ctrl Pts',(3.03490304960601,795.184682618555,93.4592786115396));
#81940=CARTESIAN_POINT('Ctrl Pts',(2.5486063539281,795.768805420002,93.6694912122997));
#81941=CARTESIAN_POINT('Ctrl Pts',(2.07201161992725,796.359670351005,93.88165210726));
#81942=CARTESIAN_POINT('Ctrl Pts',(1.60626353450439,796.958089247717,94.0959442263557));
#81943=CARTESIAN_POINT('Ctrl Pts',(1.15619334881705,797.536364311837,94.3030228958153));
#81944=CARTESIAN_POINT('Ctrl Pts',(0.71625188401368,798.121693370953,94.5120917355322));
#81945=CARTESIAN_POINT('Ctrl Pts',(0.28743872356641,798.714778005,94.7233075671941));
#81946=CARTESIAN_POINT('Ctrl Pts',(0.224074940183661,798.802415441874,94.754517976386));
#81947=CARTESIAN_POINT('Ctrl Pts',(0.160953410662966,798.890220616696,94.785775156932));
#81948=CARTESIAN_POINT('Ctrl Pts',(0.0980770791788375,798.978196277738,
94.8170797440185));
#81949=CARTESIAN_POINT('Ctrl Pts',(-0.369182434230171,799.63197908599,95.0497168235724));
#81950=CARTESIAN_POINT('Ctrl Pts',(-0.822955604702935,800.295117632775,
95.2849851591274));
#81951=CARTESIAN_POINT('Ctrl Pts',(-1.26279292192534,800.967941700168,95.5231915489782));
#81952=CARTESIAN_POINT('Ctrl Pts',(-1.48341606559332,801.305431392541,95.6426762777924));
#81953=CARTESIAN_POINT('Ctrl Pts',(-1.70054450132931,801.64534585775,95.7629004304533));
#81954=CARTESIAN_POINT('Ctrl Pts',(-1.91420412082378,801.98764121032,95.8839019515004));
#81955=CARTESIAN_POINT('Ctrl Pts',(-2.02120199779361,802.15905814024,95.9444978932736));
#81956=CARTESIAN_POINT('Ctrl Pts',(-2.12733090562511,802.331071173192,96.0052887647587));
#81957=CARTESIAN_POINT('Ctrl Pts',(-2.23260018314948,802.503668568799,96.0662790978337));
#81958=CARTESIAN_POINT('Ctrl Pts',(-2.25752083667438,802.544527972382,96.0807174885463));
#81959=CARTESIAN_POINT('Ctrl Pts',(-2.2823890579689,802.585424172706,96.0951666815795));
#81960=CARTESIAN_POINT('Ctrl Pts',(-2.3072174972792,802.626345096273,96.1096278308841));
#81961=CARTESIAN_POINT('Origin',(52.8776183915471,831.777100559639,108.439826246791));
#81962=CARTESIAN_POINT('Ctrl Pts',(-3.40945017935348,804.520999278367,96.7791350119252));
#81963=CARTESIAN_POINT('Ctrl Pts',(-3.46667793432084,804.486019404866,96.7878665218692));
#81964=CARTESIAN_POINT('Ctrl Pts',(-3.52304849176604,804.450364686567,96.7998559185783));
#81965=CARTESIAN_POINT('Ctrl Pts',(-3.57823712091559,804.414238076631,96.8150416942174));
#81966=CARTESIAN_POINT('Ctrl Pts',(-3.63506842586774,804.377036167147,96.8306794706866));
#81967=CARTESIAN_POINT('Ctrl Pts',(-3.69064613886921,804.339334172832,96.8497062468343));
#81968=CARTESIAN_POINT('Ctrl Pts',(-3.7446495153042,804.301350628926,96.8720101986567));
#81969=CARTESIAN_POINT('Ctrl Pts',(-3.80177576206803,804.261170598614,96.8956039281553));
#81970=CARTESIAN_POINT('Ctrl Pts',(-3.85714010926235,804.22067577032,96.9228644349813));
#81971=CARTESIAN_POINT('Ctrl Pts',(-3.91040432059931,804.180116757718,96.953616843281));
#81972=CARTESIAN_POINT('Ctrl Pts',(-3.96553462626411,804.138136773296,96.9854466522077));
#81973=CARTESIAN_POINT('Ctrl Pts',(-4.0184152243734,804.096088090149,97.021016895017));
#81974=CARTESIAN_POINT('Ctrl Pts',(-4.06871448527445,804.054237640207,97.0600961959471));
#81975=CARTESIAN_POINT('Ctrl Pts',(-4.12125356143182,804.010523598741,97.1009156897322));
#81976=CARTESIAN_POINT('Ctrl Pts',(-4.17097653717914,803.967025723494,97.1455636479873));
#81977=CARTESIAN_POINT('Ctrl Pts',(-4.21754878663746,803.924036824183,97.193740329175));
#81978=CARTESIAN_POINT('Ctrl Pts',(-4.2510073136189,803.893152654657,97.2283515151526));
#81979=CARTESIAN_POINT('Ctrl Pts',(-4.28284057407814,803.862530918084,97.2647832827392));
#81980=CARTESIAN_POINT('Ctrl Pts',(-4.31293627306915,803.83227757975,97.3029132850214));
#81981=CARTESIAN_POINT('Ctrl Pts',(-4.35503392302775,803.789959424999,97.3562492613505));
#81982=CARTESIAN_POINT('Ctrl Pts',(-4.3936829806961,803.748409996973,97.412849490922));
#81983=CARTESIAN_POINT('Ctrl Pts',(-4.4286303447873,803.707907145932,97.4723270319076));
#81984=CARTESIAN_POINT('Ctrl Pts',(-4.46264936649609,803.668480213324,97.5302246104687));
#81985=CARTESIAN_POINT('Ctrl Pts',(-4.4931608496782,803.630044812499,97.5908490142823));
#81986=CARTESIAN_POINT('Ctrl Pts',(-4.51996545111149,803.592850417633,97.6538087985575));
#81987=CARTESIAN_POINT('Ctrl Pts',(-4.54516688592327,803.557880596503,97.713002997103));
#81988=CARTESIAN_POINT('Ctrl Pts',(-4.56709154016755,803.524007777126,97.7742616441211));
#81989=CARTESIAN_POINT('Ctrl Pts',(-4.58560390336969,803.491434394108,97.8372257077396));
#81990=CARTESIAN_POINT('Ctrl Pts',(-4.60352285616161,803.459905144913,97.8981714698365));
#81991=CARTESIAN_POINT('Ctrl Pts',(-4.61824441404098,803.429593543633,97.9607151154782));
#81992=CARTESIAN_POINT('Ctrl Pts',(-4.62967815148095,803.40067698333,98.0244973547518));
#81993=CARTESIAN_POINT('Ctrl Pts',(-4.64062622635985,803.372988690758,98.085570362172));
#81994=CARTESIAN_POINT('Ctrl Pts',(-4.64855954807306,803.346579693476,98.1477787580681));
#81995=CARTESIAN_POINT('Ctrl Pts',(-4.6534337763171,803.321596805669,98.2107770840891));
#81996=CARTESIAN_POINT('Ctrl Pts',(-4.65731484044172,803.30170438686,98.2609389827098));
#81997=CARTESIAN_POINT('Ctrl Pts',(-4.65925699042526,803.282716040417,98.3116010570751));
#81998=CARTESIAN_POINT('Ctrl Pts',(-4.659256990425,803.264699682484,98.3625762498986));
#81999=CARTESIAN_POINT('Origin',(108.644128965869,804.142030366665,98.6726132747675));
#82000=CARTESIAN_POINT('Ctrl Pts',(110.421072908878,803.276519768482,98.366706730931));
#82001=CARTESIAN_POINT('Ctrl Pts',(110.421014271246,803.768657750697,96.9739242975922));
#82002=CARTESIAN_POINT('Ctrl Pts',(109.171101223695,804.532439790988,96.7831441306878));
#82003=CARTESIAN_POINT('Ctrl Pts',(110.052254005922,802.614532539069,98.1328076646065));
#82004=CARTESIAN_POINT('Ctrl Pts',(110.052305119154,803.10632016932,96.7416534710974));
#82005=CARTESIAN_POINT('Ctrl Pts',(108.812286380141,803.884051253074,96.5547193989541));
#82006=CARTESIAN_POINT('Ctrl Pts',(109.671712416757,801.960951606285,97.901782698405));
#82007=CARTESIAN_POINT('Ctrl Pts',(109.671681841165,802.453140325948,96.5090374725116));
#82008=CARTESIAN_POINT('Ctrl Pts',(108.437995444743,803.245379043133,96.3283029022672));
#82009=CARTESIAN_POINT('Ctrl Pts',(109.279637963697,801.31562045008,97.6736561886769));
#82010=CARTESIAN_POINT('Ctrl Pts',(109.279678408479,801.807888527408,96.2810525353335));
#82011=CARTESIAN_POINT('Ctrl Pts',(108.054721885659,802.614266885493,96.105245090354));
#82012=CARTESIAN_POINT('Ctrl Pts',(108.062487312194,802.626301820665,96.1096219232672));
#82013=CARTESIAN_POINT('Ctrl Pts',(108.118602839649,802.589390382965,96.1176812397369));
#82014=CARTESIAN_POINT('Ctrl Pts',(108.173877147318,802.55183405875,96.1290098394246));
#82015=CARTESIAN_POINT('Ctrl Pts',(108.227991810621,802.513846617947,96.1435497736361));
#82016=CARTESIAN_POINT('Ctrl Pts',(108.283722724182,802.474724600908,96.1585239741071));
#82017=CARTESIAN_POINT('Ctrl Pts',(108.338223437648,802.435145655062,96.1769037122149));
#82018=CARTESIAN_POINT('Ctrl Pts',(108.391179399861,802.395339000355,96.198580674604));
#82019=CARTESIAN_POINT('Ctrl Pts',(108.447209799911,802.353221310585,96.2215161255675));
#82020=CARTESIAN_POINT('Ctrl Pts',(108.501510662581,802.31084896716,96.2481423888305));
#82021=CARTESIAN_POINT('Ctrl Pts',(108.55375011033,802.268483950337,96.2782882195284));
#82022=CARTESIAN_POINT('Ctrl Pts',(108.607829357391,802.224626897663,96.3094957436591));
#82023=CARTESIAN_POINT('Ctrl Pts',(108.659699593296,802.180777751386,96.3444746782031));
#82024=CARTESIAN_POINT('Ctrl Pts',(108.709035256812,802.137214687147,96.3829971093564));
#82025=CARTESIAN_POINT('Ctrl Pts',(108.760576879989,802.091703775133,96.4232420050129));
#82026=CARTESIAN_POINT('Ctrl Pts',(108.809352452134,802.046504974408,96.4673542972343));
#82027=CARTESIAN_POINT('Ctrl Pts',(108.855033248751,802.001922593523,96.515037567581));
#82028=CARTESIAN_POINT('Ctrl Pts',(108.887652344881,801.970087838538,96.5490865617847));
#82029=CARTESIAN_POINT('Ctrl Pts',(108.918694344536,801.938567095153,96.5849556525495));
#82030=CARTESIAN_POINT('Ctrl Pts',(108.948050870766,801.90746822385,96.6225258003466));
#82031=CARTESIAN_POINT('Ctrl Pts',(108.989460056698,801.863601353023,96.6755208047089));
#82032=CARTESIAN_POINT('Ctrl Pts',(109.027466079045,801.820625240543,96.7318402448099));
#82033=CARTESIAN_POINT('Ctrl Pts',(109.061816904743,801.778823729021,96.7910956325936));
#82034=CARTESIAN_POINT('Ctrl Pts',(109.095235650154,801.738156465776,96.8487431760892));
#82035=CARTESIAN_POINT('Ctrl Pts',(109.125194979059,801.698600727609,96.9091698637508));
#82036=CARTESIAN_POINT('Ctrl Pts',(109.151496205164,801.660409921191,96.9719830641364));
#82037=CARTESIAN_POINT('Ctrl Pts',(109.17619271011,801.624549256907,97.030963832098));
#82038=CARTESIAN_POINT('Ctrl Pts',(109.197663830857,801.589892049051,97.0920488555737));
#82039=CARTESIAN_POINT('Ctrl Pts',(109.215774451259,801.556642318281,97.1548789506565));
#82040=CARTESIAN_POINT('Ctrl Pts',(109.233295236484,801.524475480332,97.2156627657432));
#82041=CARTESIAN_POINT('Ctrl Pts',(109.247670494366,801.493626127562,97.2780798931909));
#82042=CARTESIAN_POINT('Ctrl Pts',(109.258809538119,801.464271879396,97.3417709039283));
#82043=CARTESIAN_POINT('Ctrl Pts',(109.26947065127,801.436177101411,97.4027291950817));
#82044=CARTESIAN_POINT('Ctrl Pts',(109.277166990319,801.409452143862,97.464854188198));
#82045=CARTESIAN_POINT('Ctrl Pts',(109.281853279706,801.384242796069,97.5278001497676));
#82046=CARTESIAN_POINT('Ctrl Pts',(109.285533189291,801.364447151169,97.5772284774392));
#82047=CARTESIAN_POINT('Ctrl Pts',(109.287357614049,801.345585947171,97.627162373131));
#82048=CARTESIAN_POINT('Ctrl Pts',(109.287322495866,801.327723325276,97.6774220453723));
#82049=CARTESIAN_POINT('Ctrl Pts',(109.295214075855,801.340715062203,97.6820532174938));
#82050=CARTESIAN_POINT('Ctrl Pts',(109.294861021846,801.8329774859,96.2899062835287));
#82051=CARTESIAN_POINT('Ctrl Pts',(108.069824947897,802.638398299217,96.1138965465646));
#82052=CARTESIAN_POINT('Ctrl Pts',(108.442187483773,799.934658383676,97.18505161579));
#82053=CARTESIAN_POINT('Ctrl Pts',(108.441981829264,800.427131807017,95.7932530139787));
#82054=CARTESIAN_POINT('Ctrl Pts',(107.235749064159,801.263000987828,95.6278638607556));
#82055=CARTESIAN_POINT('Ctrl Pts',(107.52710530691,798.562162368243,96.6932753022757));
#82056=CARTESIAN_POINT('Ctrl Pts',(107.52535987795,799.057721670121,95.3079216776574));
#82057=CARTESIAN_POINT('Ctrl Pts',(106.344056162865,799.922005251717,95.1533860412624));
#82058=CARTESIAN_POINT('Ctrl Pts',(105.602319018081,795.920775113123,95.7428524103056));
#82059=CARTESIAN_POINT('Ctrl Pts',(105.598173918827,796.419036535808,94.3684927787303));
#82060=CARTESIAN_POINT('Ctrl Pts',(104.467575793977,797.336433927823,94.2323842521393));
#82061=CARTESIAN_POINT('Ctrl Pts',(104.592399256266,794.648346650005,95.2830219901209));
#82062=CARTESIAN_POINT('Ctrl Pts',(104.587966674248,795.147046217482,93.9135888475786));
#82063=CARTESIAN_POINT('Ctrl Pts',(103.482351883554,796.088345213852,93.7848284793472));
#82064=CARTESIAN_POINT('Ctrl Pts',(101.456168750866,790.944845315593,93.9462813965269));
#82065=CARTESIAN_POINT('Ctrl Pts',(101.457735490723,791.445279193071,92.5880663369688));
#82066=CARTESIAN_POINT('Ctrl Pts',(100.414443555522,792.44331512699,92.4721670616595));
#82067=CARTESIAN_POINT('Ctrl Pts',(99.226526723945,788.625058813487,93.1106895076422));
#82068=CARTESIAN_POINT('Ctrl Pts',(99.233925577768,789.118118434763,91.7524962811977));
#82069=CARTESIAN_POINT('Ctrl Pts',(98.2219969540277,790.143303030444,91.6363993045642));
#82070=CARTESIAN_POINT('Ctrl Pts',(94.6762234756949,784.109404432082,91.5115703119863));
#82071=CARTESIAN_POINT('Ctrl Pts',(94.6930413876074,784.581658178514,90.1568569234352));
#82072=CARTESIAN_POINT('Ctrl Pts',(93.7255485233951,785.632982415435,90.02433712775));
#82073=CARTESIAN_POINT('Ctrl Pts',(92.3541248459539,781.91348973001,90.7476546813426));
#82074=CARTESIAN_POINT('Ctrl Pts',(92.3791378846776,782.376338799843,89.3979289669664));
#82075=CARTESIAN_POINT('Ctrl Pts',(91.4209323280296,783.423079983555,89.248233527896));
#82076=CARTESIAN_POINT('Ctrl Pts',(87.7513528206951,777.511282938626,89.2780543750025));
#82077=CARTESIAN_POINT('Ctrl Pts',(87.7764466266993,777.940567375721,87.9475638320085));
#82078=CARTESIAN_POINT('Ctrl Pts',(86.8404914765804,778.961421974556,87.7545659796536));
#82079=CARTESIAN_POINT('Ctrl Pts',(85.4690225979344,775.306343516102,88.5725577284606));
#82080=CARTESIAN_POINT('Ctrl Pts',(85.4979413206163,775.72389797577,87.259453067688));
#82081=CARTESIAN_POINT('Ctrl Pts',(84.5629483705987,776.711061799412,87.0369300296726));
#82082=CARTESIAN_POINT('Ctrl Pts',(82.1733222236736,771.902715674148,87.5663060875807));
#82083=CARTESIAN_POINT('Ctrl Pts',(82.183750371381,772.274875821215,86.2839817908659));
#82084=CARTESIAN_POINT('Ctrl Pts',(81.270476661061,773.211393613522,86.0151631449675));
#82085=CARTESIAN_POINT('Ctrl Pts',(81.096556296596,770.752364778805,87.2398363086889));
#82086=CARTESIAN_POINT('Ctrl Pts',(81.1046082428451,771.113387291667,85.9707508669623));
#82087=CARTESIAN_POINT('Ctrl Pts',(80.1941410218622,772.02430508146,85.6839344533105));
#82088=CARTESIAN_POINT('Ctrl Pts',(79.014739726505,768.4123957434,86.6105536288388));
#82089=CARTESIAN_POINT('Ctrl Pts',(79.0162099655969,768.746782235972,85.3710221059379));
#82090=CARTESIAN_POINT('Ctrl Pts',(78.1134036875601,769.600363807285,85.0463364454658));
#82091=CARTESIAN_POINT('Ctrl Pts',(78.0087611740672,767.221939997721,86.307466040044));
#82092=CARTESIAN_POINT('Ctrl Pts',(78.0071437361477,767.543114000067,85.0845274729088));
#82093=CARTESIAN_POINT('Ctrl Pts',(77.1080622694572,768.362630795394,84.7396761820318));
#82094=CARTESIAN_POINT('Ctrl Pts',(76.0927241109205,764.783750194135,85.7297309016138));
#82095=CARTESIAN_POINT('Ctrl Pts',(76.084470878905,765.073533320776,84.5431656020163));
#82096=CARTESIAN_POINT('Ctrl Pts',(75.19584029529,765.818031164947,84.1566085998454));
#82097=CARTESIAN_POINT('Ctrl Pts',(75.182623032252,763.536105161568,85.4550691342351));
#82098=CARTESIAN_POINT('Ctrl Pts',(75.1713154649656,763.81013185858,84.2883909459588));
#82099=CARTESIAN_POINT('Ctrl Pts',(74.2889243477987,764.511199556224,83.8801784199441));
#82100=CARTESIAN_POINT('Ctrl Pts',(73.4901734252389,760.96320744885,84.941329020355));
#82101=CARTESIAN_POINT('Ctrl Pts',(73.4741566583351,761.20056361727,83.8175931584094));
#82102=CARTESIAN_POINT('Ctrl Pts',(72.6087386229698,761.807693786518,83.3659796212416));
#82103=CARTESIAN_POINT('Ctrl Pts',(72.707836081372,759.63815168905,84.7022138549167));
#82104=CARTESIAN_POINT('Ctrl Pts',(72.6897377638328,759.856915801337,83.6014313699369));
#82105=CARTESIAN_POINT('Ctrl Pts',(71.8355785722929,760.411115842064,83.128212093595));
#82106=CARTESIAN_POINT('Ctrl Pts',(71.658920438192,757.571059475316,84.3774661637953));
#82107=CARTESIAN_POINT('Ctrl Pts',(71.6373194821546,757.752838052951,83.3119628596065));
#82108=CARTESIAN_POINT('Ctrl Pts',(70.8072004200214,758.229721199251,82.8090726008211));
#82109=CARTESIAN_POINT('Ctrl Pts',(71.3290696884154,756.865866044856,84.2745652736144));
#82110=CARTESIAN_POINT('Ctrl Pts',(71.3074689206998,757.037084857487,83.2213327932257));
#82111=CARTESIAN_POINT('Ctrl Pts',(70.4853541094165,757.485138318237,82.7086553235673));
#82112=CARTESIAN_POINT('Ctrl Pts',(70.7257249999294,755.447684184856,84.0846957456631));
#82113=CARTESIAN_POINT('Ctrl Pts',(70.7050549298059,755.597824860978,83.0557025153916));
#82114=CARTESIAN_POINT('Ctrl Pts',(69.899878526431,755.98817308601,82.5248701016234));
#82115=CARTESIAN_POINT('Ctrl Pts',(70.4511377454858,754.732937305474,83.9973933941209));
#82116=CARTESIAN_POINT('Ctrl Pts',(70.4310337524815,754.872430959252,82.9802998082194));
#82117=CARTESIAN_POINT('Ctrl Pts',(69.6351681246828,755.233941812227,82.441172093944));
#82118=CARTESIAN_POINT('Ctrl Pts',(69.7105470631533,752.568708941546,83.7594876855879));
#82119=CARTESIAN_POINT('Ctrl Pts',(69.6954059045199,752.682705696041,82.7772948998672));
#82120=CARTESIAN_POINT('Ctrl Pts',(68.9259081577405,752.953039927856,82.2152182103315));
#82121=CARTESIAN_POINT('Ctrl Pts',(69.3286692857491,751.099448039298,83.6331406219163));
#82122=CARTESIAN_POINT('Ctrl Pts',(69.3150421947875,751.190991418035,82.6713974262477));
#82123=CARTESIAN_POINT('Ctrl Pts',(68.5672888315565,751.408381407968,82.0984264432094));
#82124=CARTESIAN_POINT('Ctrl Pts',(68.9176924348934,748.838880031761,83.4940017770909));
#82125=CARTESIAN_POINT('Ctrl Pts',(68.9082513720638,748.899344003655,82.5559441007562));
#82126=CARTESIAN_POINT('Ctrl Pts',(68.1866424032589,749.047053332051,81.97139742283));
#82127=CARTESIAN_POINT('Ctrl Pts',(68.8074764353244,748.075842023577,83.4559769694687));
#82128=CARTESIAN_POINT('Ctrl Pts',(68.7995471274378,748.127296138224,82.5246052204508));
#82129=CARTESIAN_POINT('Ctrl Pts',(68.0857361905741,748.252477165913,81.9370102412519));
#82130=CARTESIAN_POINT('Ctrl Pts',(68.6358788294816,746.527801456371,83.3956678993834));
#82131=CARTESIAN_POINT('Ctrl Pts',(68.6309578842129,746.563507408634,82.4749758028119));
#82132=CARTESIAN_POINT('Ctrl Pts',(67.9299075561181,746.647068940509,81.8825958600769));
#82133=CARTESIAN_POINT('Ctrl Pts',(68.5746540239514,745.742195057558,83.3734373232148));
#82134=CARTESIAN_POINT('Ctrl Pts',(68.5710208199205,745.770325190704,82.456671026825));
#82135=CARTESIAN_POINT('Ctrl Pts',(67.8751177828609,745.835626086142,81.8626119544358));
#82136=CARTESIAN_POINT('Ctrl Pts',(68.4511339891996,743.3692333769,83.3264891742176));
#82137=CARTESIAN_POINT('Ctrl Pts',(68.4507140403186,743.380436487727,82.41788350119));
#82138=CARTESIAN_POINT('Ctrl Pts',(67.7656841774958,743.397293078928,81.8202937869079));
#82139=CARTESIAN_POINT('Ctrl Pts',(68.4520573306559,741.761597715518,83.3224477769537));
#82140=CARTESIAN_POINT('Ctrl Pts',(68.4520660684083,741.763107158896,82.4141868365033));
#82141=CARTESIAN_POINT('Ctrl Pts',(67.768181414692,741.761742048572,81.8164948678625));
#82142=CARTESIAN_POINT('Ctrl Pts',(68.4578519957978,740.110102294567,83.3198423992737));
#82143=CARTESIAN_POINT('Ctrl Pts',(68.4578585200934,740.111539480387,82.4117286275963));
#82144=CARTESIAN_POINT('Ctrl Pts',(67.7741541147992,740.110097758569,81.8140506910839));
#82145=CARTESIAN_POINT('Origin',(66.4578107338364,740.118392461545,83.3196239580187));
#82146=CARTESIAN_POINT('Origin',(52.8776183915471,640.125373764374,98.8443190641064));
#82147=CARTESIAN_POINT('Ctrl Pts',(67.7745968623189,740.125373764374,81.8142915850038));
#82148=CARTESIAN_POINT('Ctrl Pts',(67.8942035323011,706.959289447806,81.7651023987915));
#82149=CARTESIAN_POINT('Ctrl Pts',(68.0137456503395,673.793204547609,81.7161493121274));
#82150=CARTESIAN_POINT('Ctrl Pts',(68.1332263705164,640.627119090081,81.66742515578));
#82151=CARTESIAN_POINT('Ctrl Pts',(37.622010412585,640.627119090085,81.6674251557736));
#82152=CARTESIAN_POINT('Ctrl Pts',(37.7161153406155,666.749258887989,81.7058010809911));
#82153=CARTESIAN_POINT('Ctrl Pts',(37.8102583547102,692.871398339875,81.7443190218601));
#82154=CARTESIAN_POINT('Ctrl Pts',(37.9044409990548,718.993537433499,81.7829824784269));
#82155=CARTESIAN_POINT('Ctrl Pts',(37.9298377480952,726.037482903233,81.793408243283));
#82156=CARTESIAN_POINT('Ctrl Pts',(37.9552373778878,733.081428123876,81.803844588833));
#82157=CARTESIAN_POINT('Ctrl Pts',(37.9806399232851,740.125374460328,81.8142915860359));
#82158=CARTESIAN_POINT('Ctrl Pts',(-2.54756887983518,803.022417447735,96.2501688554413));
#82159=CARTESIAN_POINT('Ctrl Pts',(-3.76067897315835,802.223917717087,96.4241939687641));
#82160=CARTESIAN_POINT('Ctrl Pts',(-3.77095614126524,801.727425136398,97.8000254103195));
#82161=CARTESIAN_POINT('Ctrl Pts',(-2.49510594629795,802.935978449927,96.219371864756));
#82162=CARTESIAN_POINT('Ctrl Pts',(-3.71075325311643,802.135854698797,96.393779692249));
#82163=CARTESIAN_POINT('Ctrl Pts',(-3.71892210633938,801.640324877161,97.7731993356308));
#82164=CARTESIAN_POINT('Ctrl Pts',(-2.44263599469854,802.849517379784,96.1886494506309));
#82165=CARTESIAN_POINT('Ctrl Pts',(-3.66085515329841,802.047826199787,96.363461972859));
#82166=CARTESIAN_POINT('Ctrl Pts',(-3.66686675102868,801.553206555292,97.7464448827534));
#82167=CARTESIAN_POINT('Ctrl Pts',(-2.36392313096885,802.719800352555,96.1426793912113));
#82168=CARTESIAN_POINT('Ctrl Pts',(-3.58602456746336,801.915795967737,96.3181154713988));
#82169=CARTESIAN_POINT('Ctrl Pts',(-3.58875388690028,801.422509800265,97.7064217180787));
#82170=CARTESIAN_POINT('Ctrl Pts',(-2.3376840822935,802.676556934075,96.1273749027454));
#82171=CARTESIAN_POINT('Ctrl Pts',(-3.56107010939721,801.871763815172,96.3030133965861));
#82172=CARTESIAN_POINT('Ctrl Pts',(-3.56271119025831,801.378940829508,97.693098694744));
#82173=CARTESIAN_POINT('Ctrl Pts',(-2.28520294972504,802.590061552113,96.0968035718952));
#82174=CARTESIAN_POINT('Ctrl Pts',(-3.51115718317375,801.78368761136,96.2728469833879));
#82175=CARTESIAN_POINT('Ctrl Pts',(-3.5106154032456,801.291796406231,97.6664885739323));
#82176=CARTESIAN_POINT('Ctrl Pts',(-2.25892246716778,802.546846114927,96.0815333620853));
#82177=CARTESIAN_POINT('Ctrl Pts',(-3.482711717244,801.739390886515,96.2567977055715));
#82178=CARTESIAN_POINT('Ctrl Pts',(-3.48307491491547,801.247085257979,97.6489167037903));
#82179=CARTESIAN_POINT('Ctrl Pts',(-2.12724597762409,802.331001389362,96.0052527348621));
#82180=CARTESIAN_POINT('Ctrl Pts',(-3.34800333457594,801.51876669674,96.1788407103674));
#82181=CARTESIAN_POINT('Ctrl Pts',(-3.34838159956812,801.026426926903,97.5708484797001));
#82182=CARTESIAN_POINT('Ctrl Pts',(-2.02110379157191,802.158997158457,95.9444602975967));
#82183=CARTESIAN_POINT('Ctrl Pts',(-3.23932659433289,801.342952870263,96.1166961159775));
#82184=CARTESIAN_POINT('Ctrl Pts',(-3.23975939827196,800.850558213657,97.5085238064614));
#82185=CARTESIAN_POINT('Ctrl Pts',(-1.70025205868664,801.645032317437,95.7627637886631));
#82186=CARTESIAN_POINT('Ctrl Pts',(-2.91059639593457,800.817621326081,95.9309328218339));
#82187=CARTESIAN_POINT('Ctrl Pts',(-2.91128616137831,800.324991032427,97.3219922775962));
#82188=CARTESIAN_POINT('Ctrl Pts',(-1.48311342467661,801.305123534837,95.64254057864));
#82189=CARTESIAN_POINT('Ctrl Pts',(-2.68784390047268,800.470220965194,95.8079863882428));
#82190=CARTESIAN_POINT('Ctrl Pts',(-2.68882416246288,799.977336107303,97.1982295895679));
#82191=CARTESIAN_POINT('Ctrl Pts',(-0.821956157160209,800.293715588133,
95.2844669131353));
#82192=CARTESIAN_POINT('Ctrl Pts',(-2.0092020871634,799.436803763087,95.4418913907417));
#82193=CARTESIAN_POINT('Ctrl Pts',(-2.01113581282655,798.942895026148,96.8290880220157));
#82194=CARTESIAN_POINT('Ctrl Pts',(-0.368150041841871,799.630582229875,
95.0492110213477));
#82195=CARTESIAN_POINT('Ctrl Pts',(-1.54281133857619,798.759443153596,95.2014321306635));
#82196=CARTESIAN_POINT('Ctrl Pts',(-1.54556290786924,798.264694255303,96.5858881514787));
#82197=CARTESIAN_POINT('Ctrl Pts',(1.03061030691538,797.673484553947,94.3528071728653));
#82198=CARTESIAN_POINT('Ctrl Pts',(-0.106711134755086,796.762712146839,
94.4910767743835));
#82199=CARTESIAN_POINT('Ctrl Pts',(-0.110695325855799,796.264745392156,
95.8668830489244));
#82200=CARTESIAN_POINT('Ctrl Pts',(2.01312465174172,796.412063159207,93.9009736591558));
#82201=CARTESIAN_POINT('Ctrl Pts',(0.901311526995951,795.476698050913,94.0314310313919));
#82202=CARTESIAN_POINT('Ctrl Pts',(0.896808093594574,794.97805572051,95.4019733112351));
#82203=CARTESIAN_POINT('Ctrl Pts',(5.07849924016303,792.729956164408,92.5758839929726));
#82204=CARTESIAN_POINT('Ctrl Pts',(4.0306470527666,791.735946530686,92.6922147735793));
#82205=CARTESIAN_POINT('Ctrl Pts',(4.03172924159146,791.23476686307,94.0506880453146));
#82206=CARTESIAN_POINT('Ctrl Pts',(7.27664404461848,790.409107078949,91.7323566158703));
#82207=CARTESIAN_POINT('Ctrl Pts',(6.26157209028423,789.386372296047,91.8480320390701));
#82208=CARTESIAN_POINT('Ctrl Pts',(6.26821503959616,788.89247683333,93.2063626670902));
#82209=CARTESIAN_POINT('Ctrl Pts',(11.7933103381052,785.862859302431,90.1054677611424));
#82210=CARTESIAN_POINT('Ctrl Pts',(10.8240801502024,784.811849964826,90.2364798435984));
#82211=CARTESIAN_POINT('Ctrl Pts',(10.8403820254109,784.338281826247,91.5915713698604));
#82212=CARTESIAN_POINT('Ctrl Pts',(14.1122918869024,783.637701417767,89.3223002813892));
#82213=CARTESIAN_POINT('Ctrl Pts',(13.1527770859699,782.590309602832,89.4700943476909));
#82214=CARTESIAN_POINT('Ctrl Pts',(13.1774368624816,782.126095976334,90.8205764507483));
#82215=CARTESIAN_POINT('Ctrl Pts',(18.7249146873591,779.148740308681,87.8151433083763));
#82216=CARTESIAN_POINT('Ctrl Pts',(17.7880690821033,778.125688253418,88.0056748348046));
#82217=CARTESIAN_POINT('Ctrl Pts',(17.8131492667992,777.694891150616,89.3376463120531));
#82218=CARTESIAN_POINT('Ctrl Pts',(21.0203075585196,776.886334924432,87.0910859533607));
#82219=CARTESIAN_POINT('Ctrl Pts',(20.0843546720735,775.896396719256,87.3109957127761));
#82220=CARTESIAN_POINT('Ctrl Pts',(20.1135073946011,775.477223638155,88.6259100659374));
#82221=CARTESIAN_POINT('Ctrl Pts',(24.3397387087871,773.370423560442,86.0602581245099));
#82222=CARTESIAN_POINT('Ctrl Pts',(23.425414865776,772.43036838436,86.3263153651351));
#82223=CARTESIAN_POINT('Ctrl Pts',(23.4361862275068,772.056471333472,87.6108938714464));
#82224=CARTESIAN_POINT('Ctrl Pts',(25.4253996464263,772.17790967056,85.7260139011157));
#82225=CARTESIAN_POINT('Ctrl Pts',(24.5138126607302,771.263228374096,86.0100516271665));
#82226=CARTESIAN_POINT('Ctrl Pts',(24.5222414514152,770.900436422346,87.2815154680637));
#82227=CARTESIAN_POINT('Ctrl Pts',(27.5242571088241,769.743996468356,85.0826902645603));
#82228=CARTESIAN_POINT('Ctrl Pts',(26.6201843438213,768.886224410496,85.4045996990067));
#82229=CARTESIAN_POINT('Ctrl Pts',(26.6220269177733,768.550030010176,86.6467338844264));
#82230=CARTESIAN_POINT('Ctrl Pts',(28.5384523052729,768.50166160768,84.7733012266733));
#82231=CARTESIAN_POINT('Ctrl Pts',(27.6379911920885,767.677778332248,85.1154060870583));
#82232=CARTESIAN_POINT('Ctrl Pts',(27.6367436421517,767.35476598226,86.3410381049848));
#82233=CARTESIAN_POINT('Ctrl Pts',(30.4676562121875,765.948841552032,84.1850699287477));
#82234=CARTESIAN_POINT('Ctrl Pts',(29.5774139914747,765.199660947832,84.5689922057617));
#82235=CARTESIAN_POINT('Ctrl Pts',(29.5694662193078,764.908010092887,85.7584008538283));
#82236=CARTESIAN_POINT('Ctrl Pts',(31.3826991203075,764.638386759695,83.9062051751521));
#82237=CARTESIAN_POINT('Ctrl Pts',(30.4985460010245,763.932521667716,84.3118728786106));
#82238=CARTESIAN_POINT('Ctrl Pts',(30.4875123616944,763.656602738954,85.4814464761971));
#82239=CARTESIAN_POINT('Ctrl Pts',(33.0781796764642,761.929051245223,83.3874395020897));
#82240=CARTESIAN_POINT('Ctrl Pts',(32.2107225236239,761.316951014723,83.8367566227028));
#82241=CARTESIAN_POINT('Ctrl Pts',(32.1948719624217,761.077699450203,84.9634374215801));
#82242=CARTESIAN_POINT('Ctrl Pts',(33.8585030159751,760.530256860817,83.147540342318));
#82243=CARTESIAN_POINT('Ctrl Pts',(33.0021498927262,759.971065301871,83.6186294465493));
#82244=CARTESIAN_POINT('Ctrl Pts',(32.9841687445563,759.750391677565,84.7223482483494));
#82245=CARTESIAN_POINT('Ctrl Pts',(34.8968479257256,758.347247245236,82.8254124815966));
#82246=CARTESIAN_POINT('Ctrl Pts',(34.0644292190259,757.865367363984,83.3264590338104));
#82247=CARTESIAN_POINT('Ctrl Pts',(34.0428118160153,757.681740104667,84.3948146040165));
#82248=CARTESIAN_POINT('Ctrl Pts',(35.2209007078652,757.605400534592,82.7243472537898));
#82249=CARTESIAN_POINT('Ctrl Pts',(34.3963889580535,757.15231636156,83.2352634977894));
#82250=CARTESIAN_POINT('Ctrl Pts',(34.3747602646247,756.979163746297,84.2913421825726));
#82251=CARTESIAN_POINT('Ctrl Pts',(35.8196885745711,756.089473367867,82.536445429766));
#82252=CARTESIAN_POINT('Ctrl Pts',(35.0123043239642,755.694916051544,83.0659664510821));
#82253=CARTESIAN_POINT('Ctrl Pts',(34.9915640255228,755.54314104189,84.0973654783811));
#82254=CARTESIAN_POINT('Ctrl Pts',(36.0904492393661,755.325097075514,82.4508556938986));
#82255=CARTESIAN_POINT('Ctrl Pts',(35.292528911043,754.959832059304,82.988886942784));
#82256=CARTESIAN_POINT('Ctrl Pts',(35.2723340002733,754.818874589516,84.008141624083));
#82257=CARTESIAN_POINT('Ctrl Pts',(36.8135735373189,753.020164341297,82.2205312756795));
#82258=CARTESIAN_POINT('Ctrl Pts',(36.042391668946,752.747409898035,82.7820512032344));
#82259=CARTESIAN_POINT('Ctrl Pts',(36.0272207560278,752.632179790114,83.7657201066036));
#82260=CARTESIAN_POINT('Ctrl Pts',(37.1771034358654,751.464582237428,82.1021362636218));
#82261=CARTESIAN_POINT('Ctrl Pts',(36.4280933234008,751.245242086986,82.6747341408129));
#82262=CARTESIAN_POINT('Ctrl Pts',(36.414375945687,751.152783996483,83.6375840405036));
#82263=CARTESIAN_POINT('Ctrl Pts',(37.6907126543852,748.305382907416,81.9307673070529));
#82264=CARTESIAN_POINT('Ctrl Pts',(36.9762334614121,748.184766944419,82.5192847281391));
#82265=CARTESIAN_POINT('Ctrl Pts',(36.9690167893174,748.128934992039,83.4497201824271));
#82266=CARTESIAN_POINT('Ctrl Pts',(37.8401034447293,746.700925585337,81.8780397031153));
#82267=CARTESIAN_POINT('Ctrl Pts',(37.1400301940856,746.619999140862,82.4708341127755));
#82268=CARTESIAN_POINT('Ctrl Pts',(37.1353188681197,746.583923140769,83.3906420629135));
#82269=CARTESIAN_POINT('Ctrl Pts',(37.9518992948506,744.251109993819,81.8349070904933));
#82270=CARTESIAN_POINT('Ctrl Pts',(37.263127800321,744.216555382476,82.4312579044147));
#82271=CARTESIAN_POINT('Ctrl Pts',(37.2615409843506,744.200268989692,83.3427055344115));
#82272=CARTESIAN_POINT('Ctrl Pts',(37.9707386166179,743.429305592017,81.8264396253836));
#82273=CARTESIAN_POINT('Ctrl Pts',(37.2842851583786,743.40744096781,82.4234417302218));
#82274=CARTESIAN_POINT('Ctrl Pts',(37.2834266463915,743.396567644625,83.3333441910137));
#82275=CARTESIAN_POINT('Ctrl Pts',(37.9868489066019,741.782335097605,81.8166385183344));
#82276=CARTESIAN_POINT('Ctrl Pts',(37.3028776730937,741.778675123994,82.4143081461178));
#82277=CARTESIAN_POINT('Ctrl Pts',(37.3028300875899,741.774995661547,83.3225770714669));
#82278=CARTESIAN_POINT('Ctrl Pts',(37.9841298949872,740.955816068756,81.8153066626739));
#82279=CARTESIAN_POINT('Ctrl Pts',(37.3003420559413,740.957253716847,82.412981445933));
#82280=CARTESIAN_POINT('Ctrl Pts',(37.3003369686651,740.955796719301,83.3211559311962));
#82281=CARTESIAN_POINT('Ctrl Pts',(37.9811378013137,740.125371330475,81.8140733335412));
#82282=CARTESIAN_POINT('Ctrl Pts',(37.2974432528674,740.126811574677,82.4117412974523));
#82283=CARTESIAN_POINT('Ctrl Pts',(37.2974382339422,740.125373764374,83.3198410924311));
#82284=CARTESIAN_POINT('Origin',(39.2974260809896,740.118401563543,83.3196239724233));
#82285=CARTESIAN_POINT('Ctrl Pts',(-2.30721749727922,802.626345096273,96.1096278308841));
#82286=CARTESIAN_POINT('Ctrl Pts',(-2.36327072866609,802.589348633611,96.1176523786537));
#82287=CARTESIAN_POINT('Ctrl Pts',(-2.41849852049417,802.551715366678,96.1289510061921));
#82288=CARTESIAN_POINT('Ctrl Pts',(-2.47257991396617,802.513656987001,96.1434674812622));
#82289=CARTESIAN_POINT('Ctrl Pts',(-2.52823332824809,802.474492338403,96.1584059166302));
#82290=CARTESIAN_POINT('Ctrl Pts',(-2.58267247133486,802.434877827384,96.1767515168295));
#82291=CARTESIAN_POINT('Ctrl Pts',(-2.63558008449285,802.395040475326,96.1983975246404));
#82292=CARTESIAN_POINT('Ctrl Pts',(-2.69144357855432,802.352977461192,96.2212528673146));
#82293=CARTESIAN_POINT('Ctrl Pts',(-2.74559941542201,802.310666270982,96.2477873359821));
#82294=CARTESIAN_POINT('Ctrl Pts',(-2.79771392683107,802.268365353768,96.2778317474554));
#82295=CARTESIAN_POINT('Ctrl Pts',(-2.85156635968805,802.224653780112,96.3088780838374));
#82296=CARTESIAN_POINT('Ctrl Pts',(-2.90323918786958,802.180953239413,96.3436719467398));
#82297=CARTESIAN_POINT('Ctrl Pts',(-2.95240600655323,802.13753719224,96.3819880306071));
#82298=CARTESIAN_POINT('Ctrl Pts',(-3.00361526460589,802.092317598561,96.4218958033462));
#82299=CARTESIAN_POINT('Ctrl Pts',(-3.05210620578357,802.047406519098,96.4656244285225));
#82300=CARTESIAN_POINT('Ctrl Pts',(-3.09755173275986,802.003100720221,96.5128822403463));
#82301=CARTESIAN_POINT('Ctrl Pts',(-3.13083736450424,801.970649858636,96.5474952424627));
#82302=CARTESIAN_POINT('Ctrl Pts',(-3.16249016323363,801.938523416787,96.5840007665001));
#82303=CARTESIAN_POINT('Ctrl Pts',(-3.19239386993921,801.906834880987,96.6222719698307));
#82304=CARTESIAN_POINT('Ctrl Pts',(-3.23322357536797,801.863568218598,96.6745264269044));
#82305=CARTESIAN_POINT('Ctrl Pts',(-3.2707467664661,801.821165312288,96.730017165873));
#82306=CARTESIAN_POINT('Ctrl Pts',(-3.30472114590546,801.779906743377,96.7883698877386));
#82307=CARTESIAN_POINT('Ctrl Pts',(-3.33789162255928,801.739624435962,96.8453418657488));
#82308=CARTESIAN_POINT('Ctrl Pts',(-3.36767931860476,801.70043280346,96.9050422820145));
#82309=CARTESIAN_POINT('Ctrl Pts',(-3.39389274176312,801.662584602277,96.9670880638343));
#82310=CARTESIAN_POINT('Ctrl Pts',(-3.41866210564239,801.626821403337,97.0257158339574));
#82311=CARTESIAN_POINT('Ctrl Pts',(-3.44024009918937,801.592257712198,97.0864377315033));
#82312=CARTESIAN_POINT('Ctrl Pts',(-3.45849568331896,801.559100137027,97.1488969208789));
#82313=CARTESIAN_POINT('Ctrl Pts',(-3.47620000246389,801.526943823171,97.2094700263129));
#82314=CARTESIAN_POINT('Ctrl Pts',(-3.49077920080706,801.496110179152,97.271677116829));
#82315=CARTESIAN_POINT('Ctrl Pts',(-3.50214642651331,801.466779625618,97.3351593149313));
#82316=CARTESIAN_POINT('Ctrl Pts',(-3.51304904452183,801.438647887107,97.3960468326192));
#82317=CARTESIAN_POINT('Ctrl Pts',(-3.52099660020155,801.411899132525,97.4581071320463));
#82318=CARTESIAN_POINT('Ctrl Pts',(-3.52594744762757,801.386681807434,97.5209938678202));
#82319=CARTESIAN_POINT('Ctrl Pts',(-3.53001391253826,801.365969117504,97.5726469854316));
#82320=CARTESIAN_POINT('Ctrl Pts',(-3.53205915571888,801.346289518382,97.6248570357437));
#82321=CARTESIAN_POINT('Ctrl Pts',(-3.53208119303051,801.3277173574,97.6774182477473));
#82322=CARTESIAN_POINT('Ctrl Pts',(-3.40946931693737,804.521033637143,96.7791471510659));
#82323=CARTESIAN_POINT('Ctrl Pts',(-4.65925736534058,803.756954223787,96.969801323411));
#82324=CARTESIAN_POINT('Ctrl Pts',(-4.65925854064561,803.26470246339,98.3625772327603));
#82325=CARTESIAN_POINT('Ctrl Pts',(-3.05089567652535,803.877265759675,96.5517004996727));
#82326=CARTESIAN_POINT('Ctrl Pts',(-4.29249081153572,803.098952748285,96.7374561156329));
#82327=CARTESIAN_POINT('Ctrl Pts',(-4.29249163071458,802.606767441921,98.1300418153432));
#82328=CARTESIAN_POINT('Ctrl Pts',(-2.68053925162189,803.241833344296,96.3270499699154));
#82329=CARTESIAN_POINT('Ctrl Pts',(-3.91415453452997,802.44937988459,96.5076786811755));
#82330=CARTESIAN_POINT('Ctrl Pts',(-3.91414269854377,801.957105620144,97.9004419917104));
#82331=CARTESIAN_POINT('Ctrl Pts',(-2.29945272409813,802.614310079946,96.105250940801));
#82332=CARTESIAN_POINT('Ctrl Pts',(-3.52444864420587,801.807911322885,96.2810249800505));
#82333=CARTESIAN_POINT('Ctrl Pts',(-3.52439708867275,801.31561163008,97.6736597068728));
#82334=CARTESIAN_POINT('Ctrl Pts',(37.6198584342843,640.029588266083,99.5508769219774));
#82335=CARTESIAN_POINT('Ctrl Pts',(36.9480411577294,640.030997493993,98.9541445975251));
#82336=CARTESIAN_POINT('Ctrl Pts',(36.9480366099606,640.029588266083,98.0555746669669));
#82337=CARTESIAN_POINT('Ctrl Pts',(37.7400559519511,673.39485105406,99.5018629213698));
#82338=CARTESIAN_POINT('Ctrl Pts',(37.0645737053678,673.414978395905,98.9047878032409));
#82339=CARTESIAN_POINT('Ctrl Pts',(37.0645038212888,673.394851054046,98.0032473080201));
#82340=CARTESIAN_POINT('Ctrl Pts',(37.8603155876735,706.760113449952,99.4526172749795));
#82341=CARTESIAN_POINT('Ctrl Pts',(37.1810433321196,706.780933775647,98.8552405413389));
#82342=CARTESIAN_POINT('Ctrl Pts',(37.1809710312484,706.760113449936,97.9506580829349));
#82343=CARTESIAN_POINT('Ctrl Pts',(37.9806405542058,740.125375436351,99.4031326849135));
#82344=CARTESIAN_POINT('Ctrl Pts',(37.2974428811024,740.126813453391,98.8055008811664));
#82345=CARTESIAN_POINT('Ctrl Pts',(37.2974382397787,740.125375436351,97.8977989293328));
#82346=CARTESIAN_POINT('Ctrl Pts',(36.9501223944842,640.627119090084,98.0546383469715));
#82347=CARTESIAN_POINT('Ctrl Pts',(37.0658943424063,673.793204392933,98.0026202559452));
#82348=CARTESIAN_POINT('Ctrl Pts',(37.1816662884245,706.959289150332,97.9503433686471));
#82349=CARTESIAN_POINT('Ctrl Pts',(37.2974382346222,740.125373959158,97.8977997652524));
#82350=CARTESIAN_POINT('Ctrl Pts',(37.9806399237917,740.125374600818,99.4031321373354));
#82351=CARTESIAN_POINT('Ctrl Pts',(37.9617902823362,734.898502237979,99.4108842010231));
#82352=CARTESIAN_POINT('Ctrl Pts',(37.9429422647548,729.671635581994,99.4186303922604));
#82353=CARTESIAN_POINT('Ctrl Pts',(37.9240958291834,724.444766469215,99.4263707511508));
#82354=CARTESIAN_POINT('Ctrl Pts',(37.8233558620347,696.505551081905,99.4677453387957));
#82355=CARTESIAN_POINT('Ctrl Pts',(37.722661352726,668.56633528394,99.5089531833321));
#82356=CARTESIAN_POINT('Ctrl Pts',(37.622010412585,640.627119090081,99.549998567806));
#82357=CARTESIAN_POINT('Origin',(52.8776183915471,640.125373764374,82.3731046594733));
#82358=CARTESIAN_POINT('Ctrl Pts',(67.7745962349168,740.125373763053,99.4031326874004));
#82359=CARTESIAN_POINT('Ctrl Pts',(68.4577939078287,740.126811780092,98.8055008836706));
#82360=CARTESIAN_POINT('Ctrl Pts',(68.4577985491564,740.125373763053,97.8977989319926));
#82361=CARTESIAN_POINT('Ctrl Pts',(67.8949211990607,706.760112339463,99.4526172769356));
#82362=CARTESIAN_POINT('Ctrl Pts',(68.5741934539237,706.78093266449,98.8552405439302));
#82363=CARTESIAN_POINT('Ctrl Pts',(68.5742657557221,706.760112339449,97.9506580860804));
#82364=CARTESIAN_POINT('Ctrl Pts',(68.0151808329475,673.394850504227,99.5018629223341));
#82365=CARTESIAN_POINT('Ctrl Pts',(68.6906630793029,673.414977845443,98.9047878029075));
#82366=CARTESIAN_POINT('Ctrl Pts',(68.6907329637246,673.394850504214,98.0032473081996));
#82367=CARTESIAN_POINT('Ctrl Pts',(68.1353783487679,640.029588276093,99.5508769219679));
#82368=CARTESIAN_POINT('Ctrl Pts',(68.8071956253259,640.030997504003,98.9541445975185));
#82369=CARTESIAN_POINT('Ctrl Pts',(68.8072001730986,640.029588276093,98.05557466696));
#82370=CARTESIAN_POINT('Ctrl Pts',(68.1332263705092,640.627119090085,99.5499985678061));
#82371=CARTESIAN_POINT('Ctrl Pts',(68.0137456499717,673.793204547633,99.501274411779));
#82372=CARTESIAN_POINT('Ctrl Pts',(67.8942035319655,706.959289448019,99.4523213250808));
#82373=CARTESIAN_POINT('Ctrl Pts',(67.7745968623189,740.125373764374,99.4031321385759));
#82374=CARTESIAN_POINT('Ctrl Pts',(68.4577985491519,740.125373764374,97.897799765561));
#82375=CARTESIAN_POINT('Ctrl Pts',(68.5735704941848,706.959289289235,97.9503433698041));
#82376=CARTESIAN_POINT('Ctrl Pts',(68.6893424406885,673.793204392753,98.0026202555698));
#82377=CARTESIAN_POINT('Ctrl Pts',(68.80511438861,640.627119090078,98.0546383469682));
#82378=CARTESIAN_POINT('Ctrl Pts',(68.1353783487637,640.029588276122,81.6665468016082));
#82379=CARTESIAN_POINT('Ctrl Pts',(68.8071956253297,640.030997504033,82.2632791260614));
#82380=CARTESIAN_POINT('Ctrl Pts',(68.8072001730985,640.029588276122,83.1618490566285));
#82381=CARTESIAN_POINT('Ctrl Pts',(68.0151808335876,673.394850502988,81.7155608018083));
#82382=CARTESIAN_POINT('Ctrl Pts',(68.6906630786356,673.414977844198,82.3126359204306));
#82383=CARTESIAN_POINT('Ctrl Pts',(68.690732963729,673.394850502972,83.2141764146837));
#82384=CARTESIAN_POINT('Ctrl Pts',(67.8949211993995,706.760112337766,81.7648064469326));
#82385=CARTESIAN_POINT('Ctrl Pts',(68.5741934539143,706.780932662796,82.3621831796554));
#82386=CARTESIAN_POINT('Ctrl Pts',(68.574265755728,706.760112337753,83.2667656382088));
#82387=CARTESIAN_POINT('Ctrl Pts',(67.7745962349126,740.125373763053,81.8142910361756));
#82388=CARTESIAN_POINT('Ctrl Pts',(68.4577939078327,740.126811780092,82.4119228399093));
#82389=CARTESIAN_POINT('Ctrl Pts',(68.4577985491564,740.125373763053,83.319624791596));
#82390=CARTESIAN_POINT('Ctrl Pts',(68.80511438861,640.627119090084,83.1627853766079));
#82391=CARTESIAN_POINT('Ctrl Pts',(68.6893424406879,673.793204392933,83.2148034676149));
#82392=CARTESIAN_POINT('Ctrl Pts',(68.5735704941839,706.95928928949,83.2670803544752));
#82393=CARTESIAN_POINT('Ctrl Pts',(68.4577985491519,740.125373764374,83.3196239580187));
#82394=CARTESIAN_POINT('Ctrl Pts',(37.9806405532016,740.12537515524,81.8142910382409));
#82395=CARTESIAN_POINT('Ctrl Pts',(37.2974428801211,740.12681317228,82.4119228419864));
#82396=CARTESIAN_POINT('Ctrl Pts',(37.2974382387975,740.12537515524,83.3196247938016));
#82397=CARTESIAN_POINT('Ctrl Pts',(37.86031558737,706.760113264802,81.7648064480086));
#82398=CARTESIAN_POINT('Ctrl Pts',(37.1810433314535,706.780933590387,82.362183181023));
#82399=CARTESIAN_POINT('Ctrl Pts',(37.1809710306022,706.76011326479,83.2667656389741));
#82400=CARTESIAN_POINT('Ctrl Pts',(37.740055951603,673.394850962724,81.7155608020926));
#82401=CARTESIAN_POINT('Ctrl Pts',(37.0645737050292,673.414978304463,82.3126359218093));
#82402=CARTESIAN_POINT('Ctrl Pts',(37.06450382097,673.394850962711,83.2141764151761));
#82403=CARTESIAN_POINT('Ctrl Pts',(37.6198584342997,640.029588267741,81.6665468015964));
#82404=CARTESIAN_POINT('Ctrl Pts',(36.9480411577352,640.030997495651,82.2632791260495));
#82405=CARTESIAN_POINT('Ctrl Pts',(36.9480366099664,640.029588267741,83.1618490566154));
#82406=CARTESIAN_POINT('Ctrl Pts',(37.2974382345426,740.12537393637,83.3196239582912));
#82407=CARTESIAN_POINT('Ctrl Pts',(37.1816662880619,706.959289046462,83.2670803533975));
#82408=CARTESIAN_POINT('Ctrl Pts',(37.0658943424057,673.793204392754,83.2148034673805));
#82409=CARTESIAN_POINT('Ctrl Pts',(36.9501223944842,640.627119090078,83.1627853766038));
#82410=CARTESIAN_POINT('Origin',(36.9483709657826,640.125373764374,82.287785267134));
#82411=CARTESIAN_POINT('Origin',(68.8068658173115,640.125373764374,82.287785267134));
#82412=CARTESIAN_POINT('Ctrl Pts',(37.2974381894958,740.125361031455,98.7804137130792));
#82413=CARTESIAN_POINT('Ctrl Pts',(37.3237628455944,747.666788861133,98.7691088591345));
#82414=CARTESIAN_POINT('Ctrl Pts',(37.350097372228,755.208210967482,98.7577876187542));
#82415=CARTESIAN_POINT('Ctrl Pts',(27.632882335034,768.384896418847,105.310835626506));
#82416=CARTESIAN_POINT('Ctrl Pts',(20.0424193057215,772.226303264399,106.668518782974));
#82417=CARTESIAN_POINT('Ctrl Pts',(13.2983736491593,777.107328840337,108.39363837514));
#82418=CARTESIAN_POINT('Ctrl Pts',(39.7898594872664,740.125360272474,101.147186527103));
#82419=CARTESIAN_POINT('Ctrl Pts',(39.8138888831648,748.116316296691,101.129143905661));
#82420=CARTESIAN_POINT('Ctrl Pts',(39.8379218896383,756.107266958529,101.11108900417));
#82421=CARTESIAN_POINT('Ctrl Pts',(32.8646428197398,769.386481710472,105.664840290342));
#82422=CARTESIAN_POINT('Ctrl Pts',(26.4798688189832,773.811767639453,107.228875594274));
#82423=CARTESIAN_POINT('Ctrl Pts',(21.001327165595,779.233378063583,109.145056107309));
#82424=CARTESIAN_POINT('Ctrl Pts',(42.7362987166043,740.12535970087,103.0351353954));
#82425=CARTESIAN_POINT('Ctrl Pts',(42.7558869385823,748.454864485732,103.011405070401));
#82426=CARTESIAN_POINT('Ctrl Pts',(42.7754757177386,756.784364143077,102.987665643325));
#82427=CARTESIAN_POINT('Ctrl Pts',(37.9535760120706,770.177419744143,105.944385861491));
#82428=CARTESIAN_POINT('Ctrl Pts',(33.008775321197,775.040599666662,107.663186445134));
#82429=CARTESIAN_POINT('Ctrl Pts',(28.8582165463779,780.867648688703,109.722662643155));
#82430=CARTESIAN_POINT('Ctrl Pts',(46.0036740674455,740.125359318221,104.339521998396));
#82431=CARTESIAN_POINT('Ctrl Pts',(46.0173362799933,748.681498353339,104.311576952405));
#82432=CARTESIAN_POINT('Ctrl Pts',(46.0309981446169,757.237632403596,104.283624962077));
#82433=CARTESIAN_POINT('Ctrl Pts',(42.9549355603365,770.721385630642,106.136637190634));
#82434=CARTESIAN_POINT('Ctrl Pts',(39.606300767173,775.876482116324,107.958615601677));
#82435=CARTESIAN_POINT('Ctrl Pts',(36.8253774496378,781.973823505111,110.113622251634));
#82436=CARTESIAN_POINT('Ctrl Pts',(49.4406462293589,740.125359126107,104.9998462381));
#82437=CARTESIAN_POINT('Ctrl Pts',(49.4475586751773,748.795282824599,104.969582372301));
#82438=CARTESIAN_POINT('Ctrl Pts',(49.4544709472461,757.465201607624,104.939312647404));
#82439=CARTESIAN_POINT('Ctrl Pts',(47.9163274999357,770.996796588943,106.233969488297));
#82440=CARTESIAN_POINT('Ctrl Pts',(46.241959498809,776.297839866931,108.107537689874));
#82441=CARTESIAN_POINT('Ctrl Pts',(44.8514979205924,782.530327410416,110.31030956155));
#82442=CARTESIAN_POINT('Ctrl Pts',(56.3145905537352,740.125359126107,104.9998462381));
#82443=CARTESIAN_POINT('Ctrl Pts',(56.3076781079168,748.7952828246,104.969582372301));
#82444=CARTESIAN_POINT('Ctrl Pts',(56.3007658357219,757.465201607906,104.939312647392));
#82445=CARTESIAN_POINT('Ctrl Pts',(57.8390930067729,770.996827303478,106.233967161403));
#82446=CARTESIAN_POINT('Ctrl Pts',(59.5132769913723,776.297839943397,108.107537701204));
#82447=CARTESIAN_POINT('Ctrl Pts',(60.9037388625016,782.530327410416,110.31030956155));
#82448=CARTESIAN_POINT('Ctrl Pts',(59.7515627156487,740.125359318221,104.339521998396));
#82449=CARTESIAN_POINT('Ctrl Pts',(59.7379005030991,748.681498353538,104.311576952411));
#82450=CARTESIAN_POINT('Ctrl Pts',(59.7242386383603,757.237632404556,104.283624962066));
#82451=CARTESIAN_POINT('Ctrl Pts',(62.8004665740107,770.721447059711,106.136632536847));
#82452=CARTESIAN_POINT('Ctrl Pts',(66.1489357522997,775.876482269256,107.958615624337));
#82453=CARTESIAN_POINT('Ctrl Pts',(68.9298593334563,781.973823505111,110.113622251634));
#82454=CARTESIAN_POINT('Ctrl Pts',(63.0189380664898,740.12535970087,103.0351353954));
#82455=CARTESIAN_POINT('Ctrl Pts',(62.9993498445084,748.454864486128,103.011405070414));
#82456=CARTESIAN_POINT('Ctrl Pts',(62.9797610652604,756.784364144573,102.98766564332));
#82457=CARTESIAN_POINT('Ctrl Pts',(67.8017893775537,770.17749653048,105.944380044258));
#82458=CARTESIAN_POINT('Ctrl Pts',(72.7464612568582,775.040599857826,107.66318647346));
#82459=CARTESIAN_POINT('Ctrl Pts',(76.8970202367163,780.867648688703,109.722662643155));
#82460=CARTESIAN_POINT('Ctrl Pts',(65.9653772958277,740.125360272474,101.147186527103));
#82461=CARTESIAN_POINT('Ctrl Pts',(65.9413478999259,748.116316297088,101.129143905674));
#82462=CARTESIAN_POINT('Ctrl Pts',(65.9173148933985,756.107266959884,101.111089004171));
#82463=CARTESIAN_POINT('Ctrl Pts',(72.8906674528,769.386543139541,105.664835636555));
#82464=CARTESIAN_POINT('Ctrl Pts',(79.2753678469458,773.811767792385,107.228875616935));
#82465=CARTESIAN_POINT('Ctrl Pts',(84.7539096174991,779.233378063583,109.145056107309));
#82466=CARTESIAN_POINT('Ctrl Pts',(68.4577985935984,740.125361031455,98.7804137130792));
#82467=CARTESIAN_POINT('Ctrl Pts',(68.4314739374997,747.666788861133,98.7691088591345));
#82468=CARTESIAN_POINT('Ctrl Pts',(68.4051394108661,755.208210967482,98.7577876187542));
#82469=CARTESIAN_POINT('Ctrl Pts',(78.12235444806,768.384896418847,105.310835626506));
#82470=CARTESIAN_POINT('Ctrl Pts',(85.7128174773725,772.226303264399,106.668518782974));
#82471=CARTESIAN_POINT('Ctrl Pts',(92.4568631339348,777.107328840337,108.39363837514));
#82472=CARTESIAN_POINT('Origin',(49.7723662973504,740.125373764374,87.0815594473992));
#82473=CARTESIAN_POINT('Origin',(55.9828704857687,740.125373764387,87.0815594474413));
#82474=CARTESIAN_POINT('Origin',(52.8776183915471,640.125373764374,82.3731046594733));
#82475=CARTESIAN_POINT('Ctrl Pts',(61.8796042537708,737.489494249471,103.141409944702));
#82476=CARTESIAN_POINT('Ctrl Pts',(61.8795904670124,737.049866679283,103.143088473426));
#82477=CARTESIAN_POINT('Ctrl Pts',(61.8462475343457,736.616839151068,103.159344525209));
#82478=CARTESIAN_POINT('Ctrl Pts',(61.7810191782632,736.190073934242,103.188826529972));
#82479=CARTESIAN_POINT('Ctrl Pts',(61.7588991064281,736.045350414904,103.198824391368));
#82480=CARTESIAN_POINT('Ctrl Pts',(61.7331118049536,735.901347140534,103.210343460409));
#82481=CARTESIAN_POINT('Ctrl Pts',(61.7037124152504,735.758051166241,103.223331663321));
#82482=CARTESIAN_POINT('Ctrl Pts',(61.7024284846643,735.751793142312,103.223898884312));
#82483=CARTESIAN_POINT('Ctrl Pts',(61.7011376103645,735.745536471594,103.224468906265));
#82484=CARTESIAN_POINT('Ctrl Pts',(61.6998397898271,735.739281153977,103.225041724595));
#82485=CARTESIAN_POINT('Ctrl Pts',(61.6473911496994,735.486485876722,103.24819095175));
#82486=CARTESIAN_POINT('Ctrl Pts',(61.5836086936033,735.235957110305,103.275902401703));
#82487=CARTESIAN_POINT('Ctrl Pts',(61.5083050324455,734.987567502205,103.307883344724));
#82488=CARTESIAN_POINT('Ctrl Pts',(61.5011236194725,734.963879565568,103.310933241045));
#82489=CARTESIAN_POINT('Ctrl Pts',(61.4938373887345,734.940211087047,103.314021982181));
#82490=CARTESIAN_POINT('Ctrl Pts',(61.4864461547222,734.916561958224,103.317149323662));
#82491=CARTESIAN_POINT('Ctrl Pts',(61.4836783635224,734.907706082395,103.31832041745));
#82492=CARTESIAN_POINT('Ctrl Pts',(61.4808959536254,734.898853893324,103.319496860068));
#82493=CARTESIAN_POINT('Ctrl Pts',(61.4780989983619,734.890005548072,103.32067860039));
#82494=CARTESIAN_POINT('Ctrl Pts',(61.3930671039362,734.621001760591,103.356605388201));
#82495=CARTESIAN_POINT('Ctrl Pts',(61.2946694414231,734.355838081379,103.397395085336));
#82496=CARTESIAN_POINT('Ctrl Pts',(61.1850563833084,734.099023223897,103.441579862578));
#82497=CARTESIAN_POINT('Ctrl Pts',(61.1804741420644,734.088287389569,103.443426953719));
#82498=CARTESIAN_POINT('Ctrl Pts',(61.1758717233044,734.077563534859,103.445280281205));
#82499=CARTESIAN_POINT('Ctrl Pts',(61.171249132145,734.066851644088,103.447139790914));
#82500=CARTESIAN_POINT('Ctrl Pts',(61.0302565652223,733.740130780315,103.503856259691));
#82501=CARTESIAN_POINT('Ctrl Pts',(60.8704863579398,733.424488578447,103.566326522464));
#82502=CARTESIAN_POINT('Ctrl Pts',(60.6921688089864,733.119635342625,103.632993159259));
#82503=CARTESIAN_POINT('Ctrl Pts',(60.5866039466843,732.93916073398,103.672460134747));
#82504=CARTESIAN_POINT('Ctrl Pts',(60.4745396709947,732.7624668695,103.713397939859));
#82505=CARTESIAN_POINT('Ctrl Pts',(60.3560312363458,732.589489897496,103.755485520567));
#82506=CARTESIAN_POINT('Ctrl Pts',(60.347596357518,732.577178201681,103.758481118682));
#82507=CARTESIAN_POINT('Ctrl Pts',(60.3391264396999,732.564883413902,103.761483211003));
#82508=CARTESIAN_POINT('Ctrl Pts',(60.3306220595767,732.552606246971,103.764491483777));
#82509=CARTESIAN_POINT('Ctrl Pts',(60.2054970233299,732.371972157826,103.808752233466));
#82510=CARTESIAN_POINT('Ctrl Pts',(60.0728060717286,732.195023121539,103.85438736651));
#82511=CARTESIAN_POINT('Ctrl Pts',(59.9344436855003,732.024134138079,103.900375897542));
#82512=CARTESIAN_POINT('Ctrl Pts',(59.9003812038466,731.982064157771,103.911697496838));
#82513=CARTESIAN_POINT('Ctrl Pts',(59.8659751152151,731.940361241186,103.923040526528));
#82514=CARTESIAN_POINT('Ctrl Pts',(59.8312538652178,731.899060345914,103.934389804448));
#82515=CARTESIAN_POINT('Ctrl Pts',(59.821130197731,731.887018252653,103.937698911001));
#82516=CARTESIAN_POINT('Ctrl Pts',(59.8109780058676,731.875007261272,103.941009221813));
#82517=CARTESIAN_POINT('Ctrl Pts',(59.8007973552984,731.863027348642,103.944320590203));
#82518=CARTESIAN_POINT('Ctrl Pts',(59.6242019572846,731.655221626935,104.001760182566));
#82519=CARTESIAN_POINT('Ctrl Pts',(59.4389525551288,731.456653794244,104.059546382713));
#82520=CARTESIAN_POINT('Ctrl Pts',(59.2452344512833,731.267076299754,104.116965618561));
#82521=CARTESIAN_POINT('Ctrl Pts',(59.2338983396636,731.255982490784,104.120325711675));
#82522=CARTESIAN_POINT('Ctrl Pts',(59.2225323659722,731.2449184774,104.123684829486));
#82523=CARTESIAN_POINT('Ctrl Pts',(59.2111365846961,731.233884354556,104.127042811653));
#82524=CARTESIAN_POINT('Ctrl Pts',(59.0732523283383,731.100376016158,104.1676730118));
#82525=CARTESIAN_POINT('Ctrl Pts',(58.9310931515999,730.971347054013,104.208111285362));
#82526=CARTESIAN_POINT('Ctrl Pts',(58.7846121092527,730.846778632298,104.248118262814));
#82527=CARTESIAN_POINT('Ctrl Pts',(58.7121076139363,730.785120342569,104.26792072778));
#82528=CARTESIAN_POINT('Ctrl Pts',(58.6385436048391,730.724555332511,104.287617604263));
#82529=CARTESIAN_POINT('Ctrl Pts',(58.5639105593564,730.665084102829,104.307180093771));
#82530=CARTESIAN_POINT('Ctrl Pts',(58.446848215123,730.571803150457,104.337863966661));
#82531=CARTESIAN_POINT('Ctrl Pts',(58.327000083616,730.481096837117,104.368256829114));
#82532=CARTESIAN_POINT('Ctrl Pts',(58.2045733181375,730.393210204539,104.398180402797));
#82533=CARTESIAN_POINT('Ctrl Pts',(58.1032142839657,730.320447486682,104.422954597523));
#82534=CARTESIAN_POINT('Ctrl Pts',(58.0000884337886,730.249616951538,104.447407062917));
#82535=CARTESIAN_POINT('Ctrl Pts',(57.8953327097942,730.180838956165,104.471439405193));
#82536=CARTESIAN_POINT('Ctrl Pts',(57.8829736747637,730.172724558004,104.474274730545));
#82537=CARTESIAN_POINT('Ctrl Pts',(57.8706004834804,730.164644069944,104.477102260258));
#82538=CARTESIAN_POINT('Ctrl Pts',(57.858213342344,730.156597577331,104.479921881953));
#82539=CARTESIAN_POINT('Ctrl Pts',(57.4392032376927,729.884415184763,104.575299012839));
#82540=CARTESIAN_POINT('Ctrl Pts',(57.0021628088544,729.649538680741,104.662096415195));
#82541=CARTESIAN_POINT('Ctrl Pts',(56.547072539648,729.450947454989,104.737462545629));
#82542=CARTESIAN_POINT('Ctrl Pts',(56.4820482176787,729.42257229367,104.748231027978));
#82543=CARTESIAN_POINT('Ctrl Pts',(56.4166554466581,729.394937957736,104.758766192916));
#82544=CARTESIAN_POINT('Ctrl Pts',(56.3508942152867,729.368041516593,104.769059779925));
#82545=CARTESIAN_POINT('Ctrl Pts',(56.3404401460206,729.363765786761,104.77069615244));
#82546=CARTESIAN_POINT('Ctrl Pts',(56.329976698201,729.35950885027,104.772326424363));
#82547=CARTESIAN_POINT('Ctrl Pts',(56.3195038552598,729.355270730177,104.773950560435));
#82548=CARTESIAN_POINT('Ctrl Pts',(56.0754485372618,729.256507122941,104.811798836003));
#82549=CARTESIAN_POINT('Ctrl Pts',(55.8262484873397,729.167949961071,104.84631974904));
#82550=CARTESIAN_POINT('Ctrl Pts',(55.5718285705163,729.089905039709,104.877053064662));
#82551=CARTESIAN_POINT('Ctrl Pts',(55.5547359345939,729.084661765349,104.879117814077));
#82552=CARTESIAN_POINT('Ctrl Pts',(55.5376197452286,729.079465921373,104.881165475601));
#82553=CARTESIAN_POINT('Ctrl Pts',(55.520479982504,729.074317593171,104.883195912995));
#82554=CARTESIAN_POINT('Ctrl Pts',(55.511843802133,729.071723514613,104.884218985709));
#82555=CARTESIAN_POINT('Ctrl Pts',(55.5032005793578,729.069141445982,104.885237709746));
#82556=CARTESIAN_POINT('Ctrl Pts',(55.4945505473297,729.066571444255,104.88625205199));
#82557=CARTESIAN_POINT('Ctrl Pts',(55.2191338591722,728.98474268781,104.918548670129));
#82558=CARTESIAN_POINT('Ctrl Pts',(54.9366264377297,728.915110056549,104.946425904167));
#82559=CARTESIAN_POINT('Ctrl Pts',(54.6542663207744,728.859520795137,104.968821856728));
#82560=CARTESIAN_POINT('Ctrl Pts',(54.6481856147052,728.858323664455,104.969304159987));
#82561=CARTESIAN_POINT('Ctrl Pts',(54.6421043009935,728.857132748841,104.969784023243));
#82562=CARTESIAN_POINT('Ctrl Pts',(54.6360223788474,728.855948047957,104.970261445308));
#82563=CARTESIAN_POINT('Ctrl Pts',(54.059132722657,728.743575401716,105.015546446442));
#82564=CARTESIAN_POINT('Ctrl Pts',(53.4767411004789,728.68707816909,105.038869503257));
#82565=CARTESIAN_POINT('Ctrl Pts',(52.8888265844506,728.686362168155,105.039162721828));
#82566=CARTESIAN_POINT('Ctrl Pts',(52.88871717262,728.686362034906,105.039162776396));
#82567=CARTESIAN_POINT('Ctrl Pts',(52.8886077603945,728.686361903625,105.039162830157));
#82568=CARTESIAN_POINT('Ctrl Pts',(52.8884983477746,728.686361774311,105.039162883111));
#82569=CARTESIAN_POINT('Ctrl Pts',(52.6528529895801,728.686083267348,105.039276930853));
#82570=CARTESIAN_POINT('Ctrl Pts',(52.4154382016483,728.694925935922,105.035647251309));
#82571=CARTESIAN_POINT('Ctrl Pts',(52.1785782191425,728.712949886856,105.028285481323));
#82572=CARTESIAN_POINT('Ctrl Pts',(52.11990863315,728.717414371435,105.026461990531));
#82573=CARTESIAN_POINT('Ctrl Pts',(52.0612730714328,728.72244239549,105.024409426725));
#82574=CARTESIAN_POINT('Ctrl Pts',(52.0027068898726,728.728035331038,105.02212778052));
#82575=CARTESIAN_POINT('Ctrl Pts',(51.999601646668,728.728331874618,105.022006805135));
#82576=CARTESIAN_POINT('Ctrl Pts',(51.9964966087559,728.728630004985,105.021885186128));
#82577=CARTESIAN_POINT('Ctrl Pts',(51.9933917816137,728.728929722308,105.021762923512));
#82578=CARTESIAN_POINT('Ctrl Pts',(51.7015274348803,728.757104173523,105.010269820423));
#82579=CARTESIAN_POINT('Ctrl Pts',(51.4134962561136,728.798950066402,104.993234307881));
#82580=CARTESIAN_POINT('Ctrl Pts',(51.1290331392348,728.854038354221,104.971030027237));
#82581=CARTESIAN_POINT('Ctrl Pts',(51.1230292865439,728.855201042617,104.970561385708));
#82582=CARTESIAN_POINT('Ctrl Pts',(51.1170270590945,728.856369626789,104.970090443887));
#82583=CARTESIAN_POINT('Ctrl Pts',(51.1110264549796,728.857544102496,104.969617205344));
#82584=CARTESIAN_POINT('Ctrl Pts',(50.760369668679,728.926176838348,104.941962605324));
#82585=CARTESIAN_POINT('Ctrl Pts',(50.4151645113868,729.014797017035,104.90646128262));
#82586=CARTESIAN_POINT('Ctrl Pts',(50.0754187952665,729.123669682408,104.86374653985));
#82587=CARTESIAN_POINT('Ctrl Pts',(49.8641924928849,729.191357866383,104.837189980799));
#82588=CARTESIAN_POINT('Ctrl Pts',(49.6550766140004,729.266875282715,104.807844895762));
#82589=CARTESIAN_POINT('Ctrl Pts',(49.4480747596083,729.350295343021,104.775860965201));
#82590=CARTESIAN_POINT('Ctrl Pts',(49.4375295289826,729.354544985022,104.774231617845));
#82591=CARTESIAN_POINT('Ctrl Pts',(49.4269898221273,729.358815150135,104.772595427554));
#82592=CARTESIAN_POINT('Ctrl Pts',(49.4164556399806,729.363105847858,104.770952414218));
#82593=CARTESIAN_POINT('Ctrl Pts',(49.0488154420395,729.512850074624,104.713611679116));
#82594=CARTESIAN_POINT('Ctrl Pts',(48.6958839685112,729.684306267898,104.649249296768));
#82595=CARTESIAN_POINT('Ctrl Pts',(48.35682671435,729.876945078386,104.579525681863));
#82596=CARTESIAN_POINT('Ctrl Pts',(48.2028987101414,729.964400831854,104.54787198103));
#82597=CARTESIAN_POINT('Ctrl Pts',(48.0518304648117,730.056223118857,104.515113321302));
#82598=CARTESIAN_POINT('Ctrl Pts',(47.9035448503638,730.15236579935,104.481405401508));
#82599=CARTESIAN_POINT('Ctrl Pts',(47.8912655859373,730.160327201411,104.478614109433));
#82600=CARTESIAN_POINT('Ctrl Pts',(47.8790055110362,730.168318239008,104.475816332613));
#82601=CARTESIAN_POINT('Ctrl Pts',(47.8667645865555,730.176338880992,104.473012161201));
#82602=CARTESIAN_POINT('Ctrl Pts',(47.6376248244894,730.326478521067,104.420520442044));
#82603=CARTESIAN_POINT('Ctrl Pts',(47.4152527800419,730.487078105255,104.365776743866));
#82604=CARTESIAN_POINT('Ctrl Pts',(47.1996985589347,730.658424243244,104.309365278181));
#82605=CARTESIAN_POINT('Ctrl Pts',(47.1874393157864,730.668169234353,104.306156981583));
#82606=CARTESIAN_POINT('Ctrl Pts',(47.1752017887997,730.677949282337,104.302943203536));
#82607=CARTESIAN_POINT('Ctrl Pts',(47.1629860410042,730.687764410395,104.299724064378));
#82608=CARTESIAN_POINT('Ctrl Pts',(46.9909866530897,730.825962746382,104.254398147855));
#82609=CARTESIAN_POINT('Ctrl Pts',(46.8239310400841,730.970725125754,104.208155267803));
#82610=CARTESIAN_POINT('Ctrl Pts',(46.6632891329359,731.120607145755,104.161798643899));
#82611=CARTESIAN_POINT('Ctrl Pts',(46.6240170718333,731.157248741663,104.150465859081));
#82612=CARTESIAN_POINT('Ctrl Pts',(46.5851282064136,731.194196104456,104.139126316237));
#82613=CARTESIAN_POINT('Ctrl Pts',(46.5466437390096,731.231427760247,104.127791806588));
#82614=CARTESIAN_POINT('Ctrl Pts',(46.5351811948828,731.242517156209,104.124415838937));
#82615=CARTESIAN_POINT('Ctrl Pts',(46.5237536592718,731.2536325835,104.12104006282));
#82616=CARTESIAN_POINT('Ctrl Pts',(46.5123616699023,731.264773517811,104.117664779297));
#82617=CARTESIAN_POINT('Ctrl Pts',(46.2843633878658,731.4877472058,104.050112149143));
#82618=CARTESIAN_POINT('Ctrl Pts',(46.0692250098231,731.721847303384,103.982410465341));
#82619=CARTESIAN_POINT('Ctrl Pts',(45.8670654960537,731.967312670592,103.915718237435));
#82620=CARTESIAN_POINT('Ctrl Pts',(45.7143536769484,732.152737843293,103.865338756135));
#82621=CARTESIAN_POINT('Ctrl Pts',(45.569047152536,732.344647880411,103.815535785514));
#82622=CARTESIAN_POINT('Ctrl Pts',(45.4311812997561,732.543135231252,103.766813632448));
#82623=CARTESIAN_POINT('Ctrl Pts',(45.4226395749163,732.555432869144,103.763794964542));
#82624=CARTESIAN_POINT('Ctrl Pts',(45.4141262937154,732.56775599969,103.760780405758));
#82625=CARTESIAN_POINT('Ctrl Pts',(45.4056414672279,732.580104644677,103.757770077436));
#82626=CARTESIAN_POINT('Ctrl Pts',(45.2628995841321,732.787848296452,103.707126739694));
#82627=CARTESIAN_POINT('Ctrl Pts',(45.1277025931781,733.004005641326,103.657461813213));
#82628=CARTESIAN_POINT('Ctrl Pts',(45.0025610201077,733.224954135452,103.610237725581));
#82629=CARTESIAN_POINT('Ctrl Pts',(44.9916710856471,733.244181276051,103.606128242165));
#82630=CARTESIAN_POINT('Ctrl Pts',(44.9808573007471,733.263444667264,103.602037248998));
#82631=CARTESIAN_POINT('Ctrl Pts',(44.9701213212071,733.282741905032,103.597965713246));
#82632=CARTESIAN_POINT('Ctrl Pts',(44.9634793631087,733.294680400649,103.595446802907));
#82633=CARTESIAN_POINT('Ctrl Pts',(44.9568671680185,733.306631773498,103.592935333914));
#82634=CARTESIAN_POINT('Ctrl Pts',(44.9502851239598,733.318595466034,103.590431533745));
#82635=CARTESIAN_POINT('Ctrl Pts',(44.8167011978043,733.561401045296,103.539616398831));
#82636=CARTESIAN_POINT('Ctrl Pts',(44.6953101553414,733.809279305862,103.491905524418));
#82637=CARTESIAN_POINT('Ctrl Pts',(44.5859555352944,734.062282106168,103.447931161836));
#82638=CARTESIAN_POINT('Ctrl Pts',(44.5813216007246,734.073003175127,103.446067735134));
#82639=CARTESIAN_POINT('Ctrl Pts',(44.57670927537,734.083733432462,103.444211017472));
#82640=CARTESIAN_POINT('Ctrl Pts',(44.5721185456116,734.094472880908,103.442361056568));
#82641=CARTESIAN_POINT('Ctrl Pts',(44.4105096418914,734.472537062695,103.377236300951));
#82642=CARTESIAN_POINT('Ctrl Pts',(44.2754369813562,734.861905124845,103.32045882081));
#82643=CARTESIAN_POINT('Ctrl Pts',(44.1681996948913,735.263402492546,103.274231479426));
#82644=CARTESIAN_POINT('Ctrl Pts',(44.1276253708223,735.415313127801,103.256740892039));
#82645=CARTESIAN_POINT('Ctrl Pts',(44.0910361632143,735.568960400019,103.240760963358));
#82646=CARTESIAN_POINT('Ctrl Pts',(44.0585035980047,735.724389967507,103.226412308778));
#82647=CARTESIAN_POINT('Ctrl Pts',(44.0571410537863,735.730899741857,103.225811351669));
#82648=CARTESIAN_POINT('Ctrl Pts',(44.0557855452771,735.737413050662,103.22521322064));
#82649=CARTESIAN_POINT('Ctrl Pts',(44.054437086145,735.743929870542,103.224617928189));
#82650=CARTESIAN_POINT('Ctrl Pts',(44.0251843913813,735.885302002801,103.211703997045));
#82651=CARTESIAN_POINT('Ctrl Pts',(43.9994306999042,736.027799875058,103.200209958833));
#82652=CARTESIAN_POINT('Ctrl Pts',(43.9772758840869,736.170913964547,103.19020770992));
#82653=CARTESIAN_POINT('Ctrl Pts',(43.9551210682695,736.314028054035,103.180205461008));
#82654=CARTESIAN_POINT('Ctrl Pts',(43.9365652126234,736.457757751576,103.17169511312));
#82655=CARTESIAN_POINT('Ctrl Pts',(43.9216507621959,736.6015839673,103.164724639108));
#82656=CARTESIAN_POINT('Ctrl Pts',(43.9063925566538,736.74872515581,103.157593506404));
#82657=CARTESIAN_POINT('Ctrl Pts',(43.8949033349003,736.896283772816,103.152054681657));
#82658=CARTESIAN_POINT('Ctrl Pts',(43.8872145218739,737.044266546973,103.148150887835));
#82659=CARTESIAN_POINT('Ctrl Pts',(43.8795257088476,737.192249321131,103.144247094013));
#82660=CARTESIAN_POINT('Ctrl Pts',(43.8756371967118,737.340656799868,103.141978216393));
#82661=CARTESIAN_POINT('Ctrl Pts',(43.8756325293234,737.489494249471,103.141409944702));
#82662=CARTESIAN_POINT('Ctrl Pts',(15.7871623891209,777.809475003739,108.316029302452));
#82663=CARTESIAN_POINT('Ctrl Pts',(15.7828592118407,777.701521672783,108.603706188413));
#82664=CARTESIAN_POINT('Ctrl Pts',(15.9637713943952,777.935743349876,108.686420476388));
#82665=CARTESIAN_POINT('Ctrl Pts',(17.1698777637827,776.859899239153,107.980583473227));
#82666=CARTESIAN_POINT('Ctrl Pts',(17.1658604835569,776.751736583642,108.268251210865));
#82667=CARTESIAN_POINT('Ctrl Pts',(17.339905451348,776.990753940025,108.352595674445));
#82668=CARTESIAN_POINT('Ctrl Pts',(18.5839869581375,775.970726517344,107.663779924925));
#82669=CARTESIAN_POINT('Ctrl Pts',(18.5775897517564,775.864254818958,107.951030268325));
#82670=CARTESIAN_POINT('Ctrl Pts',(18.7474923713148,776.104630519359,108.036859377413));
#82671=CARTESIAN_POINT('Ctrl Pts',(21.4288123221645,774.335785651368,107.073001766124));
#82672=CARTESIAN_POINT('Ctrl Pts',(21.4233211378568,774.229827357484,107.357671335684));
#82673=CARTESIAN_POINT('Ctrl Pts',(21.5778907227146,774.475289361177,107.448008465933));
#82674=CARTESIAN_POINT('Ctrl Pts',(22.8577706644518,773.585932431183,106.799533790745));
#82675=CARTESIAN_POINT('Ctrl Pts',(22.8530525134455,773.479965851209,107.082603184221));
#82676=CARTESIAN_POINT('Ctrl Pts',(22.998957483572,773.728099094563,107.175447339692));
#82677=CARTESIAN_POINT('Ctrl Pts',(25.7716023470914,772.18478907632,106.316079490884));
#82678=CARTESIAN_POINT('Ctrl Pts',(25.7641886004944,772.080644591425,106.598115865289));
#82679=CARTESIAN_POINT('Ctrl Pts',(25.8953600097582,772.333644099618,106.694294509729));
#82680=CARTESIAN_POINT('Ctrl Pts',(27.2563198999602,771.533314665731,106.106856054866));
#82681=CARTESIAN_POINT('Ctrl Pts',(27.251586921119,771.427992638627,106.388475167844));
#82682=CARTESIAN_POINT('Ctrl Pts',(27.3707066300181,771.686096682895,106.486434551977));
#82683=CARTESIAN_POINT('Ctrl Pts',(30.2816206589377,770.320021916191,105.779318909421));
#82684=CARTESIAN_POINT('Ctrl Pts',(30.2707752197921,770.215782961016,106.063698689885));
#82685=CARTESIAN_POINT('Ctrl Pts',(30.3762932668855,770.482514096521,106.162191817292));
#82686=CARTESIAN_POINT('Ctrl Pts',(31.8218958654417,769.758147156968,105.661459556942));
#82687=CARTESIAN_POINT('Ctrl Pts',(31.8149887412563,769.651659865527,105.948249651328));
#82688=CARTESIAN_POINT('Ctrl Pts',(31.906520346948,769.926326252646,106.04624309019));
#82689=CARTESIAN_POINT('Ctrl Pts',(34.1753342422536,768.982641272906,105.558519931726));
#82690=CARTESIAN_POINT('Ctrl Pts',(34.1546169585506,768.877637047113,105.851399684763));
#82691=CARTESIAN_POINT('Ctrl Pts',(34.2448266873315,769.16068073807,105.946414538527));
#82692=CARTESIAN_POINT('Ctrl Pts',(34.9686229099064,768.734994611625,105.536323043755));
#82693=CARTESIAN_POINT('Ctrl Pts',(34.947012343891,768.629165255762,105.831524846475));
#82694=CARTESIAN_POINT('Ctrl Pts',(35.0332146223605,768.916496206878,105.92529234965));
#82695=CARTESIAN_POINT('Ctrl Pts',(36.5574672658585,768.267097781214,105.514313342663));
#82696=CARTESIAN_POINT('Ctrl Pts',(36.5323909593653,768.159538131973,105.814595596256));
#82697=CARTESIAN_POINT('Ctrl Pts',(36.6126042630737,768.455745087938,105.9054342665));
#82698=CARTESIAN_POINT('Ctrl Pts',(37.3535733947877,768.046590379996,105.514400128375));
#82699=CARTESIAN_POINT('Ctrl Pts',(37.3276962200189,767.937856780718,105.817623550911));
#82700=CARTESIAN_POINT('Ctrl Pts',(37.4041927108883,768.238916686194,105.906602202054));
#82701=CARTESIAN_POINT('Ctrl Pts',(39.7470698872341,767.426930329457,105.540910201916));
#82702=CARTESIAN_POINT('Ctrl Pts',(39.731369122651,767.310558107932,105.853533619489));
#82703=CARTESIAN_POINT('Ctrl Pts',(39.7851879275338,767.63026353926,105.936276431145));
#82704=CARTESIAN_POINT('Ctrl Pts',(41.3501040612565,767.069220619382,105.593941179774));
#82705=CARTESIAN_POINT('Ctrl Pts',(41.3351409056594,766.950282574883,105.914278418857));
#82706=CARTESIAN_POINT('Ctrl Pts',(41.3808256323271,767.280032673843,105.991321543562));
#82707=CARTESIAN_POINT('Ctrl Pts',(44.5738166034429,766.480398389306,105.718196950375));
#82708=CARTESIAN_POINT('Ctrl Pts',(44.5615972127706,766.353558912604,106.052595889704));
#82709=CARTESIAN_POINT('Ctrl Pts',(44.5923634296551,766.704367233879,106.118970464199));
#82710=CARTESIAN_POINT('Ctrl Pts',(46.1946605516339,766.249522535964,105.78850353175));
#82711=CARTESIAN_POINT('Ctrl Pts',(46.1795127759105,766.120994876181,106.129399020199));
#82712=CARTESIAN_POINT('Ctrl Pts',(46.2083274763445,766.479215938456,106.190660953083));
#82713=CARTESIAN_POINT('Ctrl Pts',(49.4574855150692,765.934275375266,105.892868516371));
#82714=CARTESIAN_POINT('Ctrl Pts',(49.4546256912783,765.799410469687,106.243931276121));
#82715=CARTESIAN_POINT('Ctrl Pts',(49.463598562072,766.171873580197,106.296940787133));
#82716=CARTESIAN_POINT('Ctrl Pts',(51.099964532512,765.850120640634,105.926129110136));
#82717=CARTESIAN_POINT('Ctrl Pts',(51.0910382647445,765.714667095532,106.279827188356));
#82718=CARTESIAN_POINT('Ctrl Pts',(51.102948592707,766.089969488739,106.330715610695));
#82719=CARTESIAN_POINT('Ctrl Pts',(53.5812393839398,765.844168786106,105.928376604794));
#82720=CARTESIAN_POINT('Ctrl Pts',(53.5850396314526,765.708577852611,106.282289428977));
#82721=CARTESIAN_POINT('Ctrl Pts',(53.5800634567942,766.084172742205,106.33299999645));
#82722=CARTESIAN_POINT('Ctrl Pts',(54.411880554151,765.86217585081,105.92146709385));
#82723=CARTESIAN_POINT('Ctrl Pts',(54.4179864165666,765.726919467555,106.274755736027));
#82724=CARTESIAN_POINT('Ctrl Pts',(54.4092728216049,766.101706740817,106.325979308644));
#82725=CARTESIAN_POINT('Ctrl Pts',(56.0769319609754,765.93844695356,105.893509488094));
#82726=CARTESIAN_POINT('Ctrl Pts',(56.0911552800048,765.80490169404,106.244116471363));
#82727=CARTESIAN_POINT('Ctrl Pts',(56.0712773854469,766.176009378732,106.297551934537));
#82728=CARTESIAN_POINT('Ctrl Pts',(56.9052458395736,765.996396478854,105.872599600657));
#82729=CARTESIAN_POINT('Ctrl Pts',(56.9214628881391,765.863871224801,106.221288358478));
#82730=CARTESIAN_POINT('Ctrl Pts',(56.8979108032853,766.232465009037,106.276287758478));
#82731=CARTESIAN_POINT('Ctrl Pts',(59.3783911870065,766.226174100899,105.795738329226));
#82732=CARTESIAN_POINT('Ctrl Pts',(59.3931930839897,766.097281081923,106.13732691571));
#82733=CARTESIAN_POINT('Ctrl Pts',(59.3652210008115,766.456444148206,106.198036053344));
#82734=CARTESIAN_POINT('Ctrl Pts',(61.0112655596819,766.453952146128,105.725310064261));
#82735=CARTESIAN_POINT('Ctrl Pts',(61.0230698567076,766.326720958392,106.060446968748));
#82736=CARTESIAN_POINT('Ctrl Pts',(60.9932650699687,766.678550277211,106.126240847154));
#82737=CARTESIAN_POINT('Ctrl Pts',(64.2501406514068,767.036718468604,105.599412980091));
#82738=CARTESIAN_POINT('Ctrl Pts',(64.2650219723685,766.917450919191,105.920451345278));
#82739=CARTESIAN_POINT('Ctrl Pts',(64.220087663195,767.248223944424,105.99697671647));
#82740=CARTESIAN_POINT('Ctrl Pts',(65.8563267979194,767.391477721513,105.544877839256));
#82741=CARTESIAN_POINT('Ctrl Pts',(65.8720329977456,767.274797690945,105.858171285359));
#82742=CARTESIAN_POINT('Ctrl Pts',(65.8189446590444,767.595514746263,105.940437566371));
#82743=CARTESIAN_POINT('Ctrl Pts',(69.0465943635938,768.210053193601,105.505173430379));
#82744=CARTESIAN_POINT('Ctrl Pts',(69.057730705995,768.098890004912,105.806099333311));
#82745=CARTESIAN_POINT('Ctrl Pts',(68.9922854012551,768.399315245165,105.896535263205));
#82746=CARTESIAN_POINT('Ctrl Pts',(70.6305164306212,768.673731102989,105.52051972908));
#82747=CARTESIAN_POINT('Ctrl Pts',(70.644943034338,768.565368486617,105.815477540819));
#82748=CARTESIAN_POINT('Ctrl Pts',(70.5668278970275,768.855706852748,105.909665906585));
#82749=CARTESIAN_POINT('Ctrl Pts',(73.7781993814608,769.703475797329,105.65147939074));
#82750=CARTESIAN_POINT('Ctrl Pts',(73.785156923816,769.596881243375,105.938580705688));
#82751=CARTESIAN_POINT('Ctrl Pts',(73.6945831500112,769.872258227292,106.036461068767));
#82752=CARTESIAN_POINT('Ctrl Pts',(75.3459978283876,770.271662966608,105.767902085136));
#82753=CARTESIAN_POINT('Ctrl Pts',(75.3568953147369,770.167357396806,106.052433260717));
#82754=CARTESIAN_POINT('Ctrl Pts',(75.2521594979732,770.434601013187,106.150924723143));
#82755=CARTESIAN_POINT('Ctrl Pts',(78.4094844858746,771.494821615298,106.09492936714));
#82756=CARTESIAN_POINT('Ctrl Pts',(78.414133676991,771.389464389472,106.376558566266));
#82757=CARTESIAN_POINT('Ctrl Pts',(78.2956674291651,771.647853007347,106.474594343472));
#82758=CARTESIAN_POINT('Ctrl Pts',(79.9105925242892,772.151408559331,106.30497861231));
#82759=CARTESIAN_POINT('Ctrl Pts',(79.9180899961921,772.047304534831,106.587006825142));
#82760=CARTESIAN_POINT('Ctrl Pts',(79.7872875510178,772.300446180308,106.683256580676));
#82761=CARTESIAN_POINT('Ctrl Pts',(82.8525638161391,773.562668707001,106.791100861697));
#82762=CARTESIAN_POINT('Ctrl Pts',(82.8572888565633,773.456721640073,107.074131615572));
#82763=CARTESIAN_POINT('Ctrl Pts',(82.7116297096421,773.704923756985,107.16704469137));
#82764=CARTESIAN_POINT('Ctrl Pts',(84.2932699293538,774.317537975393,107.066385590134));
#82765=CARTESIAN_POINT('Ctrl Pts',(84.298806954681,774.211617420184,107.351034210259));
#82766=CARTESIAN_POINT('Ctrl Pts',(84.1443675648991,774.457105296261,107.44141406158));
#82767=CARTESIAN_POINT('Ctrl Pts',(87.1578941883669,775.962233307482,107.660731979537));
#82768=CARTESIAN_POINT('Ctrl Pts',(87.1643322846048,775.855786966959,107.947981090005));
#82769=CARTESIAN_POINT('Ctrl Pts',(86.9944506659982,776.09616644414,108.033821604836));
#82770=CARTESIAN_POINT('Ctrl Pts',(88.5799295501548,776.856148047137,107.979260687991));
#82771=CARTESIAN_POINT('Ctrl Pts',(88.5839431068136,776.747982826875,108.26692813987));
#82772=CARTESIAN_POINT('Ctrl Pts',(88.4099278287071,776.987021304641,108.351279441427));
#82773=CARTESIAN_POINT('Ctrl Pts',(89.9686252865639,777.809853363037,108.316162883459));
#82774=CARTESIAN_POINT('Ctrl Pts',(89.9729284260661,777.701900006605,108.603839733057));
#82775=CARTESIAN_POINT('Ctrl Pts',(89.792013646137,777.936119871348,108.686553408827));
#82776=CARTESIAN_POINT('Ctrl Pts',(16.0893414574741,777.849661935782,108.656004008529));
#82777=CARTESIAN_POINT('Ctrl Pts',(17.4250549733219,776.937175921057,108.333500400375));
#82778=CARTESIAN_POINT('Ctrl Pts',(18.78943598776,776.080497252125,108.028135460872));
#82779=CARTESIAN_POINT('Ctrl Pts',(21.5746899384678,774.476977569018,107.448620490165));
#82780=CARTESIAN_POINT('Ctrl Pts',(22.9955938975846,773.729725682315,107.176024929388));
#82781=CARTESIAN_POINT('Ctrl Pts',(25.8934985433138,772.334397900271,106.694534848672));
#82782=CARTESIAN_POINT('Ctrl Pts',(27.3704856350576,771.686064132665,106.486387701304));
#82783=CARTESIAN_POINT('Ctrl Pts',(30.3808686758457,770.480671981398,106.161721933409));
#82784=CARTESIAN_POINT('Ctrl Pts',(31.9142587560915,769.923462674222,106.04565513536));
#82785=CARTESIAN_POINT('Ctrl Pts',(34.2576802253298,769.15654052208,105.945964322096));
#82786=CARTESIAN_POINT('Ctrl Pts',(35.0478636523885,768.911965834192,105.924938629994));
#82787=CARTESIAN_POINT('Ctrl Pts',(36.6303099055664,768.450709294541,105.905345473651));
#82788=CARTESIAN_POINT('Ctrl Pts',(37.4232324031954,768.233741281857,105.906677444993));
#82789=CARTESIAN_POINT('Ctrl Pts',(39.8074008004172,767.625011695292,105.936830078864));
#82790=CARTESIAN_POINT('Ctrl Pts',(41.4040107345446,767.275207462003,105.99215472231));
#82791=CARTESIAN_POINT('Ctrl Pts',(44.6144245059283,766.700953763019,106.119909037887));
#82792=CARTESIAN_POINT('Ctrl Pts',(46.2282835033238,766.476775822931,106.191423389735));
#82793=CARTESIAN_POINT('Ctrl Pts',(49.4766332220309,766.171063900259,106.297232632525));
#82794=CARTESIAN_POINT('Ctrl Pts',(51.1111753031026,766.089792523124,106.330747957394));
#82795=CARTESIAN_POINT('Ctrl Pts',(53.5801372868367,766.084145679822,106.332973315604));
#82796=CARTESIAN_POINT('Ctrl Pts',(54.4064440289033,766.101597865186,106.325986242852));
#82797=CARTESIAN_POINT('Ctrl Pts',(56.0628277007067,766.175473742229,106.297718036996));
#82798=CARTESIAN_POINT('Ctrl Pts',(56.8869548009683,766.231598277818,106.276572947795));
#82799=CARTESIAN_POINT('Ctrl Pts',(59.3478646853131,766.454407478501,106.198677774663));
#82800=CARTESIAN_POINT('Ctrl Pts',(60.9731755266814,766.675510114496,106.127094439787));
#82801=CARTESIAN_POINT('Ctrl Pts',(64.1977890163342,767.243651270107,105.997794517429));
#82802=CARTESIAN_POINT('Ctrl Pts',(65.7971573448773,767.590423963616,105.941009947412));
#82803=CARTESIAN_POINT('Ctrl Pts',(68.9737932300432,768.394076466195,105.896488785951));
#82804=CARTESIAN_POINT('Ctrl Pts',(70.5510930280338,768.850829333817,105.909275429647));
#82805=CARTESIAN_POINT('Ctrl Pts',(73.6851181293508,769.868817507906,106.035790294461));
#82806=CARTESIAN_POINT('Ctrl Pts',(75.2463606945133,770.432304387266,106.15035314656));
#82807=CARTESIAN_POINT('Ctrl Pts',(78.2952107601735,771.647525172689,106.474453855161));
#82808=CARTESIAN_POINT('Ctrl Pts',(79.7886644455849,772.300974854605,106.683420921211));
#82809=CARTESIAN_POINT('Ctrl Pts',(82.7147733195567,773.706431016707,107.167578148489));
#82810=CARTESIAN_POINT('Ctrl Pts',(84.1474203625525,774.458709583747,107.441995642768));
#82811=CARTESIAN_POINT('Ctrl Pts',(86.9521465126742,776.071846592112,108.025029756641));
#82812=CARTESIAN_POINT('Ctrl Pts',(88.3242703519922,776.933137527661,108.332073090122));
#82813=CARTESIAN_POINT('Ctrl Pts',(89.6658953259192,777.849661935669,108.656004008489));
#82814=CARTESIAN_POINT('Ctrl Pts',(88.5738513044493,778.181878049576,108.773653956565));
#82815=CARTESIAN_POINT('Ctrl Pts',(83.8434238890686,785.148186360683,109.114308839679));
#82816=CARTESIAN_POINT('Ctrl Pts',(78.9738504955049,791.633263347778,111.406354474977));
#82817=CARTESIAN_POINT('Ctrl Pts',(87.9149776371255,777.742127291872,108.618238413247));
#82818=CARTESIAN_POINT('Ctrl Pts',(83.2725051483006,784.767138659038,108.979633688774));
#82819=CARTESIAN_POINT('Ctrl Pts',(78.4934733905516,791.312643755968,111.293036662796));
#82820=CARTESIAN_POINT('Ctrl Pts',(87.2882571412732,777.341259228713,108.47646064782));
#82821=CARTESIAN_POINT('Ctrl Pts',(82.7150583236353,784.410224910016,108.853488293304));
#82822=CARTESIAN_POINT('Ctrl Pts',(78.0073420881403,791.00099847986,111.182890677438));
#82823=CARTESIAN_POINT('Ctrl Pts',(86.0362516952194,776.570985822674,108.20271274568));
#82824=CARTESIAN_POINT('Ctrl Pts',(81.604148087287,783.72393950889,108.610931811799));
#82825=CARTESIAN_POINT('Ctrl Pts',(77.0417726934468,790.401519506022,110.971014524206));
#82826=CARTESIAN_POINT('Ctrl Pts',(85.4124909221331,776.201653664868,108.070824267304));
#82827=CARTESIAN_POINT('Ctrl Pts',(81.0515796632365,783.39441895453,108.494468098035));
#82828=CARTESIAN_POINT('Ctrl Pts',(76.5625713693442,790.113291377843,110.869144951265));
#82829=CARTESIAN_POINT('Ctrl Pts',(84.0792612027146,775.445672384301,107.800616740213));
#82830=CARTESIAN_POINT('Ctrl Pts',(79.8976647185069,782.734867224681,108.261360200414));
#82831=CARTESIAN_POINT('Ctrl Pts',(75.5934183244409,789.553692399723,110.671363737892));
#82832=CARTESIAN_POINT('Ctrl Pts',(83.3720539242186,775.059903900003,107.6624783517));
#82833=CARTESIAN_POINT('Ctrl Pts',(79.2974971757814,782.405212171218,108.144848950272));
#82834=CARTESIAN_POINT('Ctrl Pts',(75.1035387365079,789.2822084411,110.575412121025));
#82835=CARTESIAN_POINT('Ctrl Pts',(82.1654585207305,774.436382978644,107.442289651568));
#82836=CARTESIAN_POINT('Ctrl Pts',(78.3167674194848,781.898680004742,107.965823343682));
#82837=CARTESIAN_POINT('Ctrl Pts',(74.3552830957901,788.896051377323,110.438931148736));
#82838=CARTESIAN_POINT('Ctrl Pts',(81.7385250148577,774.220948387259,107.366715554214));
#82839=CARTESIAN_POINT('Ctrl Pts',(77.976199525919,781.727802549079,107.905429469083));
#82840=CARTESIAN_POINT('Ctrl Pts',(74.1035832785893,788.77090952714,110.394701784601));
#82841=CARTESIAN_POINT('Ctrl Pts',(80.8079497421642,773.765682033111,107.209530118557));
#82842=CARTESIAN_POINT('Ctrl Pts',(77.2531183817485,781.378821137396,107.78208763009));
#82843=CARTESIAN_POINT('Ctrl Pts',(73.5938901808835,788.530494361478,110.309730930405));
#82844=CARTESIAN_POINT('Ctrl Pts',(80.3034332507445,773.525337785074,107.127690866966));
#82845=CARTESIAN_POINT('Ctrl Pts',(76.8698599874927,781.200311547758,107.718996301082));
#82846=CARTESIAN_POINT('Ctrl Pts',(73.3353014539425,788.414941956932,110.268890800825));
#82847=CARTESIAN_POINT('Ctrl Pts',(79.1770575653734,773.008703161511,106.957283814441));
#82848=CARTESIAN_POINT('Ctrl Pts',(76.0409616383071,780.833266548411,107.589270179072));
#82849=CARTESIAN_POINT('Ctrl Pts',(72.8120842823484,788.199188971456,110.192636395573));
#82850=CARTESIAN_POINT('Ctrl Pts',(78.5568496943687,772.73295592847,106.868769852518));
#82851=CARTESIAN_POINT('Ctrl Pts',(75.5965095740638,780.645113872109,107.522770656896));
#82852=CARTESIAN_POINT('Ctrl Pts',(72.5482099436597,788.099250448862,110.157314740184));
#82853=CARTESIAN_POINT('Ctrl Pts',(77.4911048517436,772.281537917275,106.732807228027));
#82854=CARTESIAN_POINT('Ctrl Pts',(74.8588910374908,780.353097020446,107.419562020953));
#82855=CARTESIAN_POINT('Ctrl Pts',(72.1475773980314,787.966232967754,110.110301861602));
#82856=CARTESIAN_POINT('Ctrl Pts',(77.112950447673,772.124710631934,106.686988491034));
#82857=CARTESIAN_POINT('Ctrl Pts',(74.6010028008535,780.254108042824,107.384575966848));
#82858=CARTESIAN_POINT('Ctrl Pts',(72.0132232095821,787.924731631362,110.095633885088));
#82859=CARTESIAN_POINT('Ctrl Pts',(76.3037627940189,771.798066830141,106.59588420746));
#82860=CARTESIAN_POINT('Ctrl Pts',(74.0574741870081,780.053376333228,107.313630588775));
#82861=CARTESIAN_POINT('Ctrl Pts',(71.7425915643583,787.848467048447,110.068679401009));
#82862=CARTESIAN_POINT('Ctrl Pts',(75.8722540562148,771.628097477578,106.550578461549));
#82863=CARTESIAN_POINT('Ctrl Pts',(73.7715798531127,779.951560540875,107.277645442728));
#82864=CARTESIAN_POINT('Ctrl Pts',(71.6063114236022,787.813713205088,110.05639621684));
#82865=CARTESIAN_POINT('Ctrl Pts',(74.9599655844954,771.279645950925,106.46373018065));
#82866=CARTESIAN_POINT('Ctrl Pts',(73.1736720938016,779.748117469616,107.205741777664));
#82867=CARTESIAN_POINT('Ctrl Pts',(71.3315223578334,787.752013970454,110.034589619675));
#82868=CARTESIAN_POINT('Ctrl Pts',(74.4788746718596,771.101147210338,106.422253178248));
#82869=CARTESIAN_POINT('Ctrl Pts',(72.8614810857166,779.646493791832,107.169824531404));
#82870=CARTESIAN_POINT('Ctrl Pts',(71.1930079058333,787.725087942696,110.0250730504));
#82871=CARTESIAN_POINT('Ctrl Pts',(73.496993747821,770.748822516026,106.347734551176));
#82872=CARTESIAN_POINT('Ctrl Pts',(72.2258102743165,779.450406994966,107.100520822657));
#82873=CARTESIAN_POINT('Ctrl Pts',(70.9135678426254,787.679683282299,110.009025507111));
#82874=CARTESIAN_POINT('Ctrl Pts',(72.9972861502008,770.575443021603,106.314830495441));
#82875=CARTESIAN_POINT('Ctrl Pts',(71.9028611425821,779.356169439202,107.067214081826));
#82876=CARTESIAN_POINT('Ctrl Pts',(70.7726394832558,787.661214277631,110.002497935947));
#82877=CARTESIAN_POINT('Ctrl Pts',(72.0255934206576,770.249325984699,106.260112822916));
#82878=CARTESIAN_POINT('Ctrl Pts',(71.2697212485457,779.18247231621,107.005823641377));
#82879=CARTESIAN_POINT('Ctrl Pts',(70.4884658286637,787.632393555839,109.992311717692));
#82880=CARTESIAN_POINT('Ctrl Pts',(71.5536373679969,770.096525865296,106.238228677174));
#82881=CARTESIAN_POINT('Ctrl Pts',(70.9594066510123,779.102962134233,106.977722052762));
#82882=CARTESIAN_POINT('Ctrl Pts',(70.344949670124,787.622012052336,109.988642543087));
#82883=CARTESIAN_POINT('Ctrl Pts',(70.6681422002458,769.818470054936,106.204087028555));
#82884=CARTESIAN_POINT('Ctrl Pts',(70.3679066564915,778.961275090666,106.927645057479));
#82885=CARTESIAN_POINT('Ctrl Pts',(70.0571733336436,787.608223198133,109.983769095454));
#82886=CARTESIAN_POINT('Ctrl Pts',(70.2562198335574,769.693596329677,106.191779838153));
#82887=CARTESIAN_POINT('Ctrl Pts',(70.0879120630911,778.899274121479,106.905731817103));
#82888=CARTESIAN_POINT('Ctrl Pts',(69.9136476562238,787.604807391686,109.982561833879));
#82889=CARTESIAN_POINT('Ctrl Pts',(69.1075565099042,769.354665279132,106.164335933203));
#82890=CARTESIAN_POINT('Ctrl Pts',(69.2923238767039,778.734902877756,106.847637457941));
#82891=CARTESIAN_POINT('Ctrl Pts',(69.4839004401929,787.602523253,109.981754541982));
#82892=CARTESIAN_POINT('Ctrl Pts',(68.4559672015376,769.17518744114,106.158151845178));
#82893=CARTESIAN_POINT('Ctrl Pts',(68.8203566681227,778.653557517144,106.818887255123));
#82894=CARTESIAN_POINT('Ctrl Pts',(69.1984902703543,787.611441170196,109.984906435664));
#82895=CARTESIAN_POINT('Ctrl Pts',(67.2950904119738,768.868275425604,106.154657878201));
#82896=CARTESIAN_POINT('Ctrl Pts',(67.9491799021657,778.522040766329,106.772404785367));
#82897=CARTESIAN_POINT('Ctrl Pts',(68.6288985832237,787.641067693366,109.995377451391));
#82898=CARTESIAN_POINT('Ctrl Pts',(66.7851640278802,768.740976392566,106.157639466173));
#82899=CARTESIAN_POINT('Ctrl Pts',(67.549698766656,778.472018174541,106.754725108905));
#82900=CARTESIAN_POINT('Ctrl Pts',(68.3447257023204,787.661859177433,110.002725865358));
#82901=CARTESIAN_POINT('Ctrl Pts',(65.8509965373988,768.516718306576,106.167242031038));
#82902=CARTESIAN_POINT('Ctrl Pts',(66.794624228746,778.390000059683,106.725737131935));
#82903=CARTESIAN_POINT('Ctrl Pts',(67.7770957888854,787.710311740259,110.019850640494));
#82904=CARTESIAN_POINT('Ctrl Pts',(65.4272737571728,768.420031205163,106.173980523856));
#82905=CARTESIAN_POINT('Ctrl Pts',(66.4393274595632,778.358174956261,106.714489063581));
#82906=CARTESIAN_POINT('Ctrl Pts',(67.4936435311311,787.738018639783,110.029643196272));
#82907=CARTESIAN_POINT('Ctrl Pts',(64.6361872575302,768.246354011442,106.188976594821));
#82908=CARTESIAN_POINT('Ctrl Pts',(65.7576292395194,778.305889398473,106.69600957831));
#82909=CARTESIAN_POINT('Ctrl Pts',(66.9271483164738,787.797360269187,110.050616535977));
#82910=CARTESIAN_POINT('Ctrl Pts',(64.2691108829029,768.169487022388,106.197273275863));
#82911=CARTESIAN_POINT('Ctrl Pts',(65.4313953294225,778.285505642855,106.68880526938));
#82912=CARTESIAN_POINT('Ctrl Pts',(66.6441075879408,787.829016383441,110.061804877866));
#82913=CARTESIAN_POINT('Ctrl Pts',(63.2269996462562,767.959563358908,106.222950194576));
#82914=CARTESIAN_POINT('Ctrl Pts',(64.4828994295554,778.235670861743,106.671191971545));
#82915=CARTESIAN_POINT('Ctrl Pts',(65.7953010971783,787.927014271945,110.096440647505));
#82916=CARTESIAN_POINT('Ctrl Pts',(62.6097075508497,767.846709151702,106.241045178976));
#82917=CARTESIAN_POINT('Ctrl Pts',(63.8904323523067,778.21725275906,106.664682390869));
#82918=CARTESIAN_POINT('Ctrl Pts',(65.2298349915925,787.99623168283,110.120904422542));
#82919=CARTESIAN_POINT('Ctrl Pts',(61.4590052374346,767.651437052883,106.275936414629));
#82920=CARTESIAN_POINT('Ctrl Pts',(62.748362851604,778.194057714248,106.656484477185));
#82921=CARTESIAN_POINT('Ctrl Pts',(64.0987686108381,788.133378954464,110.169376908831));
#82922=CARTESIAN_POINT('Ctrl Pts',(60.926821211362,767.569468956964,106.292826110456));
#82923=CARTESIAN_POINT('Ctrl Pts',(62.1994558233975,778.18956414367,106.654896297299));
#82924=CARTESIAN_POINT('Ctrl Pts',(63.5331799072629,788.201419861245,110.193424867509));
#82925=CARTESIAN_POINT('Ctrl Pts',(59.4092177133849,767.354659251409,106.340244800808));
#82926=CARTESIAN_POINT('Ctrl Pts',(60.592599303396,778.186156421342,106.65369189296));
#82927=CARTESIAN_POINT('Ctrl Pts',(61.8354805457418,788.396586698252,110.262403431342));
#82928=CARTESIAN_POINT('Ctrl Pts',(58.5007011856502,767.252229641939,106.36749379104));
#82929=CARTESIAN_POINT('Ctrl Pts',(59.5741477724552,778.196813737576,106.657458549082));
#82930=CARTESIAN_POINT('Ctrl Pts',(60.7023962859907,788.514369519008,110.304031865479));
#82931=CARTESIAN_POINT('Ctrl Pts',(56.7697487845424,767.09500330296,106.41105217881));
#82932=CARTESIAN_POINT('Ctrl Pts',(57.579404677287,778.218730226506,106.665204577855));
#82933=CARTESIAN_POINT('Ctrl Pts',(58.4317005834261,788.706490328621,110.371933860166));
#82934=CARTESIAN_POINT('Ctrl Pts',(55.9515831390504,767.041203218348,106.427412017473));
#82935=CARTESIAN_POINT('Ctrl Pts',(56.6066138022518,778.230530097354,106.669375051334));
#82936=CARTESIAN_POINT('Ctrl Pts',(57.2963394038202,788.780952969837,110.398251477078));
#82937=CARTESIAN_POINT('Ctrl Pts',(54.354843997501,766.971158844204,106.448937284848));
#82938=CARTESIAN_POINT('Ctrl Pts',(54.6828513340098,778.246666962928,106.675078365885));
#82939=CARTESIAN_POINT('Ctrl Pts',(55.0285659862819,788.879478327426,110.433073672139));
#82940=CARTESIAN_POINT('Ctrl Pts',(53.5768772428552,766.955076749816,106.454128934655));
#82941=CARTESIAN_POINT('Ctrl Pts',(53.7321495971161,778.251150846421,106.676663121963));
#82942=CARTESIAN_POINT('Ctrl Pts',(53.8957206869194,788.90368428377,110.44162887614));
#82943=CARTESIAN_POINT('Ctrl Pts',(52.0222390159911,766.957423826263,106.453384325924));
#82944=CARTESIAN_POINT('Ctrl Pts',(51.8322941590422,778.250536615474,106.67644603184));
#82945=CARTESIAN_POINT('Ctrl Pts',(51.6321856100123,788.900233488439,110.44040924831));
#82946=CARTESIAN_POINT('Ctrl Pts',(51.2442658197987,766.975858807195,106.447448325547));
#82947=CARTESIAN_POINT('Ctrl Pts',(50.8826289700665,778.245446491303,106.674647009886));
#82948=CARTESIAN_POINT('Ctrl Pts',(50.5014953947721,788.872587267927,110.430638138547));
#82949=CARTESIAN_POINT('Ctrl Pts',(49.6481191527577,767.050640179407,106.424565547509));
#82950=CARTESIAN_POINT('Ctrl Pts',(48.9632488386254,778.228521988974,106.668665317918));
#82951=CARTESIAN_POINT('Ctrl Pts',(48.2421630907403,788.768016093984,110.393679147422));
#82952=CARTESIAN_POINT('Ctrl Pts',(48.8307699445029,767.106785567727,106.407600455105));
#82953=CARTESIAN_POINT('Ctrl Pts',(47.9941274109117,778.216541598047,106.664431042419));
#82954=CARTESIAN_POINT('Ctrl Pts',(47.113525345716,788.690986627767,110.366454327704));
#82955=CARTESIAN_POINT('Ctrl Pts',(47.099562606948,767.269023789712,106.3630646157));
#82956=CARTESIAN_POINT('Ctrl Pts',(46.0065892381932,778.19512484894,106.656861638777));
#82957=CARTESIAN_POINT('Ctrl Pts',(44.8579854286538,788.495169122572,110.297245795717));
#82958=CARTESIAN_POINT('Ctrl Pts',(46.1884599507835,767.374227192424,106.33538318268));
#82959=CARTESIAN_POINT('Ctrl Pts',(44.9898074938279,778.185072718314,106.65330887556));
#82960=CARTESIAN_POINT('Ctrl Pts',(43.7310987807227,788.376007567032,110.255130070057));
#82961=CARTESIAN_POINT('Ctrl Pts',(44.6599688000924,767.595039520773,106.287523900011));
#82962=CARTESIAN_POINT('Ctrl Pts',(43.3812833108911,778.190851690929,106.655351360106));
#82963=CARTESIAN_POINT('Ctrl Pts',(42.0414880433933,788.179960166242,110.185840285188));
#82964=CARTESIAN_POINT('Ctrl Pts',(44.1229651056719,767.679321827364,106.270522681015));
#82965=CARTESIAN_POINT('Ctrl Pts',(42.8311204157762,778.196385262059,106.65730711133));
#82966=CARTESIAN_POINT('Ctrl Pts',(41.478400047932,788.111830043881,110.161760794705));
#82967=CARTESIAN_POINT('Ctrl Pts',(42.9585131381123,767.880518992648,106.235593765515));
#82968=CARTESIAN_POINT('Ctrl Pts',(41.684402157246,778.222618365023,106.666578777572));
#82969=CARTESIAN_POINT('Ctrl Pts',(40.3522402774629,787.97517952959,110.113463879269));
#82970=CARTESIAN_POINT('Ctrl Pts',(42.3324438370369,767.996929545801,106.21756013989));
#82971=CARTESIAN_POINT('Ctrl Pts',(41.0886358099137,778.243004169485,106.673783810619));
#82972=CARTESIAN_POINT('Ctrl Pts',(39.7892076533655,787.906542750337,110.089205319098));
#82973=CARTESIAN_POINT('Ctrl Pts',(41.2706386875018,768.214470254944,106.192394945541));
#82974=CARTESIAN_POINT('Ctrl Pts',(40.1319615807423,778.29735667139,106.69299382386));
#82975=CARTESIAN_POINT('Ctrl Pts',(38.9442264979715,787.810332049824,110.055201202166));
#82976=CARTESIAN_POINT('Ctrl Pts',(40.8958775623199,768.294267732256,106.18434076263));
#82977=CARTESIAN_POINT('Ctrl Pts',(39.8024487847689,778.319513361772,106.700824747908));
#82978=CARTESIAN_POINT('Ctrl Pts',(38.662488217245,787.779426833836,110.044278253132));
#82979=CARTESIAN_POINT('Ctrl Pts',(40.0857541413549,768.475159029144,106.170123670993));
#82980=CARTESIAN_POINT('Ctrl Pts',(39.1123933899711,778.376231169052,106.720870740139));
#82981=CARTESIAN_POINT('Ctrl Pts',(38.0987161989031,787.722035297116,110.023994142163));
#82982=CARTESIAN_POINT('Ctrl Pts',(39.6507046877265,768.576114921759,106.163914476279));
#82983=CARTESIAN_POINT('Ctrl Pts',(38.7520321209999,778.410706406896,106.733055455671));
#82984=CARTESIAN_POINT('Ctrl Pts',(37.8166840316626,787.695525489556,110.01462467919));
#82985=CARTESIAN_POINT('Ctrl Pts',(38.6875932077418,768.811386493074,106.156016095358));
#82986=CARTESIAN_POINT('Ctrl Pts',(37.9837524896163,778.499588578614,106.764469422558));
#82987=CARTESIAN_POINT('Ctrl Pts',(37.2521088113107,787.650146756091,109.998586299356));
#82988=CARTESIAN_POINT('Ctrl Pts',(38.16001983477,768.945417238923,106.154189393271));
#82989=CARTESIAN_POINT('Ctrl Pts',(37.5761167951056,778.553814431039,106.7836346736));
#82990=CARTESIAN_POINT('Ctrl Pts',(36.9695690548407,787.631228525103,109.99189995641));
#82991=CARTESIAN_POINT('Ctrl Pts',(36.9532834034759,769.270474682901,106.161569740109));
#82992=CARTESIAN_POINT('Ctrl Pts',(36.6834835598239,778.696633881445,106.834111899758));
#82993=CARTESIAN_POINT('Ctrl Pts',(36.4036171345023,787.606439911982,109.983138821789));
#82994=CARTESIAN_POINT('Ctrl Pts',(36.2725027848239,769.461655907321,106.170500609688));
#82995=CARTESIAN_POINT('Ctrl Pts',(36.1977184022626,778.785219903999,106.865421197509));
#82996=CARTESIAN_POINT('Ctrl Pts',(36.1202098960075,787.600495865408,109.981037994608));
#82997=CARTESIAN_POINT('Ctrl Pts',(35.0747520244915,769.822544499692,106.204756011053));
#82998=CARTESIAN_POINT('Ctrl Pts',(35.3790433873196,778.963412841933,106.928400611112));
#82999=CARTESIAN_POINT('Ctrl Pts',(35.6939666874706,787.608515394358,109.983872367487));
#83000=CARTESIAN_POINT('Ctrl Pts',(34.6457340436867,769.955453947562,106.219805597645));
#83001=CARTESIAN_POINT('Ctrl Pts',(35.0910332971829,779.030509162521,106.95211472106));
#83002=CARTESIAN_POINT('Ctrl Pts',(35.5516937213439,787.614058603793,109.98583152526));
#83003=CARTESIAN_POINT('Ctrl Pts',(33.7312343792939,770.249022021035,106.260244813743));
#83004=CARTESIAN_POINT('Ctrl Pts',(34.4862671715431,779.18240510027,107.005799884985));
#83005=CARTESIAN_POINT('Ctrl Pts',(35.2666546143195,787.632521014431,109.992356765871));
#83006=CARTESIAN_POINT('Ctrl Pts',(33.2440379163932,770.410411212385,106.285871093897));
#83007=CARTESIAN_POINT('Ctrl Pts',(34.1684624290794,779.267617800876,107.03591693661));
#83008=CARTESIAN_POINT('Ctrl Pts',(35.1235149780168,787.645538139296,109.996957458244));
#83009=CARTESIAN_POINT('Ctrl Pts',(32.259690132129,770.748325877485,106.347650981772));
#83010=CARTESIAN_POINT('Ctrl Pts',(33.5298937723489,779.450220385751,107.100454868647));
#83011=CARTESIAN_POINT('Ctrl Pts',(34.8411271130687,787.679795133055,110.009065038953));
#83012=CARTESIAN_POINT('Ctrl Pts',(31.762501164651,770.924854912313,106.383805863243));
#83013=CARTESIAN_POINT('Ctrl Pts',(33.2088787785457,779.547622607324,107.134880109408));
#83014=CARTESIAN_POINT('Ctrl Pts',(34.7014294761367,787.70105383366,110.016578583053));
#83015=CARTESIAN_POINT('Ctrl Pts',(30.8016313863479,771.277106071563,106.463016442903));
#83016=CARTESIAN_POINT('Ctrl Pts',(32.5854182318755,779.746708986598,107.20524397213));
#83017=CARTESIAN_POINT('Ctrl Pts',(34.4249901431715,787.751730477205,110.034489423568));
#83018=CARTESIAN_POINT('Ctrl Pts',(30.338486235497,771.452534880892,106.505935931361));
#83019=CARTESIAN_POINT('Ctrl Pts',(32.2832227399766,779.848236956052,107.241127391809));
#83020=CARTESIAN_POINT('Ctrl Pts',(34.2882421003274,787.781130901128,110.044880528171));
#83021=CARTESIAN_POINT('Ctrl Pts',(29.030519462635,771.961590961752,106.638170728346));
#83022=CARTESIAN_POINT('Ctrl Pts',(31.4200055420069,780.150349731569,107.347904268904));
#83023=CARTESIAN_POINT('Ctrl Pts',(33.8819357641858,787.880201606199,110.079895467484));
#83024=CARTESIAN_POINT('Ctrl Pts',(28.2689843845276,772.276572686069,106.730103740878));
#83025=CARTESIAN_POINT('Ctrl Pts',(30.9030724009608,780.347718738259,107.417661154068));
#83026=CARTESIAN_POINT('Ctrl Pts',(33.6162769933636,787.960635684765,110.108323592405));
#83027=CARTESIAN_POINT('Ctrl Pts',(26.9222137772097,772.854600754735,106.907363636004));
#83028=CARTESIAN_POINT('Ctrl Pts',(29.9621884190293,780.727290843087,107.551814778971));
#83029=CARTESIAN_POINT('Ctrl Pts',(33.092297454712,788.141758829008,110.172338640035));
#83030=CARTESIAN_POINT('Ctrl Pts',(26.3325994493358,773.11952290612,106.993320051036));
#83031=CARTESIAN_POINT('Ctrl Pts',(29.5359678693991,780.910440753884,107.616546154532));
#83032=CARTESIAN_POINT('Ctrl Pts',(32.8339653751143,788.242416670986,110.207914527233));
#83033=CARTESIAN_POINT('Ctrl Pts',(25.2579283778626,773.617013896509,107.158722030965));
#83034=CARTESIAN_POINT('Ctrl Pts',(28.7390226055063,781.26782836661,107.742859029362));
#83035=CARTESIAN_POINT('Ctrl Pts',(32.3224322386645,788.457895445242,110.284072016962));
#83036=CARTESIAN_POINT('Ctrl Pts',(24.7730747796453,773.849677797855,107.238310108299));
#83037=CARTESIAN_POINT('Ctrl Pts',(28.3683890273826,781.442147786514,107.804469410656));
#83038=CARTESIAN_POINT('Ctrl Pts',(32.069242790029,788.572748419678,110.324664944275));
#83039=CARTESIAN_POINT('Ctrl Pts',(23.8701844394258,774.294398766932,107.392397926644));
#83040=CARTESIAN_POINT('Ctrl Pts',(27.6628084392416,781.785649366179,107.925874491486));
#83041=CARTESIAN_POINT('Ctrl Pts',(31.5665966864075,788.81275794636,110.40949243193));
#83042=CARTESIAN_POINT('Ctrl Pts',(23.4527729129437,774.506259872119,107.466876025996));
#83043=CARTESIAN_POINT('Ctrl Pts',(27.3282358841123,781.95473047245,107.985633475494));
#83044=CARTESIAN_POINT('Ctrl Pts',(31.3172707008355,788.937895174379,110.453720162436));
#83045=CARTESIAN_POINT('Ctrl Pts',(22.2749915223958,775.118189983364,107.68330074963));
#83046=CARTESIAN_POINT('Ctrl Pts',(26.3668555933542,782.454445946986,108.162249832477));
#83047=CARTESIAN_POINT('Ctrl Pts',(30.5786420327287,789.322073679573,110.589501845176));
#83048=CARTESIAN_POINT('Ctrl Pts',(21.5833243793265,775.497036466794,107.818980673689));
#83049=CARTESIAN_POINT('Ctrl Pts',(25.778292337407,782.77915976542,108.277014682795));
#83050=CARTESIAN_POINT('Ctrl Pts',(30.0963148301091,789.590657952587,110.684428615035));
#83051=CARTESIAN_POINT('Ctrl Pts',(20.2781860531485,776.23958244733,108.084377327684));
#83052=CARTESIAN_POINT('Ctrl Pts',(24.646734284643,783.428111818108,108.506376296241));
#83053=CARTESIAN_POINT('Ctrl Pts',(29.1436129446067,790.142589946348,110.879500056716));
#83054=CARTESIAN_POINT('Ctrl Pts',(19.6668691668151,776.602439087497,108.213913923102));
#83055=CARTESIAN_POINT('Ctrl Pts',(24.104872557406,783.75198935753,108.620845577318));
#83056=CARTESIAN_POINT('Ctrl Pts',(28.6733263532804,790.426046475611,110.979683185149));
#83057=CARTESIAN_POINT('Ctrl Pts',(18.4402065432691,777.358402958426,108.482528589129));
#83058=CARTESIAN_POINT('Ctrl Pts',(23.01638179156,784.425478984283,108.858879599368));
#83059=CARTESIAN_POINT('Ctrl Pts',(27.7271624247458,791.014305376711,111.187593785036));
#83060=CARTESIAN_POINT('Ctrl Pts',(17.8263068741335,777.751461542779,108.621536767266));
#83061=CARTESIAN_POINT('Ctrl Pts',(22.4706348085142,784.775231435535,108.982493950034));
#83062=CARTESIAN_POINT('Ctrl Pts',(27.2515765493364,791.319458697228,111.295445293627));
#83063=CARTESIAN_POINT('Ctrl Pts',(17.1827964457161,778.180936484659,108.773321213211));
#83064=CARTESIAN_POINT('Ctrl Pts',(21.9130382745855,785.147368653583,109.1140198343));
#83065=CARTESIAN_POINT('Ctrl Pts',(26.7824206252748,791.632573132854,111.406110529669));
#83066=CARTESIAN_POINT('Ctrl Pts',(55.7276456603534,788.847878152655,110.421905101156));
#83067=CARTESIAN_POINT('Ctrl Pts',(55.8725641695401,788.842398318866,110.41996834248));
#83068=CARTESIAN_POINT('Ctrl Pts',(56.0174997454617,788.836507669495,110.417886387678));
#83069=CARTESIAN_POINT('Ctrl Pts',(56.1624523198427,788.830207971405,110.415659861218));
#83070=CARTESIAN_POINT('Ctrl Pts',(57.296339635109,788.780928765541,110.398242922464));
#83071=CARTESIAN_POINT('Ctrl Pts',(58.4317006497298,788.706476146093,110.371928847582));
#83072=CARTESIAN_POINT('Ctrl Pts',(59.567047823892,788.610423506175,110.337980594612));
#83073=CARTESIAN_POINT('Ctrl Pts',(60.0784213303319,788.567160285554,110.322689908596));
#83074=CARTESIAN_POINT('Ctrl Pts',(60.5893354360563,788.519489778419,110.305841538403));
#83075=CARTESIAN_POINT('Ctrl Pts',(61.0998792915351,788.46826787082,110.287737983121));
#83076=CARTESIAN_POINT('Ctrl Pts',(61.7228414790833,788.405767242783,110.265648146411));
#83077=CARTESIAN_POINT('Ctrl Pts',(62.345254962281,788.337983235991,110.241690984881));
#83078=CARTESIAN_POINT('Ctrl Pts',(62.9672801200892,788.266475473581,110.21641772212));
#83079=CARTESIAN_POINT('Ctrl Pts',(63.2383859190671,788.235309259774,110.205402527625));
#83080=CARTESIAN_POINT('Ctrl Pts',(63.5094202672636,788.203457902004,110.194145180072));
#83081=CARTESIAN_POINT('Ctrl Pts',(63.7804110897448,788.171191083345,110.182740994583));
#83082=CARTESIAN_POINT('Ctrl Pts',(64.0750803558359,788.136104877523,110.170340342274));
#83083=CARTESIAN_POINT('Ctrl Pts',(64.3696983593313,788.100525711438,110.157765461128));
#83084=CARTESIAN_POINT('Ctrl Pts',(64.6643013465014,788.064801985003,110.145139487464));
#83085=CARTESIAN_POINT('Ctrl Pts',(65.2298341777321,787.996225150983,110.120902113966));
#83086=CARTESIAN_POINT('Ctrl Pts',(65.7953001791059,787.927004653761,110.096437248114));
#83087=CARTESIAN_POINT('Ctrl Pts',(66.3611718962303,787.86168084646,110.073349604327));
#83088=CARTESIAN_POINT('Ctrl Pts',(66.3936068769028,787.857936576578,110.07202625266));
#83089=CARTESIAN_POINT('Ctrl Pts',(66.4260432428301,787.854205614206,110.070707604317));
#83090=CARTESIAN_POINT('Ctrl Pts',(66.4584811470731,787.850489430807,110.069394179364));
#83091=CARTESIAN_POINT('Ctrl Pts',(42.7661933181638,788.263968022319,110.215531504003));
#83092=CARTESIAN_POINT('Ctrl Pts',(43.8388165649104,788.387349366501,110.259138645749));
#83093=CARTESIAN_POINT('Ctrl Pts',(44.9118861838019,788.499848583716,110.298899675619));
#83094=CARTESIAN_POINT('Ctrl Pts',(45.9857553871849,788.593077875169,110.33185006171));
#83095=CARTESIAN_POINT('Ctrl Pts',(46.6204803621889,788.648182313867,110.351325834851));
#83096=CARTESIAN_POINT('Ctrl Pts',(47.2554797595624,788.69667299997,110.368464084043));
#83097=CARTESIAN_POINT('Ctrl Pts',(47.8907831607379,788.737861036833,110.383021329903));
#83098=CARTESIAN_POINT('Ctrl Pts',(48.3842772970703,788.769855285001,110.394329179758));
#83099=CARTESIAN_POINT('Ctrl Pts',(48.8779550586805,788.797440912187,110.404078873788));
#83100=CARTESIAN_POINT('Ctrl Pts',(49.3718294922987,788.820296888119,110.412156949034));
#83101=CARTESIAN_POINT('Ctrl Pts',(50.5014957115572,788.872576621917,110.430634375888));
#83102=CARTESIAN_POINT('Ctrl Pts',(51.6321862379869,788.900215353204,110.440402838705));
#83103=CARTESIAN_POINT('Ctrl Pts',(52.7639531549206,788.901955122284,110.441017731963));
#83104=CARTESIAN_POINT('Ctrl Pts',(52.8520451148785,788.902090538566,110.441065592659));
#83105=CARTESIAN_POINT('Ctrl Pts',(52.9401436011452,788.902068984546,110.441057974739));
#83106=CARTESIAN_POINT('Ctrl Pts',(53.0282485972464,788.901890883653,110.440995027858));
#83107=CARTESIAN_POINT('Ctrl Pts',(28.4218514088844,790.583031932319,111.035167157285));
#83108=CARTESIAN_POINT('Ctrl Pts',(28.8178561793361,790.339188506334,110.948984639894));
#83109=CARTESIAN_POINT('Ctrl Pts',(29.2170541634323,790.100042996678,110.864462525091));
#83110=CARTESIAN_POINT('Ctrl Pts',(29.6199625150174,789.866621843685,110.781963591621));
#83111=CARTESIAN_POINT('Ctrl Pts',(29.9403508812464,789.681007865825,110.716361331439));
#83112=CARTESIAN_POINT('Ctrl Pts',(30.2630464352065,789.498965415945,110.652021370092));
#83113=CARTESIAN_POINT('Ctrl Pts',(30.5891590962137,789.32205998929,110.589497006568));
#83114=CARTESIAN_POINT('Ctrl Pts',(30.7244461380251,789.248671204633,110.5635589269));
#83115=CARTESIAN_POINT('Ctrl Pts',(30.8603209078513,789.176166054629,110.537933153616));
#83116=CARTESIAN_POINT('Ctrl Pts',(30.9968610193644,789.104654262708,110.512658466691));
#83117=CARTESIAN_POINT('Ctrl Pts',(31.0215692479453,789.091713525503,110.508084772302));
#83118=CARTESIAN_POINT('Ctrl Pts',(31.0462980416312,789.078806144513,110.503522867128));
#83119=CARTESIAN_POINT('Ctrl Pts',(31.0710482020822,789.065932555418,110.498972905153));
#83120=CARTESIAN_POINT('Ctrl Pts',(31.317568884694,788.937706882794,110.453653613826));
#83121=CARTESIAN_POINT('Ctrl Pts',(31.5668006079514,788.812638621386,110.409450258449));
#83122=CARTESIAN_POINT('Ctrl Pts',(31.8179138799322,788.692742276541,110.367074833385));
#83123=CARTESIAN_POINT('Ctrl Pts',(31.990334141305,788.610418634494,110.337978872795));
#83124=CARTESIAN_POINT('Ctrl Pts',(32.1635810675995,788.530542075654,110.30974779421));
#83125=CARTESIAN_POINT('Ctrl Pts',(32.3379854760787,788.453693822171,110.282587021203));
#83126=CARTESIAN_POINT('Ctrl Pts',(32.4178161094536,788.418517849253,110.270154642165));
#83127=CARTESIAN_POINT('Ctrl Pts',(32.4978789650267,788.383983087561,110.257948888871));
#83128=CARTESIAN_POINT('Ctrl Pts',(32.5781960071056,788.35015014966,110.24599118385));
#83129=CARTESIAN_POINT('Ctrl Pts',(32.8339631335456,788.242410209518,110.207912243532));
#83130=CARTESIAN_POINT('Ctrl Pts',(33.0922962422252,788.141755327546,110.1723374025));
#83131=CARTESIAN_POINT('Ctrl Pts',(33.354286616325,788.051195694031,110.140330563854));
#83132=CARTESIAN_POINT('Ctrl Pts',(33.4778110484393,788.008498219588,110.12523983168));
#83133=CARTESIAN_POINT('Ctrl Pts',(33.6021510102252,787.968051834242,110.110944710562));
#83134=CARTESIAN_POINT('Ctrl Pts',(33.7274682578125,787.930302473205,110.097602809089));
#83135=CARTESIAN_POINT('Ctrl Pts',(33.8679812561842,787.887975690515,110.082643091924));
#83136=CARTESIAN_POINT('Ctrl Pts',(34.0096692762972,787.849054278572,110.068886948005));
#83137=CARTESIAN_POINT('Ctrl Pts',(34.1528056083597,787.814150653876,110.056550826044));
#83138=CARTESIAN_POINT('Ctrl Pts',(34.2882334261246,787.781126741243,110.044879057927));
#83139=CARTESIAN_POINT('Ctrl Pts',(34.424967282988,787.751725783049,110.034487764496));
#83140=CARTESIAN_POINT('Ctrl Pts',(34.563207601984,787.726381449949,110.025530219632));
#83141=CARTESIAN_POINT('Ctrl Pts',(34.7013791320057,787.701049728298,110.01657713208));
#83142=CARTESIAN_POINT('Ctrl Pts',(34.8410619689514,787.679788099456,110.009062553043));
#83143=CARTESIAN_POINT('Ctrl Pts',(34.9823190110975,787.662651728054,110.003005979566));
#83144=CARTESIAN_POINT('Ctrl Pts',(35.054858148777,787.653851758966,109.999895772735));
#83145=CARTESIAN_POINT('Ctrl Pts',(35.1279311989363,787.646134864626,109.997168361168));
#83146=CARTESIAN_POINT('Ctrl Pts',(35.201196182069,787.639458454135,109.994808691798));
#83147=CARTESIAN_POINT('Ctrl Pts',(35.2704926162082,787.633143685196,109.99257683879));
#83148=CARTESIAN_POINT('Ctrl Pts',(35.3399150435733,787.627763108406,109.990675160896));
#83149=CARTESIAN_POINT('Ctrl Pts',(35.40917327038,787.623277492044,109.989089792298));
#83150=CARTESIAN_POINT('Ctrl Pts',(35.5517549337684,787.61404296971,109.985825999648));
#83151=CARTESIAN_POINT('Ctrl Pts',(35.6940149178129,787.608502739353,109.983867894781));
#83152=CARTESIAN_POINT('Ctrl Pts',(35.8360475033717,787.605830235265,109.98292334141));
#83153=CARTESIAN_POINT('Ctrl Pts',(36.0908674215757,787.601035509672,109.981228723152));
#83154=CARTESIAN_POINT('Ctrl Pts',(36.3449657656687,787.605316731778,109.982741851903));
#83155=CARTESIAN_POINT('Ctrl Pts',(36.5987997780528,787.6151913345,109.98623187062));
#83156=CARTESIAN_POINT('Ctrl Pts',(36.6280676541629,787.616329907879,109.986634280977));
#83157=CARTESIAN_POINT('Ctrl Pts',(36.6573320118389,787.617542895409,109.987062991812));
#83158=CARTESIAN_POINT('Ctrl Pts',(36.686593549319,787.618824991082,109.987516127804));
#83159=CARTESIAN_POINT('Ctrl Pts',(36.6986198925109,787.619351925889,109.987702364394));
#83160=CARTESIAN_POINT('Ctrl Pts',(36.7106457504267,787.61989066731,109.987892773841));
#83161=CARTESIAN_POINT('Ctrl Pts',(36.7226711608112,787.620441007396,109.988087282649));
#83162=CARTESIAN_POINT('Ctrl Pts',(36.9935849295287,787.632839312507,109.992469263181));
#83163=CARTESIAN_POINT('Ctrl Pts',(37.2641062977475,787.651109175024,109.998926450771));
#83164=CARTESIAN_POINT('Ctrl Pts',(37.5343966207417,787.67283391909,110.006604710399));
#83165=CARTESIAN_POINT('Ctrl Pts',(37.7681335687267,787.691620664088,110.013244581747));
#83166=CARTESIAN_POINT('Ctrl Pts',(38.0016954672153,787.713024821358,110.020809535154));
#83167=CARTESIAN_POINT('Ctrl Pts',(38.2351440760971,787.736118419525,110.028971594138));
#83168=CARTESIAN_POINT('Ctrl Pts',(38.2836351952192,787.740915340034,110.030666988154));
#83169=CARTESIAN_POINT('Ctrl Pts',(38.3321214618988,787.745785478162,110.032388259753));
#83170=CARTESIAN_POINT('Ctrl Pts',(38.3806034200487,787.750720481976,110.034132457081));
#83171=CARTESIAN_POINT('Ctrl Pts',(38.6624894118298,787.779413804146,110.044273647999));
#83172=CARTESIAN_POINT('Ctrl Pts',(38.9442281267435,787.810323481981,110.055198174001));
#83173=CARTESIAN_POINT('Ctrl Pts',(39.2258874928907,787.842397522499,110.066534225172));
#83174=CARTESIAN_POINT('Ctrl Pts',(39.3986909004619,787.86207555974,110.073489109356));
#83175=CARTESIAN_POINT('Ctrl Pts',(39.5714666607601,787.882176445889,110.080593442651));
#83176=CARTESIAN_POINT('Ctrl Pts',(39.7442240872993,787.902559549599,110.087797521182));
#83177=CARTESIAN_POINT('Ctrl Pts',(17.244803233355,778.140660313945,108.758852681557));
#83178=CARTESIAN_POINT('Ctrl Pts',(17.4302427942975,778.017216179823,108.715223348388));
#83179=CARTESIAN_POINT('Ctrl Pts',(17.6161195650913,777.895023168326,108.672035343682));
#83180=CARTESIAN_POINT('Ctrl Pts',(17.8025176283173,777.773958439212,108.629218349539));
#83181=CARTESIAN_POINT('Ctrl Pts',(17.9870250009404,777.654121705398,108.586835660812));
#83182=CARTESIAN_POINT('Ctrl Pts',(18.1720429482635,777.535390196698,108.544816419935));
#83183=CARTESIAN_POINT('Ctrl Pts',(18.3576213362097,777.417677845536,108.503114059011));
#83184=CARTESIAN_POINT('Ctrl Pts',(18.5421857868206,777.300608634714,108.461639545635));
#83185=CARTESIAN_POINT('Ctrl Pts',(18.7273043691045,777.184547269975,108.420478415007));
#83186=CARTESIAN_POINT('Ctrl Pts',(18.912997562236,777.069445629894,108.379607264944));
#83187=CARTESIAN_POINT('Ctrl Pts',(19.1038171142841,776.951166424126,108.337607801123));
#83188=CARTESIAN_POINT('Ctrl Pts',(19.2952433373739,776.833900304558,108.295914413569));
#83189=CARTESIAN_POINT('Ctrl Pts',(19.4872703008399,776.717638363243,108.254526995366));
#83190=CARTESIAN_POINT('Ctrl Pts',(19.6751476855667,776.603888767441,108.214033932558));
#83191=CARTESIAN_POINT('Ctrl Pts',(19.8635997887069,776.491100501578,108.173833868963));
#83192=CARTESIAN_POINT('Ctrl Pts',(20.052598145976,776.379307612994,108.133950440718));
#83193=CARTESIAN_POINT('Ctrl Pts',(20.2478580091165,776.263811031752,108.092745676544));
#83194=CARTESIAN_POINT('Ctrl Pts',(20.4437007248949,776.149376625192,108.051878811667));
#83195=CARTESIAN_POINT('Ctrl Pts',(20.6400739635806,776.036089498082,108.01140147736));
#83196=CARTESIAN_POINT('Ctrl Pts',(20.8364472022663,775.922802370972,107.970924143053));
#83197=CARTESIAN_POINT('Ctrl Pts',(21.0333506142589,775.810662609105,107.93083646242));
#83198=CARTESIAN_POINT('Ctrl Pts',(21.230715589858,775.69980296013,107.891214563218));
#83199=CARTESIAN_POINT('Ctrl Pts',(21.4510621334662,775.576034594425,107.846979011728));
#83200=CARTESIAN_POINT('Ctrl Pts',(21.6721167421861,775.453725728634,107.803275358442));
#83201=CARTESIAN_POINT('Ctrl Pts',(21.8938661721106,775.332765884813,107.760111498484));
#83202=CARTESIAN_POINT('Ctrl Pts',(22.1268288785303,775.205689424709,107.714764957397));
#83203=CARTESIAN_POINT('Ctrl Pts',(22.3605582172284,775.080102215295,107.670014400197));
#83204=CARTESIAN_POINT('Ctrl Pts',(22.5950407446481,774.955928755215,107.625894992143));
#83205=CARTESIAN_POINT('Ctrl Pts',(22.8503193797093,774.820742429185,107.577862661582));
#83206=CARTESIAN_POINT('Ctrl Pts',(23.1064903655798,774.687231914115,107.53057856877));
#83207=CARTESIAN_POINT('Ctrl Pts',(23.3635434284907,774.555356825587,107.48411523043));
#83208=CARTESIAN_POINT('Ctrl Pts',(23.6348421915746,774.416173312291,107.435076926519));
#83209=CARTESIAN_POINT('Ctrl Pts',(23.9071230928796,774.278812126388,107.386953297135));
#83210=CARTESIAN_POINT('Ctrl Pts',(24.1803878516845,774.143279983621,107.339853560423));
#83211=CARTESIAN_POINT('Ctrl Pts',(24.476664170325,773.9963347116,107.288787566174));
#83212=CARTESIAN_POINT('Ctrl Pts',(24.7740963725344,773.851540100502,107.238925693366));
#83213=CARTESIAN_POINT('Ctrl Pts',(25.0727111866745,773.708957217398,107.190427006648));
#83214=CARTESIAN_POINT('Ctrl Pts',(25.1730175253031,773.661062852222,107.174136034257));
#83215=CARTESIAN_POINT('Ctrl Pts',(25.2734575369564,773.613418408341,107.157998991203));
#83216=CARTESIAN_POINT('Ctrl Pts',(25.3740329818863,773.566027188085,107.142022184744));
#83217=CARTESIAN_POINT('Ctrl Pts',(25.6843444268857,773.419808217358,107.092727986718));
#83218=CARTESIAN_POINT('Ctrl Pts',(25.9959755695988,773.2758580971,107.04490895962));
#83219=CARTESIAN_POINT('Ctrl Pts',(26.3088451966942,773.134131453208,106.998692394593));
#83220=CARTESIAN_POINT('Ctrl Pts',(26.6298522170826,772.988718655909,106.951273787776));
#83221=CARTESIAN_POINT('Ctrl Pts',(26.9521628990224,772.8456475125,106.905542763938));
#83222=CARTESIAN_POINT('Ctrl Pts',(27.2757410475479,772.704884152336,106.861629835336));
#83223=CARTESIAN_POINT('Ctrl Pts',(27.5998714259456,772.563880560462,106.817641963384));
#83224=CARTESIAN_POINT('Ctrl Pts',(27.9252738053818,772.425193467478,106.775478905283));
#83225=CARTESIAN_POINT('Ctrl Pts',(28.2519616068956,772.288789746552,106.735255966003));
#83226=CARTESIAN_POINT('Ctrl Pts',(28.5781188910106,772.152607535418,106.695098345872));
#83227=CARTESIAN_POINT('Ctrl Pts',(28.9055577145741,772.018701882974,106.656874901712));
#83228=CARTESIAN_POINT('Ctrl Pts',(29.2343372719155,771.887030087691,106.620678159765));
#83229=CARTESIAN_POINT('Ctrl Pts',(29.3798300670145,771.828762178073,106.604660238207));
#83230=CARTESIAN_POINT('Ctrl Pts',(29.5255859903457,771.770931537783,106.589038877081));
#83231=CARTESIAN_POINT('Ctrl Pts',(29.6716128056531,771.71353344704,106.573820461869));
#83232=CARTESIAN_POINT('Ctrl Pts',(29.98499083181,771.590355383173,106.54116127588));
#83233=CARTESIAN_POINT('Ctrl Pts',(30.2996186961208,771.469154223282,106.510354321007));
#83234=CARTESIAN_POINT('Ctrl Pts',(30.6154250134758,771.349953382847,106.48146631183));
#83235=CARTESIAN_POINT('Ctrl Pts',(30.9329624820416,771.230099120781,106.452419947644));
#83236=CARTESIAN_POINT('Ctrl Pts',(31.2516915141686,771.112267420327,106.425313820703));
#83237=CARTESIAN_POINT('Ctrl Pts',(31.5715845956891,770.996474616581,106.400189136909));
#83238=CARTESIAN_POINT('Ctrl Pts',(31.8930543690029,770.88011109226,106.374940618357));
#83239=CARTESIAN_POINT('Ctrl Pts',(32.2156998911378,770.765806805995,106.351693262802));
#83240=CARTESIAN_POINT('Ctrl Pts',(32.5395359463363,770.653567465855,106.330459565991));
#83241=CARTESIAN_POINT('Ctrl Pts',(32.8669620803978,770.540083829177,106.308990470297));
#83242=CARTESIAN_POINT('Ctrl Pts',(33.1956054823697,770.428711338438,106.289580054316));
#83243=CARTESIAN_POINT('Ctrl Pts',(33.5255221042312,770.319442106759,106.272209275265));
#83244=CARTESIAN_POINT('Ctrl Pts',(33.7242078623965,770.253636873856,106.261748067259));
#83245=CARTESIAN_POINT('Ctrl Pts',(33.9233561640316,770.188594174724,106.252025971253));
#83246=CARTESIAN_POINT('Ctrl Pts',(34.1229857448722,770.124309587169,106.243033090213));
#83247=CARTESIAN_POINT('Ctrl Pts',(34.4053309678074,770.03338896244,106.230314048319));
#83248=CARTESIAN_POINT('Ctrl Pts',(34.6888310896164,769.943954899535,106.219056503782));
#83249=CARTESIAN_POINT('Ctrl Pts',(34.9731646028604,769.856111120652,106.209232445828));
#83250=CARTESIAN_POINT('Ctrl Pts',(35.2621382182265,769.766833799519,106.199248066878));
#83251=CARTESIAN_POINT('Ctrl Pts',(35.551972690203,769.679199164546,106.190744375241));
#83252=CARTESIAN_POINT('Ctrl Pts',(35.8423794454014,769.593326894789,106.18367117377));
#83253=CARTESIAN_POINT('Ctrl Pts',(36.0301478417598,769.53780443157,106.179097851444));
#83254=CARTESIAN_POINT('Ctrl Pts',(36.2181564792175,769.483018947022,106.175122122085));
#83255=CARTESIAN_POINT('Ctrl Pts',(36.4063377647076,769.429004905351,106.171725880262));
#83256=CARTESIAN_POINT('Ctrl Pts',(36.7463662342535,769.331405870062,106.16558914405));
#83257=CARTESIAN_POINT('Ctrl Pts',(37.0867097552781,769.236368553691,106.161342180024));
#83258=CARTESIAN_POINT('Ctrl Pts',(37.4273506666537,769.143933968207,106.158823323891));
#83259=CARTESIAN_POINT('Ctrl Pts',(37.7829651679578,769.047436225504,106.156193746122));
#83260=CARTESIAN_POINT('Ctrl Pts',(38.1389040062214,768.953775170179,106.155447471501));
#83261=CARTESIAN_POINT('Ctrl Pts',(38.4951922026422,768.862988805248,106.156367580926));
#83262=CARTESIAN_POINT('Ctrl Pts',(38.5660483213149,768.844933844371,106.15655056589));
#83263=CARTESIAN_POINT('Ctrl Pts',(38.6369183876645,768.826992549612,106.156799359364));
#83264=CARTESIAN_POINT('Ctrl Pts',(38.7078027855985,768.809165175802,106.157112113951));
#83265=CARTESIAN_POINT('Ctrl Pts',(39.0660941928767,768.71905515108,106.158692959443));
#83266=CARTESIAN_POINT('Ctrl Pts',(39.4247842952702,768.631843714424,106.161909448324));
#83267=CARTESIAN_POINT('Ctrl Pts',(39.7838264747246,768.54761783095,106.166513137719));
#83268=CARTESIAN_POINT('Ctrl Pts',(40.1704981466507,768.456910485,106.171471096358));
#83269=CARTESIAN_POINT('Ctrl Pts',(40.5575782622505,768.36966600186,106.178037739708));
#83270=CARTESIAN_POINT('Ctrl Pts',(40.9450618818424,768.285989009415,106.185873456951));
#83271=CARTESIAN_POINT('Ctrl Pts',(41.3721816802832,768.193752593886,106.194510699404));
#83272=CARTESIAN_POINT('Ctrl Pts',(41.7997918445297,768.105851072209,106.204689398667));
#83273=CARTESIAN_POINT('Ctrl Pts',(42.2279470420453,768.022416903132,106.215926170645));
#83274=CARTESIAN_POINT('Ctrl Pts',(42.5983746669712,767.950232047574,106.225647904212));
#83275=CARTESIAN_POINT('Ctrl Pts',(42.9692116538452,767.881391015369,106.236160711799));
#83276=CARTESIAN_POINT('Ctrl Pts',(43.3405227698438,767.815973740261,106.247143043839));
#83277=CARTESIAN_POINT('Ctrl Pts',(43.7894092447679,767.73688930471,106.260419835465));
#83278=CARTESIAN_POINT('Ctrl Pts',(44.2389602380122,767.662833944119,106.274384781587));
#83279=CARTESIAN_POINT('Ctrl Pts',(44.6891574273935,767.594001659024,106.288473974073));
#83280=CARTESIAN_POINT('Ctrl Pts',(45.1319036972893,767.5263085721,106.302329985541));
#83281=CARTESIAN_POINT('Ctrl Pts',(45.5752759585645,767.463667274342,106.316304786023));
#83282=CARTESIAN_POINT('Ctrl Pts',(46.0192976440156,767.406257685716,106.329888910912));
#83283=CARTESIAN_POINT('Ctrl Pts',(46.4363813545946,767.352331030709,106.342648912056));
#83284=CARTESIAN_POINT('Ctrl Pts',(46.8540388223096,767.303020623235,106.355063538047));
#83285=CARTESIAN_POINT('Ctrl Pts',(47.2723132478599,767.258469809936,106.366748379134));
#83286=CARTESIAN_POINT('Ctrl Pts',(47.5207984325909,767.232003412766,106.37369001773));
#83287=CARTESIAN_POINT('Ctrl Pts',(47.7695017500408,767.207216663347,106.380374877173));
#83288=CARTESIAN_POINT('Ctrl Pts',(48.0184352890197,767.184138393967,106.386730603336));
#83289=CARTESIAN_POINT('Ctrl Pts',(48.4103491489587,767.14780462524,106.396736877234));
#83290=CARTESIAN_POINT('Ctrl Pts',(48.8028254789344,767.115718004464,106.405926142084));
#83291=CARTESIAN_POINT('Ctrl Pts',(49.1958617553921,767.087969142023,106.414049755935));
#83292=CARTESIAN_POINT('Ctrl Pts',(49.5712128370626,767.061468876891,106.421807836878));
#83293=CARTESIAN_POINT('Ctrl Pts',(49.9470747019511,767.038924816821,106.428593946834));
#83294=CARTESIAN_POINT('Ctrl Pts',(50.32345337455,767.020411253827,106.434239309414));
#83295=CARTESIAN_POINT('Ctrl Pts',(50.6934444934781,767.002211886047,106.439788864078));
#83296=CARTESIAN_POINT('Ctrl Pts',(51.0639350090242,766.987907416256,106.444235893158));
#83297=CARTESIAN_POINT('Ctrl Pts',(51.4349383309662,766.97756326832,106.44746932169));
#83298=CARTESIAN_POINT('Ctrl Pts',(51.799639404856,766.967394836832,106.450647823845));
#83299=CARTESIAN_POINT('Ctrl Pts',(52.1648359513474,766.961053359176,106.452653536912));
#83300=CARTESIAN_POINT('Ctrl Pts',(52.5305487998093,766.958595366651,106.453430683641));
#83301=CARTESIAN_POINT('Ctrl Pts',(52.6032085014127,766.95810701355,106.453585086883));
#83302=CARTESIAN_POINT('Ctrl Pts',(52.6758886111045,766.957771936566,106.453691155307));
#83303=CARTESIAN_POINT('Ctrl Pts',(52.7485893348995,766.957590550071,106.453748693095));
#83304=CARTESIAN_POINT('Ctrl Pts',(52.7916024730424,766.957483233362,106.453782735133));
#83305=CARTESIAN_POINT('Ctrl Pts',(52.8346226593573,766.957429629665,106.453799778285));
#83306=CARTESIAN_POINT('Ctrl Pts',(52.8776498831824,766.957429760005,106.453799787005));
#83307=CARTESIAN_POINT('Ctrl Pts',(53.2527766899241,766.957430896356,106.453799863031));
#83308=CARTESIAN_POINT('Ctrl Pts',(53.6284390702103,766.961516813679,106.452500231006));
#83309=CARTESIAN_POINT('Ctrl Pts',(54.0046343511746,766.969707371652,106.4499239518));
#83310=CARTESIAN_POINT('Ctrl Pts',(54.380829632139,766.977897929626,106.447347672594));
#83311=CARTESIAN_POINT('Ctrl Pts',(54.7575577055266,766.990193160191,106.44349480217));
#83312=CARTESIAN_POINT('Ctrl Pts',(55.1348251867634,767.006606943788,106.438447973463));
#83313=CARTESIAN_POINT('Ctrl Pts',(55.4561641097655,767.020587442521,106.434149319108));
#83314=CARTESIAN_POINT('Ctrl Pts',(55.7778622926501,767.037583043997,106.428988897936));
#83315=CARTESIAN_POINT('Ctrl Pts',(56.0993921197504,767.057497379615,106.423055564023));
#83316=CARTESIAN_POINT('Ctrl Pts',(56.4262826167593,767.077743734757,106.417023307267));
#83317=CARTESIAN_POINT('Ctrl Pts',(56.7529993434126,767.101006852348,106.410192320713));
#83318=CARTESIAN_POINT('Ctrl Pts',(57.0789741399141,767.12720391569,106.402704938146));
#83319=CARTESIAN_POINT('Ctrl Pts',(57.228415709256,767.139213832715,106.39927238381));
#83320=CARTESIAN_POINT('Ctrl Pts',(57.3777011350278,767.151840645628,106.395702527817));
#83321=CARTESIAN_POINT('Ctrl Pts',(57.5267745005702,767.16507773094,106.392012248412));
#83322=CARTESIAN_POINT('Ctrl Pts',(57.9483269317961,767.202509806585,106.381576807787));
#83323=CARTESIAN_POINT('Ctrl Pts',(58.3687655186023,767.244817320047,106.370151825623));
#83324=CARTESIAN_POINT('Ctrl Pts',(58.7881688820604,767.291834998808,106.358094002693));
#83325=CARTESIAN_POINT('Ctrl Pts',(59.2221899539139,767.340491411964,106.345615921474));
#83326=CARTESIAN_POINT('Ctrl Pts',(59.6551028890472,767.394191898677,106.332460922299));
#83327=CARTESIAN_POINT('Ctrl Pts',(60.0869645521638,767.452745062953,106.319073080512));
#83328=CARTESIAN_POINT('Ctrl Pts',(60.5251884576043,767.512160840079,106.305488007294));
#83329=CARTESIAN_POINT('Ctrl Pts',(60.9623305926084,767.576573131153,106.29166436926));
#83330=CARTESIAN_POINT('Ctrl Pts',(61.3984106399046,767.645776298645,106.278099940895));
#83331=CARTESIAN_POINT('Ctrl Pts',(61.6818255091146,767.690752460212,106.269284218381));
#83332=CARTESIAN_POINT('Ctrl Pts',(61.9647909508895,767.737752127751,106.26057863376));
#83333=CARTESIAN_POINT('Ctrl Pts',(62.2473011154386,767.786718213586,106.252123551089));
#83334=CARTESIAN_POINT('Ctrl Pts',(62.6665970293828,767.859392695035,106.23957468715));
#83335=CARTESIAN_POINT('Ctrl Pts',(63.0848727254616,767.936378587464,106.227575522707));
#83336=CARTESIAN_POINT('Ctrl Pts',(63.5022363713141,768.017536835016,106.216582523638));
#83337=CARTESIAN_POINT('Ctrl Pts',(63.8968659205552,768.094274334717,106.206188321098));
#83338=CARTESIAN_POINT('Ctrl Pts',(64.2906803943568,768.174741854941,106.1966943297));
#83339=CARTESIAN_POINT('Ctrl Pts',(64.6837303810336,768.258815228337,106.188472833452));
#83340=CARTESIAN_POINT('Ctrl Pts',(65.0524210672923,768.337678148536,106.18076086501));
#83341=CARTESIAN_POINT('Ctrl Pts',(65.4204392441859,768.419713694752,106.174168906627));
#83342=CARTESIAN_POINT('Ctrl Pts',(65.7877865032849,768.504815487676,106.168985000604));
#83343=CARTESIAN_POINT('Ctrl Pts',(66.1551337623839,768.589917280599,106.163801094582));
#83344=CARTESIAN_POINT('Ctrl Pts',(66.5218106947982,768.67808522904,106.160025715033));
#83345=CARTESIAN_POINT('Ctrl Pts',(66.8877713295124,768.769210484844,106.157920728899));
#83346=CARTESIAN_POINT('Ctrl Pts',(67.2493508831965,768.859244838809,106.15584094251));
#83347=CARTESIAN_POINT('Ctrl Pts',(67.6102184648288,768.95214837915,106.155388024597));
#83348=CARTESIAN_POINT('Ctrl Pts',(67.9704601261528,769.047897806214,106.15679353994));
#83349=CARTESIAN_POINT('Ctrl Pts',(68.313064781029,769.138959454368,106.158130242911));
#83350=CARTESIAN_POINT('Ctrl Pts',(68.6551034662053,769.232595028966,106.161147869937));
#83351=CARTESIAN_POINT('Ctrl Pts',(68.9966145154768,769.328774634844,106.166016326262));
#83352=CARTESIAN_POINT('Ctrl Pts',(69.3301256614168,769.422701231482,106.170770738898));
#83353=CARTESIAN_POINT('Ctrl Pts',(69.6631338605876,769.519053985963,106.177290356695));
#83354=CARTESIAN_POINT('Ctrl Pts',(69.995636649277,769.617796797526,106.185704017807));
#83355=CARTESIAN_POINT('Ctrl Pts',(70.3185030507481,769.713677906873,106.193873839471));
#83356=CARTESIAN_POINT('Ctrl Pts',(70.6408930762567,769.811812450673,106.203829498684));
#83357=CARTESIAN_POINT('Ctrl Pts',(70.9627650543597,769.912160796529,106.21566052958));
#83358=CARTESIAN_POINT('Ctrl Pts',(71.1279096933335,769.963647078266,106.221730742145));
#83359=CARTESIAN_POINT('Ctrl Pts',(71.2929172974997,770.01571603625,106.228294174781));
#83360=CARTESIAN_POINT('Ctrl Pts',(71.4577778171004,770.068361747236,106.235359916851));
#83361=CARTESIAN_POINT('Ctrl Pts',(71.7847090879655,770.172762298928,106.249371834562));
#83362=CARTESIAN_POINT('Ctrl Pts',(72.111113040878,770.279454187517,106.26536517023));
#83363=CARTESIAN_POINT('Ctrl Pts',(72.437015064023,770.388454389171,106.283403068439));
#83364=CARTESIAN_POINT('Ctrl Pts',(72.755745340328,770.495055950141,106.301044027599));
#83365=CARTESIAN_POINT('Ctrl Pts',(73.0739957493183,770.603865216048,106.320640490581));
#83366=CARTESIAN_POINT('Ctrl Pts',(73.3917516221727,770.714885580109,106.342222081288));
#83367=CARTESIAN_POINT('Ctrl Pts',(73.5005165936022,770.75288685013,106.349609265278));
#83368=CARTESIAN_POINT('Ctrl Pts',(73.6092232721889,770.791147079065,106.357228779375));
#83369=CARTESIAN_POINT('Ctrl Pts',(73.717869934504,770.829666103205,106.365081018644));
#83370=CARTESIAN_POINT('Ctrl Pts',(73.9939731299839,770.927554298068,106.385035873287));
#83371=CARTESIAN_POINT('Ctrl Pts',(74.2698322480944,771.027190750308,106.406514466711));
#83372=CARTESIAN_POINT('Ctrl Pts',(74.5451525422015,771.128450377454,106.42948314097));
#83373=CARTESIAN_POINT('Ctrl Pts',(74.8190712176449,771.22919450543,106.452334884791));
#83374=CARTESIAN_POINT('Ctrl Pts',(75.0924565785729,771.331545169713,106.476661452536));
#83375=CARTESIAN_POINT('Ctrl Pts',(75.3649710421158,771.435390477115,106.502412606952));
#83376=CARTESIAN_POINT('Ctrl Pts',(75.5631914758016,771.510925043617,106.521143374229));
#83377=CARTESIAN_POINT('Ctrl Pts',(75.7609501554619,771.587250611355,106.540627487359));
#83378=CARTESIAN_POINT('Ctrl Pts',(75.95810121129,771.664328638783,106.560840536383));
#83379=CARTESIAN_POINT('Ctrl Pts',(76.2903210760871,771.79421306544,106.594901608922));
#83380=CARTESIAN_POINT('Ctrl Pts',(76.6210076059917,771.926275982453,106.631041202677));
#83381=CARTESIAN_POINT('Ctrl Pts',(76.9502435149238,772.060562462679,106.66917485183));
#83382=CARTESIAN_POINT('Ctrl Pts',(77.2812602282517,772.195575285166,106.707514762111));
#83383=CARTESIAN_POINT('Ctrl Pts',(77.6108109014645,772.332835291012,106.747870059369));
#83384=CARTESIAN_POINT('Ctrl Pts',(77.938935474115,772.472374376002,106.790129678487));
#83385=CARTESIAN_POINT('Ctrl Pts',(78.266895980731,772.611843689855,106.832368167314));
#83386=CARTESIAN_POINT('Ctrl Pts',(78.5934320342002,772.753589087331,106.87650862444));
#83387=CARTESIAN_POINT('Ctrl Pts',(78.918535562098,772.897637659967,106.922420647974));
#83388=CARTESIAN_POINT('Ctrl Pts',(79.2380344310416,773.03920289098,106.967541165997));
#83389=CARTESIAN_POINT('Ctrl Pts',(79.5561497471268,773.182991674586,107.014372093433));
#83390=CARTESIAN_POINT('Ctrl Pts',(79.872826046708,773.32903705898,107.062778666628));
#83391=CARTESIAN_POINT('Ctrl Pts',(80.0205711758635,773.397174441564,107.085362723023));
#83392=CARTESIAN_POINT('Ctrl Pts',(80.1680023906269,773.465803200904,107.108289644626));
#83393=CARTESIAN_POINT('Ctrl Pts',(80.3151104245496,773.53492818077,107.131545519252));
#83394=CARTESIAN_POINT('Ctrl Pts',(80.6192289859328,773.677831249161,107.179622724464));
#83395=CARTESIAN_POINT('Ctrl Pts',(80.9220023028729,773.822986743339,107.229153229747));
#83396=CARTESIAN_POINT('Ctrl Pts',(81.2234700330845,773.970314254708,107.27996471884));
#83397=CARTESIAN_POINT('Ctrl Pts',(81.5008857271214,774.10588751752,107.326722308788));
#83398=CARTESIAN_POINT('Ctrl Pts',(81.7771952718529,774.243299530907,107.374564166958));
#83399=CARTESIAN_POINT('Ctrl Pts',(82.052408977665,774.382524341856,107.423368824163));
#83400=CARTESIAN_POINT('Ctrl Pts',(82.306318838869,774.510971987005,107.468395592364));
#83401=CARTESIAN_POINT('Ctrl Pts',(82.5592955474459,774.640962327582,107.514241591404));
#83402=CARTESIAN_POINT('Ctrl Pts',(82.8113354824272,774.772513053793,107.560827758554));
#83403=CARTESIAN_POINT('Ctrl Pts',(83.0511584124714,774.897687187852,107.605155777866));
#83404=CARTESIAN_POINT('Ctrl Pts',(83.2901329115115,775.02427369952,107.65015367622));
#83405=CARTESIAN_POINT('Ctrl Pts',(83.528249378592,775.152328972771,107.695772667662));
#83406=CARTESIAN_POINT('Ctrl Pts',(83.7512300445672,775.272244451365,107.73849190173));
#83407=CARTESIAN_POINT('Ctrl Pts',(83.9734580736361,775.393447712216,107.781755638271));
#83408=CARTESIAN_POINT('Ctrl Pts',(84.1949231770313,775.516025956021,107.825543948619));
#83409=CARTESIAN_POINT('Ctrl Pts',(84.2966126723844,775.572309856115,107.845650101297));
#83410=CARTESIAN_POINT('Ctrl Pts',(84.3981413012444,775.628884255573,107.865867154406));
#83411=CARTESIAN_POINT('Ctrl Pts',(84.4995080719372,775.685760960997,107.886194872769));
#83412=CARTESIAN_POINT('Ctrl Pts',(84.6944224660258,775.795127062923,107.925282286531));
#83413=CARTESIAN_POINT('Ctrl Pts',(84.8888430390403,775.905714468591,107.964815559485));
#83414=CARTESIAN_POINT('Ctrl Pts',(85.0827036691784,776.017394830005,108.004720940244));
#83415=CARTESIAN_POINT('Ctrl Pts',(85.2743324103567,776.127789431823,108.044166896215));
#83416=CARTESIAN_POINT('Ctrl Pts',(85.4654137438478,776.239251980637,108.083976376863));
#83417=CARTESIAN_POINT('Ctrl Pts',(85.6558986329479,776.351701355677,108.124100247506));
#83418=CARTESIAN_POINT('Ctrl Pts',(85.8449854023638,776.463325375565,108.163929617237));
#83419=CARTESIAN_POINT('Ctrl Pts',(86.0334841976882,776.575921840707,108.204068743911));
#83420=CARTESIAN_POINT('Ctrl Pts',(86.2213657472959,776.689453432604,108.244492225632));
#83421=CARTESIAN_POINT('Ctrl Pts',(86.4146817443415,776.806268909854,108.286084950886));
#83422=CARTESIAN_POINT('Ctrl Pts',(86.6073438841338,776.924074263358,108.327978577234));
#83423=CARTESIAN_POINT('Ctrl Pts',(86.799345208022,777.042874482526,108.37017106729));
#83424=CARTESIAN_POINT('Ctrl Pts',(86.9860289092342,777.15838443928,108.411195004248));
#83425=CARTESIAN_POINT('Ctrl Pts',(87.1720877947107,777.274835274588,108.45250161709));
#83426=CARTESIAN_POINT('Ctrl Pts',(87.3575419166461,777.392271729837,108.49411256191));
#83427=CARTESIAN_POINT('Ctrl Pts',(87.5509199363648,777.514725892203,108.537501417461));
#83428=CARTESIAN_POINT('Ctrl Pts',(87.7436399756386,777.638251699538,108.581221070523));
#83429=CARTESIAN_POINT('Ctrl Pts',(87.9357584155001,777.762942100741,108.625322094426));
#83430=CARTESIAN_POINT('Ctrl Pts',(88.1278768553616,777.887632501944,108.66942311833));
#83431=CARTESIAN_POINT('Ctrl Pts',(88.3193935291358,778.013487920609,108.713905655094));
#83432=CARTESIAN_POINT('Ctrl Pts',(88.5104020101015,778.140638997398,108.758845147568));
#83433=CARTESIAN_POINT('Ctrl Pts',(73.5476386472354,788.511793322588,110.303121350496));
#83434=CARTESIAN_POINT('Ctrl Pts',(73.6485328417201,788.557253210302,110.319188412988));
#83435=CARTESIAN_POINT('Ctrl Pts',(73.7489162064673,788.603615273794,110.335574334926));
#83436=CARTESIAN_POINT('Ctrl Pts',(73.8487392078304,788.650697274009,110.352214706861));
#83437=CARTESIAN_POINT('Ctrl Pts',(74.1035309214589,788.770871015049,110.394688173126));
#83438=CARTESIAN_POINT('Ctrl Pts',(74.355266481156,788.896015030648,110.438918302596));
#83439=CARTESIAN_POINT('Ctrl Pts',(74.6047148824487,789.024747592744,110.484416745817));
#83440=CARTESIAN_POINT('Ctrl Pts',(74.7184820864584,789.083459308589,110.505167452757));
#83441=CARTESIAN_POINT('Ctrl Pts',(74.8317823705978,789.142903575577,110.526177068057));
#83442=CARTESIAN_POINT('Ctrl Pts',(74.9446503073713,789.203009286023,110.547420459854));
#83443=CARTESIAN_POINT('Ctrl Pts',(75.3267059948401,789.406465902505,110.61932891224));
#83444=CARTESIAN_POINT('Ctrl Pts',(75.7039441998201,789.617479744584,110.693908343871));
#83445=CARTESIAN_POINT('Ctrl Pts',(76.0780101827947,789.833468278297,110.77024599984));
#83446=CARTESIAN_POINT('Ctrl Pts',(76.1516852545629,789.876008823139,110.785281267783));
#83447=CARTESIAN_POINT('Ctrl Pts',(76.2252355766988,789.918744947225,110.800385660048));
#83448=CARTESIAN_POINT('Ctrl Pts',(76.2986648253408,789.961670797666,110.815557108025));
#83449=CARTESIAN_POINT('Ctrl Pts',(76.7081990718776,790.201079563819,110.900172266577));
#83450=CARTESIAN_POINT('Ctrl Pts',(77.1139902758252,790.446347379196,110.986858211375));
#83451=CARTESIAN_POINT('Ctrl Pts',(77.5167337817441,790.696396899066,111.075234172333));
#83452=CARTESIAN_POINT('Ctrl Pts',(77.9916855340511,790.991278022859,111.179455139034));
#83453=CARTESIAN_POINT('Ctrl Pts',(78.4624432629204,791.292761109192,111.286009462679));
#83454=CARTESIAN_POINT('Ctrl Pts',(78.9278568223611,791.602604685109,111.395518666228));
#83455=CARTESIAN_POINT('Ctrl Pts',(67.5289020028163,787.735242207091,110.028661911016));
#83456=CARTESIAN_POINT('Ctrl Pts',(67.7061220726526,787.717742978049,110.022477091371));
#83457=CARTESIAN_POINT('Ctrl Pts',(67.883445519993,787.70123378808,110.016642185034));
#83458=CARTESIAN_POINT('Ctrl Pts',(68.0609107392751,787.686085392946,110.011288229635));
#83459=CARTESIAN_POINT('Ctrl Pts',(68.2456467398798,787.670316365394,110.005714921739));
#83460=CARTESIAN_POINT('Ctrl Pts',(68.4305343439629,787.656002508816,110.000655920503));
#83461=CARTESIAN_POINT('Ctrl Pts',(68.6156463726316,787.643845166967,109.99635910454));
#83462=CARTESIAN_POINT('Ctrl Pts',(68.7149270954738,787.637324846838,109.994054602785));
#83463=CARTESIAN_POINT('Ctrl Pts',(68.8142727465984,787.631424983268,109.991969391373));
#83464=CARTESIAN_POINT('Ctrl Pts',(68.9136943681619,787.626253429796,109.990141589392));
#83465=CARTESIAN_POINT('Ctrl Pts',(69.1777263035479,787.612519442652,109.985287533634));
#83466=CARTESIAN_POINT('Ctrl Pts',(69.4422864352835,787.603850726593,109.982223716065));
#83467=CARTESIAN_POINT('Ctrl Pts',(69.7077490719245,787.603862578117,109.982227904797));
#83468=CARTESIAN_POINT('Ctrl Pts',(69.7286265902763,787.603863510189,109.982228234223));
#83469=CARTESIAN_POINT('Ctrl Pts',(69.749509735423,787.603918333592,109.982247610669));
#83470=CARTESIAN_POINT('Ctrl Pts',(69.7703986871635,787.604028793531,109.982286650949));
#83471=CARTESIAN_POINT('Ctrl Pts',(69.9136472752219,787.604786286317,109.982554374532));
#83472=CARTESIAN_POINT('Ctrl Pts',(70.0571734867388,787.608204434059,109.983762463599));
#83473=CARTESIAN_POINT('Ctrl Pts',(70.2010623316121,787.615102231534,109.986200378618));
#83474=CARTESIAN_POINT('Ctrl Pts',(70.344950365047,787.621999990109,109.988638279889));
#83475=CARTESIAN_POINT('Ctrl Pts',(70.4884664923808,787.632385806578,109.992308978842));
#83476=CARTESIAN_POINT('Ctrl Pts',(70.6305534917093,787.64679659127,109.997402237753));
#83477=CARTESIAN_POINT('Ctrl Pts',(70.6883193644943,787.65265533668,109.999472916616));
#83478=CARTESIAN_POINT('Ctrl Pts',(70.7458938079884,787.659184277743,110.0017804653));
#83479=CARTESIAN_POINT('Ctrl Pts',(70.8032735414792,787.666394845197,110.004328923814));
#83480=CARTESIAN_POINT('Ctrl Pts',(70.8870312365736,787.676920173105,110.008048930831));
#83481=CARTESIAN_POINT('Ctrl Pts',(70.9703735131096,787.688901299224,110.012283466193));
#83482=CARTESIAN_POINT('Ctrl Pts',(71.053289968927,787.702374152363,110.017045228358));
#83483=CARTESIAN_POINT('Ctrl Pts',(71.1930103788716,787.725076914381,110.025069152622));
#83484=CARTESIAN_POINT('Ctrl Pts',(71.3315243908326,787.752005750895,110.034586714605));
#83485=CARTESIAN_POINT('Ctrl Pts',(71.4689182867618,787.782858060651,110.045490964787));
#83486=CARTESIAN_POINT('Ctrl Pts',(71.6006684907306,787.812443058411,110.055947304028));
#83487=CARTESIAN_POINT('Ctrl Pts',(71.731393808425,787.845618024237,110.067672459454));
#83488=CARTESIAN_POINT('Ctrl Pts',(71.8612276196213,787.881917432482,110.080501898549));
#83489=CARTESIAN_POINT('Origin',(52.8776183915471,826.387310726428,123.689610751183));
#83490=CARTESIAN_POINT('Origin',(52.8776183915471,887.005734436498,147.235453418339));
#83491=CARTESIAN_POINT('Origin',(51.305620893586,644.631864177561,61.5723267466062));
#83492=CARTESIAN_POINT('Origin',(54.4496157591678,644.63186463643,61.5723269068127));
#83493=CARTESIAN_POINT('Ctrl Pts',(37.2974382339422,740.125373764374,98.7804136939922));
#83494=CARTESIAN_POINT('Ctrl Pts',(37.3237628811582,747.666799047464,98.7691088438472));
#83495=CARTESIAN_POINT('Ctrl Pts',(37.3500875283232,755.208224315958,98.7577942572374));
#83496=CARTESIAN_POINT('Ctrl Pts',(27.6328772087504,768.384899013174,105.310836543429));
#83497=CARTESIAN_POINT('Ctrl Pts',(20.0424170283973,772.22630491262,106.668519365511));
#83498=CARTESIAN_POINT('Ctrl Pts',(13.2983736491593,777.107328840337,108.39363837514));
#83499=CARTESIAN_POINT('Ctrl Pts',(39.7898595278376,740.125373764374,101.14718649664));
#83500=CARTESIAN_POINT('Ctrl Pts',(39.8138889156218,748.116327090208,101.129143881277));
#83501=CARTESIAN_POINT('Ctrl Pts',(39.8379148254437,756.107280410872,101.111093617291));
#83502=CARTESIAN_POINT('Ctrl Pts',(32.8646385077286,769.386484699126,105.664841346626));
#83503=CARTESIAN_POINT('Ctrl Pts',(26.4798669689934,773.811769470219,107.228876241329));
#83504=CARTESIAN_POINT('Ctrl Pts',(21.001327165595,779.233378063583,109.145056107309));
#83505=CARTESIAN_POINT('Ctrl Pts',(42.736298749677,740.125373764374,103.035135355334));
#83506=CARTESIAN_POINT('Ctrl Pts',(42.755886965038,748.454875736532,103.011405038338));
#83507=CARTESIAN_POINT('Ctrl Pts',(42.7754708329722,756.784377710745,102.987668638594));
#83508=CARTESIAN_POINT('Ctrl Pts',(37.9535726725575,770.177423028533,105.944387022298));
#83509=CARTESIAN_POINT('Ctrl Pts',(33.0087739196395,775.040601634335,107.663187140576));
#83510=CARTESIAN_POINT('Ctrl Pts',(28.8582165463779,780.867648688703,109.722662643155));
#83511=CARTESIAN_POINT('Ctrl Pts',(46.0036740905127,740.125373764374,104.339521951214));
#83512=CARTESIAN_POINT('Ctrl Pts',(46.0173362984446,748.681509910258,104.311576914651));
#83513=CARTESIAN_POINT('Ctrl Pts',(46.0309950284494,757.237646063144,104.283626839249));
#83514=CARTESIAN_POINT('Ctrl Pts',(42.9549332988076,770.72138911218,106.136638421123));
#83515=CARTESIAN_POINT('Ctrl Pts',(39.6062998281129,775.87648417527,107.958616329378));
#83516=CARTESIAN_POINT('Ctrl Pts',(36.8253774496378,781.973823505111,110.113622251634));
#83517=CARTESIAN_POINT('Ctrl Pts',(49.4406462410299,740.125373764373,104.999846187002));
#83518=CARTESIAN_POINT('Ctrl Pts',(49.4475586845128,748.795294535209,104.969582331416));
#83519=CARTESIAN_POINT('Ctrl Pts',(49.4544693890487,757.465215315637,104.93931395894));
#83520=CARTESIAN_POINT('Ctrl Pts',(47.9163263691371,770.996800169048,106.233970753627));
#83521=CARTESIAN_POINT('Ctrl Pts',(46.2419590292789,776.297841971512,108.107538433704));
#83522=CARTESIAN_POINT('Ctrl Pts',(44.8514979205924,782.530327410416,110.31030956155));
#83523=CARTESIAN_POINT('Ctrl Pts',(56.3145905420643,740.125373764374,104.999846187002));
#83524=CARTESIAN_POINT('Ctrl Pts',(56.3076780985813,748.79529453521,104.969582331416));
#83525=CARTESIAN_POINT('Ctrl Pts',(56.3007673941054,757.465215315951,104.939313958926));
#83526=CARTESIAN_POINT('Ctrl Pts',(57.8390941374472,770.996830883562,106.233968426735));
#83527=CARTESIAN_POINT('Ctrl Pts',(59.5132774609024,776.297842047978,108.107538445034));
#83528=CARTESIAN_POINT('Ctrl Pts',(60.9037388625016,782.530327410416,110.31030956155));
#83529=CARTESIAN_POINT('Ctrl Pts',(59.7515626925815,740.125373764374,104.339521951214));
#83530=CARTESIAN_POINT('Ctrl Pts',(59.7379004846479,748.681509910457,104.311576914657));
#83531=CARTESIAN_POINT('Ctrl Pts',(59.7242417546954,757.237646064166,104.283626839233));
#83532=CARTESIAN_POINT('Ctrl Pts',(62.8004688354278,770.721450541208,106.136633767339));
#83533=CARTESIAN_POINT('Ctrl Pts',(66.1489366913599,775.876484328201,107.958616352038));
#83534=CARTESIAN_POINT('Ctrl Pts',(68.9298593334563,781.973823505111,110.113622251634));
#83535=CARTESIAN_POINT('Ctrl Pts',(63.0189380334171,740.125373764374,103.035135355334));
#83536=CARTESIAN_POINT('Ctrl Pts',(62.9993498180528,748.454875736928,103.011405038351));
#83537=CARTESIAN_POINT('Ctrl Pts',(62.9797659501571,756.784377712319,102.987668638583));
#83538=CARTESIAN_POINT('Ctrl Pts',(67.8017927169798,770.177499814818,105.944381205068));
#83539=CARTESIAN_POINT('Ctrl Pts',(72.7464626584159,775.0406018255,107.663187168902));
#83540=CARTESIAN_POINT('Ctrl Pts',(76.8970202367163,780.867648688703,109.722662643155));
#83541=CARTESIAN_POINT('Ctrl Pts',(65.9653772552566,740.125373764374,101.14718649664));
#83542=CARTESIAN_POINT('Ctrl Pts',(65.9413478674689,748.116327090604,101.12914388129));
#83543=CARTESIAN_POINT('Ctrl Pts',(65.9173219576676,756.107280412289,101.111093617287));
#83544=CARTESIAN_POINT('Ctrl Pts',(72.8906717647615,769.386546128155,105.664836692843));
#83545=CARTESIAN_POINT('Ctrl Pts',(79.2753696969357,773.81176962315,107.228876263989));
#83546=CARTESIAN_POINT('Ctrl Pts',(84.7539096174991,779.233378063583,109.145056107309));
#83547=CARTESIAN_POINT('Ctrl Pts',(68.4577985491519,740.125373764374,98.7804136939922));
#83548=CARTESIAN_POINT('Ctrl Pts',(68.4314739019359,747.666799047464,98.7691088438472));
#83549=CARTESIAN_POINT('Ctrl Pts',(68.4051492547709,755.208224315958,98.7577942572374));
#83550=CARTESIAN_POINT('Ctrl Pts',(78.1223595743435,768.384899013174,105.310836543429));
#83551=CARTESIAN_POINT('Ctrl Pts',(85.7128197546968,772.22630491262,106.668519365511));
#83552=CARTESIAN_POINT('Ctrl Pts',(92.4568631339348,777.107328840337,108.39363837514));
#83553=CARTESIAN_POINT('Ctrl Pts',(61.1807573575412,737.487748923763,102.682654164686));
#83554=CARTESIAN_POINT('Ctrl Pts',(61.1807573575412,737.490646661967,103.444319534016));
#83555=CARTESIAN_POINT('Ctrl Pts',(61.8796042537708,737.489494249471,103.141409944702));
#83556=CARTESIAN_POINT('Ctrl Pts',(61.1807573575412,736.932983697653,102.684891852733));
#83557=CARTESIAN_POINT('Ctrl Pts',(61.1809509020401,736.958112818667,103.4462282913));
#83558=CARTESIAN_POINT('Ctrl Pts',(61.8795858086402,736.901322056595,103.143655627156));
#83559=CARTESIAN_POINT('Ctrl Pts',(61.1257247484325,736.388809219359,102.712651269588));
#83560=CARTESIAN_POINT('Ctrl Pts',(61.1315244238093,736.439502901679,103.467444860905));
#83561=CARTESIAN_POINT('Ctrl Pts',(61.8199032205241,736.324378385116,103.172000328419));
#83562=CARTESIAN_POINT('Ctrl Pts',(60.9649930899463,735.587567421577,102.788007703544));
#83563=CARTESIAN_POINT('Ctrl Pts',(60.981820887591,735.660697899481,103.527070137866));
#83564=CARTESIAN_POINT('Ctrl Pts',(61.6456182738998,735.474887256523,103.248996797997));
#83565=CARTESIAN_POINT('Ctrl Pts',(60.8982825197972,735.322998250083,102.818743893064));
#83566=CARTESIAN_POINT('Ctrl Pts',(60.9199522152394,735.404098567403,103.551302444857));
#83567=CARTESIAN_POINT('Ctrl Pts',(61.5732848924775,735.19438620833,103.280406636733));
#83568=CARTESIAN_POINT('Ctrl Pts',(60.7381098070039,734.798906562277,102.890642890349));
#83569=CARTESIAN_POINT('Ctrl Pts',(60.7697965738214,734.892509407837,103.608706401083));
#83570=CARTESIAN_POINT('Ctrl Pts',(61.3996158945904,734.638734667783,103.353888537477));
#83571=CARTESIAN_POINT('Ctrl Pts',(60.6447435666911,734.540287656224,102.931744025724));
#83572=CARTESIAN_POINT('Ctrl Pts',(60.6820947269692,734.63910185468,103.641656972148));
#83573=CARTESIAN_POINT('Ctrl Pts',(61.2983842846201,734.364542199337,103.395897601165));
#83574=CARTESIAN_POINT('Ctrl Pts',(60.3311877109548,733.788965343319,103.065815369317));
#83575=CARTESIAN_POINT('Ctrl Pts',(60.3866007381818,733.90349987622,103.749743252493));
#83576=CARTESIAN_POINT('Ctrl Pts',(60.958418488567,733.567976616374,103.532937356843));
#83577=CARTESIAN_POINT('Ctrl Pts',(60.0762481608013,733.314787297901,103.170272691237));
#83578=CARTESIAN_POINT('Ctrl Pts',(60.1442935975249,733.43158872955,103.835289846909));
#83579=CARTESIAN_POINT('Ctrl Pts',(60.6820115486397,733.065244427314,103.639715549476));
#83580=CARTESIAN_POINT('Ctrl Pts',(59.6252595505857,732.641678750238,103.34014197422));
#83581=CARTESIAN_POINT('Ctrl Pts',(59.7019880275959,732.748764058181,103.979323506016));
#83582=CARTESIAN_POINT('Ctrl Pts',(60.1930545417937,732.351602501481,103.813365835641));
#83583=CARTESIAN_POINT('Ctrl Pts',(59.4626751707199,732.42299274092,103.399206463738));
#83584=CARTESIAN_POINT('Ctrl Pts',(59.5432261215717,732.527629412984,104.029360742554));
#83585=CARTESIAN_POINT('Ctrl Pts',(60.0167833769942,732.119747616557,103.873746066075));
#83586=CARTESIAN_POINT('Ctrl Pts',(59.1204278078766,732.006685289033,103.517848709794));
#83587=CARTESIAN_POINT('Ctrl Pts',(59.2067025055535,732.105084204966,104.130742222411));
#83588=CARTESIAN_POINT('Ctrl Pts',(59.6457267679576,731.678370883142,103.995032772172));
#83589=CARTESIAN_POINT('Ctrl Pts',(58.9402283766131,731.808090210619,103.577647519589));
#83590=CARTESIAN_POINT('Ctrl Pts',(59.0287912923034,731.902472536105,104.182228416435));
#83591=CARTESIAN_POINT('Ctrl Pts',(59.4503597030529,731.467816768717,104.056165212955));
#83592=CARTESIAN_POINT('Ctrl Pts',(58.3726318318003,731.240067038385,103.756066170503));
#83593=CARTESIAN_POINT('Ctrl Pts',(58.4698094265145,731.326084508652,104.335651640274));
#83594=CARTESIAN_POINT('Ctrl Pts',(58.8349904857801,730.865588269116,104.238564540963));
#83595=CARTESIAN_POINT('Ctrl Pts',(57.9571860672587,730.897183698347,103.874066021539));
#83596=CARTESIAN_POINT('Ctrl Pts',(58.0545173909263,730.970975749466,104.439583656015));
#83597=CARTESIAN_POINT('Ctrl Pts',(58.3845815167719,730.50205711538,104.35919918526));
#83598=CARTESIAN_POINT('Ctrl Pts',(57.0546474823471,730.291222974584,104.09363972318));
#83599=CARTESIAN_POINT('Ctrl Pts',(57.1452072958055,730.343809488644,104.634257597851));
#83600=CARTESIAN_POINT('Ctrl Pts',(57.4060930165886,729.859606532818,104.583677606931));
#83601=CARTESIAN_POINT('Ctrl Pts',(56.5798557797467,730.036068845983,104.192221461437));
#83602=CARTESIAN_POINT('Ctrl Pts',(56.6630499090508,730.07624833159,104.723128595975));
#83603=CARTESIAN_POINT('Ctrl Pts',(56.891349737683,729.58908748456,104.684462416802));
#83604=CARTESIAN_POINT('Ctrl Pts',(55.8320913800377,729.723329995616,104.31634306445));
#83605=CARTESIAN_POINT('Ctrl Pts',(55.8988443964391,729.748595063217,104.83536748852));
#83606=CARTESIAN_POINT('Ctrl Pts',(56.0806674621493,729.257516067056,104.811358313865));
#83607=CARTESIAN_POINT('Ctrl Pts',(55.5768657910945,729.630840873543,104.353761308194));
#83608=CARTESIAN_POINT('Ctrl Pts',(55.6386235138817,729.651816413208,104.869210413042));
#83609=CARTESIAN_POINT('Ctrl Pts',(55.8039673529785,729.159457417016,104.84961300737));
#83610=CARTESIAN_POINT('Ctrl Pts',(55.0538963656352,729.470220949813,104.419458032274));
#83611=CARTESIAN_POINT('Ctrl Pts',(55.1051328898357,729.483964632797,104.928620527236));
#83612=CARTESIAN_POINT('Ctrl Pts',(55.2369964086371,728.989165252824,104.916778416946));
#83613=CARTESIAN_POINT('Ctrl Pts',(54.7851014678237,729.402035764568,104.447762052157));
#83614=CARTESIAN_POINT('Ctrl Pts',(54.8302761550589,729.412455456162,104.954337757205));
#83615=CARTESIAN_POINT('Ctrl Pts',(54.9455860846029,728.916874079002,104.945715242535));
#83616=CARTESIAN_POINT('Ctrl Pts',(53.9789685647692,729.239738639677,104.515565791446));
#83617=CARTESIAN_POINT('Ctrl Pts',(54.0082608735909,729.243006873554,105.015710454987));
#83618=CARTESIAN_POINT('Ctrl Pts',(54.0716288994501,728.744803714473,105.015034956347));
#83619=CARTESIAN_POINT('Ctrl Pts',(53.4361694424363,729.185298984108,104.538875891959));
#83620=CARTESIAN_POINT('Ctrl Pts',(53.4496161456551,729.185332137448,105.037159942866));
#83621=CARTESIAN_POINT('Ctrl Pts',(53.4831622362376,728.68708580134,105.038866301411));
#83622=CARTESIAN_POINT('Ctrl Pts',(52.6138504499604,729.184275098991,104.539310798033));
#83623=CARTESIAN_POINT('Ctrl Pts',(52.6075136823759,729.184259004066,105.037555700089));
#83624=CARTESIAN_POINT('Ctrl Pts',(52.5916587586709,728.686000260307,105.039310932355));
#83625=CARTESIAN_POINT('Ctrl Pts',(52.3370055315343,729.197621489013,104.533629664186));
#83626=CARTESIAN_POINT('Ctrl Pts',(52.3236418415964,729.198286299786,105.032370697334));
#83627=CARTESIAN_POINT('Ctrl Pts',(52.2915219403397,728.700150345916,105.033502765101));
#83628=CARTESIAN_POINT('Ctrl Pts',(51.7870175816165,729.251908649559,104.510663500195));
#83629=CARTESIAN_POINT('Ctrl Pts',(51.7606605684528,729.255166215058,105.01148612717));
#83630=CARTESIAN_POINT('Ctrl Pts',(51.695261374346,728.757706580342,105.010023081021));
#83631=CARTESIAN_POINT('Ctrl Pts',(51.5157722085268,729.292506544129,104.493525021637));
#83632=CARTESIAN_POINT('Ctrl Pts',(51.482794014801,729.297802076253,104.995868437499));
#83633=CARTESIAN_POINT('Ctrl Pts',(51.4011949421538,728.800749207109,104.99250139366));
#83634=CARTESIAN_POINT('Ctrl Pts',(50.7128226027646,729.453210985855,104.426373808672));
#83635=CARTESIAN_POINT('Ctrl Pts',(50.659795046494,729.466453778642,104.934771634819));
#83636=CARTESIAN_POINT('Ctrl Pts',(50.5306889001451,728.971130979045,104.923848793536));
#83637=CARTESIAN_POINT('Ctrl Pts',(50.1916745911165,729.611899298158,104.360612213778));
#83638=CARTESIAN_POINT('Ctrl Pts',(50.12567436779,729.634048243943,104.874648394563));
#83639=CARTESIAN_POINT('Ctrl Pts',(49.9656928764268,729.13937521528,104.856616947866));
#83640=CARTESIAN_POINT('Ctrl Pts',(49.1784470909822,730.033928888822,104.193027849295));
#83641=CARTESIAN_POINT('Ctrl Pts',(49.0951325681358,730.074079498543,104.723829183479));
#83642=CARTESIAN_POINT('Ctrl Pts',(48.8672111471257,729.586818662584,104.68528682235));
#83643=CARTESIAN_POINT('Ctrl Pts',(48.7027982162775,730.290339076695,104.094018837663));
#83644=CARTESIAN_POINT('Ctrl Pts',(48.6124016060787,730.342788849866,104.634629987258));
#83645=CARTESIAN_POINT('Ctrl Pts',(48.3515385393433,729.858669408582,104.584065199752));
#83646=CARTESIAN_POINT('Ctrl Pts',(48.0320729801837,730.739768842028,103.931077496968));
#83647=CARTESIAN_POINT('Ctrl Pts',(47.9412391106486,730.804777879081,104.491144118451));
#83648=CARTESIAN_POINT('Ctrl Pts',(47.624370852353,730.335163020942,104.417484147719));
#83649=CARTESIAN_POINT('Ctrl Pts',(47.8156813845902,730.900472889617,103.874347068112));
#83650=CARTESIAN_POINT('Ctrl Pts',(47.7238916112771,730.970992477136,104.44101889853));
#83651=CARTESIAN_POINT('Ctrl Pts',(47.389768913752,730.505544375239,104.359486753798));
#83652=CARTESIAN_POINT('Ctrl Pts',(47.3973220744942,731.244211137401,103.757431495977));
#83653=CARTESIAN_POINT('Ctrl Pts',(47.3052179858964,731.324859887805,104.338424006517));
#83654=CARTESIAN_POINT('Ctrl Pts',(46.9362012231384,730.869981918465,104.239960877132));
#83655=CARTESIAN_POINT('Ctrl Pts',(47.1963552596799,731.426598283342,103.697495897006));
#83656=CARTESIAN_POINT('Ctrl Pts',(47.1049878887212,731.512287596286,104.286106464377));
#83657=CARTESIAN_POINT('Ctrl Pts',(46.718320595536,731.063352088166,104.178687517304));
#83658=CARTESIAN_POINT('Ctrl Pts',(46.6264326450995,731.996527007362,103.518418939747));
#83659=CARTESIAN_POINT('Ctrl Pts',(46.5346004165947,732.099997089064,104.129613768312));
#83660=CARTESIAN_POINT('Ctrl Pts',(46.100429550514,731.667600888059,103.995615183088));
#83661=CARTESIAN_POINT('Ctrl Pts',(46.2862941213449,732.409628760885,103.398906187144));
#83662=CARTESIAN_POINT('Ctrl Pts',(46.2017494877472,732.520766276813,104.02759395401));
#83663=CARTESIAN_POINT('Ctrl Pts',(45.7316592763466,732.105578881428,103.873438096382));
#83664=CARTESIAN_POINT('Ctrl Pts',(45.8352318176212,733.080982096968,103.229178588061));
#83665=CARTESIAN_POINT('Ctrl Pts',(45.7665725264928,733.190705968255,103.886013091801));
#83666=CARTESIAN_POINT('Ctrl Pts',(45.2426224560662,732.817359900666,103.699932564948));
#83667=CARTESIAN_POINT('Ctrl Pts',(45.6941245720904,733.31484502054,103.173914949951));
#83668=CARTESIAN_POINT('Ctrl Pts',(45.6304395608493,733.424882397453,103.840011653334));
#83669=CARTESIAN_POINT('Ctrl Pts',(45.0896344539317,733.065305626168,103.643439885389));
#83670=CARTESIAN_POINT('Ctrl Pts',(45.4370595664475,733.792644756091,103.070197444028));
#83671=CARTESIAN_POINT('Ctrl Pts',(45.3833924746706,733.900859143644,103.754294935155));
#83672=CARTESIAN_POINT('Ctrl Pts',(44.8109232393786,733.571877596802,103.537418520231));
#83673=CARTESIAN_POINT('Ctrl Pts',(45.3208753235868,734.036579304987,103.021686463586));
#83674=CARTESIAN_POINT('Ctrl Pts',(45.2728079392524,734.142444713245,103.714681228453));
#83675=CARTESIAN_POINT('Ctrl Pts',(44.6849544916996,733.830501442806,103.487831436724));
#83676=CARTESIAN_POINT('Ctrl Pts',(45.0086600428394,734.783512511873,102.888228488882));
#83677=CARTESIAN_POINT('Ctrl Pts',(44.9743839861276,734.884162275861,103.605552967253));
#83678=CARTESIAN_POINT('Ctrl Pts',(44.3464422296916,734.622413615477,103.351418560461));
#83679=CARTESIAN_POINT('Ctrl Pts',(44.8485632569221,735.301485450629,102.81531169835));
#83680=CARTESIAN_POINT('Ctrl Pts',(44.8268749830078,735.387060666504,103.548333060095));
#83681=CARTESIAN_POINT('Ctrl Pts',(44.1728555580203,735.171577946915,103.276895349789));
#83682=CARTESIAN_POINT('Ctrl Pts',(44.6301364121208,736.381170716927,102.712981257937));
#83683=CARTESIAN_POINT('Ctrl Pts',(44.6242435666643,736.43229980519,103.467685458753));
#83684=CARTESIAN_POINT('Ctrl Pts',(43.93601074888,736.316279906073,103.172337185597));
#83685=CARTESIAN_POINT('Ctrl Pts',(44.574479425553,736.934722944003,102.684884837068));
#83686=CARTESIAN_POINT('Ctrl Pts',(44.574286483178,736.959771156344,103.446222347099));
#83687=CARTESIAN_POINT('Ctrl Pts',(43.8756509159712,736.903165979843,103.143648586643));
#83688=CARTESIAN_POINT('Ctrl Pts',(44.574479425553,737.487748923763,102.682654164686));
#83689=CARTESIAN_POINT('Ctrl Pts',(44.574479425553,737.490646661967,103.444319534016));
#83690=CARTESIAN_POINT('Ctrl Pts',(43.8756325293234,737.489494249471,103.141409944702));
#83691=CARTESIAN_POINT('Origin',(61.1807573575412,751.59614455564,112.60871186179));
#83692=CARTESIAN_POINT('',(61.1807573575412,751.59614455564,112.60871186179));
#83693=CARTESIAN_POINT('Origin',(44.574479425553,751.59614455564,112.60871186179));
#83694=CARTESIAN_POINT('',(44.574479425553,751.59614455564,112.60871186179));
#83695=CARTESIAN_POINT('Origin',(52.8776183915471,751.59614455564,112.60871186179));
#83696=CARTESIAN_POINT('Origin',(52.8776183915471,827.175936191914,121.458286566849));
#83697=CARTESIAN_POINT('Origin',(52.8776183915471,825.559694878252,125.51834395973));
#83698=CARTESIAN_POINT('Origin',(52.8776183915471,827.175936191914,121.458286566849));
#83699=CARTESIAN_POINT('Origin',(52.8776183915471,825.559694878252,125.51834395973));
#83700=CARTESIAN_POINT('Origin',(52.8776183915471,827.175936191914,121.458286566849));
#83701=CARTESIAN_POINT('Origin',(52.8776183915471,825.559694878252,125.51834395973));
#83702=CARTESIAN_POINT('Origin',(52.8776183915471,827.175936191914,121.458286566849));
#83703=CARTESIAN_POINT('Origin',(52.8776183915471,825.559694878252,125.51834395973));
#83704=CARTESIAN_POINT('Origin',(52.8776183915471,827.175936191914,121.458286566849));
#83705=CARTESIAN_POINT('Origin',(52.8776183915471,825.559694878252,125.51834395973));
#83706=CARTESIAN_POINT('Origin',(52.8776183915471,827.175936191914,121.458286566849));
#83707=CARTESIAN_POINT('Origin',(52.8776183915471,825.559694878252,125.51834395973));
#83708=CARTESIAN_POINT('Origin',(52.8776183915471,827.175936191914,121.458286566849));
#83709=CARTESIAN_POINT('Origin',(52.8776183915471,825.559694878252,125.51834395973));
#83710=CARTESIAN_POINT('Origin',(52.8776183915471,827.175936191914,121.458286566849));
#83711=CARTESIAN_POINT('Origin',(52.8776183915471,825.559694878252,125.51834395973));
#83712=CARTESIAN_POINT('Origin',(52.8776183915471,827.175936191914,121.458286566849));
#83713=CARTESIAN_POINT('Origin',(52.8776183915471,825.559694878252,125.51834395973));
#83714=CARTESIAN_POINT('Origin',(52.8776183915471,827.175936191914,121.458286566849));
#83715=CARTESIAN_POINT('Origin',(52.8776183915471,825.559694878252,125.51834395973));
#83716=CARTESIAN_POINT('Origin',(52.8776183915471,827.175936191914,121.458286566849));
#83717=CARTESIAN_POINT('Origin',(52.8776183915471,825.559694878252,125.51834395973));
#83718=CARTESIAN_POINT('Origin',(52.8776183915471,827.175936191914,121.458286566849));
#83719=CARTESIAN_POINT('Origin',(52.8776183915471,825.559694878252,125.51834395973));
#83720=CARTESIAN_POINT('Origin',(52.8776183915471,827.175936191914,121.458286566849));
#83721=CARTESIAN_POINT('Origin',(52.8776183915471,825.559694878252,125.51834395973));
#83722=CARTESIAN_POINT('Origin',(52.8776183915471,827.175936191914,121.458286566849));
#83723=CARTESIAN_POINT('Origin',(52.8776183915471,825.559694878252,125.51834395973));
#83724=CARTESIAN_POINT('Origin',(52.8776183915471,827.175936191914,121.458286566849));
#83725=CARTESIAN_POINT('Origin',(52.8776183915471,825.559694878252,125.51834395973));
#83726=CARTESIAN_POINT('Origin',(52.8776183915471,827.175936191914,121.458286566849));
#83727=CARTESIAN_POINT('Origin',(52.8776183915471,825.559694878252,125.51834395973));
#83728=CARTESIAN_POINT('Origin',(52.8776183915471,827.175936191914,121.458286566849));
#83729=CARTESIAN_POINT('Origin',(52.8776183915471,825.559694878252,125.51834395973));
#83730=CARTESIAN_POINT('Origin',(52.8776183915471,827.175936191914,121.458286566849));
#83731=CARTESIAN_POINT('Origin',(52.8776183915471,825.559694878252,125.51834395973));
#83732=CARTESIAN_POINT('Origin',(52.8776183915471,827.175936191914,121.458286566849));
#83733=CARTESIAN_POINT('Origin',(52.8776183915471,825.559694878252,125.51834395973));
#83734=CARTESIAN_POINT('Origin',(52.8776183915471,827.175936191914,121.458286566849));
#83735=CARTESIAN_POINT('Origin',(52.8776183915471,825.559694878252,125.51834395973));
#83736=CARTESIAN_POINT('Origin',(52.8776183915471,827.175936191914,121.458286566849));
#83737=CARTESIAN_POINT('Origin',(52.8776183915471,825.559694878252,125.51834395973));
#83738=CARTESIAN_POINT('Origin',(52.8776183915471,827.175936191914,121.458286566849));
#83739=CARTESIAN_POINT('Origin',(52.8776183915471,825.559694878252,125.51834395973));
#83740=CARTESIAN_POINT('Origin',(52.8776183915471,827.175936191914,121.458286566849));
#83741=CARTESIAN_POINT('Origin',(52.8776183915471,825.559694878252,125.51834395973));
#83742=CARTESIAN_POINT('Origin',(52.8776183915471,827.175936191914,121.458286566849));
#83743=CARTESIAN_POINT('Origin',(52.8776183915471,825.559694878252,125.51834395973));
#83744=CARTESIAN_POINT('Origin',(52.8776183915471,827.175936191914,121.458286566849));
#83745=CARTESIAN_POINT('Origin',(52.8776183915471,825.559694878252,125.51834395973));
#83746=CARTESIAN_POINT('Origin',(52.8776183915471,827.175936191914,121.458286566849));
#83747=CARTESIAN_POINT('Origin',(52.8776183915471,825.559694878252,125.51834395973));
#83748=CARTESIAN_POINT('Origin',(52.8776183915471,827.175936191914,121.458286566849));
#83749=CARTESIAN_POINT('Origin',(52.8776183915471,825.559694878252,125.51834395973));
#83750=CARTESIAN_POINT('Origin',(52.8776183915471,827.175936191914,121.458286566849));
#83751=CARTESIAN_POINT('Origin',(52.8776183915471,825.559694878252,125.51834395973));
#83752=CARTESIAN_POINT('Origin',(52.8776183915471,827.175936191914,121.458286566849));
#83753=CARTESIAN_POINT('Origin',(52.8776183915471,825.559694878252,125.51834395973));
#83754=CARTESIAN_POINT('Origin',(52.8776183915471,827.175936191914,121.458286566849));
#83755=CARTESIAN_POINT('Origin',(52.8776183915471,825.559694878252,125.51834395973));
#83756=CARTESIAN_POINT('Origin',(52.8776183915471,827.175936191914,121.458286566849));
#83757=CARTESIAN_POINT('Origin',(52.8776183915471,825.559694878252,125.51834395973));
#83758=CARTESIAN_POINT('Origin',(52.8776183915471,827.175936191914,121.458286566849));
#83759=CARTESIAN_POINT('Origin',(52.8776183915471,825.559694878252,125.51834395973));
#83760=CARTESIAN_POINT('Origin',(52.8776183915471,827.175936191914,121.458286566849));
#83761=CARTESIAN_POINT('Origin',(52.8776183915471,825.559694878252,125.51834395973));
#83762=CARTESIAN_POINT('Origin',(52.8776183915471,827.175936191914,121.458286566849));
#83763=CARTESIAN_POINT('Origin',(52.8776183915471,825.559694878252,125.51834395973));
#83764=CARTESIAN_POINT('Origin',(52.8776183915471,827.175936191914,121.458286566849));
#83765=CARTESIAN_POINT('Origin',(52.8776183915471,825.559694878252,125.51834395973));
#83766=CARTESIAN_POINT('Origin',(52.8776183915471,827.175936191914,121.458286566849));
#83767=CARTESIAN_POINT('Origin',(52.8776183915471,825.559694878252,125.51834395973));
#83768=CARTESIAN_POINT('Origin',(52.8776183915471,827.175936191914,121.458286566849));
#83769=CARTESIAN_POINT('Origin',(52.8776183915471,825.559694878252,125.51834395973));
#83770=CARTESIAN_POINT('Origin',(52.8776183915471,827.175936191914,121.458286566849));
#83771=CARTESIAN_POINT('Origin',(52.8776183915471,825.559694878252,125.51834395973));
#83772=CARTESIAN_POINT('Origin',(52.8776183915471,827.175936191914,121.458286566849));
#83773=CARTESIAN_POINT('Origin',(52.8776183915471,825.559694878252,125.51834395973));
#83774=CARTESIAN_POINT('Origin',(52.8776183915471,827.175936191914,121.458286566849));
#83775=CARTESIAN_POINT('Origin',(52.8776183915471,825.559694878252,125.51834395973));
#83776=CARTESIAN_POINT('Origin',(52.8776183915471,827.175936191914,121.458286566849));
#83777=CARTESIAN_POINT('Origin',(52.8776183915471,825.559694878252,125.51834395973));
#83778=CARTESIAN_POINT('Origin',(52.8776183915471,827.175936191914,121.458286566849));
#83779=CARTESIAN_POINT('Origin',(52.8776183915471,825.559694878252,125.51834395973));
#83780=CARTESIAN_POINT('Origin',(52.8776183915471,827.175936191914,121.458286566849));
#83781=CARTESIAN_POINT('Origin',(52.8776183915471,825.559694878252,125.51834395973));
#83782=CARTESIAN_POINT('Origin',(52.8776183915471,827.175936191914,121.458286566849));
#83783=CARTESIAN_POINT('Origin',(52.8776183915471,825.559694878252,125.51834395973));
#83784=CARTESIAN_POINT('Origin',(52.8776183915471,827.175936191914,121.458286566849));
#83785=CARTESIAN_POINT('Origin',(52.8776183915471,825.559694878252,125.51834395973));
#83786=CARTESIAN_POINT('Origin',(52.8776183915471,827.175936191914,121.458286566849));
#83787=CARTESIAN_POINT('Origin',(52.8776183915471,825.559694878252,125.51834395973));
#83788=CARTESIAN_POINT('Origin',(52.8776183915471,827.175936191914,121.458286566849));
#83789=CARTESIAN_POINT('Origin',(52.8776183915471,825.559694878252,125.51834395973));
#83790=CARTESIAN_POINT('Origin',(52.8776183915471,827.175936191914,121.458286566849));
#83791=CARTESIAN_POINT('Origin',(52.8776183915471,825.559694878252,125.51834395973));
#83792=CARTESIAN_POINT('Origin',(52.8776183915471,827.175936191914,121.458286566849));
#83793=CARTESIAN_POINT('Origin',(52.8776183915471,825.559694878252,125.51834395973));
#83794=CARTESIAN_POINT('Origin',(52.8776183915471,827.175936191914,121.458286566849));
#83795=CARTESIAN_POINT('Origin',(52.8776183915471,825.559694878252,125.51834395973));
#83796=CARTESIAN_POINT('Origin',(52.8776183915471,827.175936191914,121.458286566849));
#83797=CARTESIAN_POINT('Origin',(52.8776183915471,825.559694878252,125.51834395973));
#83798=CARTESIAN_POINT('Origin',(52.8776183915471,827.175936191914,121.458286566849));
#83799=CARTESIAN_POINT('Origin',(52.8776183915471,825.559694878252,125.51834395973));
#83800=CARTESIAN_POINT('Origin',(52.8776183915471,827.175936191914,121.458286566849));
#83801=CARTESIAN_POINT('Origin',(52.8776183915471,825.559694878252,125.51834395973));
#83802=CARTESIAN_POINT('Origin',(52.8776183915471,827.175936191914,121.458286566849));
#83803=CARTESIAN_POINT('Origin',(52.8776183915471,825.559694878252,125.51834395973));
#83804=CARTESIAN_POINT('Origin',(52.8776183915471,827.175936191914,121.458286566849));
#83805=CARTESIAN_POINT('Origin',(52.8776183915471,825.559694878252,125.51834395973));
#83806=CARTESIAN_POINT('Origin',(52.8776183915471,827.175936191914,121.458286566849));
#83807=CARTESIAN_POINT('Origin',(52.8776183915471,825.559694878252,125.51834395973));
#83808=CARTESIAN_POINT('Origin',(52.8776183915471,827.175936191914,121.458286566849));
#83809=CARTESIAN_POINT('Origin',(52.8776183915471,825.559694878252,125.51834395973));
#83810=CARTESIAN_POINT('Origin',(52.8776183915471,827.175936191914,121.458286566849));
#83811=CARTESIAN_POINT('Origin',(52.8776183915471,825.559694878252,125.51834395973));
#83812=CARTESIAN_POINT('Origin',(52.8776183915471,827.175936191914,121.458286566849));
#83813=CARTESIAN_POINT('Origin',(52.8776183915471,825.559694878252,125.51834395973));
#83814=CARTESIAN_POINT('Origin',(52.8776183915471,827.175936191914,121.458286566849));
#83815=CARTESIAN_POINT('Origin',(52.8776183915471,825.559694878252,125.51834395973));
#83816=CARTESIAN_POINT('Origin',(52.8776183915471,827.175936191914,121.458286566849));
#83817=CARTESIAN_POINT('Origin',(52.8776183915471,825.559694878252,125.51834395973));
#83818=CARTESIAN_POINT('Origin',(52.8776183915471,827.175936191914,121.458286566849));
#83819=CARTESIAN_POINT('Origin',(52.8776183915471,825.559694878252,125.51834395973));
#83820=CARTESIAN_POINT('Origin',(52.8776183915471,827.175936191914,121.458286566849));
#83821=CARTESIAN_POINT('Origin',(52.8776183915471,825.559694878252,125.51834395973));
#83822=CARTESIAN_POINT('Origin',(52.8776183915471,827.175936191914,121.458286566849));
#83823=CARTESIAN_POINT('Origin',(52.8776183915471,825.559694878252,125.51834395973));
#83824=CARTESIAN_POINT('Origin',(52.8776183915471,827.175936191914,121.458286566849));
#83825=CARTESIAN_POINT('Origin',(52.8776183915471,825.559694878252,125.51834395973));
#83826=CARTESIAN_POINT('Origin',(52.8776183915471,827.175936191914,121.458286566849));
#83827=CARTESIAN_POINT('Origin',(52.8776183915471,825.559694878252,125.51834395973));
#83828=CARTESIAN_POINT('Origin',(52.8776183915471,827.175936191914,121.458286566849));
#83829=CARTESIAN_POINT('Origin',(52.8776183915471,825.559694878252,125.51834395973));
#83830=CARTESIAN_POINT('Origin',(52.8776183915471,827.175936191914,121.458286566849));
#83831=CARTESIAN_POINT('Origin',(52.8776183915471,825.559694878252,125.51834395973));
#83832=CARTESIAN_POINT('Origin',(52.8776183915471,827.175936191914,121.458286566849));
#83833=CARTESIAN_POINT('Origin',(52.8776183915471,825.559694878252,125.51834395973));
#83834=CARTESIAN_POINT('Origin',(52.8776183915471,827.175936191914,121.458286566849));
#83835=CARTESIAN_POINT('Origin',(52.8776183915471,825.559694878252,125.51834395973));
#83836=CARTESIAN_POINT('Origin',(52.8776183915471,827.175936191914,121.458286566849));
#83837=CARTESIAN_POINT('Origin',(52.8776183915471,825.559694878252,125.51834395973));
#83838=CARTESIAN_POINT('Origin',(52.8776183915471,827.175936191914,121.458286566849));
#83839=CARTESIAN_POINT('Origin',(52.8776183915471,825.559694878252,125.51834395973));
#83840=CARTESIAN_POINT('Origin',(52.8776183915471,827.175936191914,121.458286566849));
#83841=CARTESIAN_POINT('Origin',(52.8776183915471,825.559694878252,125.51834395973));
#83842=CARTESIAN_POINT('Origin',(52.8776183915471,827.175936191914,121.458286566849));
#83843=CARTESIAN_POINT('Origin',(52.8776183915471,825.559694878252,125.51834395973));
#83844=CARTESIAN_POINT('Origin',(52.8776183915471,827.175936191914,121.458286566849));
#83845=CARTESIAN_POINT('Origin',(52.8776183915471,825.559694878252,125.51834395973));
#83846=CARTESIAN_POINT('Origin',(52.8776183915471,827.175936191914,121.458286566849));
#83847=CARTESIAN_POINT('Origin',(52.8776183915471,825.559694878252,125.51834395973));
#83848=CARTESIAN_POINT('Origin',(52.8776183915471,827.175936191914,121.458286566849));
#83849=CARTESIAN_POINT('Origin',(52.8776183915471,825.559694878252,125.51834395973));
#83850=CARTESIAN_POINT('Origin',(52.8776183915471,827.175936191914,121.458286566849));
#83851=CARTESIAN_POINT('Origin',(52.8776183915471,825.559694878252,125.51834395973));
#83852=CARTESIAN_POINT('Origin',(52.8776183915471,827.175936191914,121.458286566849));
#83853=CARTESIAN_POINT('Origin',(52.8776183915471,825.559694878252,125.51834395973));
#83854=CARTESIAN_POINT('Origin',(52.8776183915471,827.175936191914,121.458286566849));
#83855=CARTESIAN_POINT('Origin',(52.8776183915471,825.559694878252,125.51834395973));
#83856=CARTESIAN_POINT('Origin',(52.8776183915471,827.175936191914,121.458286566849));
#83857=CARTESIAN_POINT('Origin',(52.8776183915471,825.559694878252,125.51834395973));
#83858=CARTESIAN_POINT('Origin',(52.8776183915471,827.175936191914,121.458286566849));
#83859=CARTESIAN_POINT('Origin',(52.8776183915471,825.559694878252,125.51834395973));
#83860=CARTESIAN_POINT('Origin',(52.8776183915471,827.175936191914,121.458286566849));
#83861=CARTESIAN_POINT('Origin',(52.8776183915471,825.559694878252,125.51834395973));
#83862=CARTESIAN_POINT('Origin',(52.8776183915471,827.175936191914,121.458286566849));
#83863=CARTESIAN_POINT('Origin',(52.8776183915471,825.559694878252,125.51834395973));
#83864=CARTESIAN_POINT('Origin',(52.8776183915471,827.175936191914,121.458286566849));
#83865=CARTESIAN_POINT('Origin',(52.8776183915471,825.559694878252,125.51834395973));
#83866=CARTESIAN_POINT('Origin',(52.8776183915471,827.175936191914,121.458286566849));
#83867=CARTESIAN_POINT('Origin',(52.8776183915471,825.559694878252,125.51834395973));
#83868=CARTESIAN_POINT('Origin',(52.8776183915471,827.175936191914,121.458286566849));
#83869=CARTESIAN_POINT('Origin',(52.8776183915471,825.559694878252,125.51834395973));
#83870=CARTESIAN_POINT('Origin',(52.8776183915471,827.175936191914,121.458286566849));
#83871=CARTESIAN_POINT('Origin',(52.8776183915471,825.559694878252,125.51834395973));
#83872=CARTESIAN_POINT('Origin',(52.8776183915471,827.175936191914,121.458286566849));
#83873=CARTESIAN_POINT('Origin',(52.8776183915471,825.559694878252,125.51834395973));
#83874=CARTESIAN_POINT('Origin',(52.8776183915471,827.175936191914,121.458286566849));
#83875=CARTESIAN_POINT('Origin',(52.8776183915471,825.559694878252,125.51834395973));
#83876=CARTESIAN_POINT('Origin',(52.8776183915471,827.175936191914,121.458286566849));
#83877=CARTESIAN_POINT('Origin',(52.8776183915471,825.559694878252,125.51834395973));
#83878=CARTESIAN_POINT('Origin',(52.8776183915471,827.175936191914,121.458286566849));
#83879=CARTESIAN_POINT('Origin',(52.8776183915471,825.559694878252,125.51834395973));
#83880=CARTESIAN_POINT('Origin',(52.8776183915471,827.175936191914,121.458286566849));
#83881=CARTESIAN_POINT('Origin',(52.8776183915471,825.559694878252,125.51834395973));
#83882=CARTESIAN_POINT('Origin',(52.8776183915471,827.175936191914,121.458286566849));
#83883=CARTESIAN_POINT('Origin',(52.8776183915471,825.559694878252,125.51834395973));
#83884=CARTESIAN_POINT('Origin',(52.8776183915471,827.175936191914,121.458286566849));
#83885=CARTESIAN_POINT('Origin',(52.8776183915471,825.559694878252,125.51834395973));
#83886=CARTESIAN_POINT('Origin',(52.8776183915471,827.175936191914,121.458286566849));
#83887=CARTESIAN_POINT('Origin',(52.8776183915471,825.559694878252,125.51834395973));
#83888=CARTESIAN_POINT('Origin',(52.8776183915471,827.175936191914,121.458286566849));
#83889=CARTESIAN_POINT('Origin',(52.8776183915471,825.559694878252,125.51834395973));
#83890=CARTESIAN_POINT('Origin',(52.8776183915471,827.175936191914,121.458286566849));
#83891=CARTESIAN_POINT('Origin',(52.8776183915471,825.559694878252,125.51834395973));
#83892=CARTESIAN_POINT('Origin',(52.8776183915471,827.175936191914,121.458286566849));
#83893=CARTESIAN_POINT('Origin',(52.8776183915471,825.559694878252,125.51834395973));
#83894=CARTESIAN_POINT('Origin',(52.8776183915471,827.175936191914,121.458286566849));
#83895=CARTESIAN_POINT('Origin',(52.8776183915471,825.559694878252,125.51834395973));
#83896=CARTESIAN_POINT('Origin',(52.8776183915471,827.175936191914,121.458286566849));
#83897=CARTESIAN_POINT('Origin',(52.8776183915471,825.559694878252,125.51834395973));
#83898=CARTESIAN_POINT('Origin',(52.8776183915471,827.175936191914,121.458286566849));
#83899=CARTESIAN_POINT('Origin',(52.8776183915471,825.559694878252,125.51834395973));
#83900=CARTESIAN_POINT('Origin',(52.8776183915471,827.175936191914,121.458286566849));
#83901=CARTESIAN_POINT('Origin',(52.8776183915471,825.559694878252,125.51834395973));
#83902=CARTESIAN_POINT('Origin',(52.8776183915471,827.175936191914,121.458286566849));
#83903=CARTESIAN_POINT('Origin',(52.8776183915471,825.559694878252,125.51834395973));
#83904=CARTESIAN_POINT('Origin',(52.8776183915471,827.175936191914,121.458286566849));
#83905=CARTESIAN_POINT('Origin',(52.8776183915471,825.559694878252,125.51834395973));
#83906=CARTESIAN_POINT('Origin',(52.8776183915471,827.175936191914,121.458286566849));
#83907=CARTESIAN_POINT('Origin',(52.8776183915471,825.559694878252,125.51834395973));
#83908=CARTESIAN_POINT('Origin',(52.8776183915471,827.175936191914,121.458286566849));
#83909=CARTESIAN_POINT('Origin',(52.8776183915471,825.559694878252,125.51834395973));
#83910=CARTESIAN_POINT('Origin',(52.8776183915471,827.175936191914,121.458286566849));
#83911=CARTESIAN_POINT('Origin',(52.8776183915471,825.559694878252,125.51834395973));
#83912=CARTESIAN_POINT('Origin',(52.8776183915471,827.175936191914,121.458286566849));
#83913=CARTESIAN_POINT('Origin',(52.8776183915471,825.559694878252,125.51834395973));
#83914=CARTESIAN_POINT('Origin',(52.8776183915471,827.175936191914,121.458286566849));
#83915=CARTESIAN_POINT('Origin',(52.8776183915471,825.559694878252,125.51834395973));
#83916=CARTESIAN_POINT('Origin',(52.8776183915471,827.175936191914,121.458286566849));
#83917=CARTESIAN_POINT('Origin',(52.8776183915471,825.559694878252,125.51834395973));
#83918=CARTESIAN_POINT('Origin',(52.8776183915471,827.175936191914,121.458286566849));
#83919=CARTESIAN_POINT('Origin',(52.8776183915471,825.559694878252,125.51834395973));
#83920=CARTESIAN_POINT('Origin',(52.8776183915471,827.175936191914,121.458286566849));
#83921=CARTESIAN_POINT('Origin',(52.8776183915471,825.559694878252,125.51834395973));
#83922=CARTESIAN_POINT('Origin',(52.8776183915471,827.175936191914,121.458286566849));
#83923=CARTESIAN_POINT('Origin',(52.8776183915471,825.559694878252,125.51834395973));
#83924=CARTESIAN_POINT('Origin',(52.8776183915471,827.175936191914,121.458286566849));
#83925=CARTESIAN_POINT('Origin',(52.8776183915471,825.559694878252,125.51834395973));
#83926=CARTESIAN_POINT('Origin',(52.8776183915471,827.175936191914,121.458286566849));
#83927=CARTESIAN_POINT('Origin',(52.8776183915471,825.559694878252,125.51834395973));
#83928=CARTESIAN_POINT('Origin',(52.8776183915471,827.175936191914,121.458286566849));
#83929=CARTESIAN_POINT('Origin',(52.8776183915471,825.559694878252,125.51834395973));
#83930=CARTESIAN_POINT('Origin',(52.8776183915471,827.175936191914,121.458286566849));
#83931=CARTESIAN_POINT('Origin',(52.8776183915471,825.559694878252,125.51834395973));
#83932=CARTESIAN_POINT('Origin',(52.8776183915471,827.175936191914,121.458286566849));
#83933=CARTESIAN_POINT('Origin',(52.8776183915471,825.559694878252,125.51834395973));
#83934=CARTESIAN_POINT('Origin',(52.8776183915471,827.175936191914,121.458286566849));
#83935=CARTESIAN_POINT('Origin',(52.8776183915471,825.559694878252,125.51834395973));
#83936=CARTESIAN_POINT('Origin',(52.8776183915471,827.175936191914,121.458286566849));
#83937=CARTESIAN_POINT('Origin',(52.8776183915471,825.559694878252,125.51834395973));
#83938=CARTESIAN_POINT('Origin',(52.8776183915471,827.175936191914,121.458286566849));
#83939=CARTESIAN_POINT('Origin',(52.8776183915471,825.559694878252,125.51834395973));
#83940=CARTESIAN_POINT('Origin',(52.8776183915471,827.175936191914,121.458286566849));
#83941=CARTESIAN_POINT('Origin',(52.8776183915471,825.559694878252,125.51834395973));
#83942=CARTESIAN_POINT('Origin',(52.8776183915471,827.175936191914,121.458286566849));
#83943=CARTESIAN_POINT('Origin',(52.8776183915471,825.559694878252,125.51834395973));
#83944=CARTESIAN_POINT('Origin',(52.8776183915471,827.175936191914,121.458286566849));
#83945=CARTESIAN_POINT('Origin',(52.8776183915471,825.559694878252,125.51834395973));
#83946=CARTESIAN_POINT('Origin',(52.8776183915471,827.175936191914,121.458286566849));
#83947=CARTESIAN_POINT('Origin',(52.8776183915471,825.559694878252,125.51834395973));
#83948=CARTESIAN_POINT('Origin',(52.8776183915471,827.175936191914,121.458286566849));
#83949=CARTESIAN_POINT('Origin',(52.8776183915471,825.559694878252,125.51834395973));
#83950=CARTESIAN_POINT('Origin',(52.8776183915471,827.175936191914,121.458286566849));
#83951=CARTESIAN_POINT('Origin',(52.8776183915471,825.559694878252,125.51834395973));
#83952=CARTESIAN_POINT('Origin',(52.8776183915471,827.175936191914,121.458286566849));
#83953=CARTESIAN_POINT('Origin',(52.8776183915471,825.559694878252,125.51834395973));
#83954=CARTESIAN_POINT('Origin',(52.8776183915471,827.175936191914,121.458286566849));
#83955=CARTESIAN_POINT('Origin',(52.8776183915471,825.559694878252,125.51834395973));
#83956=CARTESIAN_POINT('Origin',(52.8776183915471,827.175936191914,121.458286566849));
#83957=CARTESIAN_POINT('Origin',(52.8776183915471,825.559694878252,125.51834395973));
#83958=CARTESIAN_POINT('Origin',(52.8776183915471,827.175936191914,121.458286566849));
#83959=CARTESIAN_POINT('Origin',(52.8776183915471,825.559694878252,125.51834395973));
#83960=CARTESIAN_POINT('Origin',(52.8776183915471,827.175936191914,121.458286566849));
#83961=CARTESIAN_POINT('Origin',(52.8776183915471,825.559694878252,125.51834395973));
#83962=CARTESIAN_POINT('Origin',(52.8776183915471,827.175936191914,121.458286566849));
#83963=CARTESIAN_POINT('Origin',(52.8776183915471,825.559694878252,125.51834395973));
#83964=CARTESIAN_POINT('Origin',(52.8776183915471,827.175936191914,121.458286566849));
#83965=CARTESIAN_POINT('Origin',(52.8776183915471,825.559694878252,125.51834395973));
#83966=CARTESIAN_POINT('Origin',(52.8776183915471,827.175936191914,121.458286566849));
#83967=CARTESIAN_POINT('Origin',(52.8776183915471,825.559694878252,125.51834395973));
#83968=CARTESIAN_POINT('Origin',(52.8776183915471,827.175936191914,121.458286566849));
#83969=CARTESIAN_POINT('Origin',(52.8776183915471,825.559694878252,125.51834395973));
#83970=CARTESIAN_POINT('Origin',(52.8776183915471,827.175936191914,121.458286566849));
#83971=CARTESIAN_POINT('Origin',(52.8776183915471,825.559694878252,125.51834395973));
#83972=CARTESIAN_POINT('Origin',(52.8776183915471,827.175936191914,121.458286566849));
#83973=CARTESIAN_POINT('Origin',(52.8776183915471,825.559694878252,125.51834395973));
#83974=CARTESIAN_POINT('Origin',(52.8776183915471,827.175936191914,121.458286566849));
#83975=CARTESIAN_POINT('Origin',(52.8776183915471,825.559694878252,125.51834395973));
#83976=CARTESIAN_POINT('Origin',(52.8776183915471,827.175936191914,121.458286566849));
#83977=CARTESIAN_POINT('Origin',(52.8776183915471,825.559694878252,125.51834395973));
#83978=CARTESIAN_POINT('Origin',(52.8776183915471,827.175936191914,121.458286566849));
#83979=CARTESIAN_POINT('Origin',(52.8776183915471,825.559694878252,125.51834395973));
#83980=CARTESIAN_POINT('Origin',(52.8776183915471,827.175936191914,121.458286566849));
#83981=CARTESIAN_POINT('Origin',(52.8776183915471,825.559694878252,125.51834395973));
#83982=CARTESIAN_POINT('Origin',(52.8776183915471,827.175936191914,121.458286566849));
#83983=CARTESIAN_POINT('Origin',(52.8776183915471,825.559694878252,125.51834395973));
#83984=CARTESIAN_POINT('Origin',(52.8776183915471,827.175936191914,121.458286566849));
#83985=CARTESIAN_POINT('Origin',(52.8776183915471,825.559694878252,125.51834395973));
#83986=CARTESIAN_POINT('Origin',(52.8776183915471,827.175936191914,121.458286566849));
#83987=CARTESIAN_POINT('Origin',(52.8776183915471,825.559694878252,125.51834395973));
#83988=CARTESIAN_POINT('Origin',(52.8776183915471,827.175936191914,121.458286566849));
#83989=CARTESIAN_POINT('Origin',(52.8776183915471,825.559694878252,125.51834395973));
#83990=CARTESIAN_POINT('Origin',(52.8776183915471,827.175936191914,121.458286566849));
#83991=CARTESIAN_POINT('Origin',(52.8776183915471,825.559694878252,125.51834395973));
#83992=CARTESIAN_POINT('Origin',(52.8776183915471,827.175936191914,121.458286566849));
#83993=CARTESIAN_POINT('Origin',(52.8776183915471,825.559694878252,125.51834395973));
#83994=CARTESIAN_POINT('Origin',(52.8776183915471,827.175936191914,121.458286566849));
#83995=CARTESIAN_POINT('Origin',(52.8776183915471,825.559694878252,125.51834395973));
#83996=CARTESIAN_POINT('Origin',(52.8776183915471,827.175936191914,121.458286566849));
#83997=CARTESIAN_POINT('Origin',(52.8776183915471,825.559694878252,125.51834395973));
#83998=CARTESIAN_POINT('Origin',(52.8776183915471,827.175936191914,121.458286566849));
#83999=CARTESIAN_POINT('Origin',(52.8776183915471,825.559694878252,125.51834395973));
#84000=CARTESIAN_POINT('Origin',(52.8776183915471,827.175936191914,121.458286566849));
#84001=CARTESIAN_POINT('Origin',(52.8776183915471,825.559694878252,125.51834395973));
#84002=CARTESIAN_POINT('Origin',(52.8776183915471,827.175936191914,121.458286566849));
#84003=CARTESIAN_POINT('Origin',(52.8776183915471,825.559694878252,125.51834395973));
#84004=CARTESIAN_POINT('Origin',(52.8776183915471,827.175936191914,121.458286566849));
#84005=CARTESIAN_POINT('Origin',(52.8776183915471,825.559694878252,125.51834395973));
#84006=CARTESIAN_POINT('Origin',(52.8776183915471,827.175936191914,121.458286566849));
#84007=CARTESIAN_POINT('Origin',(52.8776183915471,825.559694878252,125.51834395973));
#84008=CARTESIAN_POINT('Origin',(52.8776183915471,827.175936191914,121.458286566849));
#84009=CARTESIAN_POINT('Origin',(52.8776183915471,825.559694878252,125.51834395973));
#84010=CARTESIAN_POINT('Origin',(52.8776183915471,827.175936191914,121.458286566849));
#84011=CARTESIAN_POINT('Origin',(52.8776183915471,825.559694878252,125.51834395973));
#84012=CARTESIAN_POINT('Origin',(52.8776183915471,827.175936191914,121.458286566849));
#84013=CARTESIAN_POINT('Origin',(52.8776183915471,825.559694878252,125.51834395973));
#84014=CARTESIAN_POINT('Origin',(52.8776183915471,827.175936191914,121.458286566849));
#84015=CARTESIAN_POINT('Origin',(52.8776183915471,825.559694878252,125.51834395973));
#84016=CARTESIAN_POINT('Origin',(52.8776183915471,827.175936191914,121.458286566849));
#84017=CARTESIAN_POINT('Origin',(52.8776183915471,825.559694878252,125.51834395973));
#84018=CARTESIAN_POINT('Origin',(52.8776183915471,827.175936191914,121.458286566849));
#84019=CARTESIAN_POINT('Origin',(52.8776183915471,825.559694878252,125.51834395973));
#84020=CARTESIAN_POINT('Origin',(52.8776183915471,827.175936191914,121.458286566849));
#84021=CARTESIAN_POINT('Origin',(52.8776183915471,825.559694878252,125.51834395973));
#84022=CARTESIAN_POINT('Origin',(52.8776183915471,827.175936191914,121.458286566849));
#84023=CARTESIAN_POINT('Origin',(52.8776183915471,825.559694878252,125.51834395973));
#84024=CARTESIAN_POINT('Origin',(52.8776183915471,827.175936191914,121.458286566849));
#84025=CARTESIAN_POINT('Origin',(52.8776183915471,825.559694878252,125.51834395973));
#84026=CARTESIAN_POINT('Origin',(52.8776183915471,827.175936191914,121.458286566849));
#84027=CARTESIAN_POINT('Origin',(52.8776183915471,825.559694878252,125.51834395973));
#84028=CARTESIAN_POINT('Origin',(52.8776183915471,827.175936191914,121.458286566849));
#84029=CARTESIAN_POINT('Origin',(52.8776183915471,825.559694878252,125.51834395973));
#84030=CARTESIAN_POINT('Origin',(52.8776183915471,827.175936191914,121.458286566849));
#84031=CARTESIAN_POINT('Origin',(52.8776183915471,825.559694878252,125.51834395973));
#84032=CARTESIAN_POINT('Origin',(52.8776183915471,827.175936191914,121.458286566849));
#84033=CARTESIAN_POINT('Origin',(52.8776183915471,825.559694878252,125.51834395973));
#84034=CARTESIAN_POINT('Origin',(52.8776183915471,827.175936191914,121.458286566849));
#84035=CARTESIAN_POINT('Origin',(52.8776183915471,825.559694878252,125.51834395973));
#84036=CARTESIAN_POINT('Origin',(52.8776183915471,827.175936191914,121.458286566849));
#84037=CARTESIAN_POINT('Origin',(52.8776183915471,825.559694878252,125.51834395973));
#84038=CARTESIAN_POINT('Origin',(52.8776183915471,827.175936191914,121.458286566849));
#84039=CARTESIAN_POINT('Origin',(52.8776183915471,825.559694878252,125.51834395973));
#84040=CARTESIAN_POINT('Origin',(52.8776183915471,827.175936191914,121.458286566849));
#84041=CARTESIAN_POINT('Origin',(52.8776183915471,825.559694878252,125.51834395973));
#84042=CARTESIAN_POINT('Origin',(52.8776183915471,827.175936191914,121.458286566849));
#84043=CARTESIAN_POINT('Origin',(52.8776183915471,825.559694878252,125.51834395973));
#84044=CARTESIAN_POINT('Origin',(52.8776183915471,827.175936191914,121.458286566849));
#84045=CARTESIAN_POINT('Origin',(52.8776183915471,825.559694878252,125.51834395973));
#84046=CARTESIAN_POINT('Origin',(52.8776183915471,827.175936191914,121.458286566849));
#84047=CARTESIAN_POINT('Origin',(52.8776183915471,825.559694878252,125.51834395973));
#84048=CARTESIAN_POINT('Origin',(52.8776183915471,827.175936191914,121.458286566849));
#84049=CARTESIAN_POINT('Origin',(52.8776183915471,825.559694878252,125.51834395973));
#84050=CARTESIAN_POINT('Origin',(52.8776183915471,827.175936191914,121.458286566849));
#84051=CARTESIAN_POINT('Origin',(52.8776183915471,825.559694878252,125.51834395973));
#84052=CARTESIAN_POINT('Origin',(52.8776183915471,827.175936191914,121.458286566849));
#84053=CARTESIAN_POINT('Origin',(52.8776183915471,825.559694878252,125.51834395973));
#84054=CARTESIAN_POINT('Origin',(52.8776183915471,827.175936191914,121.458286566849));
#84055=CARTESIAN_POINT('Origin',(52.8776183915471,825.559694878252,125.51834395973));
#84056=CARTESIAN_POINT('Origin',(52.8776183915471,827.175936191914,121.458286566849));
#84057=CARTESIAN_POINT('Origin',(52.8776183915471,825.559694878252,125.51834395973));
#84058=CARTESIAN_POINT('Origin',(52.8776183915471,827.175936191914,121.458286566849));
#84059=CARTESIAN_POINT('Origin',(52.8776183915471,825.559694878252,125.51834395973));
#84060=CARTESIAN_POINT('Origin',(52.8776183915471,827.175936191914,121.458286566849));
#84061=CARTESIAN_POINT('Origin',(52.8776183915471,825.559694878252,125.51834395973));
#84062=CARTESIAN_POINT('Origin',(52.8776183915471,827.175936191914,121.458286566849));
#84063=CARTESIAN_POINT('Origin',(52.8776183915471,825.559694878252,125.51834395973));
#84064=CARTESIAN_POINT('Origin',(52.8776183915471,827.175936191914,121.458286566849));
#84065=CARTESIAN_POINT('Origin',(52.8776183915471,825.559694878252,125.51834395973));
#84066=CARTESIAN_POINT('Origin',(52.8776183915471,827.175936191914,121.458286566849));
#84067=CARTESIAN_POINT('Origin',(52.8776183915471,825.559694878252,125.51834395973));
#84068=CARTESIAN_POINT('Origin',(52.8776183915471,827.175936191914,121.458286566849));
#84069=CARTESIAN_POINT('Origin',(52.8776183915471,825.559694878252,125.51834395973));
#84070=CARTESIAN_POINT('Origin',(52.8776183915471,827.175936191914,121.458286566849));
#84071=CARTESIAN_POINT('Origin',(52.8776183915471,825.559694878252,125.51834395973));
#84072=CARTESIAN_POINT('Origin',(52.8776183915471,827.175936191914,121.458286566849));
#84073=CARTESIAN_POINT('Origin',(52.8776183915471,825.559694878252,125.51834395973));
#84074=CARTESIAN_POINT('Origin',(52.8776183915471,827.175936191914,121.458286566849));
#84075=CARTESIAN_POINT('Origin',(52.8776183915471,825.559694878252,125.51834395973));
#84076=CARTESIAN_POINT('Origin',(52.8776183915471,827.175936191914,121.458286566849));
#84077=CARTESIAN_POINT('Origin',(52.8776183915471,825.559694878252,125.51834395973));
#84078=CARTESIAN_POINT('Origin',(52.8776183915471,827.175936191914,121.458286566849));
#84079=CARTESIAN_POINT('Origin',(52.8776183915471,825.559694878252,125.51834395973));
#84080=CARTESIAN_POINT('Origin',(52.8776183915471,827.175936191914,121.458286566849));
#84081=CARTESIAN_POINT('Origin',(52.8776183915471,825.559694878252,125.51834395973));
#84082=CARTESIAN_POINT('Origin',(52.8776183915471,827.175936191914,121.458286566849));
#84083=CARTESIAN_POINT('Origin',(52.8776183915471,825.559694878252,125.51834395973));
#84084=CARTESIAN_POINT('Origin',(52.8776183915471,827.175936191914,121.458286566849));
#84085=CARTESIAN_POINT('Origin',(52.8776183915471,825.559694878252,125.51834395973));
#84086=CARTESIAN_POINT('Origin',(52.8776183915471,827.175936191914,121.458286566849));
#84087=CARTESIAN_POINT('Origin',(52.8776183915471,825.559694878252,125.51834395973));
#84088=CARTESIAN_POINT('Origin',(52.8776183915471,827.175936191914,121.458286566849));
#84089=CARTESIAN_POINT('Origin',(52.8776183915471,825.559694878252,125.51834395973));
#84090=CARTESIAN_POINT('Origin',(52.8776183915471,827.175936191914,121.458286566849));
#84091=CARTESIAN_POINT('Origin',(52.8776183915471,825.559694878252,125.51834395973));
#84092=CARTESIAN_POINT('Origin',(52.8776183915471,827.175936191914,121.458286566849));
#84093=CARTESIAN_POINT('Origin',(52.8776183915471,825.559694878252,125.51834395973));
#84094=CARTESIAN_POINT('Origin',(52.8776183915471,827.175936191914,121.458286566849));
#84095=CARTESIAN_POINT('Origin',(52.8776183915471,825.559694878252,125.51834395973));
#84096=CARTESIAN_POINT('Origin',(52.8776183915471,827.175936191914,121.458286566849));
#84097=CARTESIAN_POINT('Origin',(52.8776183915471,825.559694878252,125.51834395973));
#84098=CARTESIAN_POINT('Origin',(52.8776183915471,827.175936191914,121.458286566849));
#84099=CARTESIAN_POINT('Origin',(52.8776183915471,825.559694878252,125.51834395973));
#84100=CARTESIAN_POINT('Origin',(52.8776183915471,827.175936191914,121.458286566849));
#84101=CARTESIAN_POINT('Origin',(52.8776183915471,825.559694878252,125.51834395973));
#84102=CARTESIAN_POINT('Origin',(52.8776183915471,827.175936191914,121.458286566849));
#84103=CARTESIAN_POINT('Origin',(52.8776183915471,825.559694878252,125.51834395973));
#84104=CARTESIAN_POINT('Origin',(52.8776183915471,827.175936191914,121.458286566849));
#84105=CARTESIAN_POINT('Origin',(52.8776183915471,825.559694878252,125.51834395973));
#84106=CARTESIAN_POINT('Origin',(52.8776183915471,827.175936191914,121.458286566849));
#84107=CARTESIAN_POINT('Origin',(52.8776183915471,825.559694878252,125.51834395973));
#84108=CARTESIAN_POINT('Origin',(52.8776183915471,827.175936191914,121.458286566849));
#84109=CARTESIAN_POINT('Origin',(52.8776183915471,825.559694878252,125.51834395973));
#84110=CARTESIAN_POINT('Origin',(52.8776183915471,827.175936191914,121.458286566849));
#84111=CARTESIAN_POINT('Origin',(52.8776183915471,825.559694878252,125.51834395973));
#84112=CARTESIAN_POINT('Origin',(52.8776183915471,827.175936191914,121.458286566849));
#84113=CARTESIAN_POINT('Origin',(52.8776183915471,825.559694878252,125.51834395973));
#84114=CARTESIAN_POINT('Origin',(52.8776183915471,827.175936191914,121.458286566849));
#84115=CARTESIAN_POINT('Origin',(52.8776183915471,825.559694878252,125.51834395973));
#84116=CARTESIAN_POINT('Origin',(52.8776183915471,827.175936191914,121.458286566849));
#84117=CARTESIAN_POINT('Origin',(52.8776183915471,825.559694878252,125.51834395973));
#84118=CARTESIAN_POINT('Origin',(52.8776183915471,827.175936191914,121.458286566849));
#84119=CARTESIAN_POINT('Origin',(52.8776183915471,825.559694878252,125.51834395973));
#84120=CARTESIAN_POINT('Origin',(52.8776183915471,827.175936191914,121.458286566849));
#84121=CARTESIAN_POINT('Origin',(52.8776183915471,825.559694878252,125.51834395973));
#84122=CARTESIAN_POINT('Origin',(52.8776183915471,827.175936191914,121.458286566849));
#84123=CARTESIAN_POINT('Origin',(52.8776183915471,825.559694878252,125.51834395973));
#84124=CARTESIAN_POINT('Origin',(52.8776183915471,827.175936191914,121.458286566849));
#84125=CARTESIAN_POINT('Origin',(52.8776183915471,825.559694878252,125.51834395973));
#84126=CARTESIAN_POINT('Origin',(52.8776183915471,827.175936191914,121.458286566849));
#84127=CARTESIAN_POINT('Origin',(52.8776183915471,825.559694878252,125.51834395973));
#84128=CARTESIAN_POINT('Origin',(52.8776183915471,827.175936191914,121.458286566849));
#84129=CARTESIAN_POINT('Origin',(52.8776183915471,825.559694878252,125.51834395973));
#84130=CARTESIAN_POINT('Origin',(52.8776183915471,827.175936191914,121.458286566849));
#84131=CARTESIAN_POINT('Origin',(52.8776183915471,825.559694878252,125.51834395973));
#84132=CARTESIAN_POINT('Origin',(52.8776183915471,827.175936191914,121.458286566849));
#84133=CARTESIAN_POINT('Origin',(52.8776183915471,825.559694878252,125.51834395973));
#84134=CARTESIAN_POINT('Origin',(52.8776183915471,827.175936191914,121.458286566849));
#84135=CARTESIAN_POINT('Origin',(52.8776183915471,825.559694878252,125.51834395973));
#84136=CARTESIAN_POINT('Origin',(52.8776183915471,827.175936191914,121.458286566849));
#84137=CARTESIAN_POINT('Origin',(52.8776183915471,825.559694878252,125.51834395973));
#84138=CARTESIAN_POINT('Origin',(52.8776183915471,827.175936191914,121.458286566849));
#84139=CARTESIAN_POINT('Origin',(52.8776183915471,825.559694878252,125.51834395973));
#84140=CARTESIAN_POINT('Origin',(52.8776183915471,827.175936191914,121.458286566849));
#84141=CARTESIAN_POINT('Origin',(52.8776183915471,825.559694878252,125.51834395973));
#84142=CARTESIAN_POINT('Origin',(52.8776183915471,827.175936191914,121.458286566849));
#84143=CARTESIAN_POINT('Origin',(52.8776183915471,825.559694878252,125.51834395973));
#84144=CARTESIAN_POINT('Origin',(52.8776183915471,827.175936191914,121.458286566849));
#84145=CARTESIAN_POINT('Origin',(52.8776183915471,825.559694878252,125.51834395973));
#84146=CARTESIAN_POINT('Origin',(52.8776183915471,827.175936191914,121.458286566849));
#84147=CARTESIAN_POINT('Origin',(52.8776183915471,825.559694878252,125.51834395973));
#84148=CARTESIAN_POINT('Origin',(52.8776183915471,827.175936191914,121.458286566849));
#84149=CARTESIAN_POINT('Origin',(52.8776183915471,825.559694878252,125.51834395973));
#84150=CARTESIAN_POINT('Origin',(52.8776183915471,827.175936191914,121.458286566849));
#84151=CARTESIAN_POINT('Origin',(52.8776183915471,825.559694878252,125.51834395973));
#84152=CARTESIAN_POINT('Origin',(52.8776183915471,827.175936191914,121.458286566849));
#84153=CARTESIAN_POINT('Origin',(52.8776183915471,825.559694878252,125.51834395973));
#84154=CARTESIAN_POINT('Origin',(52.8776183915471,827.175936191914,121.458286566849));
#84155=CARTESIAN_POINT('Origin',(52.8776183915471,825.559694878252,125.51834395973));
#84156=CARTESIAN_POINT('Origin',(52.8776183915471,827.175936191914,121.458286566849));
#84157=CARTESIAN_POINT('Origin',(52.8776183915471,825.559694878252,125.51834395973));
#84158=CARTESIAN_POINT('Origin',(52.8776183915471,827.175936191914,121.458286566849));
#84159=CARTESIAN_POINT('Origin',(52.8776183915471,825.559694878252,125.51834395973));
#84160=CARTESIAN_POINT('Origin',(52.8776183915471,827.175936191914,121.458286566849));
#84161=CARTESIAN_POINT('Origin',(52.8776183915471,825.559694878252,125.51834395973));
#84162=CARTESIAN_POINT('Origin',(52.8776183915471,827.175936191914,121.458286566849));
#84163=CARTESIAN_POINT('Origin',(52.8776183915471,825.559694878252,125.51834395973));
#84164=CARTESIAN_POINT('Origin',(52.8776183915471,827.175936191914,121.458286566849));
#84165=CARTESIAN_POINT('Origin',(52.8776183915471,825.559694878252,125.51834395973));
#84166=CARTESIAN_POINT('Origin',(52.8776183915471,827.175936191914,121.458286566849));
#84167=CARTESIAN_POINT('Origin',(52.8776183915471,825.559694878252,125.51834395973));
#84168=CARTESIAN_POINT('Origin',(52.8776183915471,827.175936191914,121.458286566849));
#84169=CARTESIAN_POINT('Origin',(52.8776183915471,825.559694878252,125.51834395973));
#84170=CARTESIAN_POINT('Origin',(52.8776183915471,827.175936191914,121.458286566849));
#84171=CARTESIAN_POINT('Origin',(52.8776183915471,825.559694878252,125.51834395973));
#84172=CARTESIAN_POINT('Origin',(52.8776183915471,827.175936191914,121.458286566849));
#84173=CARTESIAN_POINT('Origin',(52.8776183915471,825.559694878252,125.51834395973));
#84174=CARTESIAN_POINT('Origin',(52.8776183915471,827.175936191914,121.458286566849));
#84175=CARTESIAN_POINT('Origin',(52.8776183915471,825.559694878252,125.51834395973));
#84176=CARTESIAN_POINT('Origin',(52.8776183915471,827.175936191914,121.458286566849));
#84177=CARTESIAN_POINT('Origin',(52.8776183915471,825.559694878252,125.51834395973));
#84178=CARTESIAN_POINT('Origin',(52.8776183915471,827.175936191914,121.458286566849));
#84179=CARTESIAN_POINT('Origin',(52.8776183915471,825.559694878252,125.51834395973));
#84180=CARTESIAN_POINT('Origin',(52.8776183915471,827.175936191914,121.458286566849));
#84181=CARTESIAN_POINT('Origin',(52.8776183915471,825.559694878252,125.51834395973));
#84182=CARTESIAN_POINT('Origin',(52.8776183915471,827.175936191914,121.458286566849));
#84183=CARTESIAN_POINT('Origin',(52.8776183915471,825.559694878252,125.51834395973));
#84184=CARTESIAN_POINT('Origin',(52.8776183915471,827.175936191914,121.458286566849));
#84185=CARTESIAN_POINT('Origin',(52.8776183915471,825.559694878252,125.51834395973));
#84186=CARTESIAN_POINT('Origin',(52.8776183915471,827.175936191914,121.458286566849));
#84187=CARTESIAN_POINT('Origin',(52.8776183915471,825.559694878252,125.51834395973));
#84188=CARTESIAN_POINT('Origin',(52.8776183915471,827.175936191914,121.458286566849));
#84189=CARTESIAN_POINT('Origin',(52.8776183915471,825.559694878252,125.51834395973));
#84190=CARTESIAN_POINT('Origin',(52.8776183915471,827.175936191914,121.458286566849));
#84191=CARTESIAN_POINT('Origin',(52.8776183915471,825.559694878252,125.51834395973));
#84192=CARTESIAN_POINT('Origin',(52.8776183915471,827.175936191914,121.458286566849));
#84193=CARTESIAN_POINT('Origin',(52.8776183915471,825.559694878252,125.51834395973));
#84194=CARTESIAN_POINT('Origin',(52.8776183915471,827.175936191914,121.458286566849));
#84195=CARTESIAN_POINT('Origin',(52.8776183915471,825.559694878252,125.51834395973));
#84196=CARTESIAN_POINT('Origin',(52.8776183915471,827.175936191914,121.458286566849));
#84197=CARTESIAN_POINT('Origin',(52.8776183915471,825.559694878252,125.51834395973));
#84198=CARTESIAN_POINT('Origin',(52.8776183915471,827.175936191914,121.458286566849));
#84199=CARTESIAN_POINT('Origin',(52.8776183915471,825.559694878252,125.51834395973));
#84200=CARTESIAN_POINT('Origin',(52.8776183915471,827.175936191914,121.458286566849));
#84201=CARTESIAN_POINT('Origin',(52.8776183915471,825.559694878252,125.51834395973));
#84202=CARTESIAN_POINT('Origin',(52.8776183915471,827.175936191914,121.458286566849));
#84203=CARTESIAN_POINT('Origin',(52.8776183915471,825.559694878252,125.51834395973));
#84204=CARTESIAN_POINT('Origin',(52.8776183915471,827.175936191914,121.458286566849));
#84205=CARTESIAN_POINT('Origin',(52.8776183915471,825.559694878252,125.51834395973));
#84206=CARTESIAN_POINT('Origin',(52.8776183915471,827.175936191914,121.458286566849));
#84207=CARTESIAN_POINT('Origin',(52.8776183915471,825.559694878252,125.51834395973));
#84208=CARTESIAN_POINT('Origin',(52.8776183915471,827.175936191914,121.458286566849));
#84209=CARTESIAN_POINT('Origin',(52.8776183915471,825.559694878252,125.51834395973));
#84210=CARTESIAN_POINT('Origin',(52.8776183915471,827.175936191914,121.458286566849));
#84211=CARTESIAN_POINT('Origin',(52.8776183915471,825.559694878252,125.51834395973));
#84212=CARTESIAN_POINT('Origin',(52.8776183915471,827.175936191914,121.458286566849));
#84213=CARTESIAN_POINT('Ctrl Pts',(3.84082565589434,825.316688336501,125.465893547845));
#84214=CARTESIAN_POINT('Ctrl Pts',(3.8442236582366,824.679598781654,125.240724542698));
#84215=CARTESIAN_POINT('Ctrl Pts',(3.86158552590586,824.042711504904,125.015627029475));
#84216=CARTESIAN_POINT('Ctrl Pts',(3.89290384275382,823.406298553624,124.790697158922));
#84217=CARTESIAN_POINT('Ctrl Pts',(2.81394584476287,825.297442889065,125.504849768887));
#84218=CARTESIAN_POINT('Ctrl Pts',(2.81741500469536,824.647012037505,125.274965498068));
#84219=CARTESIAN_POINT('Ctrl Pts',(2.83514044735389,823.996787699948,125.045154216285));
#84220=CARTESIAN_POINT('Ctrl Pts',(2.86711460128858,823.347047620715,124.815514087779));
#84221=CARTESIAN_POINT('Ctrl Pts',(1.76405870526505,825.258413667814,125.599434679541));
#84222=CARTESIAN_POINT('Ctrl Pts',(1.76760061707955,824.594342606667,125.364729497126));
#84223=CARTESIAN_POINT('Ctrl Pts',(1.78569778065552,823.930482390338,125.130098834403));
#84224=CARTESIAN_POINT('Ctrl Pts',(1.8183424657619,823.267116587731,124.895642914219));
#84225=CARTESIAN_POINT('Origin',(52.8776183915471,827.175936191914,121.458286566849));
#84226=CARTESIAN_POINT('Ctrl Pts',(0.000492700221437848,819.600382093278,
123.878802654728));
#84227=CARTESIAN_POINT('Ctrl Pts',(0.0733770646291771,819.010988593857,
123.670491049405));
#84228=CARTESIAN_POINT('Ctrl Pts',(0.157334275777137,818.422906232969,123.462642844803));
#84229=CARTESIAN_POINT('Ctrl Pts',(0.252337935209915,817.836319919877,123.255323394113));
#84230=CARTESIAN_POINT('Ctrl Pts',(-0.948554213994308,819.448222594439,
123.977266388053));
#84231=CARTESIAN_POINT('Ctrl Pts',(-0.87436170962564,818.848250568395,123.765215973488));
#84232=CARTESIAN_POINT('Ctrl Pts',(-0.788897621333276,818.249613213403,
123.553637276833));
#84233=CARTESIAN_POINT('Ctrl Pts',(-0.692188821376213,817.652498757506,
123.342596824246));
#84234=CARTESIAN_POINT('Ctrl Pts',(-1.91572574332748,819.278466654302,124.11917574241));
#84235=CARTESIAN_POINT('Ctrl Pts',(-1.84020011653079,818.667714076086,123.903315115938));
#84236=CARTESIAN_POINT('Ctrl Pts',(-1.75320037320342,818.058320150858,123.687934683404));
#84237=CARTESIAN_POINT('Ctrl Pts',(-1.65475386845653,817.450476488823,123.473102166337));
#84238=CARTESIAN_POINT('Origin',(52.8776183915471,827.175936191914,121.458286566849));
#84239=CARTESIAN_POINT('Ctrl Pts',(2.46855401679697,809.370840123866,120.258308875262));
#84240=CARTESIAN_POINT('Ctrl Pts',(2.67073628760838,808.806131617377,120.058721781679));
#84241=CARTESIAN_POINT('Ctrl Pts',(2.88355991138435,808.244909852193,119.86036702045));
#84242=CARTESIAN_POINT('Ctrl Pts',(3.10695729599134,807.687353070633,119.663307588441));
#84243=CARTESIAN_POINT('Ctrl Pts',(1.56447923623846,809.035572744419,120.291078774796));
#84244=CARTESIAN_POINT('Ctrl Pts',(1.77028759879318,808.460736322933,120.087912133367));
#84245=CARTESIAN_POINT('Ctrl Pts',(1.98692816448921,807.889449176641,119.885999925883));
#84246=CARTESIAN_POINT('Ctrl Pts',(2.21433212894391,807.321892744598,119.685406279047));
#84247=CARTESIAN_POINT('Ctrl Pts',(0.643150928951218,808.679241949644,120.36596729256));
#84248=CARTESIAN_POINT('Ctrl Pts',(0.852654584240296,808.094084330198,120.159152790545));
#84249=CARTESIAN_POINT('Ctrl Pts',(1.07318493506676,807.512539713244,119.95361524586));
#84250=CARTESIAN_POINT('Ctrl Pts',(1.30467194166409,806.934792795578,119.749419936601));
#84251=CARTESIAN_POINT('Origin',(52.8776183915471,827.175936191914,121.458286566849));
#84252=CARTESIAN_POINT('Ctrl Pts',(5.00031415269847,815.719484412942,122.072244000229));
#84253=CARTESIAN_POINT('Ctrl Pts',(5.14465313820655,815.094556777728,121.85137342899));
#84254=CARTESIAN_POINT('Ctrl Pts',(5.30272291144696,814.472589472092,121.631549138388));
#84255=CARTESIAN_POINT('Ctrl Pts',(5.47445532125263,813.853850654815,121.412865904811));
#84256=CARTESIAN_POINT('Ctrl Pts',(3.99763435701107,815.499604445748,122.039117284757));
#84257=CARTESIAN_POINT('Ctrl Pts',(4.14499618991626,814.86158914147,121.813621088437));
#84258=CARTESIAN_POINT('Ctrl Pts',(4.30637637025783,814.226596164049,121.589193084692));
#84259=CARTESIAN_POINT('Ctrl Pts',(4.48170531959961,813.594899288235,121.365930034782));
#84260=CARTESIAN_POINT('Ctrl Pts',(2.9724864061455,815.255447616079,122.059996186536));
#84261=CARTESIAN_POINT('Ctrl Pts',(3.12293882273279,814.604051372859,121.82977071364));
#84262=CARTESIAN_POINT('Ctrl Pts',(3.28770359012886,813.95574084302,121.600635836259));
#84263=CARTESIAN_POINT('Ctrl Pts',(3.466709670646,813.31079554312,121.372690345005));
#84264=CARTESIAN_POINT('Origin',(52.8776183915471,827.175936191914,121.458286566849));
#84265=CARTESIAN_POINT('Ctrl Pts',(7.14679452608843,799.846737018268,116.886459225876));
#84266=CARTESIAN_POINT('Ctrl Pts',(7.46834327891507,799.335514201564,116.705775784797));
#84267=CARTESIAN_POINT('Ctrl Pts',(7.79948339953489,798.829763525227,116.527026383277));
#84268=CARTESIAN_POINT('Ctrl Pts',(8.14011016077353,798.329644939187,116.350267553035));
#84269=CARTESIAN_POINT('Ctrl Pts',(6.32653782350611,799.340882241166,116.857967319315));
#84270=CARTESIAN_POINT('Ctrl Pts',(6.65385407618119,798.820489811793,116.674043026856));
#84271=CARTESIAN_POINT('Ctrl Pts',(6.99093373343021,798.305667674524,116.492087464103));
#84272=CARTESIAN_POINT('Ctrl Pts',(7.3376701896266,797.796578648251,116.31215817676));
#84273=CARTESIAN_POINT('Ctrl Pts',(5.49062488819893,798.810708086188,116.870422046865));
#84274=CARTESIAN_POINT('Ctrl Pts',(5.82381872494313,798.280971023826,116.683195044925));
#84275=CARTESIAN_POINT('Ctrl Pts',(6.16695128670662,797.756904278727,116.497972124965));
#84276=CARTESIAN_POINT('Ctrl Pts',(6.5199140535566,797.238673593504,116.314811866034));
#84277=CARTESIAN_POINT('Origin',(52.8776183915471,827.175936191914,121.458286566849));
#84278=CARTESIAN_POINT('Ctrl Pts',(8.25143832150338,806.549530642949,118.829815173907));
#84279=CARTESIAN_POINT('Ctrl Pts',(8.53030342011268,805.96729913711,118.624034859448));
#84280=CARTESIAN_POINT('Ctrl Pts',(8.8219243969931,805.390649719661,118.420227443901));
#84281=CARTESIAN_POINT('Ctrl Pts',(9.12617563318484,804.819830788713,118.218480719563));
#84282=CARTESIAN_POINT('Ctrl Pts',(7.31405734151393,806.13669890325,118.72757413102));
#84283=CARTESIAN_POINT('Ctrl Pts',(7.59878005193337,805.542237519374,118.517471363854));
#84284=CARTESIAN_POINT('Ctrl Pts',(7.89652658015303,804.953475476663,118.309382936699));
#84285=CARTESIAN_POINT('Ctrl Pts',(8.20716866856419,804.370666390877,118.103398485944));
#84286=CARTESIAN_POINT('Ctrl Pts',(6.35560773678644,805.695128252369,118.678095158437));
#84287=CARTESIAN_POINT('Ctrl Pts',(6.64631971501044,805.088162111066,118.463572786888));
#84288=CARTESIAN_POINT('Ctrl Pts',(6.95032947278689,804.487015199085,118.25110712788));
#84289=CARTESIAN_POINT('Ctrl Pts',(7.26750605455168,803.891946467103,118.040789703343));
#84290=CARTESIAN_POINT('Origin',(52.8776183915471,827.175936191914,121.458286566849));
#84291=CARTESIAN_POINT('Ctrl Pts',(13.820198976375,791.445139376217,113.912623895849));
#84292=CARTESIAN_POINT('Ctrl Pts',(14.2485767358446,791.00733451784,113.757888845401));
#84293=CARTESIAN_POINT('Ctrl Pts',(14.6851662425343,790.576801200474,113.605723803585));
#84294=CARTESIAN_POINT('Ctrl Pts',(15.1298286699926,790.153676324828,113.456177155743));
#84295=CARTESIAN_POINT('Ctrl Pts',(13.1175861709652,790.78687998019,113.829937150564));
#84296=CARTESIAN_POINT('Ctrl Pts',(13.5536701154277,790.341199350592,113.672418536083));
#84297=CARTESIAN_POINT('Ctrl Pts',(13.9981135300995,789.902921071413,113.517516162705));
#84298=CARTESIAN_POINT('Ctrl Pts',(14.4507750911487,789.472184506096,113.365279286186));
#84299=CARTESIAN_POINT('Ctrl Pts',(12.4015228153398,790.101272006005,113.787392724708));
#84300=CARTESIAN_POINT('Ctrl Pts',(12.8454604690467,789.647564834443,113.627037258712));
#84301=CARTESIAN_POINT('Ctrl Pts',(13.2979081439044,789.201393326868,113.469345151344));
#84302=CARTESIAN_POINT('Ctrl Pts',(13.7587219708917,788.762899356612,113.314366545442));
#84303=CARTESIAN_POINT('Origin',(52.8776183915471,827.175936191914,121.458286566849));
#84304=CARTESIAN_POINT('Ctrl Pts',(13.4452714124558,798.220327738148,115.884933356194));
#84305=CARTESIAN_POINT('Ctrl Pts',(13.8473572187005,797.70461362743,115.702662539843));
#84306=CARTESIAN_POINT('Ctrl Pts',(14.2607352601467,797.196897982581,115.523218651965));
#84307=CARTESIAN_POINT('Ctrl Pts',(14.6852266063437,796.697400568031,115.346679364745));
#84308=CARTESIAN_POINT('Ctrl Pts',(12.6187070497033,797.63399734938,115.720502517623));
#84309=CARTESIAN_POINT('Ctrl Pts',(13.0292212104253,797.107473055197,115.534411016664));
#84310=CARTESIAN_POINT('Ctrl Pts',(13.4512643094595,796.589114887379,115.35120570107));
#84311=CARTESIAN_POINT('Ctrl Pts',(13.8846536656899,796.079147216966,115.170965871158));
#84312=CARTESIAN_POINT('Ctrl Pts',(11.7736026754359,797.015140000607,115.607204037821));
#84313=CARTESIAN_POINT('Ctrl Pts',(12.1927342403887,796.477563048284,115.417206153499));
#84314=CARTESIAN_POINT('Ctrl Pts',(12.6236367560647,795.948323643482,115.230155040579));
#84315=CARTESIAN_POINT('Ctrl Pts',(13.0661237065545,795.427650867176,115.046131664029));
#84316=CARTESIAN_POINT('Origin',(52.8776183915471,827.175936191914,121.458286566849));
#84317=CARTESIAN_POINT('Ctrl Pts',(22.1980264899163,784.534083757446,111.466793902928));
#84318=CARTESIAN_POINT('Ctrl Pts',(22.713880531712,784.189975556137,111.345174421393));
#84319=CARTESIAN_POINT('Ctrl Pts',(23.2361643237017,783.854600088267,111.226641383336));
#84320=CARTESIAN_POINT('Ctrl Pts',(23.7647115850361,783.528064128199,111.111232526427));
#84321=CARTESIAN_POINT('Ctrl Pts',(21.6467475207342,783.752542356409,111.339802088341));
#84322=CARTESIAN_POINT('Ctrl Pts',(22.1718708997924,783.402250904191,111.215997236719));
#84323=CARTESIAN_POINT('Ctrl Pts',(22.7035395646771,783.060849103155,111.095334288614));
#84324=CARTESIAN_POINT('Ctrl Pts',(23.2415842466528,782.728445646282,110.977851659803));
#84325=CARTESIAN_POINT('Ctrl Pts',(21.0849267323589,782.941344425908,111.252006419899));
#84326=CARTESIAN_POINT('Ctrl Pts',(21.6194967013644,782.58475148371,111.125974408502));
#84327=CARTESIAN_POINT('Ctrl Pts',(22.1607297011565,782.237208111092,111.003140821195));
#84328=CARTESIAN_POINT('Ctrl Pts',(22.7084534179776,781.898824956343,110.883544764827));
#84329=CARTESIAN_POINT('Origin',(52.8776183915471,827.175936191914,121.458286566849));
#84330=CARTESIAN_POINT('Ctrl Pts',(20.3722156592907,791.094625888558,113.365198749342));
#84331=CARTESIAN_POINT('Ctrl Pts',(20.8778391407687,790.670597907231,113.215332913395));
#84332=CARTESIAN_POINT('Ctrl Pts',(21.3926859167994,790.256553475804,113.068995601785));
#84333=CARTESIAN_POINT('Ctrl Pts',(21.916534279872,789.852670893462,112.926249831477));
#84334=CARTESIAN_POINT('Ctrl Pts',(19.689809879067,790.358096599145,113.146794345208));
#84335=CARTESIAN_POINT('Ctrl Pts',(20.2060482232254,789.925166739327,112.9937822842));
#84336=CARTESIAN_POINT('Ctrl Pts',(20.7317034921946,789.502430020172,112.844372823996));
#84337=CARTESIAN_POINT('Ctrl Pts',(21.2665493240224,789.090068484008,112.698630304515));
#84338=CARTESIAN_POINT('Ctrl Pts',(18.9920735300533,789.585590955693,112.978457958024));
#84339=CARTESIAN_POINT('Ctrl Pts',(19.5191652048056,789.143559232471,112.82222899052));
#84340=CARTESIAN_POINT('Ctrl Pts',(20.0558717846221,788.71193494923,112.66967836445));
#84341=CARTESIAN_POINT('Ctrl Pts',(20.6019621485449,788.290903975535,112.520871772407));
#84342=CARTESIAN_POINT('Origin',(52.8776183915471,827.175936191914,121.458286566849));
#84343=CARTESIAN_POINT('Ctrl Pts',(31.9219622709691,779.417686408915,109.655646046072));
#84344=CARTESIAN_POINT('Ctrl Pts',(32.5011814287363,779.183130129333,109.572745920458));
#84345=CARTESIAN_POINT('Ctrl Pts',(33.0847382986841,778.958334790098,109.493295641431));
#84346=CARTESIAN_POINT('Ctrl Pts',(33.6724478603244,778.743371664027,109.417320399219));
#84347=CARTESIAN_POINT('Ctrl Pts',(31.5451527574604,778.543748134616,109.495603117894));
#84348=CARTESIAN_POINT('Ctrl Pts',(32.1347870168974,778.304974232972,109.411212341936));
#84349=CARTESIAN_POINT('Ctrl Pts',(32.7288369861309,778.076136785871,109.330333445222));
#84350=CARTESIAN_POINT('Ctrl Pts',(33.3271143177676,777.857308347711,109.252992070931));
#84351=CARTESIAN_POINT('Ctrl Pts',(31.161132595897,777.638356388944,109.374173686482));
#84352=CARTESIAN_POINT('Ctrl Pts',(31.7613812609754,777.395284156583,109.288263735011));
#84353=CARTESIAN_POINT('Ctrl Pts',(32.366125126033,777.162327251614,109.205928882501));
#84354=CARTESIAN_POINT('Ctrl Pts',(32.9751724531075,776.939559534534,109.12719523375));
#84355=CARTESIAN_POINT('Origin',(52.8776183915471,827.175936191914,121.458286566849));
#84356=CARTESIAN_POINT('Ctrl Pts',(28.7148160478869,785.478954218345,111.379630155249));
#84357=CARTESIAN_POINT('Ctrl Pts',(29.3048316403161,785.162691727128,111.267852289844));
#84358=CARTESIAN_POINT('Ctrl Pts',(29.9017032114044,784.858080026341,111.160192207991));
#84359=CARTESIAN_POINT('Ctrl Pts',(30.5051719961012,784.565251175986,111.056696584164));
#84360=CARTESIAN_POINT('Ctrl Pts',(28.2069988999599,784.623787837421,111.118728900438));
#84361=CARTESIAN_POINT('Ctrl Pts',(28.8094145456246,784.30087862063,111.004601857317));
#84362=CARTESIAN_POINT('Ctrl Pts',(29.4188302585139,783.989865052919,110.894679139081));
#84363=CARTESIAN_POINT('Ctrl Pts',(30.0349818352457,783.690881969727,110.789008401135));
#84364=CARTESIAN_POINT('Ctrl Pts',(27.6877606464623,783.729919130396,110.90704547314));
#84365=CARTESIAN_POINT('Ctrl Pts',(28.3028552298343,783.400213699273,110.790516417919));
#84366=CARTESIAN_POINT('Ctrl Pts',(28.9250972096328,783.082654282895,110.678280175279));
#84367=CARTESIAN_POINT('Ctrl Pts',(29.5542168218329,782.777378554559,110.570385403623));
#84368=CARTESIAN_POINT('Origin',(52.8776183915471,827.175936191914,121.458286566849));
#84369=CARTESIAN_POINT('Ctrl Pts',(42.5551319591545,776.317087718572,108.558576546772));
#84370=CARTESIAN_POINT('Ctrl Pts',(43.1748960382436,776.20126800047,108.517641939537));
#84371=CARTESIAN_POINT('Ctrl Pts',(43.796753920824,776.095896381883,108.480400044191));
#84372=CARTESIAN_POINT('Ctrl Pts',(44.4205074850962,776.00100643385,108.446862725874));
#84373=CARTESIAN_POINT('Ctrl Pts',(42.3696630121901,775.388170827814,108.378775171248));
#84374=CARTESIAN_POINT('Ctrl Pts',(43.0005626826765,775.270270122607,108.337105072758));
#84375=CARTESIAN_POINT('Ctrl Pts',(43.6335937770019,775.163005242812,108.29919403484));
#84376=CARTESIAN_POINT('Ctrl Pts',(44.2685546136197,775.066410362653,108.265054135823));
#84377=CARTESIAN_POINT('Ctrl Pts',(42.1806476137204,774.426785367898,108.237145342521));
#84378=CARTESIAN_POINT('Ctrl Pts',(42.8228958052374,774.306763883913,108.194725689052));
#84379=CARTESIAN_POINT('Ctrl Pts',(43.4673137603,774.197569540843,108.156132713528));
#84380=CARTESIAN_POINT('Ctrl Pts',(44.1136961695466,774.099237127634,108.12137871154));
#84381=CARTESIAN_POINT('Origin',(52.8776183915471,827.175936191914,121.458286566849));
#84382=CARTESIAN_POINT('Ctrl Pts',(38.1133381600097,781.620808531784,110.015513754693));
#84383=CARTESIAN_POINT('Ctrl Pts',(38.7603804515547,781.427496535375,109.947190754287));
#84384=CARTESIAN_POINT('Ctrl Pts',(39.4115526444503,781.246932435716,109.883373291929));
#84385=CARTESIAN_POINT('Ctrl Pts',(40.0665722423738,781.079194566457,109.82408905338));
#84386=CARTESIAN_POINT('Ctrl Pts',(37.8031710004168,780.685060281388,109.725715192468));
#84387=CARTESIAN_POINT('Ctrl Pts',(38.4638063196311,780.48768719755,109.655956866354));
#84388=CARTESIAN_POINT('Ctrl Pts',(39.1286583009287,780.303329817553,109.590798730375));
#84389=CARTESIAN_POINT('Ctrl Pts',(39.7974385133204,780.132068120674,109.530269051914));
#84390=CARTESIAN_POINT('Ctrl Pts',(37.486030705108,779.708823383608,109.484436565335));
#84391=CARTESIAN_POINT('Ctrl Pts',(38.160564648583,779.507297911529,109.413210644717));
#84392=CARTESIAN_POINT('Ctrl Pts',(38.839403965417,779.319061971182,109.346681694276));
#84393=CARTESIAN_POINT('Ctrl Pts',(39.5222541565317,779.144197224472,109.284878576092));
#84394=CARTESIAN_POINT('Origin',(52.8776183915471,827.175936191914,121.458286566849));
#84395=CARTESIAN_POINT('Origin',(52.8776183915471,825.559694878252,125.51834395973));
#84396=CARTESIAN_POINT('Origin',(52.8776183915471,827.175936191914,121.458286566849));
#84397=CARTESIAN_POINT('Ctrl Pts',(53.6435222021547,775.36779391924,108.222950328633));
#84398=CARTESIAN_POINT('Ctrl Pts',(54.2751643466901,775.376386049419,108.22598707816));
#84399=CARTESIAN_POINT('Ctrl Pts',(54.9065432779137,775.395604598973,108.232779563848));
#84400=CARTESIAN_POINT('Ctrl Pts',(55.5374579069272,775.425443446955,108.243325622348));
#84401=CARTESIAN_POINT('Ctrl Pts',(53.6572481924173,774.424257074307,108.037580241535));
#84402=CARTESIAN_POINT('Ctrl Pts',(54.3002101839168,774.43300318661,108.040671413555));
#84403=CARTESIAN_POINT('Ctrl Pts',(54.9429042449805,774.452566157514,108.047585629402));
#84404=CARTESIAN_POINT('Ctrl Pts',(55.5851256829359,774.482939756375,108.058320686956));
#84405=CARTESIAN_POINT('Ctrl Pts',(53.6712359705142,773.44809401445,107.890070523166));
#84406=CARTESIAN_POINT('Ctrl Pts',(54.3257337058396,773.456997045688,107.893217155647));
#84407=CARTESIAN_POINT('Ctrl Pts',(54.979958703638,773.476911006889,107.900255423342));
#84408=CARTESIAN_POINT('Ctrl Pts',(55.6337025987302,773.507829555624,107.91118308462));
#84409=CARTESIAN_POINT('Origin',(52.8776183915471,827.175936191914,121.458286566849));
#84410=CARTESIAN_POINT('Ctrl Pts',(48.1619991748231,779.687415153512,109.332005249395));
#84411=CARTESIAN_POINT('Ctrl Pts',(48.8357364265094,779.625835415267,109.310240886297));
#84412=CARTESIAN_POINT('Ctrl Pts',(49.5106850110303,779.577464239345,109.293144876046));
#84413=CARTESIAN_POINT('Ctrl Pts',(50.1865536600841,779.542322499915,109.280724596282));
#84414=CARTESIAN_POINT('Ctrl Pts',(48.0629532561413,778.711286166964,109.02778511079));
#84415=CARTESIAN_POINT('Ctrl Pts',(48.7508415497114,778.648413020268,109.005563613381));
#84416=CARTESIAN_POINT('Ctrl Pts',(49.4399666187075,778.599025865885,108.988108521966));
#84417=CARTESIAN_POINT('Ctrl Pts',(50.130031077087,778.56314601642,108.97542736914));
#84418=CARTESIAN_POINT('Ctrl Pts',(47.9616810252838,777.693773274732,108.771738246455));
#84419=CARTESIAN_POINT('Ctrl Pts',(48.6640384418585,777.629577646898,108.749049339465));
#84420=CARTESIAN_POINT('Ctrl Pts',(49.3676586483386,777.57915167732,108.731227095611));
#84421=CARTESIAN_POINT('Ctrl Pts',(50.0722380034285,777.542517126896,108.71827920593));
#84422=CARTESIAN_POINT('Origin',(52.8776183915471,827.175936191914,121.458286566849));
#84423=CARTESIAN_POINT('Origin',(52.8776183915471,825.559694878252,125.51834395973));
#84424=CARTESIAN_POINT('Origin',(52.8776183915471,827.175936191914,121.458286566849));
#84425=CARTESIAN_POINT('Ctrl Pts',(64.7036892859012,776.620201057868,108.665594837008));
#84426=CARTESIAN_POINT('Ctrl Pts',(65.3179672524269,776.752533429287,108.712365574645));
#84427=CARTESIAN_POINT('Ctrl Pts',(65.929649521093,776.89515429438,108.762772614066));
#84428=CARTESIAN_POINT('Ctrl Pts',(66.5385422613663,777.048018459292,108.816799982235));
#84429=CARTESIAN_POINT('Ctrl Pts',(64.9163700462617,775.695883179202,108.487536320395));
#84430=CARTESIAN_POINT('Ctrl Pts',(65.5416952241698,775.830595423837,108.535148185752));
#84431=CARTESIAN_POINT('Ctrl Pts',(66.164378023034,775.975781191025,108.586461748359));
#84432=CARTESIAN_POINT('Ctrl Pts',(66.7842211264615,776.131394474147,108.641460747921));
#84433=CARTESIAN_POINT('Ctrl Pts',(65.1331213486505,774.739141244516,108.347756181132));
#84434=CARTESIAN_POINT('Ctrl Pts',(65.7697051728548,774.876278911263,108.39622527273));
#84435=CARTESIAN_POINT('Ctrl Pts',(66.4035990433899,775.024078670752,108.448462708663));
#84436=CARTESIAN_POINT('Ctrl Pts',(67.0346020912866,775.182493688035,108.504451935877));
#84437=CARTESIAN_POINT('Origin',(52.8776183915471,827.175936191914,121.458286566849));
#84438=CARTESIAN_POINT('Ctrl Pts',(58.4091473829218,779.76738491836,109.360315888696));
#84439=CARTESIAN_POINT('Ctrl Pts',(59.0834071649073,779.839801671071,109.385910419386));
#84440=CARTESIAN_POINT('Ctrl Pts',(59.7559212371808,779.925441548512,109.416178449772));
#84441=CARTESIAN_POINT('Ctrl Pts',(60.4263979154771,780.02426740677,109.451106851937));
#84442=CARTESIAN_POINT('Ctrl Pts',(58.5251440477691,778.794488373911,109.057209042452));
#84443=CARTESIAN_POINT('Ctrl Pts',(59.2135431185612,778.868423712496,109.083340292773));
#84444=CARTESIAN_POINT('Ctrl Pts',(59.9001598719503,778.955859465938,109.114243046502));
#84445=CARTESIAN_POINT('Ctrl Pts',(60.5846965070255,779.05675771141,109.149903900429));
#84446=CARTESIAN_POINT('Ctrl Pts',(58.6437438476791,777.780377886812,108.802135529116));
#84447=CARTESIAN_POINT('Ctrl Pts',(59.3465995136287,777.855865890564,108.828815543843));
#84448=CARTESIAN_POINT('Ctrl Pts',(60.0476354329541,777.945137822094,108.860367265037));
#84449=CARTESIAN_POINT('Ctrl Pts',(60.7465475508325,778.048154962186,108.896777008017));
#84450=CARTESIAN_POINT('Origin',(52.8776183915471,827.175936191914,121.458286566849));
#84451=CARTESIAN_POINT('Origin',(52.8776183915471,825.559694878252,125.51834395973));
#84452=CARTESIAN_POINT('Origin',(52.8776183915471,827.175936191914,121.458286566849));
#84453=CARTESIAN_POINT('Origin',(52.8776183915471,825.559694878252,125.51834395973));
#84454=CARTESIAN_POINT('Origin',(52.8776183915471,827.175936191914,121.458286566849));
#84455=CARTESIAN_POINT('Ctrl Pts',(75.2378334424178,780.001886138673,109.86318891898));
#84456=CARTESIAN_POINT('Ctrl Pts',(75.8111772114877,780.252813357473,109.951875088439));
#84457=CARTESIAN_POINT('Ctrl Pts',(76.3796786218251,780.51335069488,110.04395779898));
#84458=CARTESIAN_POINT('Ctrl Pts',(76.9431564894166,780.783415116447,110.139407703419));
#84459=CARTESIAN_POINT('Ctrl Pts',(75.6395522221989,779.139143914756,109.707161743586));
#84460=CARTESIAN_POINT('Ctrl Pts',(76.2231965612223,779.394579237611,109.797441229553));
#84461=CARTESIAN_POINT('Ctrl Pts',(76.8019115447451,779.659797332383,109.891178278124));
#84462=CARTESIAN_POINT('Ctrl Pts',(77.3755127336413,779.934713672844,109.98834301487));
#84463=CARTESIAN_POINT('Ctrl Pts',(76.0489516266781,778.245201444726,109.589757869781));
#84464=CARTESIAN_POINT('Ctrl Pts',(76.6430934764404,778.505231063911,109.681661135523));
#84465=CARTESIAN_POINT('Ctrl Pts',(77.2322173106074,778.77521940935,109.777084152086));
#84466=CARTESIAN_POINT('Ctrl Pts',(77.8161353727047,779.055080434516,109.875996507714));
#84467=CARTESIAN_POINT('Origin',(52.8776183915471,827.175936191914,121.458286566849));
#84468=CARTESIAN_POINT('Ctrl Pts',(68.4183096607616,781.857910547663,110.099377322435));
#84469=CARTESIAN_POINT('Ctrl Pts',(69.0612797297983,782.061204974069,110.171228451366));
#84470=CARTESIAN_POINT('Ctrl Pts',(69.6996238599015,782.277070010889,110.247522459354));
#84471=CARTESIAN_POINT('Ctrl Pts',(70.333065618516,782.505412178569,110.328226307563));
#84472=CARTESIAN_POINT('Ctrl Pts',(68.7452591349629,780.925783914164,109.810967425304));
#84473=CARTESIAN_POINT('Ctrl Pts',(69.4017561908213,781.133355306418,109.884330178681));
#84474=CARTESIAN_POINT('Ctrl Pts',(70.0535299859299,781.353761773157,109.962229281665));
#84475=CARTESIAN_POINT('Ctrl Pts',(70.7002982720667,781.586907868177,110.044631000341));
#84476=CARTESIAN_POINT('Ctrl Pts',(69.0795696415712,779.95316335926,109.571259129136));
#84477=CARTESIAN_POINT('Ctrl Pts',(69.7498982346366,780.165108010175,109.646167540096));
#84478=CARTESIAN_POINT('Ctrl Pts',(70.4154040540052,780.390158153862,109.725707875637));
#84479=CARTESIAN_POINT('Ctrl Pts',(71.0757989048528,780.628216333193,109.809845691112));
#84480=CARTESIAN_POINT('Origin',(52.8776183915471,827.175936191914,121.458286566849));
#84481=CARTESIAN_POINT('Origin',(52.8776183915471,825.559694878252,125.51834395973));
#84482=CARTESIAN_POINT('Origin',(52.8776183915471,827.175936191914,121.458286566849));
#84483=CARTESIAN_POINT('Origin',(52.8776183915471,825.559694878252,125.51834395973));
#84484=CARTESIAN_POINT('Origin',(52.8776183915471,827.175936191914,121.458286566849));
#84485=CARTESIAN_POINT('Ctrl Pts',(84.7978201531078,785.382466127243,111.767254473936));
#84486=CARTESIAN_POINT('Ctrl Pts',(85.3021477216854,785.739908233174,111.893586608527));
#84487=CARTESIAN_POINT('Ctrl Pts',(85.799642046942,786.105763910382,112.022892383889));
#84488=CARTESIAN_POINT('Ctrl Pts',(86.2901452539088,786.479917058139,112.155130766095));
#84489=CARTESIAN_POINT('Ctrl Pts',(85.3722795647444,784.614952542165,111.645559022608));
#84490=CARTESIAN_POINT('Ctrl Pts',(85.8856833829171,784.978827438946,111.774164723145));
#84491=CARTESIAN_POINT('Ctrl Pts',(86.3921309816998,785.351267323819,111.905797580278));
#84492=CARTESIAN_POINT('Ctrl Pts',(86.8914616448896,785.732154006619,112.040415821602));
#84493=CARTESIAN_POINT('Ctrl Pts',(85.9577410185038,783.817981991301,111.563287639805));
#84494=CARTESIAN_POINT('Ctrl Pts',(86.4803949145324,784.188412879694,111.694210449606));
#84495=CARTESIAN_POINT('Ctrl Pts',(86.9959672598652,784.567563072923,111.828214956761));
#84496=CARTESIAN_POINT('Ctrl Pts',(87.50429444265,784.955312251376,111.965258636247));
#84497=CARTESIAN_POINT('Origin',(52.8776183915471,827.175936191914,121.458286566849));
#84498=CARTESIAN_POINT('Ctrl Pts',(77.7523941907489,785.863531124246,111.515718880779));
#84499=CARTESIAN_POINT('Ctrl Pts',(78.3358113354591,786.188591421181,111.630606188406));
#84500=CARTESIAN_POINT('Ctrl Pts',(78.9119357508628,786.525015861201,111.749509968715));
#84501=CARTESIAN_POINT('Ctrl Pts',(79.4805184652575,786.872659058756,111.872378837532));
#84502=CARTESIAN_POINT('Ctrl Pts',(78.274356371013,785.017733856259,111.258191966894));
#84503=CARTESIAN_POINT('Ctrl Pts',(78.8700157038463,785.349615086282,111.375490023066));
#84504=CARTESIAN_POINT('Ctrl Pts',(79.458229279707,785.693098919947,111.496888831949));
#84505=CARTESIAN_POINT('Ctrl Pts',(80.0387429025715,786.048036920993,111.622335931147));
#84506=CARTESIAN_POINT('Ctrl Pts',(78.808039345768,784.133535105251,111.049797417012));
#84507=CARTESIAN_POINT('Ctrl Pts',(79.4162157681955,784.472390434162,111.169560355706));
#84508=CARTESIAN_POINT('Ctrl Pts',(80.0167899697085,784.823092181966,111.29351021967));
#84509=CARTESIAN_POINT('Ctrl Pts',(80.6095024126493,785.185488793185,111.421593444071));
#84510=CARTESIAN_POINT('Origin',(52.8776183915471,827.175936191914,121.458286566849));
#84511=CARTESIAN_POINT('Ctrl Pts',(92.9661650926069,792.518247313548,114.29315925778));
#84512=CARTESIAN_POINT('Ctrl Pts',(93.3806595130324,792.967234459711,114.451846507093));
#84513=CARTESIAN_POINT('Ctrl Pts',(93.7866039081684,793.423113039347,114.612969422174));
#84514=CARTESIAN_POINT('Ctrl Pts',(94.1838694119097,793.885738334861,114.776476854927));
#84515=CARTESIAN_POINT('Ctrl Pts',(93.6856293079454,791.88073464461,114.217671724052));
#84516=CARTESIAN_POINT('Ctrl Pts',(94.1075626087368,792.337779707844,114.379206913905));
#84517=CARTESIAN_POINT('Ctrl Pts',(94.5207924379869,792.80183988426,114.543221482119));
#84518=CARTESIAN_POINT('Ctrl Pts',(94.9251876168462,793.272767859034,114.709663362651));
#84519=CARTESIAN_POINT('Ctrl Pts',(94.4188341119727,791.216367871884,114.182274053281));
#84520=CARTESIAN_POINT('Ctrl Pts',(94.8483483635669,791.681624745213,114.346711574676));
#84521=CARTESIAN_POINT('Ctrl Pts',(95.2690027667957,792.154022773513,114.513673021864));
#84522=CARTESIAN_POINT('Ctrl Pts',(95.6806637858958,792.633411995128,114.683105393322));
#84523=CARTESIAN_POINT('Origin',(52.8776183915471,827.175936191914,121.458286566849));
#84524=CARTESIAN_POINT('Ctrl Pts',(85.9972328647244,791.603786356977,113.5456214498));
#84525=CARTESIAN_POINT('Ctrl Pts',(86.4968504914115,792.037099733043,113.698769058426));
#84526=CARTESIAN_POINT('Ctrl Pts',(86.9867952965917,792.48012280452,113.855348401947));
#84527=CARTESIAN_POINT('Ctrl Pts',(87.4668550512191,792.932663667419,114.015291654998));
#84528=CARTESIAN_POINT('Ctrl Pts',(86.6918182644616,790.878584527844,113.331530897999));
#84529=CARTESIAN_POINT('Ctrl Pts',(87.2019138847627,791.320985363089,113.487890322181));
#84530=CARTESIAN_POINT('Ctrl Pts',(87.7021338248975,791.773299525725,113.647753451688));
#84531=CARTESIAN_POINT('Ctrl Pts',(88.192261404947,792.235331087145,113.811051038723));
#84532=CARTESIAN_POINT('Ctrl Pts',(87.4019915546031,790.117715985974,113.167502367862));
#84533=CARTESIAN_POINT('Ctrl Pts',(87.9228003157242,790.569408221219,113.327145687187));
#84534=CARTESIAN_POINT('Ctrl Pts',(88.4335259854642,791.031221985746,113.49036629743));
#84535=CARTESIAN_POINT('Ctrl Pts',(88.9339473331445,791.502957236012,113.657093496435));
#84536=CARTESIAN_POINT('Origin',(52.8776183915471,827.175936191914,121.458286566849));
#84537=CARTESIAN_POINT('Ctrl Pts',(99.3836913129681,801.093665801638,117.329369223643));
#84538=CARTESIAN_POINT('Ctrl Pts',(99.6902065779454,801.614669831695,117.513509676477));
#84539=CARTESIAN_POINT('Ctrl Pts',(99.9868254004947,802.140741376905,117.69944116063));
#84540=CARTESIAN_POINT('Ctrl Pts',(100.273453568563,802.671713346455,117.887104620555));
#84541=CARTESIAN_POINT('Ctrl Pts',(100.217916781638,800.61003260618,117.30912382607));
#84542=CARTESIAN_POINT('Ctrl Pts',(100.529930314357,801.140382401292,117.496567388496));
#84543=CARTESIAN_POINT('Ctrl Pts',(100.831869882365,801.675890612593,117.685834109743));
#84544=CARTESIAN_POINT('Ctrl Pts',(101.123639583632,802.216387151997,117.876863874926));
#84545=CARTESIAN_POINT('Ctrl Pts',(101.068066047063,800.102499844735,117.32999314988));
#84546=CARTESIAN_POINT('Ctrl Pts',(101.385682799126,800.642373797997,117.520802872055));
#84547=CARTESIAN_POINT('Ctrl Pts',(101.693044675624,801.187498803613,117.713468493806));
#84548=CARTESIAN_POINT('Ctrl Pts',(101.990054052297,801.737701719013,117.907928820689));
#84549=CARTESIAN_POINT('Origin',(52.8776183915471,827.175936191914,121.458286566849));
#84550=CARTESIAN_POINT('Ctrl Pts',(92.7914283577236,798.843631763094,116.10536273626));
#84551=CARTESIAN_POINT('Ctrl Pts',(93.1830725017883,799.363954194011,116.289262288895));
#84552=CARTESIAN_POINT('Ctrl Pts',(93.5631886174356,799.891821941612,116.475828611749));
#84553=CARTESIAN_POINT('Ctrl Pts',(93.9316132340898,800.427007994094,116.664981471169));
#84554=CARTESIAN_POINT('Ctrl Pts',(93.6299721692471,798.269043655217,115.945277016441));
#84555=CARTESIAN_POINT('Ctrl Pts',(94.0298443119319,798.800297469402,116.133040089796));
#84556=CARTESIAN_POINT('Ctrl Pts',(94.4179462354163,799.339255118804,116.323525959183));
#84557=CARTESIAN_POINT('Ctrl Pts',(94.7941110347935,799.88568482236,116.516652705331));
#84558=CARTESIAN_POINT('Ctrl Pts',(94.4873670344129,797.662074949797,115.836662038794));
#84559=CARTESIAN_POINT('Ctrl Pts',(94.8956521469038,798.204505892421,116.028375487527));
#84560=CARTESIAN_POINT('Ctrl Pts',(95.2919194047924,798.754802752404,116.222869017605));
#84561=CARTESIAN_POINT('Ctrl Pts',(95.6759983916348,799.312728872205,116.420058986245));
#84562=CARTESIAN_POINT('Origin',(52.8776183915471,827.175936191914,121.458286566849));
#84563=CARTESIAN_POINT('Ctrl Pts',(103.763049025154,810.745309098518,120.745216801789));
#84564=CARTESIAN_POINT('Ctrl Pts',(103.947373053888,811.313710833613,120.946109207325));
#84565=CARTESIAN_POINT('Ctrl Pts',(104.120955679622,811.885110913332,121.148061329302));
#84566=CARTESIAN_POINT('Ctrl Pts',(104.283742090387,812.459328907384,121.351009397552));
#84567=CARTESIAN_POINT('Ctrl Pts',(104.677088626,810.434154205991,120.786938235321));
#84568=CARTESIAN_POINT('Ctrl Pts',(104.864723611516,811.012765969549,120.99143921038));
#84569=CARTESIAN_POINT('Ctrl Pts',(105.041424249458,811.594429936087,121.197018937247));
#84570=CARTESIAN_POINT('Ctrl Pts',(105.207134743288,812.178962434302,121.403612500268));
#84571=CARTESIAN_POINT('Ctrl Pts',(105.60859894153,810.102340362435,120.871081935004));
#84572=CARTESIAN_POINT('Ctrl Pts',(105.799608168593,810.691357306277,121.079260452844));
#84573=CARTESIAN_POINT('Ctrl Pts',(105.979486415616,811.283481340892,121.288537121695));
#84574=CARTESIAN_POINT('Ctrl Pts',(106.148176882671,811.878525492014,121.498845858524));
#84575=CARTESIAN_POINT('Origin',(52.8776183915471,827.175936191914,121.458286566849));
#84576=CARTESIAN_POINT('Ctrl Pts',(97.844501095678,807.253538512874,119.079062323388));
#84577=CARTESIAN_POINT('Ctrl Pts',(98.1134360590212,807.841098387078,119.286725863517));
#84578=CARTESIAN_POINT('Ctrl Pts',(98.3693602313756,808.433801630878,119.496207244492));
#84579=CARTESIAN_POINT('Ctrl Pts',(98.6121630384352,809.031392161588,119.707415958026));
#84580=CARTESIAN_POINT('Ctrl Pts',(98.7871151231428,806.85621056334,118.982521982872));
#84581=CARTESIAN_POINT('Ctrl Pts',(99.0616876102297,807.456087105858,119.194538650328));
#84582=CARTESIAN_POINT('Ctrl Pts',(99.3229765688517,808.061214835372,119.408411264947));
#84583=CARTESIAN_POINT('Ctrl Pts',(99.5708691067994,808.671332301084,119.624047421171));
#84584=CARTESIAN_POINT('Ctrl Pts',(99.7508719466112,806.430588090693,118.938656702047));
#84585=CARTESIAN_POINT('Ctrl Pts',(100.03120840688,807.043057563918,119.155124137308));
#84586=CARTESIAN_POINT('Ctrl Pts',(100.297982483717,807.660888459877,119.373486480771));
#84587=CARTESIAN_POINT('Ctrl Pts',(100.551078915019,808.283813839258,119.593649387051));
#84588=CARTESIAN_POINT('Origin',(52.8776183915471,827.175936191914,121.458286566849));
#84589=CARTESIAN_POINT('Ctrl Pts',(105.922015646428,821.04073406854,124.389683333783));
#84590=CARTESIAN_POINT('Ctrl Pts',(105.976969940256,821.633474172943,124.599177742542));
#84591=CARTESIAN_POINT('Ctrl Pts',(106.020740371651,822.227041648839,124.808964572381));
#84592=CARTESIAN_POINT('Ctrl Pts',(106.053313108912,822.821248925566,125.018977529483));
#84593=CARTESIAN_POINT('Ctrl Pts',(106.872914726583,820.914491596563,124.497433171603));
#84594=CARTESIAN_POINT('Ctrl Pts',(106.928854157205,821.517857441841,124.710683076718));
#84595=CARTESIAN_POINT('Ctrl Pts',(106.97340923816,822.122065490465,124.924230644992));
#84596=CARTESIAN_POINT('Ctrl Pts',(107.006565889793,822.726924809295,125.138008394194));
#84597=CARTESIAN_POINT('Ctrl Pts',(107.841951609362,820.771184791302,124.648706674861));
#84598=CARTESIAN_POINT('Ctrl Pts',(107.898894967643,821.385379056786,124.865783710065));
#84599=CARTESIAN_POINT('Ctrl Pts',(107.944249664856,822.000430640379,125.083163750497));
#84600=CARTESIAN_POINT('Ctrl Pts',(107.97800136866,822.616145182324,125.300778102843));
#84601=CARTESIAN_POINT('Origin',(52.8776183915471,827.175936191914,121.458286566849));
#84602=CARTESIAN_POINT('Ctrl Pts',(100.932612370989,816.47036724468,122.338107749172));
#84603=CARTESIAN_POINT('Ctrl Pts',(101.065805084989,817.097055564791,122.559600606029));
#84604=CARTESIAN_POINT('Ctrl Pts',(101.185180748678,817.726214116847,122.781966526437));
#84605=CARTESIAN_POINT('Ctrl Pts',(101.290687985324,818.357572124469,123.005109808863));
#84606=CARTESIAN_POINT('Ctrl Pts',(101.939753753683,816.265959562204,122.310820246181));
#84607=CARTESIAN_POINT('Ctrl Pts',(102.075737933939,816.905782078971,122.536955172542));
#84608=CARTESIAN_POINT('Ctrl Pts',(102.197615484758,817.548126599052,122.763981460209));
#84609=CARTESIAN_POINT('Ctrl Pts',(102.30533395265,818.192716671109,122.991801401925));
#84610=CARTESIAN_POINT('Ctrl Pts',(102.969479515644,816.037588240675,122.337754166415));
#84611=CARTESIAN_POINT('Ctrl Pts',(103.108317758664,816.690839478466,122.568635257159));
#84612=CARTESIAN_POINT('Ctrl Pts',(103.232753299529,817.346665651872,122.800426417274));
#84613=CARTESIAN_POINT('Ctrl Pts',(103.342732583845,818.004784507343,123.033027888805));
#84614=CARTESIAN_POINT('Origin',(52.8776183915471,827.175936191914,121.458286566849));
#84615=CARTESIAN_POINT('Ctrl Pts',(105.761429506502,831.539389861825,128.105886396078));
#84616=CARTESIAN_POINT('Ctrl Pts',(105.684526018595,832.12929698831,128.314379534585));
#84617=CARTESIAN_POINT('Ctrl Pts',(105.596532411993,832.717824608245,128.5223851088));
#84618=CARTESIAN_POINT('Ctrl Pts',(105.497476395537,833.304787396605,128.729837618589));
#84619=CARTESIAN_POINT('Ctrl Pts',(106.709627746758,831.601093240578,128.28105038138));
#84620=CARTESIAN_POINT('Ctrl Pts',(106.631345391663,832.201577307103,128.493281768376));
#84621=CARTESIAN_POINT('Ctrl Pts',(106.541774073826,832.800657132747,128.705016849131));
#84622=CARTESIAN_POINT('Ctrl Pts',(106.440941998903,833.398144069637,128.916188949105));
#84623=CARTESIAN_POINT('Ctrl Pts',(107.675914903239,831.649307998338,128.501051019185));
#84624=CARTESIAN_POINT('Ctrl Pts',(107.596227376105,832.260570782731,128.717091969783));
#84625=CARTESIAN_POINT('Ctrl Pts',(107.505048248806,832.870404120053,128.932627705419));
#84626=CARTESIAN_POINT('Ctrl Pts',(107.402406233289,833.478615976192,129.147590354741));
#84627=CARTESIAN_POINT('Origin',(52.8776183915471,827.175936191914,121.458286566849));
#84628=CARTESIAN_POINT('Ctrl Pts',(101.919463205941,826.096733439178,125.741939549448));
#84629=CARTESIAN_POINT('Ctrl Pts',(101.911465154775,826.733418377351,125.966965549372));
#84630=CARTESIAN_POINT('Ctrl Pts',(101.889523384275,827.369811805957,126.191888519951));
#84631=CARTESIAN_POINT('Ctrl Pts',(101.853647253075,828.005642289612,126.416612526737));
#84632=CARTESIAN_POINT('Ctrl Pts',(102.946478823582,826.093748663403,125.786887623192));
#84633=CARTESIAN_POINT('Ctrl Pts',(102.938313280277,826.743766814824,126.016626031818));
#84634=CARTESIAN_POINT('Ctrl Pts',(102.915912013585,827.393487351997,126.246259253499));
#84635=CARTESIAN_POINT('Ctrl Pts',(102.879284578122,828.042633155239,126.475689344762));
#84636=CARTESIAN_POINT('Ctrl Pts',(103.996505226553,826.071342075713,125.887605326046));
#84637=CARTESIAN_POINT('Ctrl Pts',(103.988168438367,826.734992177522,126.122161727189));
#84638=CARTESIAN_POINT('Ctrl Pts',(103.965297380245,827.398338423622,126.356610735442));
#84639=CARTESIAN_POINT('Ctrl Pts',(103.927901807182,828.061097882676,126.590852353298));
#84640=CARTESIAN_POINT('Origin',(52.8776183915471,827.175936191914,121.458286566849));
#84641=CARTESIAN_POINT('Ctrl Pts',(103.290428074605,841.770498106016,131.727402106468));
#84642=CARTESIAN_POINT('Ctrl Pts',(103.084642224443,842.334153467199,131.926616982866));
#84643=CARTESIAN_POINT('Ctrl Pts',(102.868256026129,842.89426875693,132.124580678231));
#84644=CARTESIAN_POINT('Ctrl Pts',(102.64133793703,843.450666773438,132.321230563463));
#84645=CARTESIAN_POINT('Ctrl Pts',(104.192978406205,842.015017669718,131.967882763203));
#84646=CARTESIAN_POINT('Ctrl Pts',(103.983508331965,842.588764262402,132.170664222258));
#84647=CARTESIAN_POINT('Ctrl Pts',(103.763248129479,843.158907405048,132.372172100145));
#84648=CARTESIAN_POINT('Ctrl Pts',(103.53226748172,843.725266723403,132.572342646498));
#84649=CARTESIAN_POINT('Ctrl Pts',(105.112720530425,842.249568871481,132.25432659535));
#84650=CARTESIAN_POINT('Ctrl Pts',(104.899496054949,842.8335989136,132.460742573385));
#84651=CARTESIAN_POINT('Ctrl Pts',(104.6752880562,843.413960919856,132.665862143435));
#84652=CARTESIAN_POINT('Ctrl Pts',(104.4401674661,843.990471283092,132.869620412519));
#84653=CARTESIAN_POINT('Origin',(52.8776183915471,827.175936191914,121.458286566849));
#84654=CARTESIAN_POINT('Ctrl Pts',(100.765958536865,835.701990838064,129.138530074238));
#84655=CARTESIAN_POINT('Ctrl Pts',(100.617419197977,836.324774219662,129.358642793697));
#84656=CARTESIAN_POINT('Ctrl Pts',(100.455247155973,836.94452713004,129.577684442088));
#84657=CARTESIAN_POINT('Ctrl Pts',(100.279511819792,837.56098431761,129.795561270526));
#84658=CARTESIAN_POINT('Ctrl Pts',(101.767197580229,835.89946903489,129.255457648539));
#84659=CARTESIAN_POINT('Ctrl Pts',(101.615552613017,836.535273436538,129.480172437062));
#84660=CARTESIAN_POINT('Ctrl Pts',(101.449989913085,837.16798400653,129.703793760794));
#84661=CARTESIAN_POINT('Ctrl Pts',(101.270580340559,837.797329947456,129.92622591077));
#84662=CARTESIAN_POINT('Ctrl Pts',(102.790832383946,836.0820659331,129.429603528724));
#84663=CARTESIAN_POINT('Ctrl Pts',(102.636012321573,836.731182609566,129.659023325598));
#84664=CARTESIAN_POINT('Ctrl Pts',(102.466983121322,837.377140676691,129.887326763058));
#84665=CARTESIAN_POINT('Ctrl Pts',(102.283817126965,838.019663667193,130.11441612821));
#84666=CARTESIAN_POINT('Origin',(52.8776183915471,827.175936191914,121.458286566849));
#84667=CARTESIAN_POINT('Ctrl Pts',(98.6188091293693,851.302769029011,135.10252964045));
#84668=CARTESIAN_POINT('Ctrl Pts',(98.2939262573026,851.812906345545,135.282829429041));
#84669=CARTESIAN_POINT('Ctrl Pts',(97.9594953788288,852.317528965392,135.461180137228));
#84670=CARTESIAN_POINT('Ctrl Pts',(97.6156217655107,852.816478044332,135.63752562409));
#84671=CARTESIAN_POINT('Ctrl Pts',(99.4361478251386,851.716860219949,135.403672389488));
#84672=CARTESIAN_POINT('Ctrl Pts',(99.1054596966138,852.23611306151,135.587193913055));
#84673=CARTESIAN_POINT('Ctrl Pts',(98.7650529505767,852.749752665553,135.768731528554));
#84674=CARTESIAN_POINT('Ctrl Pts',(98.4150347396632,853.257617349506,135.948228091895));
#84675=CARTESIAN_POINT('Ctrl Pts',(100.26902456131,852.124249564078,135.751775289756));
#84676=CARTESIAN_POINT('Ctrl Pts',(99.9324208153347,852.652791221614,135.938579795183));
#84677=CARTESIAN_POINT('Ctrl Pts',(99.5859245973349,853.175619227485,136.123364902786));
#84678=CARTESIAN_POINT('Ctrl Pts',(99.2296449767795,853.692569006813,136.306072446233));
#84679=CARTESIAN_POINT('Origin',(52.8776183915471,827.175936191914,121.458286566849));
#84680=CARTESIAN_POINT('Ctrl Pts',(97.5139865755203,844.864516615738,132.378233576775));
#84681=CARTESIAN_POINT('Ctrl Pts',(97.2312091993379,845.445397385802,132.583536495507));
#84682=CARTESIAN_POINT('Ctrl Pts',(96.9357387751277,846.020634534243,132.786844767402));
#84683=CARTESIAN_POINT('Ctrl Pts',(96.627701932469,846.589981532028,132.988071260757));
#84684=CARTESIAN_POINT('Ctrl Pts',(98.4487596583488,845.253923252333,132.563977905155));
#84685=CARTESIAN_POINT('Ctrl Pts',(98.1600603693754,845.846968804844,132.773580269611));
#84686=CARTESIAN_POINT('Ctrl Pts',(97.8584022150573,846.434252547228,132.981146215412));
#84687=CARTESIAN_POINT('Ctrl Pts',(97.5439144768452,847.015522787652,133.186586786147));
#84688=CARTESIAN_POINT('Ctrl Pts',(99.4044750958214,845.632687821054,132.808678028001));
#84689=CARTESIAN_POINT('Ctrl Pts',(99.1097212214331,846.238170691874,133.022676161574));
#84690=CARTESIAN_POINT('Ctrl Pts',(98.8017367090974,846.837770916207,133.234595168834));
#84691=CARTESIAN_POINT('Ctrl Pts',(98.4806535515487,847.43123152375,133.444344227781));
#84692=CARTESIAN_POINT('Origin',(52.8776183915471,827.175936191914,121.458286566849));
#84693=CARTESIAN_POINT('Ctrl Pts',(91.9417831532315,859.700313020388,138.074190482449));
#84694=CARTESIAN_POINT('Ctrl Pts',(91.5121277434549,860.135379853124,138.227957821992));
#84695=CARTESIAN_POINT('Ctrl Pts',(91.074364555794,860.563201391009,138.379164429184));
#84696=CARTESIAN_POINT('Ctrl Pts',(90.6286310070099,860.983643338031,138.52776283927));
#84697=CARTESIAN_POINT('Ctrl Pts',(92.6415135252399,860.265659888805,138.429787896317));
#84698=CARTESIAN_POINT('Ctrl Pts',(92.2041619841994,860.708519784021,138.586309567825));
#84699=CARTESIAN_POINT('Ctrl Pts',(91.7585574360481,861.144004604244,138.740224638289));
#84700=CARTESIAN_POINT('Ctrl Pts',(91.3048397590019,861.571977647906,138.891484792749));
#84701=CARTESIAN_POINT('Ctrl Pts',(93.3545782125711,860.827132606148,138.833605402784));
#84702=CARTESIAN_POINT('Ctrl Pts',(92.9093838800028,861.277934071264,138.992933893805));
#84703=CARTESIAN_POINT('Ctrl Pts',(92.4557885435564,861.721228208107,139.149609040998));
#84704=CARTESIAN_POINT('Ctrl Pts',(91.9939345898091,862.156875863715,139.303581662996));
#84705=CARTESIAN_POINT('Origin',(52.8776183915471,827.175936191914,121.458286566849));
#84706=CARTESIAN_POINT('Ctrl Pts',(92.3139898798326,853.195701951383,135.324194005371));
#84707=CARTESIAN_POINT('Ctrl Pts',(91.9087941278747,853.709482121067,135.505781301524));
#84708=CARTESIAN_POINT('Ctrl Pts',(91.492392464683,854.215234701004,135.68453137584));
#84709=CARTESIAN_POINT('Ctrl Pts',(91.0649637439505,854.712742459312,135.860367451222));
#84710=CARTESIAN_POINT('Ctrl Pts',(93.1370644539869,853.757382363456,135.571601530681));
#84711=CARTESIAN_POINT('Ctrl Pts',(92.7234118813732,854.28188561385,135.756978726381));
#84712=CARTESIAN_POINT('Ctrl Pts',(92.2983195195021,854.798193731065,135.939459484727));
#84713=CARTESIAN_POINT('Ctrl Pts',(91.8619699549135,855.306084949383,136.118965426209));
#84714=CARTESIAN_POINT('Ctrl Pts',(93.9785156047657,854.312363461301,135.87896966896));
#84715=CARTESIAN_POINT('Ctrl Pts',(93.5562173982128,854.8478292039,136.068221380331));
#84716=CARTESIAN_POINT('Ctrl Pts',(93.122240302644,855.374928529188,136.254516116739));
#84717=CARTESIAN_POINT('Ctrl Pts',(92.676770720788,855.893435036387,136.43777386049));
#84718=CARTESIAN_POINT('Origin',(52.8776183915471,827.175936191914,121.458286566849));
#84719=CARTESIAN_POINT('Ctrl Pts',(83.5602516028411,866.611482450665,140.520652182709));
#84720=CARTESIAN_POINT('Ctrl Pts',(83.0432523771499,866.953693687156,140.641601212692));
#84721=CARTESIAN_POINT('Ctrl Pts',(82.5198948914167,867.287202629092,140.759474557329));
#84722=CARTESIAN_POINT('Ctrl Pts',(81.9903439038852,867.611904284474,140.874235108896));
#84723=CARTESIAN_POINT('Ctrl Pts',(84.1086002196864,867.298879563462,140.919669805206));
#84724=CARTESIAN_POINT('Ctrl Pts',(83.5823613759883,867.647206671981,141.042780391299));
#84725=CARTESIAN_POINT('Ctrl Pts',(83.0496506397879,867.986675961771,141.162760324541));
#84726=CARTESIAN_POINT('Ctrl Pts',(82.5106357138271,868.317180564455,141.279571834033));
#84727=CARTESIAN_POINT('Ctrl Pts',(84.667374327897,867.984762138475,141.367536623201));
#84728=CARTESIAN_POINT('Ctrl Pts',(84.1317201977308,868.339321397187,141.492849862042));
#84729=CARTESIAN_POINT('Ctrl Pts',(83.589478382162,868.684864356089,141.614976435456));
#84730=CARTESIAN_POINT('Ctrl Pts',(83.0408195844131,869.021282234752,141.733877896759));
#84731=CARTESIAN_POINT('Origin',(52.8776183915471,827.175936191914,121.458286566849));
#84732=CARTESIAN_POINT('Ctrl Pts',(85.3908378832772,860.329215965232,137.846832736418));
#84733=CARTESIAN_POINT('Ctrl Pts',(84.8819518685354,860.752084986696,137.996288956734));
#84734=CARTESIAN_POINT('Ctrl Pts',(84.3638957786647,861.164937009303,138.142204830721));
#84735=CARTESIAN_POINT('Ctrl Pts',(83.8368913789253,861.5675953027,138.284517895892));
#84736=CARTESIAN_POINT('Ctrl Pts',(86.0696628273966,861.03975848912,138.147777713084));
#84737=CARTESIAN_POINT('Ctrl Pts',(85.5501520721363,861.471456351417,138.300354344482));
#84738=CARTESIAN_POINT('Ctrl Pts',(85.0212797849848,861.892928075657,138.449316712681));
#84739=CARTESIAN_POINT('Ctrl Pts',(84.4832723613125,862.303993241637,138.594601051076));
#84740=CARTESIAN_POINT('Ctrl Pts',(86.7636485216625,861.74691198598,138.509932643049));
#84741=CARTESIAN_POINT('Ctrl Pts',(86.2332757349034,862.187635870799,138.66569937621));
#84742=CARTESIAN_POINT('Ctrl Pts',(85.6933456835311,862.617919807489,138.817776278457));
#84743=CARTESIAN_POINT('Ctrl Pts',(85.1440894964343,863.037579603581,138.96609824994));
#84744=CARTESIAN_POINT('Origin',(52.8776183915471,827.175936191914,121.458286566849));
#84745=CARTESIAN_POINT('Ctrl Pts',(73.8390976335837,871.728561617911,142.332123170967));
#84746=CARTESIAN_POINT('Ctrl Pts',(73.2579608975552,871.962320061041,142.414741314184));
#84747=CARTESIAN_POINT('Ctrl Pts',(72.6725173783085,872.186321648689,142.493911054542));
#84748=CARTESIAN_POINT('Ctrl Pts',(72.0829513316637,872.400495881149,142.56960747506));
#84749=CARTESIAN_POINT('Ctrl Pts',(74.2138218059742,872.50749828857,142.764025385591));
#84750=CARTESIAN_POINT('Ctrl Pts',(73.6222962047354,872.74543558464,142.848120476832));
#84751=CARTESIAN_POINT('Ctrl Pts',(73.0263868287761,872.973441603873,142.928705518806));
#84752=CARTESIAN_POINT('Ctrl Pts',(72.4262812278209,873.191444586254,143.005755149094));
#84753=CARTESIAN_POINT('Ctrl Pts',(74.59567234048,873.286654376598,143.245433677184));
#84754=CARTESIAN_POINT('Ctrl Pts',(73.9935603025345,873.528849997446,143.331033804486));
#84755=CARTESIAN_POINT('Ctrl Pts',(73.3869860341711,873.760936603024,143.413061063744));
#84756=CARTESIAN_POINT('Ctrl Pts',(72.776140441661,873.98284114904,143.491489638634));
#84757=CARTESIAN_POINT('Origin',(52.8776183915471,827.175936191914,121.458286566849));
#84758=CARTESIAN_POINT('Ctrl Pts',(77.0446291096948,865.943081673865,139.831814242213));
#84759=CARTESIAN_POINT('Ctrl Pts',(76.4547328300808,866.25679917775,139.942692622983));
#84760=CARTESIAN_POINT('Ctrl Pts',(75.8580915804765,866.558965055531,140.049488268229));
#84761=CARTESIAN_POINT('Ctrl Pts',(75.2549597919521,866.849450451907,140.152155636127));
#84762=CARTESIAN_POINT('Ctrl Pts',(77.5495692953528,866.771277650764,140.174917758729));
#84763=CARTESIAN_POINT('Ctrl Pts',(76.9473478531268,867.091549898902,140.288112807904));
#84764=CARTESIAN_POINT('Ctrl Pts',(76.3382405129968,867.400029163813,140.39713981778));
#84765=CARTESIAN_POINT('Ctrl Pts',(75.7225070220598,867.69658389792,140.501952294994));
#84766=CARTESIAN_POINT('Ctrl Pts',(78.0657947333568,867.598694356786,140.580266045052));
#84767=CARTESIAN_POINT('Ctrl Pts',(77.4509726650595,867.925667845626,140.695829539433));
#84768=CARTESIAN_POINT('Ctrl Pts',(76.8291206212506,868.240601599858,140.807137784228));
#84769=CARTESIAN_POINT('Ctrl Pts',(76.2005037838652,868.54336131946,140.914143313267));
#84770=CARTESIAN_POINT('Origin',(52.8776183915471,827.175936191914,121.458286566849));
#84771=CARTESIAN_POINT('Ctrl Pts',(63.2008179182801,874.827293699973,143.428853925027));
#84772=CARTESIAN_POINT('Ctrl Pts',(62.5808898780519,874.942399752043,143.469536298538));
#84773=CARTESIAN_POINT('Ctrl Pts',(61.9588939175424,875.047120272489,143.506548073772));
#84774=CARTESIAN_POINT('Ctrl Pts',(61.3350257412051,875.141422312107,143.539877605362));
#84775=CARTESIAN_POINT('Ctrl Pts',(63.3851735065715,875.660694606795,143.880098746674));
#84776=CARTESIAN_POINT('Ctrl Pts',(62.7541745577303,875.777856266129,143.921507641346));
#84777=CARTESIAN_POINT('Ctrl Pts',(62.1210707589078,875.884446925102,143.959180386812));
#84778=CARTESIAN_POINT('Ctrl Pts',(61.4860613095217,875.980433046089,143.993105129741));
#84779=CARTESIAN_POINT('Ctrl Pts',(63.5730314472391,876.495363235131,144.381126406714));
#84780=CARTESIAN_POINT('Ctrl Pts',(62.9307512667703,876.614619553766,144.423275624858));
#84781=CARTESIAN_POINT('Ctrl Pts',(62.2863286050369,876.723115879801,144.461621897544));
#84782=CARTESIAN_POINT('Ctrl Pts',(61.6399662228172,876.820818076015,144.496153159522));
#84783=CARTESIAN_POINT('Origin',(52.8776183915471,827.175936191914,121.458286566849));
#84784=CARTESIAN_POINT('Ctrl Pts',(67.6425933777688,869.801569588793,141.196238235659));
#84785=CARTESIAN_POINT('Ctrl Pts',(66.9957449747181,869.993416316922,141.264043360677));
#84786=CARTESIAN_POINT('Ctrl Pts',(66.3448291753891,870.172616751141,141.327378857528));
#84787=CARTESIAN_POINT('Ctrl Pts',(65.6901240748378,870.339094330465,141.386217666971));
#84788=CARTESIAN_POINT('Ctrl Pts',(67.9507110880758,870.709135201805,141.567772915938));
#84789=CARTESIAN_POINT('Ctrl Pts',(67.2903641556304,870.904985416202,141.636993008463));
#84790=CARTESIAN_POINT('Ctrl Pts',(66.6258649478717,871.087925431933,141.701650199953));
#84791=CARTESIAN_POINT('Ctrl Pts',(65.9574973631851,871.257877090326,141.761716866487));
#84792=CARTESIAN_POINT('Ctrl Pts',(68.2657065447386,871.617715220731,142.002049885831));
#84793=CARTESIAN_POINT('Ctrl Pts',(67.5915597712301,871.817658286473,142.072716530507));
#84794=CARTESIAN_POINT('Ctrl Pts',(66.9131739487192,872.00442135796,142.138724919257));
#84795=CARTESIAN_POINT('Ctrl Pts',(66.2308389084616,872.177924643171,142.200046850881));
#84796=CARTESIAN_POINT('Origin',(52.8776183915471,827.175936191914,121.458286566849));
#84797=CARTESIAN_POINT('Ctrl Pts',(52.1069565671731,875.776490730993,143.765284624484));
#84798=CARTESIAN_POINT('Ctrl Pts',(51.4765013855252,875.767916475681,143.76225419254));
#84799=CARTESIAN_POINT('Ctrl Pts',(50.8463059048213,875.748823152766,143.755505966183));
#84800=CARTESIAN_POINT('Ctrl Pts',(50.2165675427821,875.719216743503,143.745042059391));
#84801=CARTESIAN_POINT('Ctrl Pts',(52.0932323946971,876.624413877709,144.221380036531));
#84802=CARTESIAN_POINT('Ctrl Pts',(51.4515498817118,876.615686929536,144.218295637763));
#84803=CARTESIAN_POINT('Ctrl Pts',(50.8101316945012,876.59625358711,144.211427237006));
#84804=CARTESIAN_POINT('Ctrl Pts',(50.1691787664591,876.566119938201,144.200776985884));
#84805=CARTESIAN_POINT('Ctrl Pts',(52.0792482260038,877.473916293593,144.727097056353));
#84806=CARTESIAN_POINT('Ctrl Pts',(51.4261256866218,877.465033759884,144.723957668392));
#84807=CARTESIAN_POINT('Ctrl Pts',(50.7732721854601,877.445253956481,144.716966816603));
#84808=CARTESIAN_POINT('Ctrl Pts',(50.1208922381873,877.414583079688,144.706126690969));
#84809=CARTESIAN_POINT('Origin',(52.8776183915471,827.175936191914,121.458286566849));
#84810=CARTESIAN_POINT('Ctrl Pts',(57.5979609920746,871.730424908023,141.878222226749));
#84811=CARTESIAN_POINT('Ctrl Pts',(56.9224864915348,871.791797290229,141.899913303207));
#84812=CARTESIAN_POINT('Ctrl Pts',(56.2458102319545,871.83998496928,141.916944459455));
#84813=CARTESIAN_POINT('Ctrl Pts',(55.5682216841954,871.874967331285,141.929308409845));
#84814=CARTESIAN_POINT('Ctrl Pts',(57.6964400038153,872.677944444343,142.264027428917));
#84815=CARTESIAN_POINT('Ctrl Pts',(57.0068732928368,872.740597219109,142.286171039429));
#84816=CARTESIAN_POINT('Ctrl Pts',(56.3160797508998,872.789790222437,142.303557511292));
#84817=CARTESIAN_POINT('Ctrl Pts',(55.6243548880048,872.825502410374,142.316179406861));
#84818=CARTESIAN_POINT('Ctrl Pts',(57.7971166535088,873.627373797714,142.712864928224));
#84819=CARTESIAN_POINT('Ctrl Pts',(57.0931432531388,873.691335538026,142.73547117145));
#84820=CARTESIAN_POINT('Ctrl Pts',(56.3879173903922,873.741556300245,142.75322088808));
#84821=CARTESIAN_POINT('Ctrl Pts',(55.6817407491769,873.778014600765,142.766106485082));
#84822=CARTESIAN_POINT('Origin',(52.8776183915471,827.175936191914,121.458286566849));
#84823=CARTESIAN_POINT('Ctrl Pts',(41.05568276073,874.527241609199,143.322686086998));
#84824=CARTESIAN_POINT('Ctrl Pts',(40.4400310058198,874.395533889448,143.276136122395));
#84825=CARTESIAN_POINT('Ctrl Pts',(39.8269516528412,874.25355950477,143.225957571027));
#84826=CARTESIAN_POINT('Ctrl Pts',(39.2166372801776,874.101363051674,143.172166194807));
#84827=CARTESIAN_POINT('Ctrl Pts',(40.8444331847336,875.355795549055,143.772293777475));
#84828=CARTESIAN_POINT('Ctrl Pts',(40.2177801711254,875.221734306089,143.724911998135));
#84829=CARTESIAN_POINT('Ctrl Pts',(39.5937455264405,875.077222940201,143.673836791766));
#84830=CARTESIAN_POINT('Ctrl Pts',(38.9725252703009,874.922306844807,143.619084201937));
#84831=CARTESIAN_POINT('Ctrl Pts',(40.6291678739282,876.185517036185,144.27170857765));
#84832=CARTESIAN_POINT('Ctrl Pts',(39.9913044739241,876.04905753086,144.223479171246));
#84833=CARTESIAN_POINT('Ctrl Pts',(39.3561062836415,875.901960957186,144.171490264972));
#84834=CARTESIAN_POINT('Ctrl Pts',(38.7237728293571,875.744273520633,144.115758189407));
#84835=CARTESIAN_POINT('Origin',(52.8776183915471,827.175936191914,121.458286566849));
#84836=CARTESIAN_POINT('Ctrl Pts',(47.3453867844678,871.652360600451,141.850744181654));
#84837=CARTESIAN_POINT('Ctrl Pts',(46.6707644356192,871.580401462171,141.825311387387));
#84838=CARTESIAN_POINT('Ctrl Pts',(45.9978656469194,871.495297131312,141.795232637284));
#84839=CARTESIAN_POINT('Ctrl Pts',(45.3269785201039,871.397084045309,141.760520809568));
#84840=CARTESIAN_POINT('Ctrl Pts',(47.2301660207634,872.5966204711,142.235380472072));
#84841=CARTESIAN_POINT('Ctrl Pts',(46.541493193235,872.523162627151,142.209417984512));
#84842=CARTESIAN_POINT('Ctrl Pts',(45.8545798227468,872.436285813379,142.178712778975));
#84843=CARTESIAN_POINT('Ctrl Pts',(45.16972001138,872.336027226107,142.143278001899));
#84844=CARTESIAN_POINT('Ctrl Pts',(47.1123783978066,873.542746553868,142.682824237962));
#84845=CARTESIAN_POINT('Ctrl Pts',(46.4093420785613,873.467756616462,142.656320256735));
#84846=CARTESIAN_POINT('Ctrl Pts',(45.7081019129495,873.379067832847,142.624974639746));
#84847=CARTESIAN_POINT('Ctrl Pts',(45.008958137072,873.276718175141,142.588800807625));
#84848=CARTESIAN_POINT('Origin',(52.8776183915471,827.175936191914,121.458286566849));
#84849=CARTESIAN_POINT('Ctrl Pts',(30.5176874370867,871.137829742988,142.122382291291));
#84850=CARTESIAN_POINT('Ctrl Pts',(29.9434493604142,870.888251874385,142.034173027849));
#84851=CARTESIAN_POINT('Ctrl Pts',(29.3740019118244,870.629100035184,141.942579999254));
#84852=CARTESIAN_POINT('Ctrl Pts',(28.8095246350419,870.360455934569,141.847632084296));
#84853=CARTESIAN_POINT('Ctrl Pts',(30.1182334177546,871.905731565912,142.550119765185));
#84854=CARTESIAN_POINT('Ctrl Pts',(29.5337367357112,871.6516950573,142.460334667502));
#84855=CARTESIAN_POINT('Ctrl Pts',(28.9541162650043,871.387913541738,142.367105354631));
#84856=CARTESIAN_POINT('Ctrl Pts',(28.3795547568576,871.114470188121,142.270461221276));
#84857=CARTESIAN_POINT('Ctrl Pts',(29.7111878117354,872.673653539381,143.027221090879));
#84858=CARTESIAN_POINT('Ctrl Pts',(29.1162375604751,872.41507365472,142.93583021037));
#84859=CARTESIAN_POINT('Ctrl Pts',(28.5262507303067,872.146574476225,142.840933515793));
#84860=CARTESIAN_POINT('Ctrl Pts',(27.9414133409115,871.868240660246,142.742560927566));
#84861=CARTESIAN_POINT('Origin',(52.8776183915471,827.175936191914,121.458286566849));
#84862=CARTESIAN_POINT('Ctrl Pts',(37.3302788892939,869.558176849511,141.109984760151));
#84863=CARTESIAN_POINT('Ctrl Pts',(36.6878228196305,869.3564263923,141.038679322175));
#84864=CARTESIAN_POINT('Ctrl Pts',(36.0499205843609,869.142215425391,140.96296991846));
#84865=CARTESIAN_POINT('Ctrl Pts',(35.4168440128105,868.915635230518,140.88288881106));
#84866=CARTESIAN_POINT('Ctrl Pts',(37.0052885994072,870.462226073617,141.480217953634));
#84867=CARTESIAN_POINT('Ctrl Pts',(36.3494030948049,870.256258371419,141.407421998586));
#84868=CARTESIAN_POINT('Ctrl Pts',(35.6981666146422,870.037569694081,141.330130020498));
#84869=CARTESIAN_POINT('Ctrl Pts',(35.0518566703672,869.806253231424,141.248374955807));
#84870=CARTESIAN_POINT('Ctrl Pts',(36.6730316785943,871.367181199195,141.913359744775));
#84871=CARTESIAN_POINT('Ctrl Pts',(36.003416463167,871.156901956384,141.839039945389));
#84872=CARTESIAN_POINT('Ctrl Pts',(35.3385475906301,870.933635449105,141.760130007306));
#84873=CARTESIAN_POINT('Ctrl Pts',(34.6787083816039,870.69747681793,141.676663556422));
#84874=CARTESIAN_POINT('Origin',(52.8776183915471,827.175936191914,121.458286566849));
#84875=CARTESIAN_POINT('Ctrl Pts',(20.9538218835522,865.756712404766,140.217399249458));
#84876=CARTESIAN_POINT('Ctrl Pts',(20.4480094289833,865.400980192249,140.091671449054));
#84877=CARTESIAN_POINT('Ctrl Pts',(19.9489644671128,865.036850228768,139.962975599315));
#84878=CARTESIAN_POINT('Ctrl Pts',(19.4568438183336,864.664436938889,139.831352141753));
#84879=CARTESIAN_POINT('Ctrl Pts',(20.3821255088437,866.430260973763,140.611649556182));
#84880=CARTESIAN_POINT('Ctrl Pts',(19.8672548851911,866.068158252769,140.483670202531));
#84881=CARTESIAN_POINT('Ctrl Pts',(19.3592729475619,865.697507392565,140.352669647249));
#84882=CARTESIAN_POINT('Ctrl Pts',(18.8583393247131,865.31842486685,140.218689056083));
#84883=CARTESIAN_POINT('Ctrl Pts',(19.7995374347198,867.101999092337,141.054840453057));
#84884=CARTESIAN_POINT('Ctrl Pts',(19.2754360698645,866.733404494836,140.92456665059));
#84885=CARTESIAN_POINT('Ctrl Pts',(18.7583468932775,866.356108504748,140.791217481564));
#84886=CARTESIAN_POINT('Ctrl Pts',(18.248432395584,865.970229683947,140.654834849756));
#84887=CARTESIAN_POINT('Origin',(52.8776183915471,827.175936191914,121.458286566849));
#84888=CARTESIAN_POINT('Ctrl Pts',(28.0016339850113,865.558805254534,139.696003784806));
#84889=CARTESIAN_POINT('Ctrl Pts',(27.4171903968369,865.23579664227,139.581841611962));
#84890=CARTESIAN_POINT('Ctrl Pts',(26.8399476456599,864.901475271192,139.463681127377));
#84891=CARTESIAN_POINT('Ctrl Pts',(26.270152024064,864.555983786442,139.34157274667));
#84892=CARTESIAN_POINT('Ctrl Pts',(27.48299472275,866.377213147581,140.035543517094));
#84893=CARTESIAN_POINT('Ctrl Pts',(26.8863660734158,866.047470130534,139.919001177736));
#84894=CARTESIAN_POINT('Ctrl Pts',(26.2970883912899,865.706178495026,139.798377165856));
#84895=CARTESIAN_POINT('Ctrl Pts',(25.715413103909,865.353483860208,139.67372294819));
#84896=CARTESIAN_POINT('Ctrl Pts',(26.9527888856775,867.194666383688,140.436998441805));
#84897=CARTESIAN_POINT('Ctrl Pts',(26.3437034267223,866.858038772694,140.318022854));
#84898=CARTESIAN_POINT('Ctrl Pts',(25.7421224133561,866.509621423506,140.194880373801));
#84899=CARTESIAN_POINT('Ctrl Pts',(25.148302522587,866.149562995606,140.0676235425));
#84900=CARTESIAN_POINT('Origin',(52.8776183915471,827.175936191914,121.458286566849));
#84901=CARTESIAN_POINT('Ctrl Pts',(12.7865428347925,858.62672781395,137.694349954101));
#84902=CARTESIAN_POINT('Ctrl Pts',(12.3703603268689,858.180246532437,137.536548362142));
#84903=CARTESIAN_POINT('Ctrl Pts',(11.9626324102089,857.726883713927,137.376314602166));
#84904=CARTESIAN_POINT('Ctrl Pts',(11.5634870604064,857.266781657667,137.213698967542));
#84905=CARTESIAN_POINT('Ctrl Pts',(12.0704861765269,859.171290255116,138.042086111739));
#84906=CARTESIAN_POINT('Ctrl Pts',(11.6468703370773,858.716834483271,137.881466065073));
#84907=CARTESIAN_POINT('Ctrl Pts',(11.2318600942279,858.255374265021,137.718370410047));
#84908=CARTESIAN_POINT('Ctrl Pts',(10.8255857093128,857.787054441183,137.552850338305));
#84909=CARTESIAN_POINT('Ctrl Pts',(11.3408233400644,859.711637129034,138.437634367714));
#84910=CARTESIAN_POINT('Ctrl Pts',(10.9096329243531,859.249055339272,138.274142311366));
#84911=CARTESIAN_POINT('Ctrl Pts',(10.4872019799126,858.779343858228,138.10813038088));
#84912=CARTESIAN_POINT('Ctrl Pts',(10.0736630972495,858.302650116585,137.939650683247));
#84913=CARTESIAN_POINT('Origin',(52.8776183915471,827.175936191914,121.458286566849));
#84914=CARTESIAN_POINT('Ctrl Pts',(19.7613090894358,859.806810803219,137.661702909781));
#84915=CARTESIAN_POINT('Ctrl Pts',(19.2595092245227,859.375617365219,137.509304558998));
#84916=CARTESIAN_POINT('Ctrl Pts',(18.7672892142599,858.934717240451,137.353475536676));
#84917=CARTESIAN_POINT('Ctrl Pts',(18.2848602345987,858.484299587218,137.194282697761));
#84918=CARTESIAN_POINT('Ctrl Pts',(19.0699494553796,860.506484585855,137.958487139599));
#84919=CARTESIAN_POINT('Ctrl Pts',(18.557673659474,860.066289246865,137.802907212419));
#84920=CARTESIAN_POINT('Ctrl Pts',(18.0551777140801,859.616184577407,137.64382499256));
#84921=CARTESIAN_POINT('Ctrl Pts',(17.5626772038086,859.156363684789,137.48130873068));
#84922=CARTESIAN_POINT('Ctrl Pts',(18.3631501702965,861.202530292096,138.316374507908));
#84923=CARTESIAN_POINT('Ctrl Pts',(17.8401644917606,860.753132018958,138.157541952411));
#84924=CARTESIAN_POINT('Ctrl Pts',(17.3271631259654,860.293617246153,137.995133883631));
#84925=CARTESIAN_POINT('Ctrl Pts',(16.8243661646366,859.824183118185,137.829219979106));
#84926=CARTESIAN_POINT('Origin',(52.8776183915471,827.175936191914,121.458286566849));
#84927=CARTESIAN_POINT('Ctrl Pts',(6.37745532491532,850.043581143414,134.655040109612));
#84928=CARTESIAN_POINT('Ctrl Pts',(6.06790703385583,849.52418619948,134.471468362258));
#84929=CARTESIAN_POINT('Ctrl Pts',(5.76819589177487,848.999687435667,134.286092752267));
#84930=CARTESIAN_POINT('Ctrl Pts',(5.47841652993691,848.470250458033,134.098971810424));
#84931=CARTESIAN_POINT('Ctrl Pts',(5.54555081826099,850.435760948325,134.948213821533));
#84932=CARTESIAN_POINT('Ctrl Pts',(5.23046459784004,849.907073843545,134.761357910128));
#84933=CARTESIAN_POINT('Ctrl Pts',(4.92539151650234,849.373191609727,134.572665864339));
#84934=CARTESIAN_POINT('Ctrl Pts',(4.63042789849945,848.834282815682,134.382197262089));
#84935=CARTESIAN_POINT('Ctrl Pts',(4.69781197294163,850.820797936038,135.288297996182));
#84936=CARTESIAN_POINT('Ctrl Pts',(4.37708241508856,850.282641804893,135.098095410468));
#84937=CARTESIAN_POINT('Ctrl Pts',(4.06654533619126,849.739197497587,134.906023804368));
#84938=CARTESIAN_POINT('Ctrl Pts',(3.76629878571242,849.190636602077,134.712143822873));
#84939=CARTESIAN_POINT('Origin',(52.8776183915471,827.175936191914,121.458286566849));
#84940=CARTESIAN_POINT('Ctrl Pts',(12.9650774688681,852.569047898116,135.10234465102));
#84941=CARTESIAN_POINT('Ctrl Pts',(12.5693265975477,852.049404581664,134.918685120414));
#84942=CARTESIAN_POINT('Ctrl Pts',(12.1850749352458,851.522145076098,134.732333770876));
#84943=CARTESIAN_POINT('Ctrl Pts',(11.8124873105256,850.987495554614,134.543370539665));
#84944=CARTESIAN_POINT('Ctrl Pts',(12.1299603114578,853.119108286907,135.345529079686));
#84945=CARTESIAN_POINT('Ctrl Pts',(11.7259288763082,852.588592120988,135.158026716186));
#84946=CARTESIAN_POINT('Ctrl Pts',(11.3336372559245,852.050300407265,134.967776211001));
#84947=CARTESIAN_POINT('Ctrl Pts',(10.9532537276901,851.504464051312,134.774859173973));
#84948=CARTESIAN_POINT('Ctrl Pts',(11.2761503952751,853.662144956265,135.648865597357));
#84949=CARTESIAN_POINT('Ctrl Pts',(10.8636530491497,853.120512569574,135.457434385311));
#84950=CARTESIAN_POINT('Ctrl Pts',(10.4631415091117,852.570941709401,135.263197448131));
#84951=CARTESIAN_POINT('Ctrl Pts',(10.0747875785606,852.013668119621,135.066238105679));
#84952=CARTESIAN_POINT('Origin',(52.8776183915471,827.175936191914,121.458286566849));
#84953=CARTESIAN_POINT('Ctrl Pts',(1.99652577628784,840.395005721243,131.239611548762));
#84954=CARTESIAN_POINT('Ctrl Pts',(1.80814586333338,839.826414148728,131.038652048258));
#84955=CARTESIAN_POINT('Ctrl Pts',(1.6305160883364,839.254755063331,130.83660838491));
#84956=CARTESIAN_POINT('Ctrl Pts',(1.46369258826633,838.680209128505,130.633544411295));
#84957=CARTESIAN_POINT('Ctrl Pts',(1.08432921088779,840.615282592914,131.471458943975));
#84958=CARTESIAN_POINT('Ctrl Pts',(0.892572021606208,840.036497306922,131.266896640215));
#84959=CARTESIAN_POINT('Ctrl Pts',(0.711757698826617,839.454589513656,131.061230736733));
#84960=CARTESIAN_POINT('Ctrl Pts',(0.541943385942385,838.869743115505,130.854526230854));
#84961=CARTESIAN_POINT('Ctrl Pts',(0.154732817407261,840.825095759158,131.749222818875));
#84962=CARTESIAN_POINT('Ctrl Pts',(-0.0404660685574277,840.235922318195,
131.540988989657));
#84963=CARTESIAN_POINT('Ctrl Pts',(-0.224525683246545,839.643570326568,
131.331631753086));
#84964=CARTESIAN_POINT('Ctrl Pts',(-0.397387857645575,839.048226987384,
131.121217273072));
#84965=CARTESIAN_POINT('Origin',(52.8776183915471,827.175936191914,121.458286566849));
#84966=CARTESIAN_POINT('Ctrl Pts',(7.91273499456057,844.159523714638,132.128757411956));
#84967=CARTESIAN_POINT('Ctrl Pts',(7.64025937140726,843.574324363908,131.921928160693));
#84968=CARTESIAN_POINT('Ctrl Pts',(7.38069155747312,842.983931954819,131.713263506894));
#84969=CARTESIAN_POINT('Ctrl Pts',(7.13414281207972,842.388599549019,131.502852891109));
#84970=CARTESIAN_POINT('Ctrl Pts',(6.9725451158367,844.533646352629,132.30882139234));
#84971=CARTESIAN_POINT('Ctrl Pts',(6.69437218394524,843.936210819682,132.09766746026));
#84972=CARTESIAN_POINT('Ctrl Pts',(6.42937695614795,843.333473644509,131.884639748432));
#84973=CARTESIAN_POINT('Ctrl Pts',(6.17767301813491,842.725693180133,131.669829567555));
#84974=CARTESIAN_POINT('Ctrl Pts',(6.01132405391079,844.896832714271,132.547534652228));
#84975=CARTESIAN_POINT('Ctrl Pts',(5.72732636972265,844.286887286961,132.331959300197));
#84976=CARTESIAN_POINT('Ctrl Pts',(5.45678232180392,843.671529204637,132.114470932742));
#84977=CARTESIAN_POINT('Ctrl Pts',(5.19980787425188,843.051022230058,131.895162772548));
#84978=CARTESIAN_POINT('Origin',(52.8776183915471,827.175936191914,121.458286566849));
#84979=CARTESIAN_POINT('Ctrl Pts',(-0.162078610920046,830.096471860791,
127.594334646973));
#84980=CARTESIAN_POINT('Ctrl Pts',(-0.220920824684921,829.504313278728,
127.385045767885));
#84981=CARTESIAN_POINT('Ctrl Pts',(-0.268599504446354,828.911262785418,
127.175441657185));
#84982=CARTESIAN_POINT('Ctrl Pts',(-0.305099610353358,828.317507453808,
126.965588432779));
#84983=CARTESIAN_POINT('Ctrl Pts',(-1.11256710860028,830.132360300293,127.760025246802));
#84984=CARTESIAN_POINT('Ctrl Pts',(-1.17246379383695,829.529590045222,127.546985843418));
#84985=CARTESIAN_POINT('Ctrl Pts',(-1.22099689093594,828.925911895566,127.333625559369));
#84986=CARTESIAN_POINT('Ctrl Pts',(-1.25815109052729,828.32151627668,127.120011697418));
#84987=CARTESIAN_POINT('Ctrl Pts',(-2.08117880382292,830.154283943356,127.970323009527));
#84988=CARTESIAN_POINT('Ctrl Pts',(-2.14215006639781,829.540699679902,127.75346156968));
#84989=CARTESIAN_POINT('Ctrl Pts',(-2.19155387221951,828.926191233768,127.536273492403));
#84990=CARTESIAN_POINT('Ctrl Pts',(-2.22937463726006,828.310952446636,127.318827287906));
#84991=CARTESIAN_POINT('Origin',(52.8776183915471,825.559694878252,125.51834395973));
#84992=CARTESIAN_POINT('Origin',(52.8776183915471,826.387310726428,123.689610751183));
#84993=CARTESIAN_POINT('Origin',(52.8776183915471,825.559694878252,125.51834395973));
#84994=CARTESIAN_POINT('Origin',(52.8776183915471,826.387310726428,123.689610751183));
#84995=CARTESIAN_POINT('Origin',(52.8776183915471,825.559694878252,125.51834395973));
#84996=CARTESIAN_POINT('Origin',(52.8776183915471,826.387310726428,123.689610751183));
#84997=CARTESIAN_POINT('Origin',(52.8776183915471,825.559694878252,125.51834395973));
#84998=CARTESIAN_POINT('Origin',(52.8776183915471,826.387310726428,123.689610751183));
#84999=CARTESIAN_POINT('Origin',(52.8776183915471,825.559694878252,125.51834395973));
#85000=CARTESIAN_POINT('Origin',(52.8776183915471,826.387310726428,123.689610751183));
#85001=CARTESIAN_POINT('Origin',(52.8776183915471,825.559694878252,125.51834395973));
#85002=CARTESIAN_POINT('Origin',(52.8776183915471,826.387310726428,123.689610751183));
#130893=UNCERTAINTY_MEASURE_WITH_UNIT(LENGTH_MEASURE(0.01),#130911,
'DISTANCE_ACCURACY_VALUE',
'Maximum model space distance between geometric entities at asserted c
onnectivities');
#130900=UNCERTAINTY_MEASURE_WITH_UNIT(LENGTH_MEASURE(0.01),#130911,
'DISTANCE_ACCURACY_VALUE',
'Maximum model space distance between geometric entities at asserted c
onnectivities');
#130903=(
GEOMETRIC_REPRESENTATION_CONTEXT(3)
GLOBAL_UNCERTAINTY_ASSIGNED_CONTEXT((#130893))
GLOBAL_UNIT_ASSIGNED_CONTEXT((#130911,#130913,#130914))
REPRESENTATION_CONTEXT('','3D')
);
#130910=(
GEOMETRIC_REPRESENTATION_CONTEXT(3)
GLOBAL_UNCERTAINTY_ASSIGNED_CONTEXT((#130900))
GLOBAL_UNIT_ASSIGNED_CONTEXT((#130911,#130913,#130914))
REPRESENTATION_CONTEXT('','3D')
);
#130911=(
LENGTH_UNIT()
NAMED_UNIT(*)
SI_UNIT(.MILLI.,.METRE.)
);
#130913=(
NAMED_UNIT(*)
PLANE_ANGLE_UNIT()
SI_UNIT($,.RADIAN.)
);
#130914=(
NAMED_UNIT(*)
SI_UNIT($,.STERADIAN.)
SOLID_ANGLE_UNIT()
);
#130917=SHAPE_DEFINITION_REPRESENTATION(#130926,#130943);
#130926=PRODUCT_DEFINITION_SHAPE('',$,#130953);
#130943=SHAPE_REPRESENTATION('',(#45568),#130903);
#130950=PRODUCT_DEFINITION_CONTEXT('part definition',#130979,'design');
#130953=PRODUCT_DEFINITION('Component2','Component2',#130962,#130950);
#130962=PRODUCT_DEFINITION_FORMATION('',$,#130983);
#130979=APPLICATION_CONTEXT(
'Core Data for Automotive Mechanical Design Process');
#130980=PRODUCT_CONTEXT('part definition',#130979,'mechanical');
#130983=PRODUCT('Component2','Component2',$,(#130980));
#130991=PRESENTATION_STYLE_ASSIGNMENT((#130993));
#130993=SURFACE_STYLE_USAGE(.BOTH.,#130995);
#130995=SURFACE_SIDE_STYLE('',(#130997));
#130997=SURFACE_STYLE_FILL_AREA(#130999);
#130999=FILL_AREA_STYLE('Opaque(202,209,238)',(#131001));
#131001=FILL_AREA_STYLE_COLOUR('Opaque(202,209,238)',#131003);
#131003=COLOUR_RGB('Opaque(202,209,238)', 0.40784314, 0.44705882, 0.49803922);
ENDSEC;
END-ISO-10303-21;
